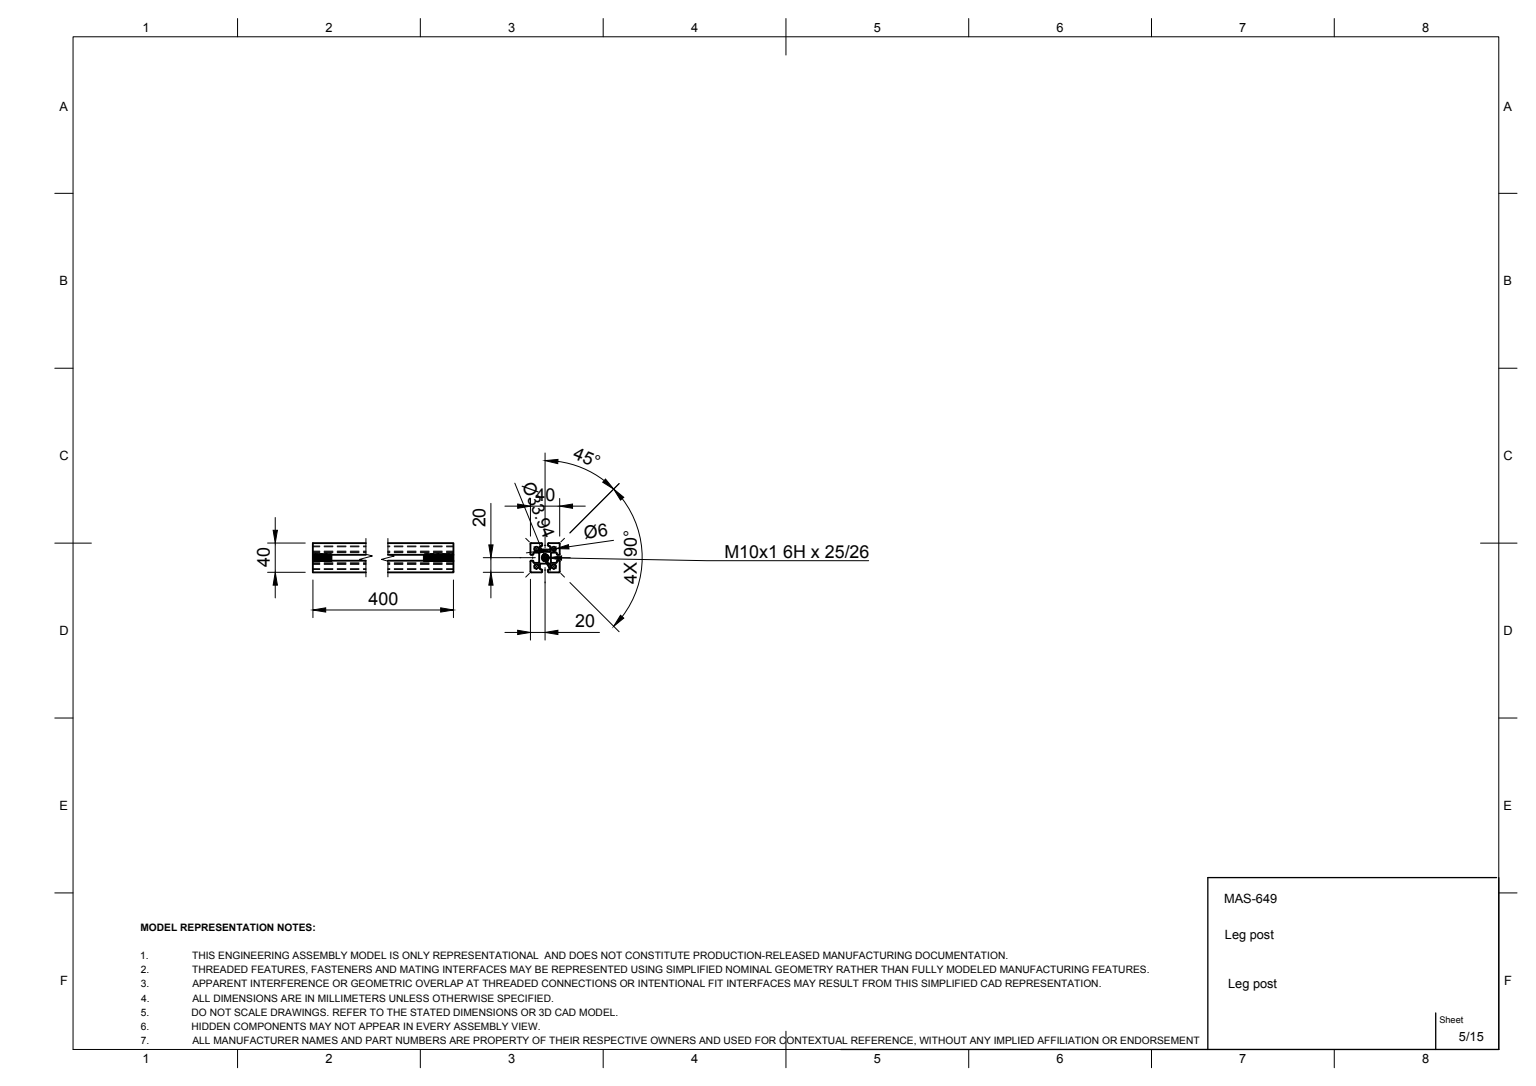
ISO-10303-21;
HEADER;
/* Generated by software containing ST-Developer
 * from STEP Tools, Inc. (www.steptools.com) 
 */

FILE_DESCRIPTION(
/* description */ ('Independent equipment support assembly with bolted 600 x 500 mm welde
d perimeter frame, four adjustable legs and swivel feet. Nominal overa
ll height 518 mm. No load rating assigned.'),
/* implementation_level */ '2;1');

FILE_NAME(
/* name */ 'Leg post.step',
/* time_stamp */ '2026-11-07T17:30:39-08:00',
/* author */ (''),
/* organization */ (''),
/* preprocessor_version */ 'ST-DEVELOPER v20.2',
/* originating_system */ 'Autodesk Translation Framework v15.17.0.0',
/* authorisation */ '');

FILE_SCHEMA (('AUTOMOTIVE_DESIGN { 1 0 10303 214 3 1 1 }'));
ENDSEC;

DATA;
#10=MECHANICAL_DESIGN_GEOMETRIC_PRESENTATION_REPRESENTATION('',(#2213),#63755);
#267=B_SPLINE_SURFACE_WITH_KNOTS('',3,3,((#36107,#36108,#36109,#36110,#36111,
#36112,#36113,#36114,#36115,#36116,#36117,#36118,#36119,#36120,#36121,#36122,
#36123,#36124,#36125,#36126,#36127,#36128,#36129,#36130,#36131,#36132,#36133,
#36134,#36135,#36136,#36137,#36138,#36139,#36140,#36141,#36142,#36143,#36144,
#36145,#36146,#36147,#36148,#36149,#36150,#36151,#36152,#36153,#36154,#36155,
#36156,#36157,#36158,#36159,#36160,#36161,#36162,#36163,#36164,#36165,#36166,
#36167,#36168,#36169,#36170,#36171,#36172,#36173,#36174,#36175,#36176,#36177,
#36178,#36179,#36180,#36181,#36182,#36183,#36184,#36185,#36186,#36187,#36188,
#36189,#36190,#36191,#36192,#36193,#36194,#36195,#36196,#36197,#36198,#36199,
#36200,#36201,#36202,#36203,#36204,#36205,#36206,#36207,#36208,#36209,#36210,
#36211,#36212,#36213,#36214,#36215,#36216,#36217,#36218,#36219,#36220,#36221,
#36222,#36223,#36224,#36225,#36226,#36227,#36228,#36229,#36230,#36231,#36232,
#36233,#36234,#36235,#36236,#36237,#36238,#36239,#36240,#36241,#36242,#36243,
#36244,#36245,#36246,#36247,#36248,#36249,#36250,#36251,#36252,#36253,#36254,
#36255,#36256,#36257,#36258,#36259,#36260,#36261,#36262,#36263,#36264,#36265,
#36266,#36267,#36268,#36269,#36270,#36271,#36272,#36273,#36274,#36275,#36276,
#36277,#36278,#36279,#36280,#36281,#36282,#36283,#36284,#36285,#36286,#36287,
#36288,#36289,#36290,#36291,#36292,#36293,#36294,#36295,#36296,#36297,#36298,
#36299,#36300,#36301,#36302,#36303,#36304,#36305,#36306,#36307,#36308,#36309,
#36310,#36311,#36312,#36313,#36314,#36315,#36316,#36317,#36318,#36319,#36320,
#36321,#36322,#36323,#36324,#36325,#36326,#36327,#36328,#36329,#36330,#36331,
#36332,#36333,#36334,#36335,#36336,#36337,#36338,#36339,#36340,#36341,#36342,
#36343,#36344,#36345,#36346,#36347,#36348,#36349,#36350,#36351,#36352,#36353,
#36354,#36355,#36356,#36357,#36358,#36359,#36360,#36361,#36362,#36363,#36364,
#36365,#36366,#36367,#36368,#36369,#36370,#36371,#36372,#36373,#36374,#36375,
#36376,#36377,#36378,#36379,#36380,#36381,#36382,#36383,#36384,#36385,#36386,
#36387,#36388,#36389,#36390,#36391,#36392,#36393,#36394,#36395,#36396,#36397,
#36398,#36399,#36400,#36401,#36402,#36403,#36404,#36405,#36406,#36407,#36408,
#36409,#36410,#36411,#36412,#36413,#36414,#36415,#36416,#36417,#36418,#36419,
#36420,#36421,#36422,#36423,#36424,#36425,#36426,#36427,#36428,#36429,#36430,
#36431,#36432,#36433,#36434,#36435,#36436,#36437,#36438,#36439,#36440,#36441,
#36442,#36443,#36444,#36445,#36446,#36447,#36448,#36449,#36450,#36451,#36452,
#36453,#36454,#36455,#36456,#36457,#36458,#36459,#36460,#36461,#36462,#36463,
#36464,#36465,#36466,#36467,#36468,#36469,#36470,#36471,#36472,#36473,#36474,
#36475,#36476,#36477,#36478,#36479,#36480,#36481,#36482,#36483,#36484,#36485,
#36486,#36487,#36488,#36489,#36490,#36491,#36492,#36493,#36494,#36495,#36496,
#36497,#36498,#36499,#36500,#36501,#36502,#36503,#36504,#36505,#36506,#36507,
#36508,#36509,#36510,#36511,#36512,#36513,#36514,#36515,#36516,#36517,#36518,
#36519,#36520,#36521,#36522,#36523,#36524,#36525,#36526,#36527,#36528,#36529,
#36530,#36531,#36532,#36533,#36534,#36535,#36536,#36537,#36538,#36539,#36540,
#36541,#36542,#36543,#36544,#36545,#36546,#36547,#36548,#36549,#36550,#36551,
#36552,#36553,#36554,#36555,#36556,#36557,#36558,#36559,#36560,#36561,#36562,
#36563,#36564,#36565,#36566,#36567,#36568,#36569,#36570,#36571,#36572,#36573,
#36574,#36575,#36576,#36577,#36578,#36579,#36580,#36581,#36582,#36583,#36584,
#36585,#36586,#36587,#36588,#36589,#36590,#36591,#36592,#36593,#36594,#36595,
#36596,#36597,#36598,#36599,#36600,#36601,#36602,#36603),(#36604,#36605,
#36606,#36607,#36608,#36609,#36610,#36611,#36612,#36613,#36614,#36615,#36616,
#36617,#36618,#36619,#36620,#36621,#36622,#36623,#36624,#36625,#36626,#36627,
#36628,#36629,#36630,#36631,#36632,#36633,#36634,#36635,#36636,#36637,#36638,
#36639,#36640,#36641,#36642,#36643,#36644,#36645,#36646,#36647,#36648,#36649,
#36650,#36651,#36652,#36653,#36654,#36655,#36656,#36657,#36658,#36659,#36660,
#36661,#36662,#36663,#36664,#36665,#36666,#36667,#36668,#36669,#36670,#36671,
#36672,#36673,#36674,#36675,#36676,#36677,#36678,#36679,#36680,#36681,#36682,
#36683,#36684,#36685,#36686,#36687,#36688,#36689,#36690,#36691,#36692,#36693,
#36694,#36695,#36696,#36697,#36698,#36699,#36700,#36701,#36702,#36703,#36704,
#36705,#36706,#36707,#36708,#36709,#36710,#36711,#36712,#36713,#36714,#36715,
#36716,#36717,#36718,#36719,#36720,#36721,#36722,#36723,#36724,#36725,#36726,
#36727,#36728,#36729,#36730,#36731,#36732,#36733,#36734,#36735,#36736,#36737,
#36738,#36739,#36740,#36741,#36742,#36743,#36744,#36745,#36746,#36747,#36748,
#36749,#36750,#36751,#36752,#36753,#36754,#36755,#36756,#36757,#36758,#36759,
#36760,#36761,#36762,#36763,#36764,#36765,#36766,#36767,#36768,#36769,#36770,
#36771,#36772,#36773,#36774,#36775,#36776,#36777,#36778,#36779,#36780,#36781,
#36782,#36783,#36784,#36785,#36786,#36787,#36788,#36789,#36790,#36791,#36792,
#36793,#36794,#36795,#36796,#36797,#36798,#36799,#36800,#36801,#36802,#36803,
#36804,#36805,#36806,#36807,#36808,#36809,#36810,#36811,#36812,#36813,#36814,
#36815,#36816,#36817,#36818,#36819,#36820,#36821,#36822,#36823,#36824,#36825,
#36826,#36827,#36828,#36829,#36830,#36831,#36832,#36833,#36834,#36835,#36836,
#36837,#36838,#36839,#36840,#36841,#36842,#36843,#36844,#36845,#36846,#36847,
#36848,#36849,#36850,#36851,#36852,#36853,#36854,#36855,#36856,#36857,#36858,
#36859,#36860,#36861,#36862,#36863,#36864,#36865,#36866,#36867,#36868,#36869,
#36870,#36871,#36872,#36873,#36874,#36875,#36876,#36877,#36878,#36879,#36880,
#36881,#36882,#36883,#36884,#36885,#36886,#36887,#36888,#36889,#36890,#36891,
#36892,#36893,#36894,#36895,#36896,#36897,#36898,#36899,#36900,#36901,#36902,
#36903,#36904,#36905,#36906,#36907,#36908,#36909,#36910,#36911,#36912,#36913,
#36914,#36915,#36916,#36917,#36918,#36919,#36920,#36921,#36922,#36923,#36924,
#36925,#36926,#36927,#36928,#36929,#36930,#36931,#36932,#36933,#36934,#36935,
#36936,#36937,#36938,#36939,#36940,#36941,#36942,#36943,#36944,#36945,#36946,
#36947,#36948,#36949,#36950,#36951,#36952,#36953,#36954,#36955,#36956,#36957,
#36958,#36959,#36960,#36961,#36962,#36963,#36964,#36965,#36966,#36967,#36968,
#36969,#36970,#36971,#36972,#36973,#36974,#36975,#36976,#36977,#36978,#36979,
#36980,#36981,#36982,#36983,#36984,#36985,#36986,#36987,#36988,#36989,#36990,
#36991,#36992,#36993,#36994,#36995,#36996,#36997,#36998,#36999,#37000,#37001,
#37002,#37003,#37004,#37005,#37006,#37007,#37008,#37009,#37010,#37011,#37012,
#37013,#37014,#37015,#37016,#37017,#37018,#37019,#37020,#37021,#37022,#37023,
#37024,#37025,#37026,#37027,#37028,#37029,#37030,#37031,#37032,#37033,#37034,
#37035,#37036,#37037,#37038,#37039,#37040,#37041,#37042,#37043,#37044,#37045,
#37046,#37047,#37048,#37049,#37050,#37051,#37052,#37053,#37054,#37055,#37056,
#37057,#37058,#37059,#37060,#37061,#37062,#37063,#37064,#37065,#37066,#37067,
#37068,#37069,#37070,#37071,#37072,#37073,#37074,#37075,#37076,#37077,#37078,
#37079,#37080,#37081,#37082,#37083,#37084,#37085,#37086,#37087,#37088,#37089,
#37090,#37091,#37092,#37093,#37094,#37095,#37096,#37097,#37098,#37099,#37100),
(#37101,#37102,#37103,#37104,#37105,#37106,#37107,#37108,#37109,#37110,
#37111,#37112,#37113,#37114,#37115,#37116,#37117,#37118,#37119,#37120,#37121,
#37122,#37123,#37124,#37125,#37126,#37127,#37128,#37129,#37130,#37131,#37132,
#37133,#37134,#37135,#37136,#37137,#37138,#37139,#37140,#37141,#37142,#37143,
#37144,#37145,#37146,#37147,#37148,#37149,#37150,#37151,#37152,#37153,#37154,
#37155,#37156,#37157,#37158,#37159,#37160,#37161,#37162,#37163,#37164,#37165,
#37166,#37167,#37168,#37169,#37170,#37171,#37172,#37173,#37174,#37175,#37176,
#37177,#37178,#37179,#37180,#37181,#37182,#37183,#37184,#37185,#37186,#37187,
#37188,#37189,#37190,#37191,#37192,#37193,#37194,#37195,#37196,#37197,#37198,
#37199,#37200,#37201,#37202,#37203,#37204,#37205,#37206,#37207,#37208,#37209,
#37210,#37211,#37212,#37213,#37214,#37215,#37216,#37217,#37218,#37219,#37220,
#37221,#37222,#37223,#37224,#37225,#37226,#37227,#37228,#37229,#37230,#37231,
#37232,#37233,#37234,#37235,#37236,#37237,#37238,#37239,#37240,#37241,#37242,
#37243,#37244,#37245,#37246,#37247,#37248,#37249,#37250,#37251,#37252,#37253,
#37254,#37255,#37256,#37257,#37258,#37259,#37260,#37261,#37262,#37263,#37264,
#37265,#37266,#37267,#37268,#37269,#37270,#37271,#37272,#37273,#37274,#37275,
#37276,#37277,#37278,#37279,#37280,#37281,#37282,#37283,#37284,#37285,#37286,
#37287,#37288,#37289,#37290,#37291,#37292,#37293,#37294,#37295,#37296,#37297,
#37298,#37299,#37300,#37301,#37302,#37303,#37304,#37305,#37306,#37307,#37308,
#37309,#37310,#37311,#37312,#37313,#37314,#37315,#37316,#37317,#37318,#37319,
#37320,#37321,#37322,#37323,#37324,#37325,#37326,#37327,#37328,#37329,#37330,
#37331,#37332,#37333,#37334,#37335,#37336,#37337,#37338,#37339,#37340,#37341,
#37342,#37343,#37344,#37345,#37346,#37347,#37348,#37349,#37350,#37351,#37352,
#37353,#37354,#37355,#37356,#37357,#37358,#37359,#37360,#37361,#37362,#37363,
#37364,#37365,#37366,#37367,#37368,#37369,#37370,#37371,#37372,#37373,#37374,
#37375,#37376,#37377,#37378,#37379,#37380,#37381,#37382,#37383,#37384,#37385,
#37386,#37387,#37388,#37389,#37390,#37391,#37392,#37393,#37394,#37395,#37396,
#37397,#37398,#37399,#37400,#37401,#37402,#37403,#37404,#37405,#37406,#37407,
#37408,#37409,#37410,#37411,#37412,#37413,#37414,#37415,#37416,#37417,#37418,
#37419,#37420,#37421,#37422,#37423,#37424,#37425,#37426,#37427,#37428,#37429,
#37430,#37431,#37432,#37433,#37434,#37435,#37436,#37437,#37438,#37439,#37440,
#37441,#37442,#37443,#37444,#37445,#37446,#37447,#37448,#37449,#37450,#37451,
#37452,#37453,#37454,#37455,#37456,#37457,#37458,#37459,#37460,#37461,#37462,
#37463,#37464,#37465,#37466,#37467,#37468,#37469,#37470,#37471,#37472,#37473,
#37474,#37475,#37476,#37477,#37478,#37479,#37480,#37481,#37482,#37483,#37484,
#37485,#37486,#37487,#37488,#37489,#37490,#37491,#37492,#37493,#37494,#37495,
#37496,#37497,#37498,#37499,#37500,#37501,#37502,#37503,#37504,#37505,#37506,
#37507,#37508,#37509,#37510,#37511,#37512,#37513,#37514,#37515,#37516,#37517,
#37518,#37519,#37520,#37521,#37522,#37523,#37524,#37525,#37526,#37527,#37528,
#37529,#37530,#37531,#37532,#37533,#37534,#37535,#37536,#37537,#37538,#37539,
#37540,#37541,#37542,#37543,#37544,#37545,#37546,#37547,#37548,#37549,#37550,
#37551,#37552,#37553,#37554,#37555,#37556,#37557,#37558,#37559,#37560,#37561,
#37562,#37563,#37564,#37565,#37566,#37567,#37568,#37569,#37570,#37571,#37572,
#37573,#37574,#37575,#37576,#37577,#37578,#37579,#37580,#37581,#37582,#37583,
#37584,#37585,#37586,#37587,#37588,#37589,#37590,#37591,#37592,#37593,#37594,
#37595,#37596,#37597),(#37598,#37599,#37600,#37601,#37602,#37603,#37604,
#37605,#37606,#37607,#37608,#37609,#37610,#37611,#37612,#37613,#37614,#37615,
#37616,#37617,#37618,#37619,#37620,#37621,#37622,#37623,#37624,#37625,#37626,
#37627,#37628,#37629,#37630,#37631,#37632,#37633,#37634,#37635,#37636,#37637,
#37638,#37639,#37640,#37641,#37642,#37643,#37644,#37645,#37646,#37647,#37648,
#37649,#37650,#37651,#37652,#37653,#37654,#37655,#37656,#37657,#37658,#37659,
#37660,#37661,#37662,#37663,#37664,#37665,#37666,#37667,#37668,#37669,#37670,
#37671,#37672,#37673,#37674,#37675,#37676,#37677,#37678,#37679,#37680,#37681,
#37682,#37683,#37684,#37685,#37686,#37687,#37688,#37689,#37690,#37691,#37692,
#37693,#37694,#37695,#37696,#37697,#37698,#37699,#37700,#37701,#37702,#37703,
#37704,#37705,#37706,#37707,#37708,#37709,#37710,#37711,#37712,#37713,#37714,
#37715,#37716,#37717,#37718,#37719,#37720,#37721,#37722,#37723,#37724,#37725,
#37726,#37727,#37728,#37729,#37730,#37731,#37732,#37733,#37734,#37735,#37736,
#37737,#37738,#37739,#37740,#37741,#37742,#37743,#37744,#37745,#37746,#37747,
#37748,#37749,#37750,#37751,#37752,#37753,#37754,#37755,#37756,#37757,#37758,
#37759,#37760,#37761,#37762,#37763,#37764,#37765,#37766,#37767,#37768,#37769,
#37770,#37771,#37772,#37773,#37774,#37775,#37776,#37777,#37778,#37779,#37780,
#37781,#37782,#37783,#37784,#37785,#37786,#37787,#37788,#37789,#37790,#37791,
#37792,#37793,#37794,#37795,#37796,#37797,#37798,#37799,#37800,#37801,#37802,
#37803,#37804,#37805,#37806,#37807,#37808,#37809,#37810,#37811,#37812,#37813,
#37814,#37815,#37816,#37817,#37818,#37819,#37820,#37821,#37822,#37823,#37824,
#37825,#37826,#37827,#37828,#37829,#37830,#37831,#37832,#37833,#37834,#37835,
#37836,#37837,#37838,#37839,#37840,#37841,#37842,#37843,#37844,#37845,#37846,
#37847,#37848,#37849,#37850,#37851,#37852,#37853,#37854,#37855,#37856,#37857,
#37858,#37859,#37860,#37861,#37862,#37863,#37864,#37865,#37866,#37867,#37868,
#37869,#37870,#37871,#37872,#37873,#37874,#37875,#37876,#37877,#37878,#37879,
#37880,#37881,#37882,#37883,#37884,#37885,#37886,#37887,#37888,#37889,#37890,
#37891,#37892,#37893,#37894,#37895,#37896,#37897,#37898,#37899,#37900,#37901,
#37902,#37903,#37904,#37905,#37906,#37907,#37908,#37909,#37910,#37911,#37912,
#37913,#37914,#37915,#37916,#37917,#37918,#37919,#37920,#37921,#37922,#37923,
#37924,#37925,#37926,#37927,#37928,#37929,#37930,#37931,#37932,#37933,#37934,
#37935,#37936,#37937,#37938,#37939,#37940,#37941,#37942,#37943,#37944,#37945,
#37946,#37947,#37948,#37949,#37950,#37951,#37952,#37953,#37954,#37955,#37956,
#37957,#37958,#37959,#37960,#37961,#37962,#37963,#37964,#37965,#37966,#37967,
#37968,#37969,#37970,#37971,#37972,#37973,#37974,#37975,#37976,#37977,#37978,
#37979,#37980,#37981,#37982,#37983,#37984,#37985,#37986,#37987,#37988,#37989,
#37990,#37991,#37992,#37993,#37994,#37995,#37996,#37997,#37998,#37999,#38000,
#38001,#38002,#38003,#38004,#38005,#38006,#38007,#38008,#38009,#38010,#38011,
#38012,#38013,#38014,#38015,#38016,#38017,#38018,#38019,#38020,#38021,#38022,
#38023,#38024,#38025,#38026,#38027,#38028,#38029,#38030,#38031,#38032,#38033,
#38034,#38035,#38036,#38037,#38038,#38039,#38040,#38041,#38042,#38043,#38044,
#38045,#38046,#38047,#38048,#38049,#38050,#38051,#38052,#38053,#38054,#38055,
#38056,#38057,#38058,#38059,#38060,#38061,#38062,#38063,#38064,#38065,#38066,
#38067,#38068,#38069,#38070,#38071,#38072,#38073,#38074,#38075,#38076,#38077,
#38078,#38079,#38080,#38081,#38082,#38083,#38084,#38085,#38086,#38087,#38088,
#38089,#38090,#38091,#38092,#38093,#38094)),.UNSPECIFIED.,.F.,.F.,.F.,(4,
4),(4,1,1,1,1,1,1,1,1,1,1,1,1,1,1,1,1,1,1,1,1,1,1,1,1,1,1,1,1,1,1,1,1,1,
1,1,1,1,1,1,1,1,1,1,1,1,1,1,1,1,1,1,1,1,1,1,1,1,1,1,1,1,1,1,1,1,1,1,1,1,
1,1,1,1,1,1,1,1,1,1,1,1,1,1,1,1,1,1,1,1,1,1,1,1,1,1,1,1,1,1,1,1,1,1,1,1,
1,1,1,1,1,1,1,1,1,1,1,1,1,1,1,1,1,1,1,1,1,1,1,1,1,1,1,1,1,1,1,1,1,1,1,1,
1,1,1,1,1,1,1,1,1,1,1,1,1,1,1,1,1,1,1,1,1,1,1,1,1,1,1,1,1,1,1,1,1,1,1,1,
1,1,1,1,1,1,1,1,1,1,1,1,1,1,1,1,1,1,1,1,1,1,1,1,1,1,1,1,1,1,1,1,1,1,1,1,
1,1,1,1,1,1,1,1,1,1,1,1,1,1,1,1,1,1,1,1,1,1,1,1,1,1,1,1,1,1,1,1,1,1,1,1,
1,1,1,1,1,1,1,1,1,1,1,1,1,1,1,1,1,1,1,1,1,1,1,1,1,1,1,1,1,1,1,1,1,1,1,1,
1,1,1,1,1,1,1,1,1,1,1,1,1,1,1,1,1,1,1,1,1,1,1,1,1,1,1,1,1,1,1,1,1,1,1,1,
1,1,1,1,1,1,1,1,1,1,1,1,1,1,1,1,1,1,1,1,1,1,1,1,1,1,1,1,1,1,1,1,1,1,1,1,
1,1,1,1,1,1,1,1,1,1,1,1,1,1,1,1,1,1,1,1,1,1,1,1,1,1,1,1,1,1,1,1,1,1,1,1,
1,1,1,1,1,1,1,1,1,1,1,1,1,1,1,1,1,1,1,1,1,1,1,1,1,1,1,1,1,1,1,1,1,1,1,1,
1,1,1,1,1,1,1,1,1,1,1,1,1,1,1,1,1,1,1,1,1,1,1,1,1,1,1,1,1,1,1,1,1,1,1,1,
1,1,1,1,1,1,1,1,1,1,1,1,1,1,1,1,1,1,1,1,1,1,1,1,1,1,1,1,4),(0.,0.0641840294258107),
(11.8589888623082,12.3576971556948,12.8564054490814,13.355113742468,13.8538220358547,
14.3525303292413,14.8512386226279,15.3499469160145,15.8486552094011,16.3473635027878,
16.8460717961744,17.344780089561,17.8434883829476,18.3421966763342,18.8409049697209,
19.3396132631075,19.8383215564941,20.3370298498807,20.8357381432673,21.334446436654,
21.8331547300406,22.3318630234272,22.8305713168138,23.3292796102004,23.8279879035871,
24.3266961969737,24.8254044903603,25.3241127837469,25.8228210771335,26.3215293705201,
26.8202376639068,27.3189459572934,27.81765425068,28.3163625440666,28.8150708374532,
29.3137791308399,29.8124874242265,30.3111957176131,30.8099040109997,31.3086123043863,
31.807320597773,32.3060288911596,32.8047371845462,33.3034454779328,33.8021537713194,
34.3008620647061,34.7995703580927,35.2982786514793,35.7969869448659,36.2956952382525,
36.7944035316392,37.2931118250258,37.7918201184124,38.290528411799,38.7892367051856,
39.2879449985723,39.7866532919589,40.2853615853455,40.7840698787321,41.2827781721187,
41.7814864655054,42.280194758892,42.7789030522786,43.2776113456652,43.7763196390518,
44.2750279324384,44.7737362258251,45.2724445192117,45.7711528125983,46.2698611059849,
46.7685693993716,47.2672776927582,47.7659859861448,48.2646942795314,48.763402572918,
49.2621108663046,49.7608191596913,50.2595274530779,50.7582357464645,51.2569440398511,
51.7556523332377,52.2543606266244,52.753068920011,53.2517772133976,53.7504855067842,
54.2491938001708,54.7479020935575,55.2466103869441,55.7453186803307,56.2440269737173,
56.7427352671039,57.2414435604906,57.7401518538772,58.2388601472638,58.7375684406504,
59.236276734037,59.7349850274237,60.2336933208103,60.7324016141969,61.2311099075835,
61.7298182009701,62.2285264943567,62.7272347877434,63.22594308113,63.7246513745166,
64.2233596679032,64.7220679612898,65.2207762546765,65.7194845480631,66.2181928414497,
66.7169011348363,67.2156094282229,67.7143177216096,68.2130260149962,68.7117343083828,
69.2104426017694,69.709150895156,70.2078591885427,70.7065674819293,71.2052757753159,
71.7039840687025,72.2026923620891,72.7014006554758,73.2001089488624,73.698817242249,
74.1975255356356,74.6962338290222,75.1949421224089,75.6936504157955,76.1923587091821,
76.6910670025687,77.1897752959553,77.6884835893419,78.1871918827286,78.6859001761152,
79.1846084695018,79.6833167628884,80.1820250562751,80.6807333496617,81.1794416430483,
81.6781499364349,82.1768582298215,82.6755665232081,83.1742748165948,83.6729831099814,
84.171691403368,84.6703996967546,85.1691079901412,85.6678162835279,86.1665245769145,
86.6652328703011,87.1639411636877,87.6626494570743,88.161357750461,88.6600660438476,
89.1587743372342,89.6574826306208,90.1561909240074,90.654899217394,91.1536075107807,
91.6523158041673,92.1510240975539,92.6497323909405,93.1484406843271,93.6471489777138,
94.1458572711004,94.644565564487,95.1432738578736,95.6419821512603,96.1406904446469,
96.6393987380335,97.1381070314201,97.6368153248067,98.1355236181933,98.63423191158,
99.1329402049666,99.6316484983532,100.13035679174,100.629065085126,101.127773378513,
101.6264816719,102.125189965286,102.623898258673,103.12260655206,103.621314845446,
104.120023138833,104.618731432219,105.117439725606,105.616148018993,106.114856312379,
106.613564605766,107.112272899152,107.610981192539,108.109689485926,108.608397779312,
109.107106072699,109.605814366086,110.104522659472,110.603230952859,111.101939246245,
111.600647539632,112.099355833019,112.598064126405,113.096772419792,113.595480713179,
114.094189006565,114.592897299952,115.091605593338,115.590313886725,116.089022180112,
116.587730473498,117.086438766885,117.585147060271,118.083855353658,118.582563647045,
119.081271940431,119.579980233818,120.078688527205,120.577396820591,121.076105113978,
121.574813407364,122.073521700751,122.572229994138,123.070938287524,123.569646580911,
124.068354874298,124.567063167684,125.065771461071,125.564479754457,126.063188047844,
126.561896341231,127.060604634617,127.559312928004,128.058021221391,128.556729514777,
129.055437808164,129.55414610155,130.052854394937,130.551562688324,131.05027098171,
131.548979275097,132.54639586187,133.543812448643,134.541229035417,135.53864562219,
136.536062208963,137.533478795736,138.53089538251,139.528311969283,140.525728556056,
141.523145142829,142.520561729602,143.517978316376,144.515394903149,145.512811489922,
146.011519783309,146.510228076695,147.008936370082,147.507644663469,148.006352956855,
148.505061250242,149.003769543629,149.502477837015,150.001186130402,150.499894423788,
150.998602717175,151.497311010562,151.996019303948,152.494727597335,152.993435890721,
153.492144184108,153.990852477495,154.489560770881,154.988269064268,155.486977357655,
155.985685651041,156.484393944428,156.983102237814,157.481810531201,157.980518824588,
158.479227117974,158.977935411361,159.476643704748,159.975351998134,160.474060291521,
160.972768584907,161.471476878294,161.970185171681,162.468893465067,162.967601758454,
163.466310051841,163.965018345227,164.463726638614,164.962434932,165.461143225387,
165.959851518774,166.45855981216,166.957268105547,167.455976398933,167.95468469232,
168.453392985707,168.952101279093,169.45080957248,169.949517865867,170.448226159253,
170.94693445264,171.445642746026,171.944351039413,172.4430593328,172.941767626186,
173.440475919573,173.93918421296,174.437892506346,174.936600799733,175.435309093119,
175.934017386506,176.432725679893,176.931433973279,177.430142266666,177.928850560052,
178.427558853439,178.926267146826,179.424975440212,179.923683733599,180.422392026986,
180.921100320372,181.419808613759,181.918516907145,182.417225200532,182.915933493919,
183.414641787305,183.913350080692,184.412058374079,184.910766667465,185.409474960852,
185.908183254238,186.406891547625,186.905599841012,187.404308134398,187.903016427785,
188.401724721171,188.900433014558,189.399141307945,189.897849601331,190.396557894718,
190.895266188105,191.393974481491,191.892682774878,192.391391068264,192.890099361651,
193.388807655038,193.887515948424,194.386224241811,194.884932535198,195.383640828584,
195.882349121971,196.381057415357,196.879765708744,197.378474002131,197.877182295517,
198.375890588904,198.87459888229,199.373307175677,199.872015469064,200.37072376245,
200.869432055837,201.368140349224,201.86684864261,202.365556935997,202.864265229383,
203.36297352277,203.861681816157,204.360390109543,204.85909840293,205.357806696317,
205.856514989703,206.35522328309,206.853931576476,207.352639869863,207.85134816325,
208.350056456636,208.848764750023,209.347473043409,209.846181336796,210.344889630183,
210.843597923569,211.342306216956,211.841014510343,212.339722803729,212.838431097116,
213.337139390502,213.835847683889,214.334555977276,214.833264270662,215.331972564049,
215.830680857436,216.329389150822,216.828097444209,217.326805737595,217.825514030982,
218.324222324369,218.822930617755,219.321638911142,219.820347204529,220.319055497915,
220.817763791302,221.316472084688,221.815180378075,222.313888671462,222.812596964848,
223.311305258235,223.810013551621,224.308721845008,224.807430138395,225.306138431781,
225.804846725168,226.303555018555,226.802263311941,227.300971605328,227.799679898714,
228.298388192101,228.797096485488,229.295804778874,229.794513072261,230.293221365647,
230.791929659034,231.290637952421,231.789346245807,232.288054539194,232.786762832581,
233.285471125967,233.784179419354,234.28288771274,234.781596006127,235.280304299514,
235.7790125929,236.277720886287,236.776429179674,237.27513747306,237.773845766447,
238.272554059833,238.77126235322,239.269970646607,239.768678939993,240.26738723338,
240.766095526767,241.264803820153,241.76351211354,242.262220406926,242.760928700313,
243.2596369937,243.758345287086,244.257053580473,244.755761873859,245.254470167246,
245.753178460633,246.251886754019,246.750595047406,247.249303340793,247.748011634179,
248.246719927566,248.745428220952,249.244136514339,249.742844807726,250.241553101112,
250.740261394499,251.238969687886,251.737677981272,252.236386274659,252.735094568045,
253.233802861432,253.732511154819,254.231219448205,254.729927741592,255.228636034978,
255.727344328365,256.226052621752,256.724760915138,257.223469208525,257.722177501912,
258.220885795298,258.719594088685,259.218302382071,259.717010675458,260.215718968845,
260.714427262231,261.213135555618,261.711843849004,262.210552142391,262.709260435778,
263.207968729164,263.706677022551,264.205385315938,264.704093609324,265.202801902711),
 .UNSPECIFIED.);
#268=B_SPLINE_SURFACE_WITH_KNOTS('',3,3,((#38244,#38245,#38246,#38247,#38248,
#38249,#38250,#38251,#38252,#38253,#38254,#38255,#38256,#38257,#38258,#38259,
#38260,#38261,#38262,#38263,#38264,#38265,#38266,#38267,#38268,#38269,#38270,
#38271,#38272,#38273,#38274,#38275,#38276,#38277,#38278,#38279,#38280,#38281,
#38282,#38283,#38284,#38285,#38286,#38287,#38288,#38289,#38290,#38291,#38292,
#38293,#38294,#38295,#38296,#38297,#38298,#38299,#38300,#38301,#38302,#38303,
#38304,#38305,#38306,#38307,#38308,#38309,#38310,#38311,#38312,#38313,#38314,
#38315,#38316,#38317,#38318,#38319,#38320,#38321,#38322,#38323,#38324,#38325,
#38326,#38327,#38328,#38329,#38330,#38331,#38332,#38333,#38334,#38335,#38336,
#38337,#38338,#38339,#38340,#38341,#38342,#38343,#38344,#38345,#38346,#38347,
#38348,#38349,#38350,#38351,#38352,#38353,#38354,#38355,#38356,#38357,#38358,
#38359,#38360,#38361,#38362,#38363,#38364,#38365,#38366,#38367,#38368,#38369,
#38370,#38371,#38372,#38373,#38374,#38375,#38376,#38377,#38378,#38379,#38380,
#38381,#38382,#38383,#38384,#38385,#38386,#38387,#38388,#38389,#38390,#38391,
#38392,#38393,#38394,#38395,#38396,#38397,#38398,#38399,#38400,#38401,#38402,
#38403,#38404,#38405,#38406,#38407,#38408,#38409,#38410,#38411,#38412,#38413,
#38414,#38415,#38416,#38417,#38418,#38419,#38420,#38421,#38422,#38423,#38424,
#38425,#38426,#38427,#38428,#38429,#38430,#38431,#38432,#38433,#38434,#38435,
#38436,#38437,#38438,#38439,#38440,#38441,#38442,#38443,#38444,#38445,#38446,
#38447,#38448,#38449,#38450,#38451,#38452,#38453,#38454,#38455,#38456,#38457,
#38458,#38459,#38460,#38461,#38462,#38463,#38464,#38465,#38466,#38467,#38468,
#38469,#38470,#38471,#38472,#38473,#38474,#38475,#38476,#38477,#38478,#38479,
#38480,#38481,#38482,#38483,#38484,#38485,#38486,#38487,#38488,#38489,#38490,
#38491,#38492,#38493,#38494,#38495,#38496,#38497,#38498,#38499,#38500,#38501,
#38502,#38503,#38504,#38505,#38506,#38507,#38508,#38509,#38510,#38511,#38512,
#38513,#38514,#38515,#38516,#38517,#38518,#38519,#38520,#38521,#38522,#38523,
#38524,#38525,#38526,#38527,#38528,#38529,#38530,#38531,#38532,#38533,#38534,
#38535,#38536,#38537,#38538,#38539,#38540,#38541,#38542,#38543,#38544,#38545,
#38546,#38547,#38548,#38549,#38550,#38551,#38552,#38553,#38554,#38555,#38556,
#38557,#38558,#38559,#38560,#38561,#38562,#38563,#38564,#38565,#38566,#38567,
#38568,#38569,#38570,#38571,#38572,#38573,#38574,#38575,#38576,#38577,#38578,
#38579,#38580,#38581,#38582,#38583,#38584,#38585,#38586,#38587,#38588,#38589,
#38590,#38591,#38592,#38593,#38594,#38595,#38596,#38597,#38598,#38599,#38600,
#38601,#38602,#38603,#38604,#38605,#38606,#38607,#38608,#38609,#38610,#38611,
#38612,#38613,#38614,#38615,#38616,#38617,#38618,#38619,#38620,#38621,#38622,
#38623,#38624,#38625,#38626,#38627,#38628,#38629,#38630,#38631,#38632,#38633,
#38634,#38635,#38636,#38637,#38638,#38639,#38640,#38641,#38642,#38643,#38644,
#38645,#38646,#38647,#38648,#38649,#38650,#38651,#38652,#38653,#38654,#38655,
#38656,#38657,#38658,#38659,#38660,#38661,#38662,#38663,#38664,#38665,#38666,
#38667,#38668,#38669,#38670,#38671,#38672,#38673,#38674,#38675,#38676,#38677,
#38678,#38679,#38680,#38681,#38682,#38683,#38684,#38685,#38686,#38687,#38688,
#38689,#38690,#38691,#38692,#38693,#38694,#38695,#38696,#38697,#38698,#38699,
#38700,#38701,#38702,#38703,#38704,#38705,#38706,#38707,#38708,#38709,#38710,
#38711,#38712,#38713,#38714,#38715,#38716,#38717,#38718,#38719,#38720,#38721,
#38722,#38723,#38724,#38725,#38726,#38727,#38728,#38729,#38730,#38731,#38732,
#38733,#38734,#38735,#38736,#38737,#38738,#38739,#38740),(#38741,#38742,
#38743,#38744,#38745,#38746,#38747,#38748,#38749,#38750,#38751,#38752,#38753,
#38754,#38755,#38756,#38757,#38758,#38759,#38760,#38761,#38762,#38763,#38764,
#38765,#38766,#38767,#38768,#38769,#38770,#38771,#38772,#38773,#38774,#38775,
#38776,#38777,#38778,#38779,#38780,#38781,#38782,#38783,#38784,#38785,#38786,
#38787,#38788,#38789,#38790,#38791,#38792,#38793,#38794,#38795,#38796,#38797,
#38798,#38799,#38800,#38801,#38802,#38803,#38804,#38805,#38806,#38807,#38808,
#38809,#38810,#38811,#38812,#38813,#38814,#38815,#38816,#38817,#38818,#38819,
#38820,#38821,#38822,#38823,#38824,#38825,#38826,#38827,#38828,#38829,#38830,
#38831,#38832,#38833,#38834,#38835,#38836,#38837,#38838,#38839,#38840,#38841,
#38842,#38843,#38844,#38845,#38846,#38847,#38848,#38849,#38850,#38851,#38852,
#38853,#38854,#38855,#38856,#38857,#38858,#38859,#38860,#38861,#38862,#38863,
#38864,#38865,#38866,#38867,#38868,#38869,#38870,#38871,#38872,#38873,#38874,
#38875,#38876,#38877,#38878,#38879,#38880,#38881,#38882,#38883,#38884,#38885,
#38886,#38887,#38888,#38889,#38890,#38891,#38892,#38893,#38894,#38895,#38896,
#38897,#38898,#38899,#38900,#38901,#38902,#38903,#38904,#38905,#38906,#38907,
#38908,#38909,#38910,#38911,#38912,#38913,#38914,#38915,#38916,#38917,#38918,
#38919,#38920,#38921,#38922,#38923,#38924,#38925,#38926,#38927,#38928,#38929,
#38930,#38931,#38932,#38933,#38934,#38935,#38936,#38937,#38938,#38939,#38940,
#38941,#38942,#38943,#38944,#38945,#38946,#38947,#38948,#38949,#38950,#38951,
#38952,#38953,#38954,#38955,#38956,#38957,#38958,#38959,#38960,#38961,#38962,
#38963,#38964,#38965,#38966,#38967,#38968,#38969,#38970,#38971,#38972,#38973,
#38974,#38975,#38976,#38977,#38978,#38979,#38980,#38981,#38982,#38983,#38984,
#38985,#38986,#38987,#38988,#38989,#38990,#38991,#38992,#38993,#38994,#38995,
#38996,#38997,#38998,#38999,#39000,#39001,#39002,#39003,#39004,#39005,#39006,
#39007,#39008,#39009,#39010,#39011,#39012,#39013,#39014,#39015,#39016,#39017,
#39018,#39019,#39020,#39021,#39022,#39023,#39024,#39025,#39026,#39027,#39028,
#39029,#39030,#39031,#39032,#39033,#39034,#39035,#39036,#39037,#39038,#39039,
#39040,#39041,#39042,#39043,#39044,#39045,#39046,#39047,#39048,#39049,#39050,
#39051,#39052,#39053,#39054,#39055,#39056,#39057,#39058,#39059,#39060,#39061,
#39062,#39063,#39064,#39065,#39066,#39067,#39068,#39069,#39070,#39071,#39072,
#39073,#39074,#39075,#39076,#39077,#39078,#39079,#39080,#39081,#39082,#39083,
#39084,#39085,#39086,#39087,#39088,#39089,#39090,#39091,#39092,#39093,#39094,
#39095,#39096,#39097,#39098,#39099,#39100,#39101,#39102,#39103,#39104,#39105,
#39106,#39107,#39108,#39109,#39110,#39111,#39112,#39113,#39114,#39115,#39116,
#39117,#39118,#39119,#39120,#39121,#39122,#39123,#39124,#39125,#39126,#39127,
#39128,#39129,#39130,#39131,#39132,#39133,#39134,#39135,#39136,#39137,#39138,
#39139,#39140,#39141,#39142,#39143,#39144,#39145,#39146,#39147,#39148,#39149,
#39150,#39151,#39152,#39153,#39154,#39155,#39156,#39157,#39158,#39159,#39160,
#39161,#39162,#39163,#39164,#39165,#39166,#39167,#39168,#39169,#39170,#39171,
#39172,#39173,#39174,#39175,#39176,#39177,#39178,#39179,#39180,#39181,#39182,
#39183,#39184,#39185,#39186,#39187,#39188,#39189,#39190,#39191,#39192,#39193,
#39194,#39195,#39196,#39197,#39198,#39199,#39200,#39201,#39202,#39203,#39204,
#39205,#39206,#39207,#39208,#39209,#39210,#39211,#39212,#39213,#39214,#39215,
#39216,#39217,#39218,#39219,#39220,#39221,#39222,#39223,#39224,#39225,#39226,
#39227,#39228,#39229,#39230,#39231,#39232,#39233,#39234,#39235,#39236,#39237),
(#39238,#39239,#39240,#39241,#39242,#39243,#39244,#39245,#39246,#39247,
#39248,#39249,#39250,#39251,#39252,#39253,#39254,#39255,#39256,#39257,#39258,
#39259,#39260,#39261,#39262,#39263,#39264,#39265,#39266,#39267,#39268,#39269,
#39270,#39271,#39272,#39273,#39274,#39275,#39276,#39277,#39278,#39279,#39280,
#39281,#39282,#39283,#39284,#39285,#39286,#39287,#39288,#39289,#39290,#39291,
#39292,#39293,#39294,#39295,#39296,#39297,#39298,#39299,#39300,#39301,#39302,
#39303,#39304,#39305,#39306,#39307,#39308,#39309,#39310,#39311,#39312,#39313,
#39314,#39315,#39316,#39317,#39318,#39319,#39320,#39321,#39322,#39323,#39324,
#39325,#39326,#39327,#39328,#39329,#39330,#39331,#39332,#39333,#39334,#39335,
#39336,#39337,#39338,#39339,#39340,#39341,#39342,#39343,#39344,#39345,#39346,
#39347,#39348,#39349,#39350,#39351,#39352,#39353,#39354,#39355,#39356,#39357,
#39358,#39359,#39360,#39361,#39362,#39363,#39364,#39365,#39366,#39367,#39368,
#39369,#39370,#39371,#39372,#39373,#39374,#39375,#39376,#39377,#39378,#39379,
#39380,#39381,#39382,#39383,#39384,#39385,#39386,#39387,#39388,#39389,#39390,
#39391,#39392,#39393,#39394,#39395,#39396,#39397,#39398,#39399,#39400,#39401,
#39402,#39403,#39404,#39405,#39406,#39407,#39408,#39409,#39410,#39411,#39412,
#39413,#39414,#39415,#39416,#39417,#39418,#39419,#39420,#39421,#39422,#39423,
#39424,#39425,#39426,#39427,#39428,#39429,#39430,#39431,#39432,#39433,#39434,
#39435,#39436,#39437,#39438,#39439,#39440,#39441,#39442,#39443,#39444,#39445,
#39446,#39447,#39448,#39449,#39450,#39451,#39452,#39453,#39454,#39455,#39456,
#39457,#39458,#39459,#39460,#39461,#39462,#39463,#39464,#39465,#39466,#39467,
#39468,#39469,#39470,#39471,#39472,#39473,#39474,#39475,#39476,#39477,#39478,
#39479,#39480,#39481,#39482,#39483,#39484,#39485,#39486,#39487,#39488,#39489,
#39490,#39491,#39492,#39493,#39494,#39495,#39496,#39497,#39498,#39499,#39500,
#39501,#39502,#39503,#39504,#39505,#39506,#39507,#39508,#39509,#39510,#39511,
#39512,#39513,#39514,#39515,#39516,#39517,#39518,#39519,#39520,#39521,#39522,
#39523,#39524,#39525,#39526,#39527,#39528,#39529,#39530,#39531,#39532,#39533,
#39534,#39535,#39536,#39537,#39538,#39539,#39540,#39541,#39542,#39543,#39544,
#39545,#39546,#39547,#39548,#39549,#39550,#39551,#39552,#39553,#39554,#39555,
#39556,#39557,#39558,#39559,#39560,#39561,#39562,#39563,#39564,#39565,#39566,
#39567,#39568,#39569,#39570,#39571,#39572,#39573,#39574,#39575,#39576,#39577,
#39578,#39579,#39580,#39581,#39582,#39583,#39584,#39585,#39586,#39587,#39588,
#39589,#39590,#39591,#39592,#39593,#39594,#39595,#39596,#39597,#39598,#39599,
#39600,#39601,#39602,#39603,#39604,#39605,#39606,#39607,#39608,#39609,#39610,
#39611,#39612,#39613,#39614,#39615,#39616,#39617,#39618,#39619,#39620,#39621,
#39622,#39623,#39624,#39625,#39626,#39627,#39628,#39629,#39630,#39631,#39632,
#39633,#39634,#39635,#39636,#39637,#39638,#39639,#39640,#39641,#39642,#39643,
#39644,#39645,#39646,#39647,#39648,#39649,#39650,#39651,#39652,#39653,#39654,
#39655,#39656,#39657,#39658,#39659,#39660,#39661,#39662,#39663,#39664,#39665,
#39666,#39667,#39668,#39669,#39670,#39671,#39672,#39673,#39674,#39675,#39676,
#39677,#39678,#39679,#39680,#39681,#39682,#39683,#39684,#39685,#39686,#39687,
#39688,#39689,#39690,#39691,#39692,#39693,#39694,#39695,#39696,#39697,#39698,
#39699,#39700,#39701,#39702,#39703,#39704,#39705,#39706,#39707,#39708,#39709,
#39710,#39711,#39712,#39713,#39714,#39715,#39716,#39717,#39718,#39719,#39720,
#39721,#39722,#39723,#39724,#39725,#39726,#39727,#39728,#39729,#39730,#39731,
#39732,#39733,#39734),(#39735,#39736,#39737,#39738,#39739,#39740,#39741,
#39742,#39743,#39744,#39745,#39746,#39747,#39748,#39749,#39750,#39751,#39752,
#39753,#39754,#39755,#39756,#39757,#39758,#39759,#39760,#39761,#39762,#39763,
#39764,#39765,#39766,#39767,#39768,#39769,#39770,#39771,#39772,#39773,#39774,
#39775,#39776,#39777,#39778,#39779,#39780,#39781,#39782,#39783,#39784,#39785,
#39786,#39787,#39788,#39789,#39790,#39791,#39792,#39793,#39794,#39795,#39796,
#39797,#39798,#39799,#39800,#39801,#39802,#39803,#39804,#39805,#39806,#39807,
#39808,#39809,#39810,#39811,#39812,#39813,#39814,#39815,#39816,#39817,#39818,
#39819,#39820,#39821,#39822,#39823,#39824,#39825,#39826,#39827,#39828,#39829,
#39830,#39831,#39832,#39833,#39834,#39835,#39836,#39837,#39838,#39839,#39840,
#39841,#39842,#39843,#39844,#39845,#39846,#39847,#39848,#39849,#39850,#39851,
#39852,#39853,#39854,#39855,#39856,#39857,#39858,#39859,#39860,#39861,#39862,
#39863,#39864,#39865,#39866,#39867,#39868,#39869,#39870,#39871,#39872,#39873,
#39874,#39875,#39876,#39877,#39878,#39879,#39880,#39881,#39882,#39883,#39884,
#39885,#39886,#39887,#39888,#39889,#39890,#39891,#39892,#39893,#39894,#39895,
#39896,#39897,#39898,#39899,#39900,#39901,#39902,#39903,#39904,#39905,#39906,
#39907,#39908,#39909,#39910,#39911,#39912,#39913,#39914,#39915,#39916,#39917,
#39918,#39919,#39920,#39921,#39922,#39923,#39924,#39925,#39926,#39927,#39928,
#39929,#39930,#39931,#39932,#39933,#39934,#39935,#39936,#39937,#39938,#39939,
#39940,#39941,#39942,#39943,#39944,#39945,#39946,#39947,#39948,#39949,#39950,
#39951,#39952,#39953,#39954,#39955,#39956,#39957,#39958,#39959,#39960,#39961,
#39962,#39963,#39964,#39965,#39966,#39967,#39968,#39969,#39970,#39971,#39972,
#39973,#39974,#39975,#39976,#39977,#39978,#39979,#39980,#39981,#39982,#39983,
#39984,#39985,#39986,#39987,#39988,#39989,#39990,#39991,#39992,#39993,#39994,
#39995,#39996,#39997,#39998,#39999,#40000,#40001,#40002,#40003,#40004,#40005,
#40006,#40007,#40008,#40009,#40010,#40011,#40012,#40013,#40014,#40015,#40016,
#40017,#40018,#40019,#40020,#40021,#40022,#40023,#40024,#40025,#40026,#40027,
#40028,#40029,#40030,#40031,#40032,#40033,#40034,#40035,#40036,#40037,#40038,
#40039,#40040,#40041,#40042,#40043,#40044,#40045,#40046,#40047,#40048,#40049,
#40050,#40051,#40052,#40053,#40054,#40055,#40056,#40057,#40058,#40059,#40060,
#40061,#40062,#40063,#40064,#40065,#40066,#40067,#40068,#40069,#40070,#40071,
#40072,#40073,#40074,#40075,#40076,#40077,#40078,#40079,#40080,#40081,#40082,
#40083,#40084,#40085,#40086,#40087,#40088,#40089,#40090,#40091,#40092,#40093,
#40094,#40095,#40096,#40097,#40098,#40099,#40100,#40101,#40102,#40103,#40104,
#40105,#40106,#40107,#40108,#40109,#40110,#40111,#40112,#40113,#40114,#40115,
#40116,#40117,#40118,#40119,#40120,#40121,#40122,#40123,#40124,#40125,#40126,
#40127,#40128,#40129,#40130,#40131,#40132,#40133,#40134,#40135,#40136,#40137,
#40138,#40139,#40140,#40141,#40142,#40143,#40144,#40145,#40146,#40147,#40148,
#40149,#40150,#40151,#40152,#40153,#40154,#40155,#40156,#40157,#40158,#40159,
#40160,#40161,#40162,#40163,#40164,#40165,#40166,#40167,#40168,#40169,#40170,
#40171,#40172,#40173,#40174,#40175,#40176,#40177,#40178,#40179,#40180,#40181,
#40182,#40183,#40184,#40185,#40186,#40187,#40188,#40189,#40190,#40191,#40192,
#40193,#40194,#40195,#40196,#40197,#40198,#40199,#40200,#40201,#40202,#40203,
#40204,#40205,#40206,#40207,#40208,#40209,#40210,#40211,#40212,#40213,#40214,
#40215,#40216,#40217,#40218,#40219,#40220,#40221,#40222,#40223,#40224,#40225,
#40226,#40227,#40228,#40229,#40230,#40231)),.UNSPECIFIED.,.F.,.F.,.F.,(4,
4),(4,1,1,1,1,1,1,1,1,1,1,1,1,1,1,1,1,1,1,1,1,1,1,1,1,1,1,1,1,1,1,1,1,1,
1,1,1,1,1,1,1,1,1,1,1,1,1,1,1,1,1,1,1,1,1,1,1,1,1,1,1,1,1,1,1,1,1,1,1,1,
1,1,1,1,1,1,1,1,1,1,1,1,1,1,1,1,1,1,1,1,1,1,1,1,1,1,1,1,1,1,1,1,1,1,1,1,
1,1,1,1,1,1,1,1,1,1,1,1,1,1,1,1,1,1,1,1,1,1,1,1,1,1,1,1,1,1,1,1,1,1,1,1,
1,1,1,1,1,1,1,1,1,1,1,1,1,1,1,1,1,1,1,1,1,1,1,1,1,1,1,1,1,1,1,1,1,1,1,1,
1,1,1,1,1,1,1,1,1,1,1,1,1,1,1,1,1,1,1,1,1,1,1,1,1,1,1,1,1,1,1,1,1,1,1,1,
1,1,1,1,1,1,1,1,1,1,1,1,1,1,1,1,1,1,1,1,1,1,1,1,1,1,1,1,1,1,1,1,1,1,1,1,
1,1,1,1,1,1,1,1,1,1,1,1,1,1,1,1,1,1,1,1,1,1,1,1,1,1,1,1,1,1,1,1,1,1,1,1,
1,1,1,1,1,1,1,1,1,1,1,1,1,1,1,1,1,1,1,1,1,1,1,1,1,1,1,1,1,1,1,1,1,1,1,1,
1,1,1,1,1,1,1,1,1,1,1,1,1,1,1,1,1,1,1,1,1,1,1,1,1,1,1,1,1,1,1,1,1,1,1,1,
1,1,1,1,1,1,1,1,1,1,1,1,1,1,1,1,1,1,1,1,1,1,1,1,1,1,1,1,1,1,1,1,1,1,1,1,
1,1,1,1,1,1,1,1,1,1,1,1,1,1,1,1,1,1,1,1,1,1,1,1,1,1,1,1,1,1,1,1,1,1,1,1,
1,1,1,1,1,1,1,1,1,1,1,1,1,1,1,1,1,1,1,1,1,1,1,1,1,1,1,1,1,1,1,1,1,1,1,1,
1,1,1,1,1,1,1,1,1,1,1,1,1,1,1,1,1,1,1,1,1,1,1,1,1,1,1,1,4),(0.,0.0641840294258107),
(14.3989442667815,14.8976525601681,15.3963608535547,15.8950691469414,16.393777440328,
16.8924857337146,17.3911940271012,17.8899023204878,18.3886106138744,18.8873189072611,
19.3860272006477,19.8847354940343,20.3834437874209,20.8821520808075,21.3808603741942,
21.8795686675808,22.3782769609674,22.876985254354,23.3756935477406,23.8744018411273,
24.3731101345139,24.8718184279005,25.3705267212871,25.8692350146737,26.3679433080604,
26.866651601447,27.3653598948336,27.8640681882202,28.3627764816068,28.8614847749935,
29.3601930683801,29.8589013617667,30.3576096551533,30.8563179485399,31.3550262419266,
31.8537345353132,32.3524428286998,32.8511511220864,33.349859415473,33.8485677088597,
34.3472760022463,34.8459842956329,35.3446925890195,35.8434008824061,36.3421091757927,
36.8408174691794,37.339525762566,37.8382340559526,38.3369423493392,38.8356506427259,
39.3343589361125,39.8330672294991,40.3317755228857,40.8304838162723,41.3291921096589,
41.8279004030456,42.3266086964322,42.8253169898188,43.3240252832054,43.822733576592,
44.3214418699787,44.8201501633653,45.3188584567519,45.8175667501385,46.3162750435251,
46.8149833369118,47.3136916302984,47.812399923685,48.3111082170716,48.8098165104582,
49.3085248038449,49.8072330972315,50.3059413906181,50.8046496840047,51.3033579773913,
51.802066270778,52.3007745641646,52.7994828575512,53.2981911509378,53.7968994443244,
54.2956077377111,54.7943160310977,55.2930243244843,55.7917326178709,56.2904409112575,
56.7891492046442,57.2878574980308,57.7865657914174,58.285274084804,58.7839823781906,
59.2826906715772,59.7813989649639,60.2801072583505,60.7788155517371,61.2775238451237,
61.7762321385104,62.274940431897,62.7736487252836,63.2723570186702,63.7710653120568,
64.2697736054434,64.7684818988301,65.2671901922167,65.7658984856033,66.2646067789899,
66.7633150723765,67.2620233657632,67.7607316591498,68.2594399525364,68.758148245923,
69.2568565393096,69.7555648326963,70.2542731260829,70.7529814194695,71.2516897128561,
71.7503980062427,72.2491062996294,72.747814593016,73.2465228864026,73.7452311797892,
74.2439394731758,74.7426477665625,75.2413560599491,75.7400643533357,76.2387726467223,
76.7374809401089,77.2361892334956,77.7348975268822,78.2336058202688,78.7323141136554,
79.231022407042,79.7297307004287,80.2284389938153,80.7271472872019,81.2258555805885,
81.7245638739751,82.2232721673618,82.7219804607484,83.220688754135,83.7193970475216,
84.2181053409082,84.7168136342949,85.2155219276815,85.7142302210681,86.2129385144547,
86.7116468078413,87.2103551012279,87.7090633946146,88.2077716880012,88.7064799813878,
89.2051882747744,89.703896568161,90.2026048615477,90.7013131549343,91.2000214483209,
91.6987297417075,92.1974380350942,92.6961463284808,93.1948546218674,93.693562915254,
94.1922712086406,94.6909795020272,95.1896877954139,95.6883960888005,96.1871043821871,
96.6858126755737,97.1845209689603,97.683229262347,98.1819375557336,98.6806458491202,
99.1793541425068,99.6780624358935,100.17677072928,100.675479022667,101.174187316053,
101.67289560944,102.171603902827,102.670312196213,103.1690204896,103.667728782986,
104.166437076373,104.66514536976,105.163853663146,105.662561956533,106.161270249919,
106.659978543306,107.158686836693,107.657395130079,108.156103423466,108.654811716853,
109.153520010239,109.652228303626,110.150936597012,110.649644890399,111.148353183786,
111.647061477172,112.145769770559,112.644478063946,113.143186357332,113.641894650719,
114.140602944105,114.639311237492,115.138019530879,115.636727824265,116.135436117652,
116.634144411039,117.132852704425,117.631560997812,118.130269291198,118.628977584585,
119.127685877972,119.626394171358,120.125102464745,120.623810758131,121.122519051518,
121.621227344905,122.119935638291,122.618643931678,123.117352225065,123.616060518451,
124.114768811838,124.613477105224,125.112185398611,125.610893691998,126.109601985384,
126.608310278771,127.107018572158,127.605726865544,128.104435158931,128.603143452317,
129.101851745704,129.600560039091,130.099268332477,130.597976625864,131.09668491925,
131.595393212637,132.094101506024,132.59280979941,133.091518092797,133.590226386184,
134.08893467957,135.086351266343,136.083767853117,137.08118443989,138.078601026663,
139.076017613436,140.07343420021,141.070850786983,142.068267373756,143.065683960529,
144.063100547303,145.060517134076,146.057933720849,147.055350307622,148.052766894396,
148.551475187782,149.050183481169,149.548891774555,150.047600067942,150.546308361329,
151.045016654715,151.543724948102,152.042433241488,152.541141534875,153.039849828262,
153.538558121648,154.037266415035,154.535974708422,155.034683001808,155.533391295195,
156.032099588581,156.530807881968,157.029516175355,157.528224468741,158.026932762128,
158.525641055515,159.024349348901,159.523057642288,160.021765935674,160.520474229061,
161.019182522448,161.517890815834,162.016599109221,162.515307402608,163.014015695994,
163.512723989381,164.011432282767,164.510140576154,165.008848869541,165.507557162927,
166.006265456314,166.5049737497,167.003682043087,167.502390336474,168.00109862986,
168.499806923247,168.998515216634,169.49722351002,169.995931803407,170.494640096793,
170.99334839018,171.492056683567,171.990764976953,172.48947327034,172.988181563726,
173.486889857113,173.9855981505,174.484306443886,174.983014737273,175.48172303066,
175.980431324046,176.479139617433,176.977847910819,177.476556204206,177.975264497593,
178.473972790979,178.972681084366,179.471389377753,179.970097671139,180.468805964526,
180.967514257912,181.466222551299,181.964930844686,182.463639138072,182.962347431459,
183.461055724845,183.959764018232,184.458472311619,184.957180605005,185.455888898392,
185.954597191779,186.453305485165,186.952013778552,187.450722071938,187.949430365325,
188.448138658712,188.946846952098,189.445555245485,189.944263538872,190.442971832258,
190.941680125645,191.440388419031,191.939096712418,192.437805005805,192.936513299191,
193.435221592578,193.933929885965,194.432638179351,194.931346472738,195.430054766124,
195.928763059511,196.427471352898,196.926179646284,197.424887939671,197.923596233057,
198.422304526444,198.921012819831,199.419721113217,199.918429406604,200.417137699991,
200.915845993377,201.414554286764,201.91326258015,202.411970873537,202.910679166924,
203.40938746031,203.908095753697,204.406804047084,204.90551234047,205.404220633857,
205.902928927243,206.40163722063,206.900345514017,207.399053807403,207.89776210079,
208.396470394177,208.895178687563,209.39388698095,209.892595274336,210.391303567723,
210.89001186111,211.388720154496,211.887428447883,212.386136741269,212.884845034656,
213.383553328043,213.882261621429,214.380969914816,214.879678208203,215.378386501589,
215.877094794976,216.375803088362,216.874511381749,217.373219675136,217.871927968522,
218.370636261909,218.869344555295,219.368052848682,219.866761142069,220.365469435455,
220.864177728842,221.362886022229,221.861594315615,222.360302609002,222.859010902388,
223.357719195775,223.856427489162,224.355135782548,224.853844075935,225.352552369322,
225.851260662708,226.349968956095,226.848677249481,227.347385542868,227.846093836255,
228.344802129641,228.843510423028,229.342218716414,229.840927009801,230.339635303188,
230.838343596574,231.337051889961,231.835760183348,232.334468476734,232.833176770121,
233.331885063507,233.830593356894,234.329301650281,234.828009943667,235.326718237054,
235.825426530441,236.324134823827,236.822843117214,237.3215514106,237.820259703987,
238.318967997374,238.81767629076,239.316384584147,239.815092877534,240.31380117092,
240.812509464307,241.311217757693,241.80992605108,242.308634344467,242.807342637853,
243.30605093124,243.804759224626,244.303467518013,244.8021758114,245.300884104786,
245.799592398173,246.29830069156,246.797008984946,247.295717278333,247.794425571719,
248.293133865106,248.791842158493,249.290550451879,249.789258745266,250.287967038653,
250.786675332039,251.285383625426,251.784091918812,252.282800212199,252.781508505586,
253.280216798972,253.778925092359,254.277633385745,254.776341679132,255.275049972519,
255.773758265905,256.272466559292,256.771174852679,257.269883146065,257.768591439452,
258.267299732838,258.766008026225,259.264716319612,259.763424612998,260.262132906385,
260.760841199772,261.259549493158,261.758257786545,262.256966079931,262.755674373318,
263.254382666705,263.753090960091,264.251799253478,264.750507546865,265.249215840251,
265.747924133638,266.246632427024,266.745340720411,267.244049013798,267.742757307184),
 .UNSPECIFIED.);
#269=B_SPLINE_SURFACE_WITH_KNOTS('',3,3,((#40624,#40625,#40626,#40627,#40628,
#40629,#40630,#40631,#40632,#40633,#40634,#40635,#40636,#40637,#40638,#40639,
#40640,#40641,#40642,#40643,#40644,#40645,#40646,#40647,#40648,#40649,#40650,
#40651,#40652,#40653,#40654,#40655,#40656,#40657,#40658,#40659,#40660,#40661,
#40662,#40663,#40664,#40665,#40666,#40667,#40668,#40669,#40670,#40671,#40672,
#40673,#40674,#40675,#40676,#40677,#40678,#40679,#40680,#40681,#40682,#40683,
#40684,#40685,#40686,#40687,#40688,#40689,#40690,#40691,#40692,#40693,#40694,
#40695,#40696,#40697,#40698,#40699,#40700,#40701,#40702,#40703,#40704,#40705,
#40706,#40707,#40708,#40709,#40710,#40711,#40712,#40713,#40714,#40715,#40716,
#40717,#40718,#40719,#40720,#40721,#40722,#40723,#40724,#40725,#40726,#40727,
#40728,#40729,#40730,#40731,#40732,#40733,#40734,#40735,#40736,#40737,#40738,
#40739,#40740,#40741,#40742,#40743,#40744,#40745,#40746,#40747,#40748,#40749,
#40750,#40751,#40752,#40753,#40754,#40755,#40756,#40757,#40758,#40759,#40760,
#40761,#40762,#40763,#40764,#40765,#40766,#40767,#40768,#40769,#40770,#40771,
#40772,#40773,#40774,#40775,#40776,#40777,#40778,#40779,#40780,#40781,#40782,
#40783,#40784,#40785,#40786,#40787,#40788,#40789,#40790,#40791,#40792,#40793,
#40794,#40795,#40796,#40797,#40798,#40799,#40800,#40801,#40802,#40803,#40804,
#40805,#40806,#40807,#40808,#40809,#40810,#40811,#40812,#40813,#40814,#40815,
#40816,#40817,#40818,#40819,#40820,#40821,#40822,#40823,#40824,#40825,#40826,
#40827,#40828,#40829,#40830,#40831,#40832,#40833,#40834,#40835,#40836,#40837,
#40838,#40839,#40840,#40841,#40842,#40843,#40844,#40845,#40846,#40847,#40848,
#40849,#40850,#40851,#40852,#40853,#40854,#40855,#40856,#40857,#40858,#40859,
#40860,#40861,#40862,#40863,#40864,#40865,#40866,#40867,#40868,#40869,#40870,
#40871,#40872,#40873,#40874,#40875,#40876,#40877,#40878,#40879,#40880,#40881,
#40882,#40883,#40884,#40885,#40886,#40887,#40888,#40889,#40890,#40891,#40892,
#40893,#40894,#40895,#40896,#40897,#40898,#40899,#40900,#40901,#40902,#40903,
#40904,#40905,#40906,#40907,#40908,#40909,#40910,#40911,#40912,#40913,#40914,
#40915,#40916,#40917,#40918,#40919,#40920,#40921,#40922,#40923,#40924,#40925,
#40926,#40927,#40928,#40929,#40930,#40931,#40932,#40933,#40934,#40935,#40936,
#40937,#40938,#40939,#40940,#40941,#40942,#40943,#40944,#40945,#40946),
(#40947,#40948,#40949,#40950,#40951,#40952,#40953,#40954,#40955,#40956,
#40957,#40958,#40959,#40960,#40961,#40962,#40963,#40964,#40965,#40966,#40967,
#40968,#40969,#40970,#40971,#40972,#40973,#40974,#40975,#40976,#40977,#40978,
#40979,#40980,#40981,#40982,#40983,#40984,#40985,#40986,#40987,#40988,#40989,
#40990,#40991,#40992,#40993,#40994,#40995,#40996,#40997,#40998,#40999,#41000,
#41001,#41002,#41003,#41004,#41005,#41006,#41007,#41008,#41009,#41010,#41011,
#41012,#41013,#41014,#41015,#41016,#41017,#41018,#41019,#41020,#41021,#41022,
#41023,#41024,#41025,#41026,#41027,#41028,#41029,#41030,#41031,#41032,#41033,
#41034,#41035,#41036,#41037,#41038,#41039,#41040,#41041,#41042,#41043,#41044,
#41045,#41046,#41047,#41048,#41049,#41050,#41051,#41052,#41053,#41054,#41055,
#41056,#41057,#41058,#41059,#41060,#41061,#41062,#41063,#41064,#41065,#41066,
#41067,#41068,#41069,#41070,#41071,#41072,#41073,#41074,#41075,#41076,#41077,
#41078,#41079,#41080,#41081,#41082,#41083,#41084,#41085,#41086,#41087,#41088,
#41089,#41090,#41091,#41092,#41093,#41094,#41095,#41096,#41097,#41098,#41099,
#41100,#41101,#41102,#41103,#41104,#41105,#41106,#41107,#41108,#41109,#41110,
#41111,#41112,#41113,#41114,#41115,#41116,#41117,#41118,#41119,#41120,#41121,
#41122,#41123,#41124,#41125,#41126,#41127,#41128,#41129,#41130,#41131,#41132,
#41133,#41134,#41135,#41136,#41137,#41138,#41139,#41140,#41141,#41142,#41143,
#41144,#41145,#41146,#41147,#41148,#41149,#41150,#41151,#41152,#41153,#41154,
#41155,#41156,#41157,#41158,#41159,#41160,#41161,#41162,#41163,#41164,#41165,
#41166,#41167,#41168,#41169,#41170,#41171,#41172,#41173,#41174,#41175,#41176,
#41177,#41178,#41179,#41180,#41181,#41182,#41183,#41184,#41185,#41186,#41187,
#41188,#41189,#41190,#41191,#41192,#41193,#41194,#41195,#41196,#41197,#41198,
#41199,#41200,#41201,#41202,#41203,#41204,#41205,#41206,#41207,#41208,#41209,
#41210,#41211,#41212,#41213,#41214,#41215,#41216,#41217,#41218,#41219,#41220,
#41221,#41222,#41223,#41224,#41225,#41226,#41227,#41228,#41229,#41230,#41231,
#41232,#41233,#41234,#41235,#41236,#41237,#41238,#41239,#41240,#41241,#41242,
#41243,#41244,#41245,#41246,#41247,#41248,#41249,#41250,#41251,#41252,#41253,
#41254,#41255,#41256,#41257,#41258,#41259,#41260,#41261,#41262,#41263,#41264,
#41265,#41266,#41267,#41268,#41269),(#41270,#41271,#41272,#41273,#41274,
#41275,#41276,#41277,#41278,#41279,#41280,#41281,#41282,#41283,#41284,#41285,
#41286,#41287,#41288,#41289,#41290,#41291,#41292,#41293,#41294,#41295,#41296,
#41297,#41298,#41299,#41300,#41301,#41302,#41303,#41304,#41305,#41306,#41307,
#41308,#41309,#41310,#41311,#41312,#41313,#41314,#41315,#41316,#41317,#41318,
#41319,#41320,#41321,#41322,#41323,#41324,#41325,#41326,#41327,#41328,#41329,
#41330,#41331,#41332,#41333,#41334,#41335,#41336,#41337,#41338,#41339,#41340,
#41341,#41342,#41343,#41344,#41345,#41346,#41347,#41348,#41349,#41350,#41351,
#41352,#41353,#41354,#41355,#41356,#41357,#41358,#41359,#41360,#41361,#41362,
#41363,#41364,#41365,#41366,#41367,#41368,#41369,#41370,#41371,#41372,#41373,
#41374,#41375,#41376,#41377,#41378,#41379,#41380,#41381,#41382,#41383,#41384,
#41385,#41386,#41387,#41388,#41389,#41390,#41391,#41392,#41393,#41394,#41395,
#41396,#41397,#41398,#41399,#41400,#41401,#41402,#41403,#41404,#41405,#41406,
#41407,#41408,#41409,#41410,#41411,#41412,#41413,#41414,#41415,#41416,#41417,
#41418,#41419,#41420,#41421,#41422,#41423,#41424,#41425,#41426,#41427,#41428,
#41429,#41430,#41431,#41432,#41433,#41434,#41435,#41436,#41437,#41438,#41439,
#41440,#41441,#41442,#41443,#41444,#41445,#41446,#41447,#41448,#41449,#41450,
#41451,#41452,#41453,#41454,#41455,#41456,#41457,#41458,#41459,#41460,#41461,
#41462,#41463,#41464,#41465,#41466,#41467,#41468,#41469,#41470,#41471,#41472,
#41473,#41474,#41475,#41476,#41477,#41478,#41479,#41480,#41481,#41482,#41483,
#41484,#41485,#41486,#41487,#41488,#41489,#41490,#41491,#41492,#41493,#41494,
#41495,#41496,#41497,#41498,#41499,#41500,#41501,#41502,#41503,#41504,#41505,
#41506,#41507,#41508,#41509,#41510,#41511,#41512,#41513,#41514,#41515,#41516,
#41517,#41518,#41519,#41520,#41521,#41522,#41523,#41524,#41525,#41526,#41527,
#41528,#41529,#41530,#41531,#41532,#41533,#41534,#41535,#41536,#41537,#41538,
#41539,#41540,#41541,#41542,#41543,#41544,#41545,#41546,#41547,#41548,#41549,
#41550,#41551,#41552,#41553,#41554,#41555,#41556,#41557,#41558,#41559,#41560,
#41561,#41562,#41563,#41564,#41565,#41566,#41567,#41568,#41569,#41570,#41571,
#41572,#41573,#41574,#41575,#41576,#41577,#41578,#41579,#41580,#41581,#41582,
#41583,#41584,#41585,#41586,#41587,#41588,#41589,#41590,#41591,#41592),
(#41593,#41594,#41595,#41596,#41597,#41598,#41599,#41600,#41601,#41602,
#41603,#41604,#41605,#41606,#41607,#41608,#41609,#41610,#41611,#41612,#41613,
#41614,#41615,#41616,#41617,#41618,#41619,#41620,#41621,#41622,#41623,#41624,
#41625,#41626,#41627,#41628,#41629,#41630,#41631,#41632,#41633,#41634,#41635,
#41636,#41637,#41638,#41639,#41640,#41641,#41642,#41643,#41644,#41645,#41646,
#41647,#41648,#41649,#41650,#41651,#41652,#41653,#41654,#41655,#41656,#41657,
#41658,#41659,#41660,#41661,#41662,#41663,#41664,#41665,#41666,#41667,#41668,
#41669,#41670,#41671,#41672,#41673,#41674,#41675,#41676,#41677,#41678,#41679,
#41680,#41681,#41682,#41683,#41684,#41685,#41686,#41687,#41688,#41689,#41690,
#41691,#41692,#41693,#41694,#41695,#41696,#41697,#41698,#41699,#41700,#41701,
#41702,#41703,#41704,#41705,#41706,#41707,#41708,#41709,#41710,#41711,#41712,
#41713,#41714,#41715,#41716,#41717,#41718,#41719,#41720,#41721,#41722,#41723,
#41724,#41725,#41726,#41727,#41728,#41729,#41730,#41731,#41732,#41733,#41734,
#41735,#41736,#41737,#41738,#41739,#41740,#41741,#41742,#41743,#41744,#41745,
#41746,#41747,#41748,#41749,#41750,#41751,#41752,#41753,#41754,#41755,#41756,
#41757,#41758,#41759,#41760,#41761,#41762,#41763,#41764,#41765,#41766,#41767,
#41768,#41769,#41770,#41771,#41772,#41773,#41774,#41775,#41776,#41777,#41778,
#41779,#41780,#41781,#41782,#41783,#41784,#41785,#41786,#41787,#41788,#41789,
#41790,#41791,#41792,#41793,#41794,#41795,#41796,#41797,#41798,#41799,#41800,
#41801,#41802,#41803,#41804,#41805,#41806,#41807,#41808,#41809,#41810,#41811,
#41812,#41813,#41814,#41815,#41816,#41817,#41818,#41819,#41820,#41821,#41822,
#41823,#41824,#41825,#41826,#41827,#41828,#41829,#41830,#41831,#41832,#41833,
#41834,#41835,#41836,#41837,#41838,#41839,#41840,#41841,#41842,#41843,#41844,
#41845,#41846,#41847,#41848,#41849,#41850,#41851,#41852,#41853,#41854,#41855,
#41856,#41857,#41858,#41859,#41860,#41861,#41862,#41863,#41864,#41865,#41866,
#41867,#41868,#41869,#41870,#41871,#41872,#41873,#41874,#41875,#41876,#41877,
#41878,#41879,#41880,#41881,#41882,#41883,#41884,#41885,#41886,#41887,#41888,
#41889,#41890,#41891,#41892,#41893,#41894,#41895,#41896,#41897,#41898,#41899,
#41900,#41901,#41902,#41903,#41904,#41905,#41906,#41907,#41908,#41909,#41910,
#41911,#41912,#41913,#41914,#41915)),.UNSPECIFIED.,.F.,.F.,.F.,(4,4),(4,
1,1,1,1,1,1,1,1,1,1,1,1,1,1,1,1,1,1,1,1,1,1,1,1,1,1,1,1,1,1,1,1,1,1,1,1,
1,1,1,1,1,1,1,1,1,1,1,1,1,1,1,1,1,1,1,1,1,1,1,1,1,1,1,1,1,1,1,1,1,1,1,1,
1,1,1,1,1,1,1,1,1,1,1,1,1,1,1,1,1,1,1,1,1,1,1,1,1,1,1,1,1,1,1,1,1,1,1,1,
1,1,1,1,1,1,1,1,1,1,1,1,1,1,1,1,1,1,1,1,1,1,1,1,1,1,1,1,1,1,1,1,1,1,1,1,
1,1,1,1,1,1,1,1,1,1,1,1,1,1,1,1,1,1,1,1,1,1,1,1,1,1,1,1,1,1,1,1,1,1,1,1,
1,1,1,1,1,1,1,1,1,1,1,1,1,1,1,1,1,1,1,1,1,1,1,1,1,1,1,1,1,1,1,1,1,1,1,1,
1,1,1,1,1,1,1,1,1,1,1,1,1,1,1,1,1,1,1,1,1,1,1,1,1,1,1,1,1,1,1,1,1,1,1,1,
1,1,1,1,1,1,1,1,1,1,1,1,1,1,1,1,1,1,1,1,1,1,1,1,1,1,1,1,1,1,1,1,1,1,1,1,
1,1,1,1,1,1,1,1,1,1,1,1,1,1,1,1,1,1,1,1,1,1,1,1,1,1,1,1,1,1,1,4),(0.,0.0641840294258124),
(11.8589888623079,12.3561639667852,12.8533390712624,13.3505141757396,13.8476892802168,
14.344864384694,14.8420394891712,15.3392145936484,15.8363896981257,16.3335648026029,
16.8307399070801,17.3279150115573,17.8250901160345,18.3222652205117,18.8194403249889,
19.3166154294662,19.8137905339434,20.3109656384206,20.8081407428978,21.305315847375,
21.8024909518522,22.2996660563294,22.7968411608067,23.2940162652839,23.7911913697611,
24.2883664742383,24.7855415787155,25.2827166831927,25.7798917876699,26.2770668921472,
26.7742419966244,27.2714171011016,27.7685922055788,28.265767310056,28.7629424145332,
29.2601175190104,29.7572926234877,30.2544677279649,30.7516428324421,31.2488179369193,
31.7459930413965,32.2431681458737,32.7403432503509,33.2375183548282,33.7346934593054,
34.2318685637826,34.7290436682598,35.226218772737,35.7233938772142,36.2205689816915,
36.7177440861687,37.2149191906459,37.7120942951231,38.2092693996003,38.7064445040775,
39.2036196085547,39.700794713032,40.1979698175092,40.6951449219864,41.1923200264636,
41.6894951309408,42.186670235418,42.6838453398952,43.1810204443725,43.6781955488497,
44.1753706533269,44.6725457578041,45.1697208622813,45.6668959667585,46.1640710712357,
46.661246175713,47.1584212801902,47.6555963846674,48.1527714891446,48.6499465936218,
49.147121698099,49.6442968025762,50.1414719070535,50.6386470115307,51.1358221160079,
51.6329972204851,52.1301723249623,52.6273474294395,53.1245225339167,53.621697638394,
54.1188727428712,54.6160478473484,55.1132229518256,55.6103980563028,56.10757316078,
56.6047482652572,57.1019233697345,57.5990984742117,58.0962735786889,58.5934486831661,
59.0906237876433,59.5877988921205,60.0849739965977,60.582149101075,61.0793242055522,
61.5764993100294,62.0736744145066,62.5708495189838,63.068024623461,63.5651997279382,
64.0623748324155,64.5595499368927,65.0567250413699,65.5539001458471,66.0510752503243,
66.5482503548015,67.0454254592788,67.542600563756,68.0397756682332,68.5369507727104,
69.0341258771876,69.5313009816648,70.028476086142,70.5256511906192,71.0228262950965,
71.5200013995737,72.0171765040509,72.5143516085281,73.0115267130053,73.5087018174825,
74.0058769219598,74.503052026437,75.0002271309142,75.4974022353914,75.9945773398686,
76.4917524443458,76.988927548823,77.4861026533003,77.9832777577775,78.4804528622547,
78.9776279667319,79.4748030712091,79.9719781756863,80.4691532801635,80.9663283846407,
81.463503489118,81.9606785935952,82.4578536980724,82.9550288025496,83.4522039070268,
83.949379011504,84.4465541159813,84.9437292204585,85.4409043249357,85.9380794294129,
86.4352545338901,86.9324296383673,87.4296047428445,87.9267798473217,88.423954951799,
88.9211300562762,89.4183051607534,89.9154802652306,90.4126553697078,90.909830474185,
91.4070055786623,91.9041806831395,92.4013557876167,92.8985308920939,93.3957059965711,
93.8928811010483,94.3900562055255,94.8872313100028,95.38440641448,95.8815815189572,
96.3787566234344,96.8759317279116,97.3731068323888,97.870281936866,98.3674570413433,
98.8646321458205,99.3618072502977,99.8589823547749,100.356157459252,100.853332563729,
101.350507668207,101.847682772684,102.344857877161,102.842032981638,103.339208086115,
103.836383190593,104.33355829507,104.830733399547,105.327908504024,105.825083608501,
106.322258712979,106.819433817456,107.316608921933,107.81378402641,108.310959130888,
108.808134235365,109.305309339842,109.802484444319,110.299659548796,110.796834653274,
111.294009757751,111.791184862228,112.288359966705,112.785535071182,113.28271017566,
113.779885280137,114.277060384614,114.774235489091,115.271410593569,115.768585698046,
116.265760802523,116.762935907,117.260111011477,117.757286115955,118.254461220432,
118.751636324909,119.248811429386,119.745986533863,120.243161638341,120.740336742818,
121.237511847295,121.734686951772,122.23186205625,122.729037160727,123.226212265204,
123.723387369681,124.220562474158,124.717737578636,125.214912683113,125.71208778759,
126.209262892067,126.706437996544,127.203613101022,127.700788205499,128.197963309976,
128.695138414453,129.192313518931,129.689488623408,130.186663727885,130.683838832362,
131.181013936839,131.678189041317,132.175364145794,132.672539250271,133.169714354748,
133.666889459226,134.164064563703,134.66123966818,135.158414772657,135.655589877134,
136.152764981612,136.649940086089,137.147115190566,137.644290295043,138.14146539952,
138.638640503998,139.135815608475,139.632990712952,140.130165817429,140.627340921906,
141.124516026384,141.621691130861,142.118866235338,142.616041339815,143.113216444293,
143.61039154877,144.107566653247,144.604741757724,145.101916862201,145.599091966679,
146.096267071156,146.593442175633,147.09061728011,147.587792384587,148.084967489065,
148.582142593542,149.079317698019,149.576492802496,150.073667906974,150.570843011451,
151.068018115928,151.565193220405,152.062368324882,152.55954342936,153.056718533837,
153.553893638314,154.051068742791,154.548243847269,155.045418951746,155.542594056223,
156.0397691607,156.536944265177,157.034119369655,157.531294474132,158.028469578609,
158.525644683086,159.022819787563,159.519994892041,160.017169996518,160.514345100995,
161.011520205472,161.508695309949,162.005870414427,162.503045518904,163.000220623381,
163.497395727858,163.994570832336,164.491745936813,164.98892104129,165.486096145767,
165.983271250244,166.480446354722,166.977621459199,167.474796563676,167.971971668153,
168.46914677263,168.966321877108,169.463496981585,169.960672086062,170.457847190539,
170.955022295017),.UNSPECIFIED.);
#270=B_SPLINE_SURFACE_WITH_KNOTS('',3,3,((#42065,#42066,#42067,#42068,#42069,
#42070,#42071,#42072,#42073,#42074,#42075,#42076,#42077,#42078,#42079,#42080,
#42081,#42082,#42083,#42084,#42085,#42086,#42087,#42088,#42089,#42090,#42091,
#42092,#42093,#42094,#42095,#42096,#42097,#42098,#42099,#42100,#42101,#42102,
#42103,#42104,#42105,#42106,#42107,#42108,#42109,#42110,#42111,#42112,#42113,
#42114,#42115,#42116,#42117,#42118,#42119,#42120,#42121,#42122,#42123,#42124,
#42125,#42126,#42127,#42128,#42129,#42130,#42131,#42132,#42133,#42134,#42135,
#42136,#42137,#42138,#42139,#42140,#42141,#42142,#42143,#42144,#42145,#42146,
#42147,#42148,#42149,#42150,#42151,#42152,#42153,#42154,#42155,#42156,#42157,
#42158,#42159,#42160,#42161,#42162,#42163,#42164,#42165,#42166,#42167,#42168,
#42169,#42170,#42171,#42172,#42173,#42174,#42175,#42176,#42177,#42178,#42179,
#42180,#42181,#42182,#42183,#42184,#42185,#42186,#42187,#42188,#42189,#42190,
#42191,#42192,#42193,#42194,#42195,#42196,#42197,#42198,#42199,#42200,#42201,
#42202,#42203,#42204,#42205,#42206,#42207,#42208,#42209,#42210,#42211,#42212,
#42213,#42214,#42215,#42216,#42217,#42218,#42219,#42220,#42221,#42222,#42223,
#42224,#42225,#42226,#42227,#42228,#42229,#42230,#42231,#42232,#42233,#42234,
#42235,#42236,#42237,#42238,#42239,#42240,#42241,#42242,#42243,#42244,#42245,
#42246,#42247,#42248,#42249,#42250,#42251,#42252,#42253,#42254,#42255,#42256,
#42257,#42258,#42259,#42260,#42261,#42262,#42263,#42264,#42265,#42266,#42267,
#42268,#42269,#42270,#42271,#42272,#42273,#42274,#42275,#42276,#42277,#42278,
#42279,#42280,#42281,#42282,#42283,#42284,#42285,#42286,#42287,#42288,#42289,
#42290,#42291,#42292,#42293,#42294,#42295,#42296,#42297,#42298,#42299,#42300,
#42301,#42302,#42303,#42304,#42305,#42306,#42307,#42308,#42309,#42310,#42311,
#42312,#42313,#42314,#42315,#42316,#42317,#42318,#42319,#42320,#42321,#42322,
#42323,#42324,#42325,#42326,#42327,#42328,#42329,#42330,#42331,#42332,#42333,
#42334,#42335,#42336,#42337,#42338,#42339,#42340,#42341,#42342,#42343,#42344,
#42345,#42346,#42347,#42348,#42349,#42350,#42351,#42352,#42353,#42354,#42355,
#42356,#42357,#42358,#42359,#42360,#42361,#42362,#42363,#42364,#42365,#42366,
#42367,#42368,#42369,#42370,#42371,#42372,#42373,#42374,#42375,#42376,#42377,
#42378,#42379,#42380,#42381,#42382,#42383,#42384,#42385,#42386,#42387),
(#42388,#42389,#42390,#42391,#42392,#42393,#42394,#42395,#42396,#42397,
#42398,#42399,#42400,#42401,#42402,#42403,#42404,#42405,#42406,#42407,#42408,
#42409,#42410,#42411,#42412,#42413,#42414,#42415,#42416,#42417,#42418,#42419,
#42420,#42421,#42422,#42423,#42424,#42425,#42426,#42427,#42428,#42429,#42430,
#42431,#42432,#42433,#42434,#42435,#42436,#42437,#42438,#42439,#42440,#42441,
#42442,#42443,#42444,#42445,#42446,#42447,#42448,#42449,#42450,#42451,#42452,
#42453,#42454,#42455,#42456,#42457,#42458,#42459,#42460,#42461,#42462,#42463,
#42464,#42465,#42466,#42467,#42468,#42469,#42470,#42471,#42472,#42473,#42474,
#42475,#42476,#42477,#42478,#42479,#42480,#42481,#42482,#42483,#42484,#42485,
#42486,#42487,#42488,#42489,#42490,#42491,#42492,#42493,#42494,#42495,#42496,
#42497,#42498,#42499,#42500,#42501,#42502,#42503,#42504,#42505,#42506,#42507,
#42508,#42509,#42510,#42511,#42512,#42513,#42514,#42515,#42516,#42517,#42518,
#42519,#42520,#42521,#42522,#42523,#42524,#42525,#42526,#42527,#42528,#42529,
#42530,#42531,#42532,#42533,#42534,#42535,#42536,#42537,#42538,#42539,#42540,
#42541,#42542,#42543,#42544,#42545,#42546,#42547,#42548,#42549,#42550,#42551,
#42552,#42553,#42554,#42555,#42556,#42557,#42558,#42559,#42560,#42561,#42562,
#42563,#42564,#42565,#42566,#42567,#42568,#42569,#42570,#42571,#42572,#42573,
#42574,#42575,#42576,#42577,#42578,#42579,#42580,#42581,#42582,#42583,#42584,
#42585,#42586,#42587,#42588,#42589,#42590,#42591,#42592,#42593,#42594,#42595,
#42596,#42597,#42598,#42599,#42600,#42601,#42602,#42603,#42604,#42605,#42606,
#42607,#42608,#42609,#42610,#42611,#42612,#42613,#42614,#42615,#42616,#42617,
#42618,#42619,#42620,#42621,#42622,#42623,#42624,#42625,#42626,#42627,#42628,
#42629,#42630,#42631,#42632,#42633,#42634,#42635,#42636,#42637,#42638,#42639,
#42640,#42641,#42642,#42643,#42644,#42645,#42646,#42647,#42648,#42649,#42650,
#42651,#42652,#42653,#42654,#42655,#42656,#42657,#42658,#42659,#42660,#42661,
#42662,#42663,#42664,#42665,#42666,#42667,#42668,#42669,#42670,#42671,#42672,
#42673,#42674,#42675,#42676,#42677,#42678,#42679,#42680,#42681,#42682,#42683,
#42684,#42685,#42686,#42687,#42688,#42689,#42690,#42691,#42692,#42693,#42694,
#42695,#42696,#42697,#42698,#42699,#42700,#42701,#42702,#42703,#42704,#42705,
#42706,#42707,#42708,#42709,#42710),(#42711,#42712,#42713,#42714,#42715,
#42716,#42717,#42718,#42719,#42720,#42721,#42722,#42723,#42724,#42725,#42726,
#42727,#42728,#42729,#42730,#42731,#42732,#42733,#42734,#42735,#42736,#42737,
#42738,#42739,#42740,#42741,#42742,#42743,#42744,#42745,#42746,#42747,#42748,
#42749,#42750,#42751,#42752,#42753,#42754,#42755,#42756,#42757,#42758,#42759,
#42760,#42761,#42762,#42763,#42764,#42765,#42766,#42767,#42768,#42769,#42770,
#42771,#42772,#42773,#42774,#42775,#42776,#42777,#42778,#42779,#42780,#42781,
#42782,#42783,#42784,#42785,#42786,#42787,#42788,#42789,#42790,#42791,#42792,
#42793,#42794,#42795,#42796,#42797,#42798,#42799,#42800,#42801,#42802,#42803,
#42804,#42805,#42806,#42807,#42808,#42809,#42810,#42811,#42812,#42813,#42814,
#42815,#42816,#42817,#42818,#42819,#42820,#42821,#42822,#42823,#42824,#42825,
#42826,#42827,#42828,#42829,#42830,#42831,#42832,#42833,#42834,#42835,#42836,
#42837,#42838,#42839,#42840,#42841,#42842,#42843,#42844,#42845,#42846,#42847,
#42848,#42849,#42850,#42851,#42852,#42853,#42854,#42855,#42856,#42857,#42858,
#42859,#42860,#42861,#42862,#42863,#42864,#42865,#42866,#42867,#42868,#42869,
#42870,#42871,#42872,#42873,#42874,#42875,#42876,#42877,#42878,#42879,#42880,
#42881,#42882,#42883,#42884,#42885,#42886,#42887,#42888,#42889,#42890,#42891,
#42892,#42893,#42894,#42895,#42896,#42897,#42898,#42899,#42900,#42901,#42902,
#42903,#42904,#42905,#42906,#42907,#42908,#42909,#42910,#42911,#42912,#42913,
#42914,#42915,#42916,#42917,#42918,#42919,#42920,#42921,#42922,#42923,#42924,
#42925,#42926,#42927,#42928,#42929,#42930,#42931,#42932,#42933,#42934,#42935,
#42936,#42937,#42938,#42939,#42940,#42941,#42942,#42943,#42944,#42945,#42946,
#42947,#42948,#42949,#42950,#42951,#42952,#42953,#42954,#42955,#42956,#42957,
#42958,#42959,#42960,#42961,#42962,#42963,#42964,#42965,#42966,#42967,#42968,
#42969,#42970,#42971,#42972,#42973,#42974,#42975,#42976,#42977,#42978,#42979,
#42980,#42981,#42982,#42983,#42984,#42985,#42986,#42987,#42988,#42989,#42990,
#42991,#42992,#42993,#42994,#42995,#42996,#42997,#42998,#42999,#43000,#43001,
#43002,#43003,#43004,#43005,#43006,#43007,#43008,#43009,#43010,#43011,#43012,
#43013,#43014,#43015,#43016,#43017,#43018,#43019,#43020,#43021,#43022,#43023,
#43024,#43025,#43026,#43027,#43028,#43029,#43030,#43031,#43032,#43033),
(#43034,#43035,#43036,#43037,#43038,#43039,#43040,#43041,#43042,#43043,
#43044,#43045,#43046,#43047,#43048,#43049,#43050,#43051,#43052,#43053,#43054,
#43055,#43056,#43057,#43058,#43059,#43060,#43061,#43062,#43063,#43064,#43065,
#43066,#43067,#43068,#43069,#43070,#43071,#43072,#43073,#43074,#43075,#43076,
#43077,#43078,#43079,#43080,#43081,#43082,#43083,#43084,#43085,#43086,#43087,
#43088,#43089,#43090,#43091,#43092,#43093,#43094,#43095,#43096,#43097,#43098,
#43099,#43100,#43101,#43102,#43103,#43104,#43105,#43106,#43107,#43108,#43109,
#43110,#43111,#43112,#43113,#43114,#43115,#43116,#43117,#43118,#43119,#43120,
#43121,#43122,#43123,#43124,#43125,#43126,#43127,#43128,#43129,#43130,#43131,
#43132,#43133,#43134,#43135,#43136,#43137,#43138,#43139,#43140,#43141,#43142,
#43143,#43144,#43145,#43146,#43147,#43148,#43149,#43150,#43151,#43152,#43153,
#43154,#43155,#43156,#43157,#43158,#43159,#43160,#43161,#43162,#43163,#43164,
#43165,#43166,#43167,#43168,#43169,#43170,#43171,#43172,#43173,#43174,#43175,
#43176,#43177,#43178,#43179,#43180,#43181,#43182,#43183,#43184,#43185,#43186,
#43187,#43188,#43189,#43190,#43191,#43192,#43193,#43194,#43195,#43196,#43197,
#43198,#43199,#43200,#43201,#43202,#43203,#43204,#43205,#43206,#43207,#43208,
#43209,#43210,#43211,#43212,#43213,#43214,#43215,#43216,#43217,#43218,#43219,
#43220,#43221,#43222,#43223,#43224,#43225,#43226,#43227,#43228,#43229,#43230,
#43231,#43232,#43233,#43234,#43235,#43236,#43237,#43238,#43239,#43240,#43241,
#43242,#43243,#43244,#43245,#43246,#43247,#43248,#43249,#43250,#43251,#43252,
#43253,#43254,#43255,#43256,#43257,#43258,#43259,#43260,#43261,#43262,#43263,
#43264,#43265,#43266,#43267,#43268,#43269,#43270,#43271,#43272,#43273,#43274,
#43275,#43276,#43277,#43278,#43279,#43280,#43281,#43282,#43283,#43284,#43285,
#43286,#43287,#43288,#43289,#43290,#43291,#43292,#43293,#43294,#43295,#43296,
#43297,#43298,#43299,#43300,#43301,#43302,#43303,#43304,#43305,#43306,#43307,
#43308,#43309,#43310,#43311,#43312,#43313,#43314,#43315,#43316,#43317,#43318,
#43319,#43320,#43321,#43322,#43323,#43324,#43325,#43326,#43327,#43328,#43329,
#43330,#43331,#43332,#43333,#43334,#43335,#43336,#43337,#43338,#43339,#43340,
#43341,#43342,#43343,#43344,#43345,#43346,#43347,#43348,#43349,#43350,#43351,
#43352,#43353,#43354,#43355,#43356)),.UNSPECIFIED.,.F.,.F.,.F.,(4,4),(4,
1,1,1,1,1,1,1,1,1,1,1,1,1,1,1,1,1,1,1,1,1,1,1,1,1,1,1,1,1,1,1,1,1,1,1,1,
1,1,1,1,1,1,1,1,1,1,1,1,1,1,1,1,1,1,1,1,1,1,1,1,1,1,1,1,1,1,1,1,1,1,1,1,
1,1,1,1,1,1,1,1,1,1,1,1,1,1,1,1,1,1,1,1,1,1,1,1,1,1,1,1,1,1,1,1,1,1,1,1,
1,1,1,1,1,1,1,1,1,1,1,1,1,1,1,1,1,1,1,1,1,1,1,1,1,1,1,1,1,1,1,1,1,1,1,1,
1,1,1,1,1,1,1,1,1,1,1,1,1,1,1,1,1,1,1,1,1,1,1,1,1,1,1,1,1,1,1,1,1,1,1,1,
1,1,1,1,1,1,1,1,1,1,1,1,1,1,1,1,1,1,1,1,1,1,1,1,1,1,1,1,1,1,1,1,1,1,1,1,
1,1,1,1,1,1,1,1,1,1,1,1,1,1,1,1,1,1,1,1,1,1,1,1,1,1,1,1,1,1,1,1,1,1,1,1,
1,1,1,1,1,1,1,1,1,1,1,1,1,1,1,1,1,1,1,1,1,1,1,1,1,1,1,1,1,1,1,1,1,1,1,1,
1,1,1,1,1,1,1,1,1,1,1,1,1,1,1,1,1,1,1,1,1,1,1,1,1,1,1,1,1,1,1,4),(0.,0.0641840294258124),
(14.398944266781,14.8961193712582,15.3932944757354,15.8904695802126,16.3876446846898,
16.884819789167,17.3819948936443,17.8791699981215,18.3763451025987,18.8735202070759,
19.3706953115531,19.8678704160303,20.3650455205075,20.8622206249848,21.359395729462,
21.8565708339392,22.3537459384164,22.8509210428936,23.3480961473708,23.845271251848,
24.3424463563253,24.8396214608025,25.3367965652797,25.8339716697569,26.3311467742341,
26.8283218787113,27.3254969831885,27.8226720876658,28.319847192143,28.8170222966202,
29.3141974010974,29.8113725055746,30.3085476100518,30.805722714529,31.3028978190063,
31.8000729234835,32.2972480279607,32.7944231324379,33.2915982369151,33.7887733413923,
34.2859484458695,34.7831235503468,35.280298654824,35.7774737593012,36.2746488637784,
36.7718239682556,37.2689990727328,37.76617417721,38.2633492816873,38.7605243861645,
39.2576994906417,39.7548745951189,40.2520496995961,40.7492248040733,41.2463999085505,
41.7435750130278,42.240750117505,42.7379252219822,43.2351003264594,43.7322754309366,
44.2294505354138,44.726625639891,45.2238007443683,45.7209758488455,46.2181509533227,
46.7153260577999,47.2125011622771,47.7096762667543,48.2068513712315,48.7040264757088,
49.201201580186,49.6983766846632,50.1955517891404,50.6927268936176,51.1899019980948,
51.687077102572,52.1842522070493,52.6814273115265,53.1786024160037,53.6757775204809,
54.1729526249581,54.6701277294353,55.1673028339125,55.6644779383898,56.161653042867,
56.6588281473442,57.1560032518214,57.6531783562986,58.1503534607758,58.647528565253,
59.1447036697303,59.6418787742075,60.1390538786847,60.6362289831619,61.1334040876391,
61.6305791921163,62.1277542965935,62.6249294010708,63.122104505548,63.6192796100252,
64.1164547145024,64.6136298189796,65.1108049234568,65.607980027934,66.1051551324113,
66.6023302368885,67.0995053413657,67.5966804458429,68.0938555503201,68.5910306547973,
69.0882057592745,69.5853808637518,70.082555968229,70.5797310727062,71.0769061771834,
71.5740812816606,72.0712563861378,72.568431490615,73.0656065950923,73.5627816995695,
74.0599568040467,74.5571319085239,75.0543070130011,75.5514821174783,76.0486572219556,
76.5458323264328,77.04300743091,77.5401825353872,78.0373576398644,78.5345327443416,
79.0317078488188,79.528882953296,80.0260580577733,80.5232331622505,81.0204082667277,
81.5175833712049,82.0147584756821,82.5119335801593,83.0091086846365,83.5062837891138,
84.003458893591,84.5006339980682,84.9978091025454,85.4949842070226,85.9921593114998,
86.4893344159771,86.9865095204543,87.4836846249315,87.9808597294087,88.4780348338859,
88.9752099383631,89.4723850428403,89.9695601473175,90.4667352517948,90.963910356272,
91.4610854607492,91.9582605652264,92.4554356697036,92.9526107741808,93.449785878658,
93.9469609831353,94.4441360876125,94.9413111920897,95.4384862965669,95.9356614010441,
96.4328365055213,96.9300116099986,97.4271867144758,97.924361818953,98.4215369234302,
98.9187120279074,99.4158871323846,99.9130622368618,100.410237341339,100.907412445816,
101.404587550293,101.901762654771,102.398937759248,102.896112863725,103.393287968202,
103.89046307268,104.387638177157,104.884813281634,105.381988386111,105.879163490588,
106.376338595066,106.873513699543,107.37068880402,107.867863908497,108.365039012974,
108.862214117452,109.359389221929,109.856564326406,110.353739430883,110.850914535361,
111.348089639838,111.845264744315,112.342439848792,112.839614953269,113.336790057747,
113.833965162224,114.331140266701,114.828315371178,115.325490475655,115.822665580133,
116.31984068461,116.817015789087,117.314190893564,117.811365998042,118.308541102519,
118.805716206996,119.302891311473,119.80006641595,120.297241520428,120.794416624905,
121.291591729382,121.788766833859,122.285941938336,122.783117042814,123.280292147291,
123.777467251768,124.274642356245,124.771817460723,125.2689925652,125.766167669677,
126.263342774154,126.760517878631,127.257692983109,127.754868087586,128.252043192063,
128.74921829654,129.246393401017,129.743568505495,130.240743609972,130.737918714449,
131.235093818926,131.732268923404,132.229444027881,132.726619132358,133.223794236835,
133.720969341312,134.21814444579,134.715319550267,135.212494654744,135.709669759221,
136.206844863698,136.704019968176,137.201195072653,137.69837017713,138.195545281607,
138.692720386085,139.189895490562,139.687070595039,140.184245699516,140.681420803993,
141.178595908471,141.675771012948,142.172946117425,142.670121221902,143.167296326379,
143.664471430857,144.161646535334,144.658821639811,145.155996744288,145.653171848766,
146.150346953243,146.64752205772,147.144697162197,147.641872266674,148.139047371152,
148.636222475629,149.133397580106,149.630572684583,150.12774778906,150.624922893538,
151.122097998015,151.619273102492,152.116448206969,152.613623311447,153.110798415924,
153.607973520401,154.105148624878,154.602323729355,155.099498833833,155.59667393831,
156.093849042787,156.591024147264,157.088199251742,157.585374356219,158.082549460696,
158.579724565173,159.07689966965,159.574074774128,160.071249878605,160.568424983082,
161.065600087559,161.562775192036,162.059950296514,162.557125400991,163.054300505468,
163.551475609945,164.048650714422,164.5458258189,165.043000923377,165.540176027854,
166.037351132331,166.534526236809,167.031701341286,167.528876445763,168.02605155024,
168.523226654717,169.020401759195,169.517576863672,170.014751968149,170.511927072626,
171.009102177104,171.506277281581,172.003452386058,172.500627490535,172.997802595012,
173.49497769949),.UNSPECIFIED.);
#312=CIRCLE('',#14743,4.51775);
#313=CIRCLE('',#14744,4.51775);
#314=CIRCLE('',#14745,4.51775);
#315=CIRCLE('',#14770,4.51775);
#316=CIRCLE('',#14772,5.0736);
#317=CIRCLE('',#14797,5.0736);
#318=CIRCLE('',#14799,4.51775);
#319=CIRCLE('',#14800,4.51775);
#320=CIRCLE('',#14801,4.51775);
#321=CIRCLE('',#14841,4.51775);
#322=CIRCLE('',#14843,5.07359999999999);
#323=CIRCLE('',#14883,5.0736);
#324=CIRCLE('',#14888,4.);
#325=CIRCLE('',#14893,4.);
#326=CIRCLE('',#14895,1.);
#327=CIRCLE('',#14896,1.);
#328=CIRCLE('',#14899,1.);
#329=CIRCLE('',#14900,1.);
#330=CIRCLE('',#14901,1.);
#331=CIRCLE('',#14902,1.);
#332=CIRCLE('',#14903,1.);
#333=CIRCLE('',#14904,1.);
#334=CIRCLE('',#14905,1.);
#335=CIRCLE('',#14906,1.);
#336=CIRCLE('',#14907,1.);
#337=CIRCLE('',#14908,1.);
#338=CIRCLE('',#14909,1.);
#339=CIRCLE('',#14910,1.);
#340=CIRCLE('',#14911,1.);
#341=CIRCLE('',#14912,1.);
#342=CIRCLE('',#14913,1.);
#343=CIRCLE('',#14914,1.);
#344=CIRCLE('',#14915,1.);
#345=CIRCLE('',#14916,1.);
#346=CIRCLE('',#14917,1.);
#347=CIRCLE('',#14918,1.);
#348=CIRCLE('',#14919,1.);
#349=CIRCLE('',#14920,1.);
#350=CIRCLE('',#14921,1.);
#351=CIRCLE('',#14922,1.);
#352=CIRCLE('',#14923,1.);
#353=CIRCLE('',#14924,1.);
#354=CIRCLE('',#14925,1.);
#355=CIRCLE('',#14926,1.);
#356=CIRCLE('',#14927,1.);
#357=CIRCLE('',#14928,1.);
#358=CIRCLE('',#14929,1.);
#359=CIRCLE('',#14930,1.);
#360=CIRCLE('',#14931,1.);
#361=CIRCLE('',#14932,1.);
#362=CIRCLE('',#14933,1.);
#363=CIRCLE('',#14934,3.);
#364=CIRCLE('',#14935,3.);
#365=CIRCLE('',#14936,3.);
#366=CIRCLE('',#14937,3.);
#367=CIRCLE('',#14939,1.);
#368=CIRCLE('',#14942,1.);
#369=CIRCLE('',#14945,1.);
#370=CIRCLE('',#14948,1.);
#371=CIRCLE('',#14951,1.);
#372=CIRCLE('',#14953,1.);
#373=CIRCLE('',#14956,1.);
#374=CIRCLE('',#14958,1.);
#375=CIRCLE('',#14961,1.);
#376=CIRCLE('',#14963,1.);
#377=CIRCLE('',#14966,1.);
#378=CIRCLE('',#14969,1.);
#379=CIRCLE('',#14972,1.);
#380=CIRCLE('',#14975,1.);
#381=CIRCLE('',#14977,1.);
#382=CIRCLE('',#14980,1.);
#383=CIRCLE('',#14982,1.);
#384=CIRCLE('',#14985,1.);
#385=CIRCLE('',#14987,1.);
#386=CIRCLE('',#14990,1.);
#387=CIRCLE('',#14993,1.);
#388=CIRCLE('',#14996,1.);
#389=CIRCLE('',#14999,1.);
#390=CIRCLE('',#15001,1.);
#391=CIRCLE('',#15004,1.);
#392=CIRCLE('',#15006,1.);
#393=CIRCLE('',#15009,1.);
#394=CIRCLE('',#15011,1.);
#395=CIRCLE('',#15014,1.);
#396=CIRCLE('',#15017,1.);
#397=CIRCLE('',#15020,1.);
#398=CIRCLE('',#15023,1.);
#399=CIRCLE('',#15025,1.);
#400=CIRCLE('',#15028,1.);
#401=CIRCLE('',#15030,1.);
#402=CIRCLE('',#15032,3.);
#403=CIRCLE('',#15034,3.);
#404=CIRCLE('',#15037,3.);
#405=CIRCLE('',#15039,3.);
#752=B_SPLINE_CURVE_WITH_KNOTS('',3,(#28046,#28047,#28048,#28049,#28050,
#28051,#28052),.UNSPECIFIED.,.F.,.F.,(4,3,4),(158.388651680658,158.598858328231,
159.096033432709),.UNSPECIFIED.);
#753=B_SPLINE_CURVE_WITH_KNOTS('',3,(#28060,#28061,#28062,#28063,#28064,
#28065,#28066,#28067,#28068,#28069,#28070,#28071,#28072,#28073,#28074,#28075),
 .UNSPECIFIED.,.F.,.F.,(4,3,3,3,3,4),(-157.079632679489,-156.610157910323,
-156.112982805845,-155.615807701368,-155.118632596891,-154.645421777951),
 .UNSPECIFIED.);
#754=B_SPLINE_CURVE_WITH_KNOTS('',3,(#28080,#28081,#28082,#28083,#28084,
#28085,#28086,#28087,#28088,#28089,#28090,#28091,#28092,#28093,#28094,#28095,
#28096,#28097,#28098,#28099,#28100,#28101,#28102,#28103,#28104,#28105,#28106,
#28107,#28108,#28109,#28110,#28111,#28112,#28113,#28114,#28115,#28116,#28117,
#28118,#28119,#28120,#28121,#28122),.UNSPECIFIED.,.F.,.F.,(4,3,3,3,3,3,
3,3,3,3,3,3,3,3,4),(152.105466373478,152.135581970028,152.632757074505,
153.129932178982,153.627107283459,154.124282387936,154.621457492414,155.118632596891,
155.615807701368,156.112982805845,156.610157910323,157.1073330148,157.604508119277,
158.101683223754,158.388651680658),.UNSPECIFIED.);
#755=B_SPLINE_CURVE_WITH_KNOTS('',3,(#28123,#28124,#28125,#28126,#28127,
#28128,#28129,#28130,#28131,#28132,#28133,#28134,#28135,#28136,#28137,#28138,
#28139,#28140,#28141,#28142,#28143,#28144,#28145,#28146,#28147,#28148,#28149,
#28150,#28151,#28152,#28153,#28154,#28155,#28156,#28157,#28158,#28159,#28160,
#28161,#28162,#28163,#28164,#28165),.UNSPECIFIED.,.F.,.F.,(4,3,3,3,3,3,
3,3,3,3,3,3,3,3,4),(-154.645421777951,-154.621457492414,-154.124282387936,
-153.627107283459,-153.129932178982,-152.632757074505,-152.135581970028,
-151.63840686555,-151.141231761073,-150.644056656596,-150.146881552119,
-149.649706447642,-149.152531343164,-148.655356238687,-148.362236470772),
 .UNSPECIFIED.);
#756=B_SPLINE_CURVE_WITH_KNOTS('',3,(#28170,#28171,#28172,#28173,#28174,
#28175,#28176,#28177,#28178,#28179,#28180,#28181,#28182,#28183,#28184,#28185,
#28186,#28187,#28188,#28189,#28190,#28191,#28192,#28193,#28194,#28195,#28196,
#28197,#28198,#28199,#28200,#28201,#28202,#28203,#28204,#28205,#28206,#28207,
#28208,#28209),.UNSPECIFIED.,.F.,.F.,(4,3,3,3,3,3,3,3,3,3,3,3,3,4),(145.822281066299,
146.169480716301,146.666655820778,147.163830925255,147.661006029733,148.15818113421,
148.655356238687,149.152531343164,149.649706447642,150.146881552119,150.644056656596,
151.141231761073,151.63840686555,152.105466373478),.UNSPECIFIED.);
#757=B_SPLINE_CURVE_WITH_KNOTS('',3,(#28210,#28211,#28212,#28213,#28214,
#28215,#28216,#28217,#28218,#28219,#28220,#28221,#28222,#28223,#28224,#28225,
#28226,#28227,#28228,#28229,#28230,#28231,#28232,#28233,#28234,#28235,#28236,
#28237,#28238,#28239,#28240,#28241,#28242,#28243,#28244,#28245,#28246,#28247,
#28248,#28249,#28250,#28251,#28252),.UNSPECIFIED.,.F.,.F.,(4,3,3,3,3,3,
3,3,3,3,3,3,3,3,4),(-148.362236470772,-148.15818113421,-147.661006029733,
-147.163830925255,-146.666655820778,-146.169480716301,-145.672305611824,
-145.175130507347,-144.677955402869,-144.180780298392,-143.683605193915,
-143.186430089438,-142.689254984961,-142.192079880483,-142.079051163592),
 .UNSPECIFIED.);
#758=B_SPLINE_CURVE_WITH_KNOTS('',3,(#28257,#28258,#28259,#28260,#28261,
#28262,#28263,#28264,#28265,#28266,#28267,#28268,#28269,#28270,#28271,#28272,
#28273,#28274,#28275,#28276,#28277,#28278,#28279,#28280,#28281,#28282,#28283,
#28284,#28285,#28286,#28287,#28288,#28289,#28290,#28291,#28292,#28293,#28294,
#28295,#28296,#28297,#28298,#28299),.UNSPECIFIED.,.F.,.F.,(4,3,3,3,3,3,
3,3,3,3,3,3,3,3,4),(139.539095759119,139.706204358097,140.203379462574,
140.700554567052,141.197729671529,141.694904776006,142.192079880483,142.689254984961,
143.186430089438,143.683605193915,144.180780298392,144.677955402869,145.175130507347,
145.672305611824,145.822281066299),.UNSPECIFIED.);
#759=B_SPLINE_CURVE_WITH_KNOTS('',3,(#28300,#28301,#28302,#28303,#28304,
#28305,#28306,#28307,#28308,#28309,#28310,#28311,#28312,#28313,#28314,#28315,
#28316,#28317,#28318,#28319,#28320,#28321,#28322,#28323,#28324,#28325,#28326,
#28327,#28328,#28329,#28330,#28331,#28332,#28333,#28334,#28335,#28336,#28337,
#28338,#28339),.UNSPECIFIED.,.F.,.F.,(4,3,3,3,3,3,3,3,3,3,3,3,3,4),(-142.079051163592,
-141.694904776006,-141.197729671529,-140.700554567052,-140.203379462574,
-139.706204358097,-139.20902925362,-138.711854149143,-138.214679044666,
-137.717503940188,-137.220328835711,-136.723153731234,-136.225978626757,
-135.795865856412),.UNSPECIFIED.);
#760=B_SPLINE_CURVE_WITH_KNOTS('',3,(#28344,#28345,#28346,#28347,#28348,
#28349,#28350,#28351,#28352,#28353,#28354,#28355,#28356,#28357,#28358,#28359,
#28360,#28361,#28362,#28363,#28364,#28365,#28366,#28367,#28368,#28369,#28370,
#28371,#28372,#28373,#28374,#28375,#28376,#28377,#28378,#28379,#28380,#28381,
#28382,#28383),.UNSPECIFIED.,.F.,.F.,(4,3,3,3,3,3,3,3,3,3,3,3,3,4),(133.255910451939,
133.740103104371,134.237278208848,134.734453313325,135.231628417802,135.72880352228,
136.225978626757,136.723153731234,137.220328835711,137.717503940188,138.214679044666,
138.711854149143,139.20902925362,139.539095759119),.UNSPECIFIED.);
#761=B_SPLINE_CURVE_WITH_KNOTS('',3,(#28384,#28385,#28386,#28387,#28388,
#28389,#28390,#28391,#28392,#28393,#28394,#28395,#28396,#28397,#28398,#28399,
#28400,#28401,#28402,#28403,#28404,#28405,#28406,#28407,#28408,#28409,#28410,
#28411,#28412,#28413,#28414,#28415,#28416,#28417,#28418,#28419,#28420,#28421,
#28422,#28423,#28424,#28425,#28426),.UNSPECIFIED.,.F.,.F.,(4,3,3,3,3,3,
3,3,3,3,3,3,3,3,4),(-135.795865856412,-135.72880352228,-135.231628417802,
-134.734453313325,-134.237278208848,-133.740103104371,-133.242927999893,
-132.745752895416,-132.248577790939,-131.751402686462,-131.254227581985,
-130.757052477507,-130.25987737303,-129.762702268553,-129.512680549233),
 .UNSPECIFIED.);
#762=B_SPLINE_CURVE_WITH_KNOTS('',3,(#28431,#28432,#28433,#28434,#28435,
#28436,#28437,#28438,#28439,#28440,#28441,#28442,#28443,#28444,#28445,#28446,
#28447,#28448,#28449,#28450,#28451,#28452,#28453,#28454,#28455,#28456,#28457,
#28458,#28459,#28460,#28461,#28462,#28463,#28464,#28465,#28466,#28467,#28468,
#28469,#28470,#28471,#28472,#28473),.UNSPECIFIED.,.F.,.F.,(4,3,3,3,3,3,
3,3,3,3,3,3,3,3,4),(126.97272514476,127.276826746167,127.774001850644,128.271176955121,
128.768352059598,129.265527164076,129.762702268553,130.25987737303,130.757052477507,
131.254227581985,131.751402686462,132.248577790939,132.745752895416,133.242927999893,
133.255910451939),.UNSPECIFIED.);
#763=B_SPLINE_CURVE_WITH_KNOTS('',3,(#28474,#28475,#28476,#28477,#28478,
#28479,#28480,#28481,#28482,#28483,#28484,#28485,#28486,#28487,#28488,#28489,
#28490,#28491,#28492,#28493,#28494,#28495,#28496,#28497,#28498,#28499,#28500,
#28501,#28502,#28503,#28504,#28505,#28506,#28507,#28508,#28509,#28510,#28511,
#28512,#28513,#28514,#28515,#28516),.UNSPECIFIED.,.F.,.F.,(4,3,3,3,3,3,
3,3,3,3,3,3,3,3,4),(-129.512680549233,-129.265527164076,-128.768352059599,
-128.271176955121,-127.774001850644,-127.276826746167,-126.77965164169,
-126.282476537213,-125.785301432735,-125.288126328258,-124.790951223781,
-124.293776119304,-123.796601014826,-123.299425910349,-123.229495242054),
 .UNSPECIFIED.);
#764=B_SPLINE_CURVE_WITH_KNOTS('',3,(#28521,#28522,#28523,#28524,#28525,
#28526,#28527,#28528,#28529,#28530,#28531,#28532,#28533,#28534,#28535,#28536,
#28537,#28538,#28539,#28540,#28541,#28542,#28543,#28544,#28545,#28546,#28547,
#28548,#28549,#28550,#28551,#28552,#28553,#28554,#28555,#28556,#28557,#28558,
#28559,#28560,#28561,#28562,#28563),.UNSPECIFIED.,.F.,.F.,(4,3,3,3,3,3,
3,3,3,3,3,3,3,3,4),(120.68953983758,120.813550387963,121.31072549244,121.807900596918,
122.305075701395,122.802250805872,123.299425910349,123.796601014826,124.293776119304,
124.790951223781,125.288126328258,125.785301432735,126.282476537212,126.77965164169,
126.97272514476),.UNSPECIFIED.);
#765=B_SPLINE_CURVE_WITH_KNOTS('',3,(#28564,#28565,#28566,#28567,#28568,
#28569,#28570,#28571,#28572,#28573,#28574,#28575,#28576,#28577,#28578,#28579,
#28580,#28581,#28582,#28583,#28584,#28585,#28586,#28587,#28588,#28589,#28590,
#28591,#28592,#28593,#28594,#28595,#28596,#28597,#28598,#28599,#28600,#28601,
#28602,#28603),.UNSPECIFIED.,.F.,.F.,(4,3,3,3,3,3,3,3,3,3,3,3,3,4),(-123.229495242054,
-122.802250805872,-122.305075701395,-121.807900596918,-121.31072549244,
-120.813550387963,-120.316375283486,-119.819200179009,-119.322025074531,
-118.824849970054,-118.327674865577,-117.8304997611,-117.333324656623,-116.946309934874),
 .UNSPECIFIED.);
#766=B_SPLINE_CURVE_WITH_KNOTS('',3,(#28608,#28609,#28610,#28611,#28612,
#28613,#28614,#28615,#28616,#28617,#28618,#28619,#28620,#28621,#28622,#28623,
#28624,#28625,#28626,#28627,#28628,#28629,#28630,#28631,#28632,#28633,#28634,
#28635,#28636,#28637,#28638,#28639,#28640,#28641,#28642,#28643,#28644,#28645,
#28646,#28647),.UNSPECIFIED.,.F.,.F.,(4,3,3,3,3,3,3,3,3,3,3,3,3,4),(114.406354530401,
114.847449134237,115.344624238714,115.841799343191,116.338974447668,116.836149552145,
117.333324656623,117.8304997611,118.327674865577,118.824849970054,119.322025074531,
119.819200179009,120.316375283486,120.68953983758),.UNSPECIFIED.);
#767=B_SPLINE_CURVE_WITH_KNOTS('',3,(#28648,#28649,#28650,#28651,#28652,
#28653,#28654,#28655,#28656,#28657,#28658,#28659,#28660,#28661,#28662,#28663,
#28664,#28665,#28666,#28667,#28668,#28669,#28670,#28671,#28672,#28673,#28674,
#28675,#28676,#28677,#28678,#28679,#28680,#28681,#28682,#28683,#28684,#28685,
#28686,#28687,#28688,#28689,#28690),.UNSPECIFIED.,.F.,.F.,(4,3,3,3,3,3,
3,3,3,3,3,3,3,3,4),(-116.946309934874,-116.836149552145,-116.338974447668,
-115.841799343191,-115.344624238714,-114.847449134237,-114.350274029759,
-113.853098925282,-113.355923820805,-112.858748716328,-112.36157361185,
-111.864398507373,-111.367223402896,-110.870048298419,-110.663124627694),
 .UNSPECIFIED.);
#768=B_SPLINE_CURVE_WITH_KNOTS('',3,(#28695,#28696,#28697,#28698,#28699,
#28700,#28701,#28702,#28703,#28704,#28705,#28706,#28707,#28708,#28709,#28710,
#28711,#28712,#28713,#28714,#28715,#28716,#28717,#28718,#28719,#28720,#28721,
#28722,#28723,#28724,#28725,#28726,#28727,#28728,#28729,#28730,#28731,#28732,
#28733,#28734,#28735,#28736,#28737),.UNSPECIFIED.,.F.,.F.,(4,3,3,3,3,3,
3,3,3,3,3,3,3,3,4),(108.123169223221,108.384172776033,108.88134788051,109.378522984987,
109.875698089464,110.372873193942,110.870048298419,111.367223402896,111.864398507373,
112.36157361185,112.858748716328,113.355923820805,113.853098925282,114.350274029759,
114.406354530401),.UNSPECIFIED.);
#769=B_SPLINE_CURVE_WITH_KNOTS('',3,(#28738,#28739,#28740,#28741,#28742,
#28743,#28744,#28745,#28746,#28747,#28748,#28749,#28750,#28751,#28752,#28753,
#28754,#28755,#28756,#28757,#28758,#28759,#28760,#28761,#28762,#28763,#28764,
#28765,#28766,#28767,#28768,#28769,#28770,#28771,#28772,#28773,#28774,#28775,
#28776,#28777,#28778,#28779,#28780),.UNSPECIFIED.,.F.,.F.,(4,3,3,3,3,3,
3,3,3,3,3,3,3,3,4),(-110.663124627694,-110.372873193942,-109.875698089464,
-109.378522984987,-108.88134788051,-108.384172776033,-107.886997671556,
-107.389822567078,-106.892647462601,-106.395472358124,-105.898297253647,
-105.401122149169,-104.903947044692,-104.406771940215,-104.379939320514),
 .UNSPECIFIED.);
#770=B_SPLINE_CURVE_WITH_KNOTS('',3,(#28785,#28786,#28787,#28788,#28789,
#28790,#28791,#28792,#28793,#28794,#28795,#28796,#28797,#28798,#28799,#28800,
#28801,#28802,#28803,#28804,#28805,#28806,#28807,#28808,#28809,#28810,#28811,
#28812,#28813,#28814,#28815,#28816,#28817,#28818,#28819,#28820,#28821,#28822,
#28823,#28824,#28825,#28826,#28827),.UNSPECIFIED.,.F.,.F.,(4,3,3,3,3,3,
3,3,3,3,3,3,3,3,4),(101.839983916041,101.920896417829,102.418071522306,
102.915246626783,103.412421731261,103.909596835738,104.406771940215,104.903947044692,
105.401122149169,105.898297253647,106.395472358124,106.892647462601,107.389822567078,
107.886997671556,108.123169223221),.UNSPECIFIED.);
#771=B_SPLINE_CURVE_WITH_KNOTS('',3,(#28828,#28829,#28830,#28831,#28832,
#28833,#28834,#28835,#28836,#28837,#28838,#28839,#28840,#28841,#28842,#28843,
#28844,#28845,#28846,#28847,#28848,#28849,#28850,#28851,#28852,#28853,#28854,
#28855,#28856,#28857,#28858,#28859,#28860,#28861,#28862,#28863,#28864,#28865,
#28866,#28867),.UNSPECIFIED.,.F.,.F.,(4,3,3,3,3,3,3,3,3,3,3,3,3,4),(-104.379939320514,
-103.909596835738,-103.412421731261,-102.915246626783,-102.418071522306,
-101.920896417829,-101.423721313352,-100.926546208875,-100.429371104397,
-99.9321959999201,-99.4350208954429,-98.9378457909657,-98.4406706864885,
-98.0967540133348),.UNSPECIFIED.);
#772=B_SPLINE_CURVE_WITH_KNOTS('',3,(#28872,#28873,#28874,#28875,#28876,
#28877,#28878,#28879,#28880,#28881,#28882,#28883,#28884,#28885,#28886,#28887,
#28888,#28889,#28890,#28891,#28892,#28893,#28894,#28895,#28896,#28897,#28898,
#28899,#28900,#28901,#28902,#28903,#28904,#28905,#28906,#28907,#28908,#28909,
#28910,#28911),.UNSPECIFIED.,.F.,.F.,(4,3,3,3,3,3,3,3,3,3,3,3,3,4),(95.5567986088618,
95.9547951641024,96.4519702685796,96.9491453730568,97.446320477534,97.9434955820112,
98.4406706864884,98.9378457909657,99.4350208954429,99.9321959999201,100.429371104397,
100.926546208875,101.423721313352,101.839983916041),.UNSPECIFIED.);
#773=B_SPLINE_CURVE_WITH_KNOTS('',3,(#28912,#28913,#28914,#28915,#28916,
#28917,#28918,#28919,#28920,#28921,#28922,#28923,#28924,#28925,#28926,#28927,
#28928,#28929,#28930,#28931,#28932,#28933,#28934,#28935,#28936,#28937,#28938,
#28939,#28940,#28941,#28942,#28943,#28944,#28945,#28946,#28947,#28948,#28949,
#28950,#28951,#28952,#28953,#28954),.UNSPECIFIED.,.F.,.F.,(4,3,3,3,3,3,
3,3,3,3,3,3,3,3,4),(-98.0967540133348,-97.9434955820113,-97.446320477534,
-96.9491453730568,-96.4519702685796,-95.9547951641024,-95.4576200596252,
-94.960444955148,-94.4632698506707,-93.9660947461935,-93.4689196417163,
-92.9717445372391,-92.4745694327619,-91.9773943282847,-91.8135687061551),
 .UNSPECIFIED.);
#774=B_SPLINE_CURVE_WITH_KNOTS('',3,(#28959,#28960,#28961,#28962,#28963,
#28964,#28965,#28966,#28967,#28968,#28969,#28970,#28971,#28972,#28973,#28974,
#28975,#28976,#28977,#28978,#28979,#28980,#28981,#28982,#28983,#28984,#28985,
#28986,#28987,#28988,#28989,#28990,#28991,#28992,#28993,#28994,#28995,#28996,
#28997,#28998,#28999,#29000,#29001),.UNSPECIFIED.,.F.,.F.,(4,3,3,3,3,3,
3,3,3,3,3,3,3,3,4),(89.2736133016821,89.4915188058986,89.9886939103758,
90.485869014853,90.9830441193302,91.4802192238075,91.9773943282847,92.4745694327619,
92.9717445372391,93.4689196417163,93.9660947461935,94.4632698506707,94.9604449551479,
95.4576200596252,95.5567986088618),.UNSPECIFIED.);
#775=B_SPLINE_CURVE_WITH_KNOTS('',3,(#29002,#29003,#29004,#29005,#29006,
#29007,#29008,#29009,#29010,#29011,#29012,#29013,#29014,#29015,#29016,#29017,
#29018,#29019,#29020,#29021,#29022,#29023,#29024,#29025,#29026,#29027,#29028,
#29029,#29030,#29031,#29032,#29033,#29034,#29035,#29036,#29037,#29038,#29039,
#29040,#29041),.UNSPECIFIED.,.F.,.F.,(4,3,3,3,3,3,3,3,3,3,3,3,3,4),(-91.8135687061551,
-91.4802192238075,-90.9830441193302,-90.485869014853,-89.9886939103758,
-89.4915188058986,-88.9943437014214,-88.4971685969442,-87.9999934924669,
-87.5028183879897,-87.0056432835125,-86.5084681790353,-86.0112930745581,
-85.5303833989759),.UNSPECIFIED.);
#776=B_SPLINE_CURVE_WITH_KNOTS('',3,(#29046,#29047,#29048,#29049,#29050,
#29051,#29052,#29053,#29054,#29055,#29056,#29057,#29058,#29059,#29060,#29061,
#29062,#29063,#29064,#29065,#29066,#29067,#29068,#29069,#29070,#29071,#29072,
#29073,#29074,#29075,#29076,#29077,#29078,#29079,#29080,#29081,#29082,#29083,
#29084,#29085,#29086,#29087,#29088),.UNSPECIFIED.,.F.,.F.,(4,3,3,3,3,3,
3,3,3,3,3,3,3,3,4),(82.9904279945029,83.0282424476948,83.525417552172,84.0225926566493,
84.5197677611265,85.0169428656037,85.5141179700809,86.0112930745581,86.5084681790353,
87.0056432835125,87.5028183879897,87.9999934924669,88.4971685969441,88.9943437014214,
89.2736133016821),.UNSPECIFIED.);
#777=B_SPLINE_CURVE_WITH_KNOTS('',3,(#29089,#29090,#29091,#29092,#29093,
#29094,#29095,#29096,#29097,#29098,#29099,#29100,#29101,#29102,#29103,#29104,
#29105,#29106,#29107,#29108,#29109,#29110,#29111,#29112,#29113,#29114,#29115,
#29116,#29117,#29118,#29119,#29120,#29121,#29122,#29123,#29124,#29125,#29126,
#29127,#29128,#29129,#29130,#29131),.UNSPECIFIED.,.F.,.F.,(4,3,3,3,3,3,
3,3,3,3,3,3,3,3,4),(-85.5303833989759,-85.5141179700809,-85.0169428656037,
-84.5197677611264,-84.0225926566492,-83.525417552172,-83.0282424476948,
-82.5310673432176,-82.0338922387404,-81.5367171342632,-81.039542029786,
-80.5423669253087,-80.0451918208315,-79.5480167163543,-79.2471980917962),
 .UNSPECIFIED.);
#778=B_SPLINE_CURVE_WITH_KNOTS('',3,(#29136,#29137,#29138,#29139,#29140,
#29141,#29142,#29143,#29144,#29145,#29146,#29147,#29148,#29149,#29150,#29151,
#29152,#29153,#29154,#29155,#29156,#29157,#29158,#29159,#29160,#29161,#29162,
#29163,#29164,#29165,#29166,#29167,#29168,#29169,#29170,#29171,#29172,#29173,
#29174,#29175),.UNSPECIFIED.,.F.,.F.,(4,3,3,3,3,3,3,3,3,3,3,3,3,4),(76.7072426873232,
77.0621411939682,77.5593162984454,78.0564914029227,78.5536665073999,79.0508416118771,
79.5480167163543,80.0451918208315,80.5423669253087,81.0395420297859,81.5367171342632,
82.0338922387404,82.5310673432176,82.9904279945029),.UNSPECIFIED.);
#779=B_SPLINE_CURVE_WITH_KNOTS('',3,(#29176,#29177,#29178,#29179,#29180,
#29181,#29182,#29183,#29184,#29185,#29186,#29187,#29188,#29189,#29190,#29191,
#29192,#29193,#29194,#29195,#29196,#29197,#29198,#29199,#29200,#29201,#29202,
#29203,#29204,#29205,#29206,#29207,#29208,#29209,#29210,#29211,#29212,#29213,
#29214,#29215,#29216,#29217,#29218),.UNSPECIFIED.,.F.,.F.,(4,3,3,3,3,3,
3,3,3,3,3,3,3,3,4),(-79.2471980917962,-79.0508416118771,-78.5536665073999,
-78.0564914029227,-77.5593162984455,-77.0621411939683,-76.564966089491,
-76.0677909850138,-75.5706158805366,-75.0734407760594,-74.5762656715822,
-74.079090567105,-73.5819154626277,-73.0847403581505,-72.9640127846165),
 .UNSPECIFIED.);
#780=B_SPLINE_CURVE_WITH_KNOTS('',3,(#29223,#29224,#29225,#29226,#29227,
#29228,#29229,#29230,#29231,#29232,#29233,#29234,#29235,#29236,#29237,#29238,
#29239,#29240,#29241,#29242,#29243,#29244,#29245,#29246,#29247,#29248,#29249,
#29250,#29251,#29252,#29253,#29254,#29255,#29256,#29257,#29258,#29259,#29260,
#29261,#29262,#29263,#29264,#29265),.UNSPECIFIED.,.F.,.F.,(4,3,3,3,3,3,
3,3,3,3,3,3,3,3,4),(70.4240573801435,70.5988648357644,71.0960399402417,
71.5932150447189,72.0903901491961,72.5875652536733,73.0847403581505,73.5819154626277,
74.0790905671049,74.5762656715822,75.0734407760594,75.5706158805366,76.0677909850138,
76.564966089491,76.7072426873232),.UNSPECIFIED.);
#781=B_SPLINE_CURVE_WITH_KNOTS('',3,(#29266,#29267,#29268,#29269,#29270,
#29271,#29272,#29273,#29274,#29275,#29276,#29277,#29278,#29279,#29280,#29281,
#29282,#29283,#29284,#29285,#29286,#29287,#29288,#29289,#29290,#29291,#29292,
#29293,#29294,#29295,#29296,#29297,#29298,#29299,#29300,#29301,#29302,#29303,
#29304,#29305),.UNSPECIFIED.,.F.,.F.,(4,3,3,3,3,3,3,3,3,3,3,3,3,4),(-72.9640127846165,
-72.5875652536733,-72.0903901491961,-71.5932150447189,-71.0960399402417,
-70.5988648357645,-70.1016897312873,-69.60451462681,-69.1073395223328,-68.6101644178556,
-68.1129893133784,-67.6158142089012,-67.1186391044239,-66.6808274774369),
 .UNSPECIFIED.);
#782=B_SPLINE_CURVE_WITH_KNOTS('',3,(#29310,#29311,#29312,#29313,#29314,
#29315,#29316,#29317,#29318,#29319,#29320,#29321,#29322,#29323,#29324,#29325,
#29326,#29327,#29328,#29329,#29330,#29331,#29332,#29333,#29334,#29335,#29336,
#29337,#29338,#29339,#29340,#29341,#29342,#29343,#29344,#29345,#29346,#29347,
#29348,#29349),.UNSPECIFIED.,.F.,.F.,(4,3,3,3,3,3,3,3,3,3,3,3,3,4),(64.1408720729639,
64.6327635820379,65.1299386865151,65.6271137909923,66.1242888954695,66.6214639999467,
67.1186391044239,67.6158142089012,68.1129893133784,68.6101644178556,69.1073395223328,
69.60451462681,70.1016897312872,70.4240573801435),.UNSPECIFIED.);
#783=B_SPLINE_CURVE_WITH_KNOTS('',3,(#29350,#29351,#29352,#29353,#29354,
#29355,#29356,#29357,#29358,#29359,#29360,#29361,#29362,#29363,#29364,#29365,
#29366,#29367,#29368,#29369,#29370,#29371,#29372,#29373,#29374,#29375,#29376,
#29377,#29378,#29379,#29380,#29381,#29382,#29383,#29384,#29385,#29386,#29387,
#29388,#29389,#29390,#29391,#29392),.UNSPECIFIED.,.F.,.F.,(4,3,3,3,3,3,
3,3,3,3,3,3,3,3,4),(-66.6808274774369,-66.6214639999467,-66.1242888954695,
-65.6271137909923,-65.1299386865151,-64.6327635820379,-64.1355884775607,
-63.6384133730835,-63.1412382686062,-62.644063164129,-62.1468880596518,
-61.6497129551746,-61.1525378506974,-60.6553627462202,-60.3976421702572),
 .UNSPECIFIED.);
#784=B_SPLINE_CURVE_WITH_KNOTS('',3,(#29397,#29398,#29399,#29400,#29401,
#29402,#29403,#29404,#29405,#29406,#29407,#29408,#29409,#29410,#29411,#29412,
#29413,#29414,#29415,#29416,#29417,#29418,#29419,#29420,#29421,#29422,#29423,
#29424,#29425,#29426,#29427,#29428,#29429,#29430,#29431,#29432,#29433,#29434,
#29435,#29436,#29437,#29438,#29439),.UNSPECIFIED.,.F.,.F.,(4,3,3,3,3,3,
3,3,3,3,3,3,3,3,4),(57.8576867657842,58.1694872238341,58.6666623283113,
59.1638374327885,59.6610125372657,60.1581876417429,60.6553627462201,61.1525378506974,
61.6497129551746,62.1468880596518,62.644063164129,63.1412382686062,63.6384133730835,
64.1355884775607,64.1408720729639),.UNSPECIFIED.);
#785=B_SPLINE_CURVE_WITH_KNOTS('',3,(#29440,#29441,#29442,#29443,#29444,
#29445,#29446,#29447,#29448,#29449,#29450,#29451,#29452,#29453,#29454,#29455,
#29456,#29457,#29458,#29459,#29460,#29461,#29462,#29463,#29464,#29465,#29466,
#29467,#29468,#29469,#29470,#29471,#29472,#29473,#29474,#29475,#29476,#29477,
#29478,#29479,#29480,#29481,#29482),.UNSPECIFIED.,.F.,.F.,(4,3,3,3,3,3,
3,3,3,3,3,3,3,3,4),(-60.3976421702572,-60.158187641743,-59.6610125372657,
-59.1638374327885,-58.6666623283113,-58.1694872238341,-57.6723121193569,
-57.1751370148797,-56.6779619104025,-56.1807868059252,-55.683611701448,
-55.1864365969708,-54.6892614924936,-54.1920863880164,-54.114456863078),
 .UNSPECIFIED.);
#786=B_SPLINE_CURVE_WITH_KNOTS('',3,(#29487,#29488,#29489,#29490,#29491,
#29492,#29493,#29494,#29495,#29496,#29497,#29498,#29499,#29500,#29501,#29502,
#29503,#29504,#29505,#29506,#29507,#29508,#29509,#29510,#29511,#29512,#29513,
#29514,#29515,#29516,#29517,#29518,#29519,#29520,#29521,#29522,#29523,#29524,
#29525,#29526,#29527,#29528,#29529),.UNSPECIFIED.,.F.,.F.,(4,3,3,3,3,3,
3,3,3,3,3,3,3,3,4),(51.5745014586045,51.7062108656303,52.2033859701075,
52.7005610745847,53.1977361790619,53.6949112835391,54.1920863880164,54.6892614924936,
55.1864365969708,55.683611701448,56.1807868059252,56.6779619104024,57.1751370148797,
57.6723121193569,57.8576867657842),.UNSPECIFIED.);
#787=B_SPLINE_CURVE_WITH_KNOTS('',3,(#29530,#29531,#29532,#29533,#29534,
#29535,#29536,#29537,#29538,#29539,#29540,#29541,#29542,#29543,#29544,#29545,
#29546,#29547,#29548,#29549,#29550,#29551,#29552,#29553,#29554,#29555,#29556,
#29557,#29558,#29559,#29560,#29561,#29562,#29563,#29564,#29565,#29566,#29567,
#29568,#29569),.UNSPECIFIED.,.F.,.F.,(4,3,3,3,3,3,3,3,3,3,3,3,3,4),(-54.114456863078,
-53.6949112835392,-53.197736179062,-52.7005610745847,-52.2033859701075,
-51.7062108656303,-51.2090357611531,-50.7118606566759,-50.2146855521987,
-49.7175104477215,-49.2203353432442,-48.723160238767,-48.2259851342898,
-47.8312715558983),.UNSPECIFIED.);
#788=B_SPLINE_CURVE_WITH_KNOTS('',3,(#29574,#29575,#29576,#29577,#29578,
#29579,#29580,#29581,#29582,#29583,#29584,#29585,#29586,#29587,#29588,#29589,
#29590,#29591,#29592,#29593,#29594,#29595,#29596,#29597,#29598,#29599,#29600,
#29601,#29602,#29603,#29604,#29605,#29606,#29607,#29608,#29609,#29610,#29611,
#29612,#29613),.UNSPECIFIED.,.F.,.F.,(4,3,3,3,3,3,3,3,3,3,3,3,3,4),(45.2913161514253,
45.7401096119037,46.2372847163809,46.7344598208582,47.2316349253354,47.7288100298126,
48.2259851342898,48.723160238767,49.2203353432442,49.7175104477214,50.2146855521987,
50.7118606566759,51.2090357611531,51.5745014586045),.UNSPECIFIED.);
#789=B_SPLINE_CURVE_WITH_KNOTS('',3,(#29614,#29615,#29616,#29617,#29618,
#29619,#29620,#29621,#29622,#29623,#29624,#29625,#29626,#29627,#29628,#29629,
#29630,#29631,#29632,#29633,#29634,#29635,#29636,#29637,#29638,#29639,#29640,
#29641,#29642,#29643,#29644,#29645,#29646,#29647,#29648,#29649,#29650,#29651,
#29652,#29653,#29654,#29655,#29656),.UNSPECIFIED.,.F.,.F.,(4,3,3,3,3,3,
3,3,3,3,3,3,3,3,4),(-47.8312715558983,-47.7288100298126,-47.2316349253354,
-46.7344598208582,-46.2372847163809,-45.7401096119037,-45.2429345074265,
-44.7457594029493,-44.2485842984721,-43.7514091939949,-43.2542340895177,
-42.7570589850404,-42.2598838805632,-41.762708776086,-41.5480862487186),
 .UNSPECIFIED.);
#790=B_SPLINE_CURVE_WITH_KNOTS('',3,(#29661,#29662,#29663,#29664,#29665,
#29666,#29667,#29668,#29669,#29670,#29671,#29672,#29673,#29674,#29675,#29676,
#29677,#29678,#29679,#29680,#29681,#29682,#29683,#29684,#29685,#29686,#29687,
#29688,#29689,#29690,#29691,#29692,#29693,#29694,#29695,#29696,#29697,#29698,
#29699,#29700,#29701,#29702,#29703),.UNSPECIFIED.,.F.,.F.,(4,3,3,3,3,3,
3,3,3,3,3,3,3,3,4),(39.0081308442456,39.2768332536999,39.7740083581771,
40.2711834626544,40.7683585671316,41.2655336716088,41.762708776086,42.2598838805632,
42.7570589850404,43.2542340895177,43.7514091939949,44.2485842984721,44.7457594029493,
45.2429345074265,45.2913161514253),.UNSPECIFIED.);
#791=B_SPLINE_CURVE_WITH_KNOTS('',3,(#29704,#29705,#29706,#29707,#29708,
#29709,#29710,#29711,#29712,#29713,#29714,#29715,#29716,#29717,#29718,#29719,
#29720,#29721,#29722,#29723,#29724,#29725,#29726,#29727,#29728,#29729,#29730,
#29731,#29732,#29733,#29734,#29735,#29736,#29737,#29738,#29739,#29740,#29741,
#29742,#29743,#29744,#29745,#29746),.UNSPECIFIED.,.F.,.F.,(4,3,3,3,3,3,
3,3,3,3,3,3,3,3,4),(-41.5480862487186,-41.2655336716088,-40.7683585671316,
-40.2711834626544,-39.7740083581772,-39.2768332536999,-38.7796581492227,
-38.2824830447455,-37.7853079402683,-37.2881328357911,-36.7909577313139,
-36.2937826268367,-35.7966075223594,-35.2994324178822,-35.2649009415389),
 .UNSPECIFIED.);
#792=B_SPLINE_CURVE_WITH_KNOTS('',3,(#29751,#29752,#29753,#29754,#29755,
#29756,#29757,#29758,#29759,#29760,#29761,#29762,#29763,#29764,#29765,#29766,
#29767,#29768,#29769,#29770,#29771,#29772,#29773,#29774,#29775,#29776,#29777,
#29778,#29779,#29780,#29781,#29782,#29783,#29784,#29785,#29786,#29787,#29788,
#29789,#29790,#29791,#29792,#29793),.UNSPECIFIED.,.F.,.F.,(4,3,3,3,3,3,
3,3,3,3,3,3,3,3,4),(32.7249455370659,32.8135568954961,33.3107319999734,
33.8079071044506,34.3050822089278,34.802257313405,35.2994324178822,35.7966075223594,
36.2937826268367,36.7909577313139,37.2881328357911,37.7853079402683,38.2824830447455,
38.7796581492227,39.0081308442456),.UNSPECIFIED.);
#793=B_SPLINE_CURVE_WITH_KNOTS('',3,(#29794,#29795,#29796,#29797,#29798,
#29799,#29800,#29801,#29802,#29803,#29804,#29805,#29806,#29807,#29808,#29809,
#29810,#29811,#29812,#29813,#29814,#29815,#29816,#29817,#29818,#29819,#29820,
#29821,#29822,#29823,#29824,#29825,#29826,#29827,#29828,#29829,#29830,#29831,
#29832,#29833),.UNSPECIFIED.,.F.,.F.,(4,3,3,3,3,3,3,3,3,3,3,3,3,4),(-35.2649009415389,
-34.802257313405,-34.3050822089278,-33.8079071044506,-33.3107319999734,
-32.8135568954962,-32.3163817910189,-31.8192066865417,-31.3220315820645,
-30.8248564775873,-30.3276813731101,-29.8305062686329,-29.3333311641557,
-28.9817156343593),.UNSPECIFIED.);
#794=B_SPLINE_CURVE_WITH_KNOTS('',3,(#29838,#29839,#29840,#29841,#29842,
#29843,#29844,#29845,#29846,#29847,#29848,#29849,#29850,#29851,#29852,#29853,
#29854,#29855,#29856,#29857,#29858,#29859,#29860,#29861,#29862,#29863,#29864,
#29865,#29866,#29867,#29868,#29869,#29870,#29871,#29872,#29873,#29874,#29875,
#29876,#29877),.UNSPECIFIED.,.F.,.F.,(4,3,3,3,3,3,3,3,3,3,3,3,3,4),(26.4417602298863,
26.8474556417696,27.3446307462468,27.841805850724,28.3389809552012,28.8361560596784,
29.3333311641556,29.8305062686329,30.3276813731101,30.8248564775873,31.3220315820645,
31.8192066865417,32.3163817910189,32.7249455370659),.UNSPECIFIED.);
#795=B_SPLINE_CURVE_WITH_KNOTS('',3,(#29878,#29879,#29880,#29881,#29882,
#29883,#29884,#29885,#29886,#29887,#29888,#29889,#29890,#29891,#29892,#29893,
#29894,#29895,#29896,#29897,#29898,#29899,#29900,#29901,#29902,#29903,#29904,
#29905,#29906,#29907,#29908,#29909,#29910,#29911,#29912,#29913,#29914,#29915,
#29916,#29917,#29918,#29919,#29920),.UNSPECIFIED.,.F.,.F.,(4,3,3,3,3,3,
3,3,3,3,3,3,3,3,4),(-28.9817156343593,-28.8361560596784,-28.3389809552012,
-27.841805850724,-27.3446307462468,-26.8474556417696,-26.3502805372924,
-25.8531054328152,-25.3559303283379,-24.8587552238607,-24.3615801193835,
-23.8644050149063,-23.3672299104291,-22.8700548059519,-22.69853032718),
 .UNSPECIFIED.);
#796=B_SPLINE_CURVE_WITH_KNOTS('',3,(#29925,#29926,#29927,#29928,#29929,
#29930,#29931,#29932,#29933,#29934,#29935,#29936,#29937,#29938,#29939,#29940,
#29941,#29942,#29943,#29944,#29945,#29946,#29947,#29948,#29949,#29950,#29951,
#29952,#29953,#29954,#29955,#29956,#29957,#29958,#29959,#29960,#29961,#29962,
#29963,#29964,#29965,#29966,#29967),.UNSPECIFIED.,.F.,.F.,(4,3,3,3,3,3,
3,3,3,3,3,3,3,3,4),(20.1585749227066,20.3841792835658,20.881354388043,21.3785294925202,
21.8757045969974,22.3728797014746,22.8700548059519,23.3672299104291,23.8644050149063,
24.3615801193835,24.8587552238607,25.3559303283379,25.8531054328151,26.3502805372924,
26.4417602298863),.UNSPECIFIED.);
#797=B_SPLINE_CURVE_WITH_KNOTS('',3,(#29968,#29969,#29970,#29971,#29972,
#29973,#29974,#29975,#29976,#29977,#29978,#29979,#29980,#29981,#29982,#29983,
#29984,#29985,#29986,#29987,#29988,#29989,#29990,#29991,#29992,#29993,#29994,
#29995,#29996,#29997,#29998,#29999,#30000,#30001,#30002,#30003,#30004,#30005,
#30006,#30007),.UNSPECIFIED.,.F.,.F.,(4,3,3,3,3,3,3,3,3,3,3,3,3,4),(-22.69853032718,
-22.3728797014747,-21.8757045969974,-21.3785294925202,-20.881354388043,
-20.3841792835658,-19.8870041790886,-19.3898290746114,-18.8926539701342,
-18.3954788656569,-17.8983037611797,-17.4011286567025,-16.9039535522253,
-16.4153450200004),.UNSPECIFIED.);
#798=B_SPLINE_CURVE_WITH_KNOTS('',3,(#30012,#30013,#30014,#30015,#30016,
#30017,#30018,#30019,#30020,#30021,#30022,#30023,#30024,#30025,#30026,#30027,
#30028,#30029,#30030,#30031,#30032,#30033,#30034,#30035,#30036,#30037,#30038,
#30039,#30040,#30041,#30042,#30043,#30044,#30045,#30046,#30047,#30048,#30049,
#30050,#30051,#30052,#30053,#30054),.UNSPECIFIED.,.F.,.F.,(4,3,3,3,3,3,
3,3,3,3,3,3,3,3,4),(13.8753896155273,13.920902925362,14.4180780298392,14.9152531343164,
15.4124282387936,15.9096033432709,16.4067784477481,16.9039535522253,17.4011286567025,
17.8983037611797,18.3954788656569,18.8926539701341,19.3898290746114,19.8870041790886,
20.1585749227066),.UNSPECIFIED.);
#799=B_SPLINE_CURVE_WITH_KNOTS('',3,(#30055,#30056,#30057,#30058,#30059,
#30060,#30061,#30062,#30063,#30064,#30065,#30066,#30067,#30068,#30069,#30070,
#30071,#30072,#30073,#30074,#30075,#30076,#30077,#30078,#30079,#30080,#30081,
#30082,#30083,#30084,#30085,#30086,#30087,#30088,#30089,#30090,#30091,#30092,
#30093,#30094,#30095,#30096,#30097),.UNSPECIFIED.,.F.,.F.,(4,3,3,3,3,3,
3,3,3,3,3,3,3,3,4),(-16.4153450200004,-16.4067784477481,-15.9096033432709,
-15.4124282387936,-14.9152531343164,-14.4180780298392,-13.920902925362,
-13.4237278208848,-12.9265527164076,-12.4293776119304,-11.9322025074531,
-11.4350274029759,-10.9378522984987,-10.4406771940215,-10.1321597128207),
 .UNSPECIFIED.);
#800=B_SPLINE_CURVE_WITH_KNOTS('',3,(#30103,#30104,#30105,#30106,#30107,
#30108,#30109,#30110,#30111,#30112,#30113,#30114,#30115,#30116,#30117,#30118,
#30119,#30120,#30121,#30122,#30123,#30124,#30125,#30126,#30127),
 .UNSPECIFIED.,.F.,.F.,(4,3,3,3,3,3,3,3,4),(-3.848974405641,-3.4802257313405,
-2.98305062686329,-2.48587552238607,-1.98870041790886,-1.49152531343164,
-0.99435020895443,-0.497175104477215,0.),.UNSPECIFIED.);
#801=B_SPLINE_CURVE_WITH_KNOTS('',3,(#30130,#30131,#30132,#30133,#30134,
#30135,#30136,#30137,#30138,#30139,#30140,#30141,#30142,#30143,#30144,#30145,
#30146,#30147,#30148,#30149,#30150,#30151,#30152,#30153,#30154,#30155,#30156,
#30157,#30158,#30159,#30160,#30161,#30162,#30163,#30164,#30165,#30166),
 .UNSPECIFIED.,.F.,.F.,(4,3,3,3,3,3,3,3,3,3,3,3,4),(2.01640075321939,2.48587552238607,
2.98305062686328,3.4802257313405,3.97740083581771,4.47457594029493,4.97175104477214,
5.46892614924935,5.96610125372657,6.46327635820378,6.960451462681,7.45762656715821,
7.59220430834767),.UNSPECIFIED.);
#802=B_SPLINE_CURVE_WITH_KNOTS('',3,(#30172,#30173,#30174,#30175,#30176,
#30177,#30178,#30179,#30180,#30181,#30182,#30183),.UNSPECIFIED.,.F.,.F.,
(4,1,1,1,1,1,1,1,1,4),(166.504410640259,166.977621459199,167.474796563676,
167.971971668153,168.46914677263,168.966321877108,169.463496981585,169.960672086062,
170.457847190539,170.955022295017),.UNSPECIFIED.);
#803=B_SPLINE_CURVE_WITH_KNOTS('',3,(#30186,#30187,#30188,#30189,#30190,
#30191,#30192,#30193,#30194,#30195,#30196,#30197,#30198,#30199),
 .UNSPECIFIED.,.F.,.F.,(4,1,1,1,1,1,1,1,1,1,1,4),(166.504410640259,166.534526236809,
167.031701341286,167.528876445763,168.02605155024,168.523226654717,169.020401759195,
169.517576863672,170.014751968149,170.511927072626,171.009102177104,171.47857694627),
 .UNSPECIFIED.);
#804=B_SPLINE_CURVE_WITH_KNOTS('',3,(#30204,#30205,#30206,#30207,#30208,
#30209,#30210,#30211,#30212,#30213,#30214,#30215,#30216,#30217,#30218,#30219,
#30220),.UNSPECIFIED.,.F.,.F.,(4,1,1,1,1,1,1,1,1,1,1,1,1,1,4),(160.22122533308,
160.514345100995,161.011520205472,161.508695309949,162.005870414427,162.503045518904,
163.000220623381,163.497395727858,163.994570832336,164.491745936813,164.98892104129,
165.486096145767,165.983271250244,166.480446354722,166.504410640259),
 .UNSPECIFIED.);
#805=B_SPLINE_CURVE_WITH_KNOTS('',3,(#30221,#30222,#30223,#30224,#30225,
#30226,#30227,#30228,#30229,#30230,#30231,#30232,#30233,#30234,#30235,#30236),
 .UNSPECIFIED.,.F.,.F.,(4,1,1,1,1,1,1,1,1,1,1,1,1,4),(160.22122533308,160.568424983082,
161.065600087559,161.562775192036,162.059950296514,162.557125400991,163.054300505468,
163.551475609945,164.048650714422,164.5458258189,165.043000923377,165.540176027854,
166.037351132331,166.504410640259),.UNSPECIFIED.);
#806=B_SPLINE_CURVE_WITH_KNOTS('',3,(#30241,#30242,#30243,#30244,#30245,
#30246,#30247,#30248,#30249,#30250,#30251,#30252,#30253,#30254,#30255,#30256,
#30257),.UNSPECIFIED.,.F.,.F.,(4,1,1,1,1,1,1,1,1,1,1,1,1,1,4),(153.9380400259,
154.051068742791,154.548243847269,155.045418951746,155.542594056223,156.0397691607,
156.536944265177,157.034119369655,157.531294474132,158.028469578609,158.525644683086,
159.022819787563,159.519994892041,160.017169996518,160.22122533308),
 .UNSPECIFIED.);
#807=B_SPLINE_CURVE_WITH_KNOTS('',3,(#30258,#30259,#30260,#30261,#30262,
#30263,#30264,#30265,#30266,#30267,#30268,#30269,#30270,#30271,#30272,#30273,
#30274),.UNSPECIFIED.,.F.,.F.,(4,1,1,1,1,1,1,1,1,1,1,1,1,1,4),(153.9380400259,
154.105148624878,154.602323729355,155.099498833833,155.59667393831,156.093849042787,
156.591024147264,157.088199251742,157.585374356219,158.082549460696,158.579724565173,
159.07689966965,159.574074774128,160.071249878605,160.22122533308),
 .UNSPECIFIED.);
#808=B_SPLINE_CURVE_WITH_KNOTS('',3,(#30279,#30280,#30281,#30282,#30283,
#30284,#30285,#30286,#30287,#30288,#30289,#30290,#30291,#30292,#30293,#30294),
 .UNSPECIFIED.,.F.,.F.,(4,1,1,1,1,1,1,1,1,1,1,1,1,4),(147.65485471872,148.084967489065,
148.582142593542,149.079317698019,149.576492802496,150.073667906974,150.570843011451,
151.068018115928,151.565193220405,152.062368324882,152.55954342936,153.056718533837,
153.553893638314,153.9380400259),.UNSPECIFIED.);
#809=B_SPLINE_CURVE_WITH_KNOTS('',3,(#30295,#30296,#30297,#30298,#30299,
#30300,#30301,#30302,#30303,#30304,#30305,#30306,#30307,#30308,#30309,#30310),
 .UNSPECIFIED.,.F.,.F.,(4,1,1,1,1,1,1,1,1,1,1,1,1,4),(147.65485471872,148.139047371152,
148.636222475629,149.133397580106,149.630572684583,150.12774778906,150.624922893538,
151.122097998015,151.619273102492,152.116448206969,152.613623311447,153.110798415924,
153.607973520401,153.9380400259),.UNSPECIFIED.);
#810=B_SPLINE_CURVE_WITH_KNOTS('',3,(#30315,#30316,#30317,#30318,#30319,
#30320,#30321,#30322,#30323,#30324,#30325,#30326,#30327,#30328,#30329,#30330,
#30331),.UNSPECIFIED.,.F.,.F.,(4,1,1,1,1,1,1,1,1,1,1,1,1,1,4),(141.371669411541,
141.621691130861,142.118866235338,142.616041339815,143.113216444293,143.61039154877,
144.107566653247,144.604741757724,145.101916862201,145.599091966679,146.096267071156,
146.593442175633,147.09061728011,147.587792384587,147.65485471872),
 .UNSPECIFIED.);
#811=B_SPLINE_CURVE_WITH_KNOTS('',3,(#30332,#30333,#30334,#30335,#30336,
#30337,#30338,#30339,#30340,#30341,#30342,#30343,#30344,#30345,#30346,#30347,
#30348),.UNSPECIFIED.,.F.,.F.,(4,1,1,1,1,1,1,1,1,1,1,1,1,1,4),(141.371669411541,
141.675771012948,142.172946117425,142.670121221902,143.167296326379,143.664471430857,
144.161646535334,144.658821639811,145.155996744288,145.653171848766,146.150346953243,
146.64752205772,147.144697162197,147.641872266674,147.65485471872),
 .UNSPECIFIED.);
#812=B_SPLINE_CURVE_WITH_KNOTS('',3,(#30353,#30354,#30355,#30356,#30357,
#30358,#30359,#30360,#30361,#30362,#30363,#30364,#30365,#30366,#30367,#30368,
#30369),.UNSPECIFIED.,.F.,.F.,(4,1,1,1,1,1,1,1,1,1,1,1,1,1,4),(135.088484104361,
135.158414772657,135.655589877134,136.152764981612,136.649940086089,137.147115190566,
137.644290295043,138.14146539952,138.638640503998,139.135815608475,139.632990712952,
140.130165817429,140.627340921906,141.124516026384,141.371669411541),
 .UNSPECIFIED.);
#813=B_SPLINE_CURVE_WITH_KNOTS('',3,(#30370,#30371,#30372,#30373,#30374,
#30375,#30376,#30377,#30378,#30379,#30380,#30381,#30382,#30383,#30384,#30385,
#30386),.UNSPECIFIED.,.F.,.F.,(4,1,1,1,1,1,1,1,1,1,1,1,1,1,4),(135.088484104361,
135.212494654744,135.709669759221,136.206844863698,136.704019968176,137.201195072653,
137.69837017713,138.195545281607,138.692720386085,139.189895490562,139.687070595039,
140.184245699516,140.681420803993,141.178595908471,141.371669411541),
 .UNSPECIFIED.);
#814=B_SPLINE_CURVE_WITH_KNOTS('',3,(#30391,#30392,#30393,#30394,#30395,
#30396,#30397,#30398,#30399,#30400,#30401,#30402,#30403,#30404,#30405,#30406),
 .UNSPECIFIED.,.F.,.F.,(4,1,1,1,1,1,1,1,1,1,1,1,1,4),(128.805298797182,
129.192313518931,129.689488623408,130.186663727885,130.683838832362,131.181013936839,
131.678189041317,132.175364145794,132.672539250271,133.169714354748,133.666889459226,
134.164064563703,134.66123966818,135.088484104361),.UNSPECIFIED.);
#815=B_SPLINE_CURVE_WITH_KNOTS('',3,(#30407,#30408,#30409,#30410,#30411,
#30412,#30413,#30414,#30415,#30416,#30417,#30418,#30419,#30420,#30421,#30422),
 .UNSPECIFIED.,.F.,.F.,(4,1,1,1,1,1,1,1,1,1,1,1,1,4),(128.805298797182,
129.246393401017,129.743568505495,130.240743609972,130.737918714449,131.235093818926,
131.732268923404,132.229444027881,132.726619132358,133.223794236835,133.720969341312,
134.21814444579,134.715319550267,135.088484104361),.UNSPECIFIED.);
#816=B_SPLINE_CURVE_WITH_KNOTS('',3,(#30427,#30428,#30429,#30430,#30431,
#30432,#30433,#30434,#30435,#30436,#30437,#30438,#30439,#30440,#30441,#30442,
#30443),.UNSPECIFIED.,.F.,.F.,(4,1,1,1,1,1,1,1,1,1,1,1,1,1,4),(122.522113490002,
122.729037160727,123.226212265204,123.723387369681,124.220562474158,124.717737578636,
125.214912683113,125.71208778759,126.209262892067,126.706437996544,127.203613101022,
127.700788205499,128.197963309976,128.695138414453,128.805298797182),
 .UNSPECIFIED.);
#817=B_SPLINE_CURVE_WITH_KNOTS('',3,(#30444,#30445,#30446,#30447,#30448,
#30449,#30450,#30451,#30452,#30453,#30454,#30455,#30456,#30457,#30458,#30459,
#30460),.UNSPECIFIED.,.F.,.F.,(4,1,1,1,1,1,1,1,1,1,1,1,1,1,4),(122.522113490002,
122.783117042814,123.280292147291,123.777467251768,124.274642356245,124.771817460723,
125.2689925652,125.766167669677,126.263342774154,126.760517878631,127.257692983109,
127.754868087586,128.252043192063,128.74921829654,128.805298797182),
 .UNSPECIFIED.);
#818=B_SPLINE_CURVE_WITH_KNOTS('',3,(#30465,#30466,#30467,#30468,#30469,
#30470,#30471,#30472,#30473,#30474,#30475,#30476,#30477,#30478,#30479,#30480,
#30481),.UNSPECIFIED.,.F.,.F.,(4,1,1,1,1,1,1,1,1,1,1,1,1,1,4),(116.238928182822,
116.265760802523,116.762935907,117.260111011477,117.757286115955,118.254461220432,
118.751636324909,119.248811429386,119.745986533863,120.243161638341,120.740336742818,
121.237511847295,121.734686951772,122.23186205625,122.522113490002),
 .UNSPECIFIED.);
#819=B_SPLINE_CURVE_WITH_KNOTS('',3,(#30482,#30483,#30484,#30485,#30486,
#30487,#30488,#30489,#30490,#30491,#30492,#30493,#30494,#30495,#30496,#30497,
#30498),.UNSPECIFIED.,.F.,.F.,(4,1,1,1,1,1,1,1,1,1,1,1,1,1,4),(116.238928182822,
116.31984068461,116.817015789087,117.314190893564,117.811365998042,118.308541102519,
118.805716206996,119.302891311473,119.80006641595,120.297241520428,120.794416624905,
121.291591729382,121.788766833859,122.285941938336,122.522113490002),
 .UNSPECIFIED.);
#820=B_SPLINE_CURVE_WITH_KNOTS('',3,(#30503,#30504,#30505,#30506,#30507,
#30508,#30509,#30510,#30511,#30512,#30513,#30514,#30515,#30516,#30517,#30518),
 .UNSPECIFIED.,.F.,.F.,(4,1,1,1,1,1,1,1,1,1,1,1,1,4),(109.955742875643,
110.299659548796,110.796834653274,111.294009757751,111.791184862228,112.288359966705,
112.785535071182,113.28271017566,113.779885280137,114.277060384614,114.774235489091,
115.271410593569,115.768585698046,116.238928182822),.UNSPECIFIED.);
#821=B_SPLINE_CURVE_WITH_KNOTS('',3,(#30519,#30520,#30521,#30522,#30523,
#30524,#30525,#30526,#30527,#30528,#30529,#30530,#30531,#30532,#30533,#30534),
 .UNSPECIFIED.,.F.,.F.,(4,1,1,1,1,1,1,1,1,1,1,1,1,4),(109.955742875643,
110.353739430883,110.850914535361,111.348089639838,111.845264744315,112.342439848792,
112.839614953269,113.336790057747,113.833965162224,114.331140266701,114.828315371178,
115.325490475655,115.822665580133,116.238928182822),.UNSPECIFIED.);
#822=B_SPLINE_CURVE_WITH_KNOTS('',3,(#30539,#30540,#30541,#30542,#30543,
#30544,#30545,#30546,#30547,#30548,#30549,#30550,#30551,#30552,#30553,#30554,
#30555),.UNSPECIFIED.,.F.,.F.,(4,1,1,1,1,1,1,1,1,1,1,1,1,1,4),(103.672557568463,
103.836383190593,104.33355829507,104.830733399547,105.327908504024,105.825083608501,
106.322258712979,106.819433817456,107.316608921933,107.81378402641,108.310959130888,
108.808134235365,109.305309339842,109.802484444319,109.955742875643),
 .UNSPECIFIED.);
#823=B_SPLINE_CURVE_WITH_KNOTS('',3,(#30556,#30557,#30558,#30559,#30560,
#30561,#30562,#30563,#30564,#30565,#30566,#30567,#30568,#30569,#30570,#30571,
#30572),.UNSPECIFIED.,.F.,.F.,(4,1,1,1,1,1,1,1,1,1,1,1,1,1,4),(103.672557568463,
103.89046307268,104.387638177157,104.884813281634,105.381988386111,105.879163490588,
106.376338595066,106.873513699543,107.37068880402,107.867863908497,108.365039012974,
108.862214117452,109.359389221929,109.856564326406,109.955742875643),
 .UNSPECIFIED.);
#824=B_SPLINE_CURVE_WITH_KNOTS('',3,(#30577,#30578,#30579,#30580,#30581,
#30582,#30583,#30584,#30585,#30586,#30587,#30588,#30589,#30590,#30591,#30592),
 .UNSPECIFIED.,.F.,.F.,(4,1,1,1,1,1,1,1,1,1,1,1,1,4),(97.3893722612839,
97.870281936866,98.3674570413433,98.8646321458205,99.3618072502977,99.8589823547749,
100.356157459252,100.853332563729,101.350507668207,101.847682772684,102.344857877161,
102.842032981638,103.339208086115,103.672557568463),.UNSPECIFIED.);
#825=B_SPLINE_CURVE_WITH_KNOTS('',3,(#30593,#30594,#30595,#30596,#30597,
#30598,#30599,#30600,#30601,#30602,#30603,#30604,#30605,#30606,#30607,#30608,
#30609),.UNSPECIFIED.,.F.,.F.,(4,1,1,1,1,1,1,1,1,1,1,1,1,1,4),(97.3893722612839,
97.4271867144758,97.924361818953,98.4215369234302,98.9187120279074,99.4158871323846,
99.9130622368618,100.410237341339,100.907412445816,101.404587550293,101.901762654771,
102.398937759248,102.896112863725,103.393287968202,103.672557568463),
 .UNSPECIFIED.);
#826=B_SPLINE_CURVE_WITH_KNOTS('',3,(#30614,#30615,#30616,#30617,#30618,
#30619,#30620,#30621,#30622,#30623,#30624,#30625,#30626,#30627,#30628,#30629,
#30630),.UNSPECIFIED.,.F.,.F.,(4,1,1,1,1,1,1,1,1,1,1,1,1,1,4),(91.1061869541042,
91.4070055786623,91.9041806831395,92.4013557876167,92.8985308920939,93.3957059965711,
93.8928811010483,94.3900562055255,94.8872313100028,95.38440641448,95.8815815189572,
96.3787566234344,96.8759317279116,97.3731068323888,97.3893722612839),
 .UNSPECIFIED.);
#827=B_SPLINE_CURVE_WITH_KNOTS('',3,(#30631,#30632,#30633,#30634,#30635,
#30636,#30637,#30638,#30639,#30640,#30641,#30642,#30643,#30644,#30645,#30646),
 .UNSPECIFIED.,.F.,.F.,(4,1,1,1,1,1,1,1,1,1,1,1,1,4),(91.1061869541042,
91.4610854607492,91.9582605652264,92.4554356697036,92.9526107741808,93.449785878658,
93.9469609831353,94.4441360876125,94.9413111920897,95.4384862965669,95.9356614010441,
96.4328365055213,96.9300116099986,97.3893722612839),.UNSPECIFIED.);
#828=B_SPLINE_CURVE_WITH_KNOTS('',3,(#30651,#30652,#30653,#30654,#30655,
#30656,#30657,#30658,#30659,#30660,#30661,#30662,#30663,#30664,#30665,#30666,
#30667),.UNSPECIFIED.,.F.,.F.,(4,1,1,1,1,1,1,1,1,1,1,1,1,1,4),(84.8230016469245,
84.9437292204585,85.4409043249357,85.9380794294129,86.4352545338901,86.9324296383673,
87.4296047428445,87.9267798473217,88.423954951799,88.9211300562762,89.4183051607534,
89.9154802652306,90.4126553697078,90.909830474185,91.1061869541042),
 .UNSPECIFIED.);
#829=B_SPLINE_CURVE_WITH_KNOTS('',3,(#30668,#30669,#30670,#30671,#30672,
#30673,#30674,#30675,#30676,#30677,#30678,#30679,#30680,#30681,#30682,#30683,
#30684),.UNSPECIFIED.,.F.,.F.,(4,1,1,1,1,1,1,1,1,1,1,1,1,1,4),(84.8230016469245,
84.9978091025454,85.4949842070226,85.9921593114998,86.4893344159771,86.9865095204543,
87.4836846249315,87.9808597294087,88.4780348338859,88.9752099383631,89.4723850428403,
89.9695601473175,90.4667352517948,90.963910356272,91.1061869541042),
 .UNSPECIFIED.);
#830=B_SPLINE_CURVE_WITH_KNOTS('',3,(#30689,#30690,#30691,#30692,#30693,
#30694,#30695,#30696,#30697,#30698,#30699,#30700,#30701,#30702,#30703,#30704),
 .UNSPECIFIED.,.F.,.F.,(4,1,1,1,1,1,1,1,1,1,1,1,1,4),(78.5398163397448,
78.9776279667319,79.4748030712091,79.9719781756863,80.4691532801635,80.9663283846407,
81.463503489118,81.9606785935952,82.4578536980724,82.9550288025496,83.4522039070268,
83.949379011504,84.4465541159813,84.8230016469245),.UNSPECIFIED.);
#831=B_SPLINE_CURVE_WITH_KNOTS('',3,(#30705,#30706,#30707,#30708,#30709,
#30710,#30711,#30712,#30713,#30714,#30715,#30716,#30717,#30718,#30719,#30720),
 .UNSPECIFIED.,.F.,.F.,(4,1,1,1,1,1,1,1,1,1,1,1,1,4),(78.5398163397448,
79.0317078488188,79.528882953296,80.0260580577733,80.5232331622505,81.0204082667277,
81.5175833712049,82.0147584756821,82.5119335801593,83.0091086846365,83.5062837891138,
84.003458893591,84.5006339980682,84.8230016469245),.UNSPECIFIED.);
#832=B_SPLINE_CURVE_WITH_KNOTS('',3,(#30725,#30726,#30727,#30728,#30729,
#30730,#30731,#30732,#30733,#30734,#30735,#30736,#30737,#30738,#30739,#30740,
#30741),.UNSPECIFIED.,.F.,.F.,(4,1,1,1,1,1,1,1,1,1,1,1,1,1,4),(72.2566310325651,
72.5143516085281,73.0115267130053,73.5087018174825,74.0058769219598,74.503052026437,
75.0002271309142,75.4974022353914,75.9945773398686,76.4917524443458,76.988927548823,
77.4861026533003,77.9832777577775,78.4804528622547,78.5398163397448),
 .UNSPECIFIED.);
#833=B_SPLINE_CURVE_WITH_KNOTS('',3,(#30742,#30743,#30744,#30745,#30746,
#30747,#30748,#30749,#30750,#30751,#30752,#30753,#30754,#30755,#30756,#30757,
#30758),.UNSPECIFIED.,.F.,.F.,(4,1,1,1,1,1,1,1,1,1,1,1,1,1,4),(72.2566310325651,
72.568431490615,73.0656065950923,73.5627816995695,74.0599568040467,74.5571319085239,
75.0543070130011,75.5514821174783,76.0486572219556,76.5458323264328,77.04300743091,
77.5401825353872,78.0373576398644,78.5345327443416,78.5398163397448),
 .UNSPECIFIED.);
#834=B_SPLINE_CURVE_WITH_KNOTS('',3,(#30763,#30764,#30765,#30766,#30767,
#30768,#30769,#30770,#30771,#30772,#30773,#30774,#30775,#30776,#30777,#30778,
#30779),.UNSPECIFIED.,.F.,.F.,(4,1,1,1,1,1,1,1,1,1,1,1,1,1,4),(65.9734457253859,
66.0510752503243,66.5482503548015,67.0454254592788,67.542600563756,68.0397756682332,
68.5369507727104,69.0341258771876,69.5313009816648,70.028476086142,70.5256511906192,
71.0228262950965,71.5200013995737,72.0171765040509,72.2566310325651),
 .UNSPECIFIED.);
#835=B_SPLINE_CURVE_WITH_KNOTS('',3,(#30780,#30781,#30782,#30783,#30784,
#30785,#30786,#30787,#30788,#30789,#30790,#30791,#30792,#30793,#30794,#30795,
#30796),.UNSPECIFIED.,.F.,.F.,(4,1,1,1,1,1,1,1,1,1,1,1,1,1,4),(65.9734457253859,
66.1051551324113,66.6023302368885,67.0995053413657,67.5966804458429,68.0938555503201,
68.5910306547973,69.0882057592745,69.5853808637518,70.082555968229,70.5797310727062,
71.0769061771834,71.5740812816606,72.0712563861378,72.2566310325651),
 .UNSPECIFIED.);
#836=B_SPLINE_CURVE_WITH_KNOTS('',3,(#30801,#30802,#30803,#30804,#30805,
#30806,#30807,#30808,#30809,#30810,#30811,#30812,#30813,#30814,#30815,#30816),
 .UNSPECIFIED.,.F.,.F.,(4,1,1,1,1,1,1,1,1,1,1,1,1,4),(59.6902604182062,
60.0849739965977,60.582149101075,61.0793242055522,61.5764993100294,62.0736744145066,
62.5708495189838,63.068024623461,63.5651997279382,64.0623748324155,64.5595499368927,
65.0567250413699,65.5539001458471,65.9734457253859),.UNSPECIFIED.);
#837=B_SPLINE_CURVE_WITH_KNOTS('',3,(#30817,#30818,#30819,#30820,#30821,
#30822,#30823,#30824,#30825,#30826,#30827,#30828,#30829,#30830,#30831,#30832),
 .UNSPECIFIED.,.F.,.F.,(4,1,1,1,1,1,1,1,1,1,1,1,1,4),(59.6902604182062,
60.1390538786847,60.6362289831619,61.1334040876391,61.6305791921163,62.1277542965935,
62.6249294010708,63.122104505548,63.6192796100252,64.1164547145024,64.6136298189796,
65.1108049234568,65.607980027934,65.9734457253859),.UNSPECIFIED.);
#838=B_SPLINE_CURVE_WITH_KNOTS('',3,(#30837,#30838,#30839,#30840,#30841,
#30842,#30843,#30844,#30845,#30846,#30847,#30848,#30849,#30850,#30851,#30852,
#30853),.UNSPECIFIED.,.F.,.F.,(4,1,1,1,1,1,1,1,1,1,1,1,1,1,4),(53.4070751110266,
53.621697638394,54.1188727428712,54.6160478473484,55.1132229518256,55.6103980563028,
56.10757316078,56.6047482652572,57.1019233697345,57.5990984742117,58.0962735786889,
58.5934486831661,59.0906237876433,59.5877988921205,59.6902604182062),
 .UNSPECIFIED.);
#839=B_SPLINE_CURVE_WITH_KNOTS('',3,(#30854,#30855,#30856,#30857,#30858,
#30859,#30860,#30861,#30862,#30863,#30864,#30865,#30866,#30867,#30868,#30869,
#30870),.UNSPECIFIED.,.F.,.F.,(4,1,1,1,1,1,1,1,1,1,1,1,1,1,4),(53.4070751110266,
53.6757775204809,54.1729526249581,54.6701277294353,55.1673028339125,55.6644779383898,
56.161653042867,56.6588281473442,57.1560032518214,57.6531783562986,58.1503534607758,
58.647528565253,59.1447036697303,59.6418787742075,59.6902604182062),
 .UNSPECIFIED.);
#840=B_SPLINE_CURVE_WITH_KNOTS('',3,(#30875,#30876,#30877,#30878,#30879,
#30880,#30881,#30882,#30883,#30884,#30885,#30886,#30887,#30888,#30889,#30890,
#30891),.UNSPECIFIED.,.F.,.F.,(4,1,1,1,1,1,1,1,1,1,1,1,1,1,4),(47.1238898038469,
47.1584212801902,47.6555963846674,48.1527714891446,48.6499465936218,49.147121698099,
49.6442968025762,50.1414719070535,50.6386470115307,51.1358221160079,51.6329972204851,
52.1301723249623,52.6273474294395,53.1245225339167,53.4070751110266),
 .UNSPECIFIED.);
#841=B_SPLINE_CURVE_WITH_KNOTS('',3,(#30892,#30893,#30894,#30895,#30896,
#30897,#30898,#30899,#30900,#30901,#30902,#30903,#30904,#30905,#30906,#30907,
#30908),.UNSPECIFIED.,.F.,.F.,(4,1,1,1,1,1,1,1,1,1,1,1,1,1,4),(47.1238898038469,
47.2125011622771,47.7096762667543,48.2068513712315,48.7040264757088,49.201201580186,
49.6983766846632,50.1955517891404,50.6927268936176,51.1899019980948,51.687077102572,
52.1842522070493,52.6814273115265,53.1786024160037,53.4070751110266),
 .UNSPECIFIED.);
#842=B_SPLINE_CURVE_WITH_KNOTS('',3,(#30913,#30914,#30915,#30916,#30917,
#30918,#30919,#30920,#30921,#30922,#30923,#30924,#30925,#30926,#30927,#30928),
 .UNSPECIFIED.,.F.,.F.,(4,1,1,1,1,1,1,1,1,1,1,1,1,4),(40.8407044966672,
41.1923200264636,41.6894951309408,42.186670235418,42.6838453398952,43.1810204443725,
43.6781955488497,44.1753706533269,44.6725457578041,45.1697208622813,45.6668959667585,
46.1640710712357,46.661246175713,47.1238898038469),.UNSPECIFIED.);
#843=B_SPLINE_CURVE_WITH_KNOTS('',3,(#30929,#30930,#30931,#30932,#30933,
#30934,#30935,#30936,#30937,#30938,#30939,#30940,#30941,#30942,#30943,#30944),
 .UNSPECIFIED.,.F.,.F.,(4,1,1,1,1,1,1,1,1,1,1,1,1,4),(40.8407044966672,
41.2463999085505,41.7435750130278,42.240750117505,42.7379252219822,43.2351003264594,
43.7322754309366,44.2294505354138,44.726625639891,45.2238007443683,45.7209758488455,
46.2181509533227,46.7153260577999,47.1238898038469),.UNSPECIFIED.);
#844=B_SPLINE_CURVE_WITH_KNOTS('',3,(#30949,#30950,#30951,#30952,#30953,
#30954,#30955,#30956,#30957,#30958,#30959,#30960,#30961,#30962,#30963,#30964,
#30965),.UNSPECIFIED.,.F.,.F.,(4,1,1,1,1,1,1,1,1,1,1,1,1,1,4),(34.557519189488,
34.7290436682598,35.226218772737,35.7233938772142,36.2205689816915,36.7177440861687,
37.2149191906459,37.7120942951231,38.2092693996003,38.7064445040775,39.2036196085547,
39.700794713032,40.1979698175092,40.6951449219864,40.8407044966672),
 .UNSPECIFIED.);
#845=B_SPLINE_CURVE_WITH_KNOTS('',3,(#30966,#30967,#30968,#30969,#30970,
#30971,#30972,#30973,#30974,#30975,#30976,#30977,#30978,#30979,#30980,#30981,
#30982),.UNSPECIFIED.,.F.,.F.,(4,1,1,1,1,1,1,1,1,1,1,1,1,1,4),(34.557519189488,
34.7831235503468,35.280298654824,35.7774737593012,36.2746488637784,36.7718239682556,
37.2689990727328,37.76617417721,38.2633492816873,38.7605243861645,39.2576994906417,
39.7548745951189,40.2520496995961,40.7492248040733,40.8407044966672),
 .UNSPECIFIED.);
#846=B_SPLINE_CURVE_WITH_KNOTS('',3,(#30987,#30988,#30989,#30990,#30991,
#30992,#30993,#30994,#30995,#30996,#30997,#30998,#30999,#31000,#31001,#31002),
 .UNSPECIFIED.,.F.,.F.,(4,1,1,1,1,1,1,1,1,1,1,1,1,4),(28.2743338823083,
28.7629424145332,29.2601175190104,29.7572926234877,30.2544677279649,30.7516428324421,
31.2488179369193,31.7459930413965,32.2431681458737,32.7403432503509,33.2375183548282,
33.7346934593054,34.2318685637826,34.557519189488),.UNSPECIFIED.);
#847=B_SPLINE_CURVE_WITH_KNOTS('',3,(#31003,#31004,#31005,#31006,#31007,
#31008,#31009,#31010,#31011,#31012,#31013,#31014,#31015,#31016,#31017,#31018,
#31019),.UNSPECIFIED.,.F.,.F.,(4,1,1,1,1,1,1,1,1,1,1,1,1,1,4),(28.2743338823083,
28.319847192143,28.8170222966202,29.3141974010974,29.8113725055746,30.3085476100518,
30.805722714529,31.3028978190063,31.8000729234835,32.2972480279607,32.7944231324379,
33.2915982369151,33.7887733413923,34.2859484458695,34.557519189488),
 .UNSPECIFIED.);
#848=B_SPLINE_CURVE_WITH_KNOTS('',3,(#31024,#31025,#31026,#31027,#31028,
#31029,#31030,#31031,#31032,#31033,#31034,#31035,#31036,#31037,#31038,#31039,
#31040),.UNSPECIFIED.,.F.,.F.,(4,1,1,1,1,1,1,1,1,1,1,1,1,1,4),(21.9911485751286,
22.2996660563294,22.7968411608067,23.2940162652839,23.7911913697611,24.2883664742383,
24.7855415787155,25.2827166831927,25.7798917876699,26.2770668921472,26.7742419966244,
27.2714171011016,27.7685922055788,28.265767310056,28.2743338823083),
 .UNSPECIFIED.);
#849=B_SPLINE_CURVE_WITH_KNOTS('',3,(#31041,#31042,#31043,#31044,#31045,
#31046,#31047,#31048,#31049,#31050,#31051,#31052,#31053,#31054,#31055,#31056),
 .UNSPECIFIED.,.F.,.F.,(4,1,1,1,1,1,1,1,1,1,1,1,1,4),(21.9911485751286,
22.3537459384164,22.8509210428936,23.3480961473708,23.845271251848,24.3424463563253,
24.8396214608025,25.3367965652797,25.8339716697569,26.3311467742341,26.8283218787113,
27.3254969831885,27.8226720876658,28.2743338823083),.UNSPECIFIED.);
#850=B_SPLINE_CURVE_WITH_KNOTS('',3,(#31062,#31063,#31064,#31065,#31066,
#31067),.UNSPECIFIED.,.F.,.F.,(4,1,1,4),(14.398944266781,14.8961193712582,
15.3932944757354,15.707963267949),.UNSPECIFIED.);
#851=B_SPLINE_CURVE_WITH_KNOTS('',3,(#31070,#31071,#31072,#31073,#31074,
#31075,#31076),.UNSPECIFIED.,.F.,.F.,(4,1,1,1,4),(13.8753896155273,14.344864384694,
14.8420394891712,15.3392145936484,15.707963267949),.UNSPECIFIED.);
#852=B_SPLINE_CURVE_WITH_KNOTS('',3,(#31082,#31083,#31084,#31085,#31086,
#31087,#31088),.UNSPECIFIED.,.F.,.F.,(4,3,4),(252.636431288351,252.845104747016,
253.343813040403),.UNSPECIFIED.);
#853=B_SPLINE_CURVE_WITH_KNOTS('',3,(#31096,#31097,#31098,#31099,#31100,
#31101,#31102,#31103,#31104,#31105,#31106,#31107,#31108,#31109,#31110,#31111),
 .UNSPECIFIED.,.F.,.F.,(4,3,3,3,3,4),(-251.327412287183,-250.85027157347,
-250.351563280083,-249.852854986696,-249.35414669331,-248.893201385645),
 .UNSPECIFIED.);
#854=B_SPLINE_CURVE_WITH_KNOTS('',3,(#31116,#31117,#31118,#31119,#31120,
#31121,#31122,#31123,#31124,#31125,#31126,#31127,#31128,#31129,#31130,#31131,
#31132,#31133,#31134,#31135,#31136,#31137,#31138,#31139,#31140,#31141,#31142,
#31143,#31144,#31145,#31146,#31147,#31148,#31149,#31150,#31151,#31152,#31153,
#31154,#31155,#31156,#31157,#31158),.UNSPECIFIED.,.F.,.F.,(4,3,3,3,3,3,
3,3,3,3,3,3,3,3,4),(246.353245981172,246.36189693299,246.860605226377,247.359313519763,
247.85802181315,248.356730106537,248.855438399923,249.35414669331,249.852854986696,
250.351563280083,250.85027157347,251.348979866856,251.847688160243,252.346396453629,
252.636431288351),.UNSPECIFIED.);
#855=B_SPLINE_CURVE_WITH_KNOTS('',3,(#31159,#31160,#31161,#31162,#31163,
#31164,#31165,#31166,#31167,#31168,#31169,#31170,#31171,#31172,#31173,#31174,
#31175,#31176,#31177,#31178,#31179,#31180,#31181,#31182,#31183,#31184,#31185,
#31186,#31187,#31188,#31189,#31190,#31191,#31192,#31193,#31194,#31195,#31196,
#31197,#31198,#31199,#31200,#31201),.UNSPECIFIED.,.F.,.F.,(4,3,3,3,3,3,
3,3,3,3,3,3,3,3,4),(-248.893201385645,-248.855438399923,-248.356730106536,
-247.85802181315,-247.359313519763,-246.860605226377,-246.36189693299,-245.863188639603,
-245.364480346217,-244.86577205283,-244.367063759444,-243.868355466057,
-243.36964717267,-242.870938879284,-242.610016078465),.UNSPECIFIED.);
#856=B_SPLINE_CURVE_WITH_KNOTS('',3,(#31206,#31207,#31208,#31209,#31210,
#31211,#31212,#31213,#31214,#31215,#31216,#31217,#31218,#31219,#31220,#31221,
#31222,#31223,#31224,#31225,#31226,#31227,#31228,#31229,#31230,#31231,#31232,
#31233,#31234,#31235,#31236,#31237,#31238,#31239,#31240,#31241,#31242,#31243,
#31244,#31245),.UNSPECIFIED.,.F.,.F.,(4,3,3,3,3,3,3,3,3,3,3,3,3,4),(240.070060673992,
240.377397412351,240.876105705737,241.374813999124,241.873522292511,242.372230585897,
242.870938879284,243.36964717267,243.868355466057,244.367063759444,244.86577205283,
245.364480346217,245.863188639603,246.353245981172),.UNSPECIFIED.);
#857=B_SPLINE_CURVE_WITH_KNOTS('',3,(#31246,#31247,#31248,#31249,#31250,
#31251,#31252,#31253,#31254,#31255,#31256,#31257,#31258,#31259,#31260,#31261,
#31262,#31263,#31264,#31265,#31266,#31267,#31268,#31269,#31270,#31271,#31272,
#31273,#31274,#31275,#31276,#31277,#31278,#31279,#31280,#31281,#31282,#31283,
#31284,#31285,#31286,#31287,#31288),.UNSPECIFIED.,.F.,.F.,(4,3,3,3,3,3,
3,3,3,3,3,3,3,3,4),(-242.610016078465,-242.372230585897,-241.87352229251,
-241.374813999124,-240.876105705737,-240.377397412351,-239.878689118964,
-239.379980825577,-238.881272532191,-238.382564238804,-237.883855945417,
-237.385147652031,-236.886439358644,-236.387731065258,-236.326830771286),
 .UNSPECIFIED.);
#858=B_SPLINE_CURVE_WITH_KNOTS('',3,(#31293,#31294,#31295,#31296,#31297,
#31298,#31299,#31300,#31301,#31302,#31303,#31304,#31305,#31306,#31307,#31308,
#31309,#31310,#31311,#31312,#31313,#31314,#31315,#31316,#31317,#31318,#31319,
#31320,#31321,#31322,#31323,#31324,#31325,#31326,#31327,#31328,#31329,#31330,
#31331,#31332,#31333,#31334,#31335),.UNSPECIFIED.,.F.,.F.,(4,3,3,3,3,3,
3,3,3,3,3,3,3,3,4),(233.786875366813,233.894189598325,234.392897891711,
234.891606185098,235.390314478484,235.889022771871,236.387731065258,236.886439358644,
237.385147652031,237.883855945418,238.382564238804,238.881272532191,239.379980825577,
239.878689118964,240.070060673992),.UNSPECIFIED.);
#859=B_SPLINE_CURVE_WITH_KNOTS('',3,(#31336,#31337,#31338,#31339,#31340,
#31341,#31342,#31343,#31344,#31345,#31346,#31347,#31348,#31349,#31350,#31351,
#31352,#31353,#31354,#31355,#31356,#31357,#31358,#31359,#31360,#31361,#31362,
#31363,#31364,#31365,#31366,#31367,#31368,#31369,#31370,#31371,#31372,#31373,
#31374,#31375),.UNSPECIFIED.,.F.,.F.,(4,3,3,3,3,3,3,3,3,3,3,3,3,4),(-236.326830771286,
-235.889022771871,-235.390314478484,-234.891606185098,-234.392897891711,
-233.894189598325,-233.395481304938,-232.896773011551,-232.398064718165,
-231.899356424778,-231.400648131391,-230.901939838005,-230.403231544618,
-230.043645464106),.UNSPECIFIED.);
#860=B_SPLINE_CURVE_WITH_KNOTS('',3,(#31380,#31381,#31382,#31383,#31384,
#31385,#31386,#31387,#31388,#31389,#31390,#31391,#31392,#31393,#31394,#31395,
#31396,#31397,#31398,#31399,#31400,#31401,#31402,#31403,#31404,#31405,#31406,
#31407,#31408,#31409,#31410,#31411,#31412,#31413,#31414,#31415,#31416,#31417,
#31418,#31419),.UNSPECIFIED.,.F.,.F.,(4,3,3,3,3,3,3,3,3,3,3,3,3,4),(227.503690059633,
227.909690077685,228.408398371072,228.907106664458,229.405814957845,229.904523251232,
230.403231544618,230.901939838005,231.400648131391,231.899356424778,232.398064718165,
232.896773011551,233.395481304938,233.786875366813),.UNSPECIFIED.);
#861=B_SPLINE_CURVE_WITH_KNOTS('',3,(#31420,#31421,#31422,#31423,#31424,
#31425,#31426,#31427,#31428,#31429,#31430,#31431,#31432,#31433,#31434,#31435,
#31436,#31437,#31438,#31439,#31440,#31441,#31442,#31443,#31444,#31445,#31446,
#31447,#31448,#31449,#31450,#31451,#31452,#31453,#31454,#31455,#31456,#31457,
#31458,#31459,#31460,#31461,#31462),.UNSPECIFIED.,.F.,.F.,(4,3,3,3,3,3,
3,3,3,3,3,3,3,3,4),(-230.043645464106,-229.904523251232,-229.405814957845,
-228.907106664458,-228.408398371072,-227.909690077685,-227.410981784298,
-226.912273490912,-226.413565197525,-225.914856904139,-225.416148610752,
-224.917440317365,-224.418732023979,-223.920023730592,-223.760460156926),
 .UNSPECIFIED.);
#862=B_SPLINE_CURVE_WITH_KNOTS('',3,(#31467,#31468,#31469,#31470,#31471,
#31472,#31473,#31474,#31475,#31476,#31477,#31478,#31479,#31480,#31481,#31482,
#31483,#31484,#31485,#31486,#31487,#31488,#31489,#31490,#31491,#31492,#31493,
#31494,#31495,#31496,#31497,#31498,#31499,#31500,#31501,#31502,#31503,#31504,
#31505,#31506,#31507,#31508,#31509),.UNSPECIFIED.,.F.,.F.,(4,3,3,3,3,3,
3,3,3,3,3,3,3,3,4),(221.220504752453,221.426482263659,221.925190557046,
222.423898850432,222.922607143819,223.421315437206,223.920023730592,224.418732023979,
224.917440317365,225.416148610752,225.914856904139,226.413565197525,226.912273490912,
227.410981784299,227.503690059633),.UNSPECIFIED.);
#863=B_SPLINE_CURVE_WITH_KNOTS('',3,(#31510,#31511,#31512,#31513,#31514,
#31515,#31516,#31517,#31518,#31519,#31520,#31521,#31522,#31523,#31524,#31525,
#31526,#31527,#31528,#31529,#31530,#31531,#31532,#31533,#31534,#31535,#31536,
#31537,#31538,#31539,#31540,#31541,#31542,#31543,#31544,#31545,#31546,#31547,
#31548,#31549),.UNSPECIFIED.,.F.,.F.,(4,3,3,3,3,3,3,3,3,3,3,3,3,4),(-223.760460156926,
-223.421315437206,-222.922607143819,-222.423898850432,-221.925190557046,
-221.426482263659,-220.927773970272,-220.429065676886,-219.930357383499,
-219.431649090113,-218.932940796726,-218.434232503339,-217.935524209953,
-217.477274849747),.UNSPECIFIED.);
#864=B_SPLINE_CURVE_WITH_KNOTS('',3,(#31554,#31555,#31556,#31557,#31558,
#31559,#31560,#31561,#31562,#31563,#31564,#31565,#31566,#31567,#31568,#31569,
#31570,#31571,#31572,#31573,#31574,#31575,#31576,#31577,#31578,#31579,#31580,
#31581,#31582,#31583,#31584,#31585,#31586,#31587,#31588,#31589,#31590,#31591,
#31592,#31593,#31594,#31595,#31596),.UNSPECIFIED.,.F.,.F.,(4,3,3,3,3,3,
3,3,3,3,3,3,3,3,4),(214.937319445274,214.943274449633,215.44198274302,215.940691036406,
216.439399329793,216.93810762318,217.436815916566,217.935524209953,218.434232503339,
218.932940796726,219.431649090113,219.930357383499,220.429065676886,220.927773970272,
221.220504752453),.UNSPECIFIED.);
#865=B_SPLINE_CURVE_WITH_KNOTS('',3,(#31597,#31598,#31599,#31600,#31601,
#31602,#31603,#31604,#31605,#31606,#31607,#31608,#31609,#31610,#31611,#31612,
#31613,#31614,#31615,#31616,#31617,#31618,#31619,#31620,#31621,#31622,#31623,
#31624,#31625,#31626,#31627,#31628,#31629,#31630,#31631,#31632,#31633,#31634,
#31635,#31636,#31637,#31638,#31639),.UNSPECIFIED.,.F.,.F.,(4,3,3,3,3,3,
3,3,3,3,3,3,3,3,4),(-217.477274849747,-217.436815916566,-216.938107623179,
-216.439399329793,-215.940691036406,-215.44198274302,-214.943274449633,
-214.444566156246,-213.94585786286,-213.447149569473,-212.948441276087,
-212.4497329827,-211.951024689313,-211.452316395927,-211.194089542567),
 .UNSPECIFIED.);
#866=B_SPLINE_CURVE_WITH_KNOTS('',3,(#31644,#31645,#31646,#31647,#31648,
#31649,#31650,#31651,#31652,#31653,#31654,#31655,#31656,#31657,#31658,#31659,
#31660,#31661,#31662,#31663,#31664,#31665,#31666,#31667,#31668,#31669,#31670,
#31671,#31672,#31673,#31674,#31675,#31676,#31677,#31678,#31679,#31680,#31681,
#31682,#31683),.UNSPECIFIED.,.F.,.F.,(4,3,3,3,3,3,3,3,3,3,3,3,3,4),(208.654134138094,
208.958774928994,209.45748322238,209.956191515767,210.454899809153,210.95360810254,
211.452316395927,211.951024689313,212.4497329827,212.948441276087,213.447149569473,
213.94585786286,214.444566156246,214.937319445274),.UNSPECIFIED.);
#867=B_SPLINE_CURVE_WITH_KNOTS('',3,(#31684,#31685,#31686,#31687,#31688,
#31689,#31690,#31691,#31692,#31693,#31694,#31695,#31696,#31697,#31698,#31699,
#31700,#31701,#31702,#31703,#31704,#31705,#31706,#31707,#31708,#31709,#31710,
#31711,#31712,#31713,#31714,#31715,#31716,#31717,#31718,#31719,#31720,#31721,
#31722,#31723,#31724,#31725,#31726),.UNSPECIFIED.,.F.,.F.,(4,3,3,3,3,3,
3,3,3,3,3,3,3,3,4),(-211.194089542567,-210.95360810254,-210.454899809153,
-209.956191515767,-209.45748322238,-208.958774928994,-208.460066635607,
-207.96135834222,-207.462650048834,-206.963941755447,-206.46523346206,-205.966525168674,
-205.467816875287,-204.969108581901,-204.910904235388),.UNSPECIFIED.);
#868=B_SPLINE_CURVE_WITH_KNOTS('',3,(#31731,#31732,#31733,#31734,#31735,
#31736,#31737,#31738,#31739,#31740,#31741,#31742,#31743,#31744,#31745,#31746,
#31747,#31748,#31749,#31750,#31751,#31752,#31753,#31754,#31755,#31756,#31757,
#31758,#31759,#31760,#31761,#31762,#31763,#31764,#31765,#31766,#31767,#31768,
#31769,#31770,#31771,#31772,#31773),.UNSPECIFIED.,.F.,.F.,(4,3,3,3,3,3,
3,3,3,3,3,3,3,3,4),(202.370948830915,202.475567114968,202.974275408354,
203.472983701741,203.971691995127,204.470400288514,204.969108581901,205.467816875287,
205.966525168674,206.46523346206,206.963941755447,207.462650048834,207.96135834222,
208.460066635607,208.654134138094),.UNSPECIFIED.);
#869=B_SPLINE_CURVE_WITH_KNOTS('',3,(#31774,#31775,#31776,#31777,#31778,
#31779,#31780,#31781,#31782,#31783,#31784,#31785,#31786,#31787,#31788,#31789,
#31790,#31791,#31792,#31793,#31794,#31795,#31796,#31797,#31798,#31799,#31800,
#31801,#31802,#31803,#31804,#31805,#31806,#31807,#31808,#31809,#31810,#31811,
#31812,#31813),.UNSPECIFIED.,.F.,.F.,(4,3,3,3,3,3,3,3,3,3,3,3,3,4),(-204.910904235388,
-204.470400288514,-203.971691995127,-203.472983701741,-202.974275408354,
-202.475567114968,-201.976858821581,-201.478150528194,-200.979442234808,
-200.480733941421,-199.982025648034,-199.483317354648,-198.984609061261,
-198.627718928208),.UNSPECIFIED.);
#870=B_SPLINE_CURVE_WITH_KNOTS('',3,(#31818,#31819,#31820,#31821,#31822,
#31823,#31824,#31825,#31826,#31827,#31828,#31829,#31830,#31831,#31832,#31833,
#31834,#31835,#31836,#31837,#31838,#31839,#31840,#31841,#31842,#31843,#31844,
#31845,#31846,#31847,#31848,#31849,#31850,#31851,#31852,#31853,#31854,#31855,
#31856,#31857),.UNSPECIFIED.,.F.,.F.,(4,3,3,3,3,3,3,3,3,3,3,3,3,4),(196.087763523735,
196.491067594328,196.989775887715,197.488484181101,197.987192474488,198.485900767875,
198.984609061261,199.483317354648,199.982025648034,200.480733941421,200.979442234808,
201.478150528194,201.976858821581,202.370948830915),.UNSPECIFIED.);
#871=B_SPLINE_CURVE_WITH_KNOTS('',3,(#31858,#31859,#31860,#31861,#31862,
#31863,#31864,#31865,#31866,#31867,#31868,#31869,#31870,#31871,#31872,#31873,
#31874,#31875,#31876,#31877,#31878,#31879,#31880,#31881,#31882,#31883,#31884,
#31885,#31886,#31887,#31888,#31889,#31890,#31891,#31892,#31893,#31894,#31895,
#31896,#31897,#31898,#31899,#31900),.UNSPECIFIED.,.F.,.F.,(4,3,3,3,3,3,
3,3,3,3,3,3,3,3,4),(-198.627718928208,-198.485900767875,-197.987192474488,
-197.488484181101,-196.989775887715,-196.491067594328,-195.992359300941,
-195.493651007555,-194.994942714168,-194.496234420782,-193.997526127395,
-193.498817834008,-193.000109540622,-192.501401247235,-192.344533621029),
 .UNSPECIFIED.);
#872=B_SPLINE_CURVE_WITH_KNOTS('',3,(#31905,#31906,#31907,#31908,#31909,
#31910,#31911,#31912,#31913,#31914,#31915,#31916,#31917,#31918,#31919,#31920,
#31921,#31922,#31923,#31924,#31925,#31926,#31927,#31928,#31929,#31930,#31931,
#31932,#31933,#31934,#31935,#31936,#31937,#31938,#31939,#31940,#31941,#31942,
#31943,#31944,#31945,#31946,#31947),.UNSPECIFIED.,.F.,.F.,(4,3,3,3,3,3,
3,3,3,3,3,3,3,3,4),(189.804578216556,190.007859780302,190.506568073689,
191.005276367075,191.503984660462,192.002692953849,192.501401247235,193.000109540622,
193.498817834008,193.997526127395,194.496234420782,194.994942714168,195.493651007555,
195.992359300941,196.087763523735),.UNSPECIFIED.);
#873=B_SPLINE_CURVE_WITH_KNOTS('',3,(#31948,#31949,#31950,#31951,#31952,
#31953,#31954,#31955,#31956,#31957,#31958,#31959,#31960,#31961,#31962,#31963,
#31964,#31965,#31966,#31967,#31968,#31969,#31970,#31971,#31972,#31973,#31974,
#31975,#31976,#31977,#31978,#31979,#31980,#31981,#31982,#31983,#31984,#31985,
#31986,#31987),.UNSPECIFIED.,.F.,.F.,(4,3,3,3,3,3,3,3,3,3,3,3,3,4),(-192.344533621029,
-192.002692953848,-191.503984660462,-191.005276367075,-190.506568073689,
-190.007859780302,-189.509151486915,-189.010443193529,-188.511734900142,
-188.013026606756,-187.514318313369,-187.015610019982,-186.516901726596,
-186.061348313849),.UNSPECIFIED.);
#874=B_SPLINE_CURVE_WITH_KNOTS('',3,(#31992,#31993,#31994,#31995,#31996,
#31997,#31998,#31999,#32000,#32001,#32002,#32003,#32004,#32005,#32006,#32007,
#32008,#32009,#32010,#32011,#32012,#32013,#32014,#32015,#32016,#32017,#32018,
#32019,#32020,#32021,#32022,#32023,#32024,#32025,#32026,#32027,#32028,#32029,
#32030,#32031,#32032,#32033,#32034),.UNSPECIFIED.,.F.,.F.,(4,3,3,3,3,3,
3,3,3,3,3,3,3,3,4),(183.521392909376,183.524651966276,184.023360259663,
184.522068553049,185.020776846436,185.519485139823,186.018193433209,186.516901726596,
187.015610019982,187.514318313369,188.013026606756,188.511734900142,189.010443193529,
189.509151486915,189.804578216556),.UNSPECIFIED.);
#875=B_SPLINE_CURVE_WITH_KNOTS('',3,(#32035,#32036,#32037,#32038,#32039,
#32040,#32041,#32042,#32043,#32044,#32045,#32046,#32047,#32048,#32049,#32050,
#32051,#32052,#32053,#32054,#32055,#32056,#32057,#32058,#32059,#32060,#32061,
#32062,#32063,#32064,#32065,#32066,#32067,#32068,#32069,#32070,#32071,#32072,
#32073,#32074,#32075,#32076,#32077),.UNSPECIFIED.,.F.,.F.,(4,3,3,3,3,3,
3,3,3,3,3,3,3,3,4),(-186.061348313849,-186.018193433209,-185.519485139822,
-185.020776846436,-184.522068553049,-184.023360259663,-183.524651966276,
-183.025943672889,-182.527235379503,-182.028527086116,-181.529818792729,
-181.031110499343,-180.532402205956,-180.03369391257,-179.77816300667),
 .UNSPECIFIED.);
#876=B_SPLINE_CURVE_WITH_KNOTS('',3,(#32082,#32083,#32084,#32085,#32086,
#32087,#32088,#32089,#32090,#32091,#32092,#32093,#32094,#32095,#32096,#32097,
#32098,#32099,#32100,#32101,#32102,#32103,#32104,#32105,#32106,#32107,#32108,
#32109,#32110,#32111,#32112,#32113,#32114,#32115,#32116,#32117,#32118,#32119,
#32120,#32121),.UNSPECIFIED.,.F.,.F.,(4,3,3,3,3,3,3,3,3,3,3,3,3,4),(177.238207602196,
177.540152445637,178.038860739023,178.53756903241,179.036277325796,179.534985619183,
180.03369391257,180.532402205956,181.031110499343,181.52981879273,182.028527086116,
182.527235379503,183.025943672889,183.521392909376),.UNSPECIFIED.);
#877=B_SPLINE_CURVE_WITH_KNOTS('',3,(#32122,#32123,#32124,#32125,#32126,
#32127,#32128,#32129,#32130,#32131,#32132,#32133,#32134,#32135,#32136,#32137,
#32138,#32139,#32140,#32141,#32142,#32143,#32144,#32145,#32146,#32147,#32148,
#32149,#32150,#32151,#32152,#32153,#32154,#32155,#32156,#32157,#32158,#32159,
#32160,#32161,#32162,#32163,#32164),.UNSPECIFIED.,.F.,.F.,(4,3,3,3,3,3,
3,3,3,3,3,3,3,3,4),(-179.77816300667,-179.534985619183,-179.036277325796,
-178.53756903241,-178.038860739023,-177.540152445637,-177.04144415225,-176.542735858863,
-176.044027565477,-175.54531927209,-175.046610978703,-174.547902685317,
-174.04919439193,-173.550486098544,-173.49497769949),.UNSPECIFIED.);
#878=B_SPLINE_CURVE_WITH_KNOTS('',3,(#32169,#32170,#32171,#32172,#32173,
#32174,#32175,#32176,#32177,#32178,#32179,#32180,#32181,#32182,#32183,#32184,
#32185,#32186,#32187,#32188,#32189,#32190,#32191,#32192,#32193,#32194,#32195,
#32196,#32197,#32198,#32199,#32200,#32201,#32202,#32203,#32204,#32205,#32206,
#32207,#32208,#32209,#32210,#32211),.UNSPECIFIED.,.F.,.F.,(4,3,3,3,3,3,
3,3,3,3,3,3,3,3,4),(170.955022295017,171.056944631611,171.555652924997,
172.054361218384,172.55306951177,173.051777805157,173.550486098544,174.04919439193,
174.547902685317,175.046610978703,175.54531927209,176.044027565477,176.542735858863,
177.04144415225,177.238207602196),.UNSPECIFIED.);
#879=B_SPLINE_CURVE_WITH_KNOTS('',3,(#32212,#32213,#32214,#32215,#32216,
#32217,#32218,#32219,#32220,#32221,#32222,#32223,#32224,#32225,#32226,#32227,
#32228,#32229,#32230,#32231,#32232,#32233,#32234,#32235,#32236,#32237,#32238,
#32239,#32240,#32241,#32242,#32243,#32244,#32245,#32246,#32247,#32248,#32249,
#32250,#32251),.UNSPECIFIED.,.F.,.F.,(4,3,3,3,3,3,3,3,3,3,3,3,3,4),(-173.49497769949,
-173.051777805157,-172.55306951177,-172.054361218384,-171.555652924997,
-171.05694463161,-170.558236338224,-170.059528044837,-169.560819751451,
-169.062111458064,-168.563403164677,-168.064694871291,-167.565986577904,
-167.21179239231),.UNSPECIFIED.);
#880=B_SPLINE_CURVE_WITH_KNOTS('',3,(#32256,#32257,#32258,#32259,#32260,
#32261,#32262,#32263,#32264,#32265,#32266,#32267,#32268,#32269,#32270,#32271,
#32272,#32273,#32274,#32275,#32276,#32277,#32278,#32279,#32280,#32281,#32282,
#32283,#32284,#32285,#32286,#32287,#32288,#32289,#32290,#32291,#32292,#32293,
#32294,#32295),.UNSPECIFIED.,.F.,.F.,(4,3,3,3,3,3,3,3,3,3,3,3,3,4),(164.671836987837,
165.072445110971,165.571153404358,166.069861697744,166.568569991131,167.067278284518,
167.565986577904,168.064694871291,168.563403164677,169.062111458064,169.560819751451,
170.059528044837,170.558236338224,170.955022295017),.UNSPECIFIED.);
#881=B_SPLINE_CURVE_WITH_KNOTS('',3,(#32296,#32297,#32298,#32299,#32300,
#32301,#32302,#32303,#32304,#32305,#32306,#32307,#32308,#32309,#32310,#32311,
#32312,#32313,#32314,#32315,#32316,#32317,#32318,#32319,#32320,#32321,#32322,
#32323,#32324,#32325,#32326,#32327,#32328,#32329,#32330,#32331,#32332,#32333,
#32334,#32335,#32336,#32337,#32338),.UNSPECIFIED.,.F.,.F.,(4,3,3,3,3,3,
3,3,3,3,3,3,3,3,4),(-167.21179239231,-167.067278284517,-166.568569991131,
-166.069861697744,-165.571153404358,-165.072445110971,-164.573736817584,
-164.075028524198,-163.576320230811,-163.077611937425,-162.578903644038,
-162.080195350651,-161.581487057265,-161.082778763878,-160.928607085131),
 .UNSPECIFIED.);
#882=B_SPLINE_CURVE_WITH_KNOTS('',3,(#32343,#32344,#32345,#32346,#32347,
#32348,#32349,#32350,#32351,#32352,#32353,#32354,#32355,#32356,#32357,#32358,
#32359,#32360,#32361,#32362,#32363,#32364,#32365,#32366,#32367,#32368,#32369,
#32370,#32371,#32372,#32373,#32374,#32375,#32376,#32377,#32378,#32379,#32380,
#32381,#32382,#32383,#32384,#32385),.UNSPECIFIED.,.F.,.F.,(4,3,3,3,3,3,
3,3,3,3,3,3,3,3,4),(158.388651680658,158.589237296945,159.087945590332,
159.586653883718,160.085362177105,160.584070470491,161.082778763878,161.581487057265,
162.080195350651,162.578903644038,163.077611937425,163.576320230811,164.075028524198,
164.573736817584,164.671836987837),.UNSPECIFIED.);
#883=B_SPLINE_CURVE_WITH_KNOTS('',3,(#32386,#32387,#32388,#32389,#32390,
#32391,#32392,#32393,#32394,#32395,#32396,#32397,#32398,#32399,#32400,#32401,
#32402,#32403,#32404,#32405,#32406,#32407,#32408,#32409,#32410,#32411,#32412,
#32413,#32414,#32415,#32416,#32417,#32418,#32419,#32420,#32421,#32422,#32423,
#32424,#32425),.UNSPECIFIED.,.F.,.F.,(4,3,3,3,3,3,3,3,3,3,3,3,3,4),(-160.928607085131,
-160.584070470491,-160.085362177105,-159.586653883718,-159.087945590332,
-158.589237296945,-158.090529003558,-157.591820710172,-157.093112416785,
-156.594404123399,-156.095695830012,-155.596987536625,-155.098279243239,
-154.645421777951),.UNSPECIFIED.);
#884=B_SPLINE_CURVE_WITH_KNOTS('',3,(#32430,#32431,#32432,#32433,#32434,
#32435,#32436,#32437,#32438,#32439,#32440,#32441,#32442,#32443,#32444,#32445,
#32446,#32447,#32448,#32449,#32450,#32451,#32452,#32453,#32454,#32455,#32456,
#32457,#32458,#32459,#32460,#32461,#32462,#32463,#32464,#32465,#32466,#32467,
#32468,#32469),.UNSPECIFIED.,.F.,.F.,(4,3,3,3,3,3,3,3,3,3,3,3,3,4),(152.105466373478,
152.604737776306,153.103446069692,153.602154363079,154.100862656465,154.599570949852,
155.098279243239,155.596987536625,156.095695830012,156.594404123399,157.093112416785,
157.591820710172,158.090529003558,158.388651680658),.UNSPECIFIED.);
#885=B_SPLINE_CURVE_WITH_KNOTS('',3,(#32470,#32471,#32472,#32473,#32474,
#32475,#32476,#32477,#32478,#32479,#32480,#32481,#32482,#32483,#32484,#32485,
#32486,#32487,#32488,#32489,#32490,#32491,#32492,#32493,#32494,#32495,#32496,
#32497,#32498,#32499,#32500,#32501,#32502,#32503,#32504,#32505,#32506,#32507,
#32508,#32509,#32510,#32511,#32512),.UNSPECIFIED.,.F.,.F.,(4,3,3,3,3,3,
3,3,3,3,3,3,3,3,4),(-154.645421777951,-154.599570949852,-154.100862656465,
-153.602154363079,-153.103446069692,-152.604737776306,-152.106029482919,
-151.607321189532,-151.108612896146,-150.609904602759,-150.111196309372,
-149.612488015986,-149.113779722599,-148.615071429213,-148.362236470772),
 .UNSPECIFIED.);
#886=B_SPLINE_CURVE_WITH_KNOTS('',3,(#32517,#32518,#32519,#32520,#32521,
#32522,#32523,#32524,#32525,#32526,#32527,#32528,#32529,#32530,#32531,#32532,
#32533,#32534,#32535,#32536,#32537,#32538,#32539,#32540,#32541,#32542,#32543,
#32544,#32545,#32546,#32547,#32548,#32549,#32550,#32551,#32552,#32553,#32554,
#32555,#32556),.UNSPECIFIED.,.F.,.F.,(4,3,3,3,3,3,3,3,3,3,3,3,3,4),(145.822281066299,
146.121529962279,146.620238255666,147.118946549053,147.617654842439,148.116363135826,
148.615071429213,149.113779722599,149.612488015986,150.111196309372,150.609904602759,
151.108612896146,151.607321189532,152.105466373478),.UNSPECIFIED.);
#887=B_SPLINE_CURVE_WITH_KNOTS('',3,(#32557,#32558,#32559,#32560,#32561,
#32562,#32563,#32564,#32565,#32566,#32567,#32568,#32569,#32570,#32571,#32572,
#32573,#32574,#32575,#32576,#32577,#32578,#32579,#32580,#32581,#32582,#32583,
#32584,#32585,#32586,#32587,#32588,#32589,#32590,#32591,#32592,#32593,#32594,
#32595,#32596,#32597,#32598,#32599),.UNSPECIFIED.,.F.,.F.,(4,3,3,3,3,3,
3,3,3,3,3,3,3,3,4),(-148.362236470772,-148.116363135826,-147.617654842439,
-147.118946549053,-146.620238255666,-146.12152996228,-145.622821668893,
-145.124113375506,-144.62540508212,-144.126696788733,-143.627988495346,
-143.12928020196,-142.630571908573,-142.131863615187,-142.079051163592),
 .UNSPECIFIED.);
#888=B_SPLINE_CURVE_WITH_KNOTS('',3,(#32604,#32605,#32606,#32607,#32608,
#32609,#32610,#32611,#32612,#32613,#32614,#32615,#32616,#32617,#32618,#32619,
#32620,#32621,#32622,#32623,#32624,#32625,#32626,#32627,#32628,#32629,#32630,
#32631,#32632,#32633,#32634,#32635,#32636,#32637,#32638,#32639,#32640,#32641,
#32642,#32643,#32644,#32645,#32646),.UNSPECIFIED.,.F.,.F.,(4,3,3,3,3,3,
3,3,3,3,3,3,3,3,4),(139.539095759119,139.638322148253,140.13703044164,140.635738735027,
141.134447028413,141.6331553218,142.131863615187,142.630571908573,143.12928020196,
143.627988495346,144.126696788733,144.62540508212,145.124113375506,145.622821668893,
145.822281066299),.UNSPECIFIED.);
#889=B_SPLINE_CURVE_WITH_KNOTS('',3,(#32647,#32648,#32649,#32650,#32651,
#32652,#32653,#32654,#32655,#32656,#32657,#32658,#32659,#32660,#32661,#32662,
#32663,#32664,#32665,#32666,#32667,#32668,#32669,#32670,#32671,#32672,#32673,
#32674,#32675,#32676,#32677,#32678,#32679,#32680,#32681,#32682,#32683,#32684,
#32685,#32686),.UNSPECIFIED.,.F.,.F.,(4,3,3,3,3,3,3,3,3,3,3,3,3,4),(-142.079051163592,
-141.6331553218,-141.134447028413,-140.635738735027,-140.13703044164,-139.638322148253,
-139.139613854867,-138.64090556148,-138.142197268094,-137.643488974707,
-137.14478068132,-136.646072387934,-136.147364094547,-135.795865856413),
 .UNSPECIFIED.);
#890=B_SPLINE_CURVE_WITH_KNOTS('',3,(#32691,#32692,#32693,#32694,#32695,
#32696,#32697,#32698,#32699,#32700,#32701,#32702,#32703,#32704,#32705,#32706,
#32707,#32708,#32709,#32710,#32711,#32712,#32713,#32714,#32715,#32716,#32717,
#32718,#32719,#32720,#32721,#32722,#32723,#32724,#32725,#32726,#32727,#32728,
#32729,#32730),.UNSPECIFIED.,.F.,.F.,(4,3,3,3,3,3,3,3,3,3,3,3,3,4),(133.25591045194,
133.653822627614,134.152530921001,134.651239214387,135.149947507774,135.648655801161,
136.147364094547,136.646072387934,137.14478068132,137.643488974707,138.142197268094,
138.64090556148,139.139613854867,139.539095759119),.UNSPECIFIED.);
#891=B_SPLINE_CURVE_WITH_KNOTS('',3,(#32731,#32732,#32733,#32734,#32735,
#32736,#32737,#32738,#32739,#32740,#32741,#32742,#32743,#32744,#32745,#32746,
#32747,#32748,#32749,#32750,#32751,#32752,#32753,#32754,#32755,#32756,#32757,
#32758,#32759,#32760,#32761),.UNSPECIFIED.,.F.,.F.,(4,3,3,3,3,3,3,3,3,3,
4),(-135.795865856413,-135.648655801161,-135.149947507774,-134.651239214387,
-134.152530921001,-133.653822627614,-132.656406040841,-131.658989454068,
-130.661572867294,-129.664156280521,-129.512680549233),.UNSPECIFIED.);
#892=B_SPLINE_CURVE_WITH_KNOTS('',3,(#32766,#32767,#32768,#32769,#32770,
#32771,#32772,#32773,#32774,#32775,#32776,#32777,#32778,#32779,#32780,#32781,
#32782,#32783,#32784,#32785,#32786,#32787),.UNSPECIFIED.,.F.,.F.,(4,3,3,
3,3,3,3,4),(126.97272514476,127.669323106975,128.666739693748,129.664156280521,
130.661572867294,131.658989454068,132.656406040841,133.25591045194),
 .UNSPECIFIED.);
#893=B_SPLINE_CURVE_WITH_KNOTS('',3,(#32788,#32789,#32790,#32791,#32792,
#32793,#32794,#32795,#32796,#32797,#32798,#32799,#32800,#32801,#32802,#32803,
#32804,#32805,#32806,#32807,#32808,#32809),.UNSPECIFIED.,.F.,.F.,(4,3,3,
3,3,3,3,4),(-129.512680549233,-128.666739693748,-127.669323106975,-126.671906520201,
-125.674489933428,-124.677073346655,-123.679656759882,-123.229495242053),
 .UNSPECIFIED.);
#894=B_SPLINE_CURVE_WITH_KNOTS('',3,(#32814,#32815,#32816,#32817,#32818,
#32819,#32820,#32821,#32822,#32823,#32824,#32825,#32826,#32827,#32828,#32829,
#32830,#32831,#32832,#32833,#32834,#32835),.UNSPECIFIED.,.F.,.F.,(4,3,3,
3,3,3,3,4),(120.68953983758,121.684823586335,122.682240173108,123.679656759882,
124.677073346655,125.674489933428,126.671906520201,126.97272514476),
 .UNSPECIFIED.);
#895=B_SPLINE_CURVE_WITH_KNOTS('',3,(#32836,#32837,#32838,#32839,#32840,
#32841,#32842,#32843,#32844,#32845,#32846,#32847,#32848,#32849,#32850,#32851,
#32852,#32853,#32854,#32855,#32856,#32857,#32858,#32859,#32860,#32861,#32862,
#32863,#32864,#32865,#32866),.UNSPECIFIED.,.F.,.F.,(4,3,3,3,3,3,3,3,3,3,
4),(-123.229495242053,-122.682240173108,-121.684823586335,-120.687406999562,
-119.689990412789,-119.191282119402,-118.692573826015,-118.193865532629,
-117.695157239242,-117.196448945856,-116.946309934874),.UNSPECIFIED.);
#896=B_SPLINE_CURVE_WITH_KNOTS('',3,(#32871,#32872,#32873,#32874,#32875,
#32876,#32877,#32878,#32879,#32880,#32881,#32882,#32883,#32884,#32885,#32886,
#32887,#32888,#32889,#32890,#32891,#32892,#32893,#32894,#32895,#32896,#32897,
#32898,#32899,#32900,#32901,#32902,#32903,#32904,#32905,#32906,#32907,#32908,
#32909,#32910),.UNSPECIFIED.,.F.,.F.,(4,3,3,3,3,3,3,3,3,3,3,3,3,4),(114.406354530401,
114.702907478922,115.201615772309,115.700324065696,116.199032359082,116.697740652469,
117.196448945856,117.695157239242,118.193865532629,118.692573826015,119.191282119402,
119.689990412789,120.687406999562,120.68953983758),.UNSPECIFIED.);
#897=B_SPLINE_CURVE_WITH_KNOTS('',3,(#32911,#32912,#32913,#32914,#32915,
#32916,#32917,#32918,#32919,#32920,#32921,#32922,#32923,#32924,#32925,#32926,
#32927,#32928,#32929,#32930,#32931,#32932,#32933,#32934,#32935,#32936,#32937,
#32938,#32939,#32940,#32941,#32942,#32943,#32944,#32945,#32946,#32947,#32948,
#32949,#32950,#32951,#32952,#32953),.UNSPECIFIED.,.F.,.F.,(4,3,3,3,3,3,
3,3,3,3,3,3,3,3,4),(-116.946309934874,-116.697740652469,-116.199032359082,
-115.700324065696,-115.201615772309,-114.702907478922,-114.204199185536,
-113.705490892149,-113.206782598763,-112.708074305376,-112.209366011989,
-111.710657718603,-111.211949425216,-110.71324113183,-110.663124627694),
 .UNSPECIFIED.);
#898=B_SPLINE_CURVE_WITH_KNOTS('',3,(#32958,#32959,#32960,#32961,#32962,
#32963,#32964,#32965,#32966,#32967,#32968,#32969,#32970,#32971,#32972,#32973,
#32974,#32975,#32976,#32977,#32978,#32979,#32980,#32981,#32982,#32983,#32984,
#32985,#32986,#32987,#32988,#32989,#32990,#32991,#32992,#32993,#32994,#32995,
#32996,#32997,#32998,#32999,#33000),.UNSPECIFIED.,.F.,.F.,(4,3,3,3,3,3,
3,3,3,3,3,3,3,3,4),(108.123169223221,108.219699664896,108.718407958283,
109.21711625167,109.715824545056,110.214532838443,110.71324113183,111.211949425216,
111.710657718603,112.209366011989,112.708074305376,113.206782598763,113.705490892149,
114.204199185536,114.406354530401),.UNSPECIFIED.);
#899=B_SPLINE_CURVE_WITH_KNOTS('',3,(#33001,#33002,#33003,#33004,#33005,
#33006,#33007,#33008,#33009,#33010,#33011,#33012,#33013,#33014,#33015,#33016,
#33017,#33018,#33019,#33020,#33021,#33022,#33023,#33024,#33025,#33026,#33027,
#33028,#33029,#33030,#33031,#33032,#33033,#33034,#33035,#33036,#33037,#33038,
#33039,#33040),.UNSPECIFIED.,.F.,.F.,(4,3,3,3,3,3,3,3,3,3,3,3,3,4),(-110.663124627694,
-110.214532838443,-109.715824545056,-109.21711625167,-108.718407958283,
-108.219699664896,-107.72099137151,-107.222283078123,-106.723574784737,
-106.22486649135,-105.726158197963,-105.227449904577,-104.72874161119,-104.379939320515),
 .UNSPECIFIED.);
#900=B_SPLINE_CURVE_WITH_KNOTS('',3,(#33045,#33046,#33047,#33048,#33049,
#33050,#33051,#33052,#33053,#33054,#33055,#33056,#33057,#33058,#33059,#33060,
#33061,#33062,#33063,#33064,#33065,#33066,#33067,#33068,#33069,#33070,#33071,
#33072,#33073,#33074,#33075,#33076,#33077,#33078,#33079,#33080,#33081,#33082,
#33083,#33084),.UNSPECIFIED.,.F.,.F.,(4,3,3,3,3,3,3,3,3,3,3,3,3,4),(101.839983916042,
102.235200144257,102.733908437644,103.23261673103,103.731325024417,104.230033317804,
104.72874161119,105.227449904577,105.726158197963,106.22486649135,106.723574784737,
107.222283078123,107.72099137151,108.123169223221),.UNSPECIFIED.);
#901=B_SPLINE_CURVE_WITH_KNOTS('',3,(#33085,#33086,#33087,#33088,#33089,
#33090,#33091,#33092,#33093,#33094,#33095,#33096,#33097,#33098,#33099,#33100,
#33101,#33102,#33103,#33104,#33105,#33106,#33107,#33108,#33109,#33110,#33111,
#33112,#33113,#33114,#33115,#33116,#33117,#33118,#33119,#33120,#33121,#33122,
#33123,#33124,#33125,#33126,#33127),.UNSPECIFIED.,.F.,.F.,(4,3,3,3,3,3,
3,3,3,3,3,3,3,3,4),(-104.379939320515,-104.230033317803,-103.731325024417,
-103.23261673103,-102.733908437644,-102.235200144257,-101.73649185087,-101.237783557484,
-100.739075264097,-100.24036697071,-99.7416586773239,-99.2429503839373,
-98.7442420905506,-98.245533797164,-98.096754013335),.UNSPECIFIED.);
#902=B_SPLINE_CURVE_WITH_KNOTS('',3,(#33132,#33133,#33134,#33135,#33136,
#33137,#33138,#33139,#33140,#33141,#33142,#33143,#33144,#33145,#33146,#33147,
#33148,#33149,#33150,#33151,#33152,#33153,#33154,#33155,#33156,#33157,#33158,
#33159,#33160,#33161,#33162,#33163,#33164,#33165,#33166,#33167,#33168,#33169,
#33170,#33171,#33172,#33173,#33174),.UNSPECIFIED.,.F.,.F.,(4,3,3,3,3,3,
3,3,3,3,3,3,3,3,4),(95.556798608862,95.751992330231,96.2507006236176,96.7494089170042,
97.2481172103908,97.7468255037774,98.2455337971641,98.7442420905507,99.2429503839373,
99.7416586773239,100.240366970711,100.739075264097,101.237783557484,101.73649185087,
101.839983916042),.UNSPECIFIED.);
#903=B_SPLINE_CURVE_WITH_KNOTS('',3,(#33175,#33176,#33177,#33178,#33179,
#33180,#33181,#33182,#33183,#33184,#33185,#33186,#33187,#33188,#33189,#33190,
#33191,#33192,#33193,#33194,#33195,#33196,#33197,#33198,#33199,#33200,#33201,
#33202,#33203,#33204,#33205,#33206,#33207,#33208,#33209,#33210,#33211,#33212,
#33213,#33214),.UNSPECIFIED.,.F.,.F.,(4,3,3,3,3,3,3,3,3,3,3,3,3,4),(-98.096754013335,
-97.7468255037774,-97.2481172103908,-96.7494089170042,-96.2507006236176,
-95.7519923302309,-95.2532840368443,-94.7545757434577,-94.2558674500711,
-93.7571591566845,-93.2584508632978,-92.7597425699112,-92.2610342765246,
-91.8135687061554),.UNSPECIFIED.);
#904=B_SPLINE_CURVE_WITH_KNOTS('',3,(#33219,#33220,#33221,#33222,#33223,
#33224,#33225,#33226,#33227,#33228,#33229,#33230,#33231,#33232,#33233,#33234,
#33235,#33236,#33237,#33238,#33239,#33240,#33241,#33242,#33243,#33244,#33245,
#33246,#33247,#33248,#33249,#33250,#33251,#33252,#33253,#33254,#33255,#33256,
#33257,#33258),.UNSPECIFIED.,.F.,.F.,(4,3,3,3,3,3,3,3,3,3,3,3,3,4),(89.2736133016824,
89.7674928095915,90.2662011029781,90.7649093963648,91.2636176897514,91.762325983138,
92.2610342765246,92.7597425699113,93.2584508632979,93.7571591566845,94.2558674500711,
94.7545757434577,95.2532840368443,95.556798608862),.UNSPECIFIED.);
#905=B_SPLINE_CURVE_WITH_KNOTS('',3,(#33259,#33260,#33261,#33262,#33263,
#33264,#33265,#33266,#33267,#33268,#33269,#33270,#33271,#33272,#33273,#33274,
#33275,#33276,#33277,#33278,#33279,#33280,#33281,#33282,#33283,#33284,#33285,
#33286,#33287,#33288,#33289,#33290,#33291,#33292,#33293,#33294,#33295,#33296,
#33297,#33298,#33299,#33300,#33301),.UNSPECIFIED.,.F.,.F.,(4,3,3,3,3,3,
3,3,3,3,3,3,3,3,4),(-91.8135687061554,-91.762325983138,-91.2636176897513,
-90.7649093963647,-90.2662011029781,-89.7674928095915,-89.2687845162049,
-88.7700762228182,-88.2713679294316,-87.772659636045,-87.2739513426584,
-86.7752430492718,-86.2765347558852,-85.7778264624986,-85.5303833989758),
 .UNSPECIFIED.);
#906=B_SPLINE_CURVE_WITH_KNOTS('',3,(#33306,#33307,#33308,#33309,#33310,
#33311,#33312,#33313,#33314,#33315,#33316,#33317,#33318,#33319,#33320,#33321,
#33322,#33323,#33324,#33325,#33326,#33327,#33328,#33329,#33330,#33331,#33332,
#33333,#33334,#33335,#33336,#33337,#33338,#33339,#33340,#33341,#33342,#33343,
#33344,#33345,#33346,#33347,#33348),.UNSPECIFIED.,.F.,.F.,(4,3,3,3,3,3,
3,3,3,3,3,3,3,3,4),(82.9904279945028,83.2842849955655,83.7829932889521,
84.2817015823387,84.7804098757253,85.279118169112,85.7778264624986,86.2765347558852,
86.7752430492718,87.2739513426584,87.772659636045,88.2713679294317,88.7700762228183,
89.2687845162049,89.2736133016824),.UNSPECIFIED.);
#907=B_SPLINE_CURVE_WITH_KNOTS('',3,(#33349,#33350,#33351,#33352,#33353,
#33354,#33355,#33356,#33357,#33358,#33359,#33360,#33361,#33362,#33363,#33364,
#33365,#33366,#33367,#33368,#33369,#33370,#33371,#33372,#33373,#33374,#33375,
#33376,#33377,#33378,#33379,#33380,#33381,#33382,#33383,#33384,#33385,#33386,
#33387,#33388,#33389,#33390,#33391),.UNSPECIFIED.,.F.,.F.,(4,3,3,3,3,3,
3,3,3,3,3,3,3,3,4),(-85.5303833989758,-85.2791181691119,-84.7804098757253,
-84.2817015823387,-83.7829932889521,-83.2842849955654,-82.7855767021788,
-82.2868684087922,-81.7881601154056,-81.289451822019,-80.7907435286323,
-80.2920352352457,-79.7933269418591,-79.2946186484725,-79.2471980917962),
 .UNSPECIFIED.);
#908=B_SPLINE_CURVE_WITH_KNOTS('',3,(#33396,#33397,#33398,#33399,#33400,
#33401,#33402,#33403,#33404,#33405,#33406,#33407,#33408,#33409,#33410,#33411,
#33412,#33413,#33414,#33415,#33416,#33417,#33418,#33419,#33420,#33421,#33422,
#33423,#33424,#33425,#33426,#33427,#33428,#33429,#33430,#33431,#33432,#33433,
#33434,#33435,#33436,#33437,#33438),.UNSPECIFIED.,.F.,.F.,(4,3,3,3,3,3,
3,3,3,3,3,3,3,3,4),(76.7072426873232,76.8010771815394,77.299785474926,77.7984937683127,
78.2972020616993,78.7959103550859,79.2946186484725,79.7933269418591,80.2920352352457,
80.7907435286324,81.289451822019,81.7881601154056,82.2868684087922,82.7855767021789,
82.9904279945028),.UNSPECIFIED.);
#909=B_SPLINE_CURVE_WITH_KNOTS('',3,(#33439,#33440,#33441,#33442,#33443,
#33444,#33445,#33446,#33447,#33448,#33449,#33450,#33451,#33452,#33453,#33454,
#33455,#33456,#33457,#33458,#33459,#33460,#33461,#33462,#33463,#33464,#33465,
#33466,#33467,#33468,#33469,#33470,#33471,#33472,#33473,#33474,#33475,#33476,
#33477,#33478),.UNSPECIFIED.,.F.,.F.,(4,3,3,3,3,3,3,3,3,3,3,3,3,4),(-79.2471980917962,
-78.7959103550859,-78.2972020616993,-77.7984937683126,-77.299785474926,
-76.8010771815394,-76.3023688881528,-75.8036605947662,-75.3049523013795,
-74.8062440079929,-74.3075357146063,-73.8088274212197,-73.3101191278331,
-72.9640127846166),.UNSPECIFIED.);
#910=B_SPLINE_CURVE_WITH_KNOTS('',3,(#33483,#33484,#33485,#33486,#33487,
#33488,#33489,#33490,#33491,#33492,#33493,#33494,#33495,#33496,#33497,#33498,
#33499,#33500,#33501,#33502,#33503,#33504,#33505,#33506,#33507,#33508,#33509,
#33510,#33511,#33512,#33513,#33514,#33515,#33516,#33517,#33518,#33519,#33520,
#33521,#33522),.UNSPECIFIED.,.F.,.F.,(4,3,3,3,3,3,3,3,3,3,3,3,3,4),(70.4240573801436,
70.8165776609,71.3152859542866,71.8139942476732,72.3127025410598,72.8114108344465,
73.3101191278331,73.8088274212197,74.3075357146063,74.8062440079929,75.3049523013796,
75.8036605947662,76.3023688881528,76.7072426873232),.UNSPECIFIED.);
#911=B_SPLINE_CURVE_WITH_KNOTS('',3,(#33523,#33524,#33525,#33526,#33527,
#33528,#33529,#33530,#33531,#33532,#33533,#33534,#33535,#33536,#33537,#33538,
#33539,#33540,#33541,#33542,#33543,#33544,#33545,#33546,#33547,#33548,#33549,
#33550,#33551,#33552,#33553,#33554,#33555,#33556,#33557,#33558,#33559,#33560,
#33561,#33562,#33563,#33564,#33565),.UNSPECIFIED.,.F.,.F.,(4,3,3,3,3,3,
3,3,3,3,3,3,3,3,4),(-72.9640127846166,-72.8114108344464,-72.3127025410598,
-71.8139942476732,-71.3152859542866,-70.8165776609,-70.3178693675133,-69.8191610741267,
-69.3204527807401,-68.8217444873535,-68.3230361939669,-67.8243279005802,
-67.3256196071936,-66.826911313807,-66.680827477437),.UNSPECIFIED.);
#912=B_SPLINE_CURVE_WITH_KNOTS('',3,(#33570,#33571,#33572,#33573,#33574,
#33575,#33576,#33577,#33578,#33579,#33580,#33581,#33582,#33583,#33584,#33585,
#33586,#33587,#33588,#33589,#33590,#33591,#33592,#33593,#33594,#33595,#33596,
#33597,#33598,#33599,#33600,#33601,#33602,#33603,#33604,#33605,#33606,#33607,
#33608,#33609,#33610,#33611,#33612),.UNSPECIFIED.,.F.,.F.,(4,3,3,3,3,3,
3,3,3,3,3,3,3,3,4),(64.140872072964,64.3333698468739,64.8320781402605,65.3307864336472,
65.8294947270338,66.3282030204204,66.826911313807,67.3256196071937,67.8243279005803,
68.3230361939669,68.8217444873535,69.3204527807401,69.8191610741268,70.3178693675134,
70.4240573801436),.UNSPECIFIED.);
#913=B_SPLINE_CURVE_WITH_KNOTS('',3,(#33613,#33614,#33615,#33616,#33617,
#33618,#33619,#33620,#33621,#33622,#33623,#33624,#33625,#33626,#33627,#33628,
#33629,#33630,#33631,#33632,#33633,#33634,#33635,#33636,#33637,#33638,#33639,
#33640,#33641,#33642,#33643,#33644,#33645,#33646,#33647,#33648,#33649,#33650,
#33651,#33652),.UNSPECIFIED.,.F.,.F.,(4,3,3,3,3,3,3,3,3,3,3,3,3,4),(-66.680827477437,
-66.3282030204204,-65.8294947270337,-65.3307864336471,-64.8320781402605,
-64.3333698468739,-63.8346615534873,-63.3359532601007,-62.837244966714,
-62.3385366733274,-61.8398283799408,-61.3411200865542,-60.8424117931676,
-60.3976421702575),.UNSPECIFIED.);
#914=B_SPLINE_CURVE_WITH_KNOTS('',3,(#33657,#33658,#33659,#33660,#33661,
#33662,#33663,#33664,#33665,#33666,#33667,#33668,#33669,#33670,#33671,#33672,
#33673,#33674,#33675,#33676,#33677,#33678,#33679,#33680,#33681,#33682,#33683,
#33684,#33685,#33686,#33687,#33688,#33689,#33690,#33691,#33692,#33693,#33694,
#33695,#33696),.UNSPECIFIED.,.F.,.F.,(4,3,3,3,3,3,3,3,3,3,3,3,3,4),(57.8576867657844,
58.3488703262345,58.8475786196211,59.3462869130077,59.8449952063944,60.343703499781,
60.8424117931676,61.3411200865542,61.8398283799408,62.3385366733274,62.8372449667141,
63.3359532601007,63.8346615534873,64.140872072964),.UNSPECIFIED.);
#915=B_SPLINE_CURVE_WITH_KNOTS('',3,(#33697,#33698,#33699,#33700,#33701,
#33702,#33703,#33704,#33705,#33706,#33707,#33708,#33709,#33710,#33711,#33712,
#33713,#33714,#33715,#33716,#33717,#33718,#33719,#33720,#33721,#33722,#33723,
#33724,#33725,#33726,#33727,#33728,#33729,#33730,#33731,#33732,#33733,#33734,
#33735,#33736,#33737,#33738,#33739),.UNSPECIFIED.,.F.,.F.,(4,3,3,3,3,3,
3,3,3,3,3,3,3,3,4),(-60.3976421702575,-60.3437034997809,-59.8449952063943,
-59.3462869130077,-58.8475786196211,-58.3488703262345,-57.8501620328479,
-57.3514537394612,-56.8527454460746,-56.354037152688,-55.8553288593014,
-55.3566205659148,-54.8579122725281,-54.3592039791415,-54.1144568630779),
 .UNSPECIFIED.);
#916=B_SPLINE_CURVE_WITH_KNOTS('',3,(#33744,#33745,#33746,#33747,#33748,
#33749,#33750,#33751,#33752,#33753,#33754,#33755,#33756,#33757,#33758,#33759,
#33760,#33761,#33762,#33763,#33764,#33765,#33766,#33767,#33768,#33769,#33770,
#33771,#33772,#33773,#33774,#33775,#33776,#33777,#33778,#33779,#33780,#33781,
#33782,#33783,#33784,#33785,#33786),.UNSPECIFIED.,.F.,.F.,(4,3,3,3,3,3,
3,3,3,3,3,3,3,3,4),(51.5745014586048,51.8656625122084,52.3643708055951,
52.8630790989817,53.3617873923683,53.8604956857549,54.3592039791415,54.8579122725282,
55.3566205659148,55.8553288593014,56.354037152688,56.8527454460746,57.3514537394612,
57.8501620328479,57.8576867657844),.UNSPECIFIED.);
#917=B_SPLINE_CURVE_WITH_KNOTS('',3,(#33787,#33788,#33789,#33790,#33791,
#33792,#33793,#33794,#33795,#33796,#33797,#33798,#33799,#33800,#33801,#33802,
#33803,#33804,#33805,#33806,#33807,#33808,#33809,#33810,#33811,#33812,#33813,
#33814,#33815,#33816,#33817,#33818,#33819,#33820,#33821,#33822,#33823,#33824,
#33825,#33826,#33827,#33828,#33829),.UNSPECIFIED.,.F.,.F.,(4,3,3,3,3,3,
3,3,3,3,3,3,3,3,4),(-54.1144568630779,-53.8604956857549,-53.3617873923683,
-52.8630790989817,-52.3643708055951,-51.8656625122084,-51.3669542188218,
-50.8682459254352,-50.3695376320486,-49.8708293386619,-49.3721210452753,
-48.8734127518887,-48.3747044585021,-47.8759961651155,-47.8312715558983),
 .UNSPECIFIED.);
#918=B_SPLINE_CURVE_WITH_KNOTS('',3,(#33834,#33835,#33836,#33837,#33838,
#33839,#33840,#33841,#33842,#33843,#33844,#33845,#33846,#33847,#33848,#33849,
#33850,#33851,#33852,#33853,#33854,#33855,#33856,#33857,#33858,#33859,#33860,
#33861,#33862,#33863,#33864,#33865,#33866,#33867,#33868,#33869,#33870,#33871,
#33872,#33873,#33874,#33875,#33876),.UNSPECIFIED.,.F.,.F.,(4,3,3,3,3,3,
3,3,3,3,3,3,3,3,4),(45.2913161514252,45.3824546981824,45.881162991569,46.3798712849556,
46.8785795783422,47.3772878717289,47.8759961651155,48.3747044585021,48.8734127518887,
49.3721210452753,49.870829338662,50.3695376320486,50.8682459254352,51.3669542188218,
51.5745014586048),.UNSPECIFIED.);
#919=B_SPLINE_CURVE_WITH_KNOTS('',3,(#33877,#33878,#33879,#33880,#33881,
#33882,#33883,#33884,#33885,#33886,#33887,#33888,#33889,#33890,#33891,#33892,
#33893,#33894,#33895,#33896,#33897,#33898,#33899,#33900,#33901,#33902,#33903,
#33904,#33905,#33906,#33907,#33908,#33909,#33910,#33911,#33912,#33913,#33914,
#33915,#33916),.UNSPECIFIED.,.F.,.F.,(4,3,3,3,3,3,3,3,3,3,3,3,3,4),(-47.8312715558983,
-47.3772878717289,-46.8785795783422,-46.3798712849556,-45.881162991569,
-45.3824546981824,-44.8837464047958,-44.3850381114091,-43.8863298180225,
-43.3876215246359,-42.8889132312493,-42.3902049378627,-41.891496644476,
-41.5480862487187),.UNSPECIFIED.);
#920=B_SPLINE_CURVE_WITH_KNOTS('',3,(#33921,#33922,#33923,#33924,#33925,
#33926,#33927,#33928,#33929,#33930,#33931,#33932,#33933,#33934,#33935,#33936,
#33937,#33938,#33939,#33940,#33941,#33942,#33943,#33944,#33945,#33946,#33947,
#33948,#33949,#33950,#33951,#33952,#33953,#33954,#33955,#33956,#33957,#33958,
#33959,#33960),.UNSPECIFIED.,.F.,.F.,(4,3,3,3,3,3,3,3,3,3,3,3,3,4),(39.0081308442456,
39.3979551775429,39.8966634709296,40.3953717643162,40.8940800577028,41.3927883510894,
41.891496644476,42.3902049378627,42.8889132312493,43.3876215246359,43.8863298180225,
44.3850381114091,44.8837464047958,45.2913161514252),.UNSPECIFIED.);
#921=B_SPLINE_CURVE_WITH_KNOTS('',3,(#33961,#33962,#33963,#33964,#33965,
#33966,#33967,#33968,#33969,#33970,#33971,#33972,#33973,#33974,#33975,#33976,
#33977,#33978,#33979,#33980,#33981,#33982,#33983,#33984,#33985,#33986,#33987,
#33988,#33989,#33990,#33991,#33992,#33993,#33994,#33995,#33996,#33997,#33998,
#33999,#34000,#34001,#34002,#34003),.UNSPECIFIED.,.F.,.F.,(4,3,3,3,3,3,
3,3,3,3,3,3,3,3,4),(-41.5480862487187,-41.3927883510894,-40.8940800577028,
-40.3953717643162,-39.8966634709296,-39.3979551775429,-38.8992468841563,
-38.4005385907697,-37.9018302973831,-37.4031220039965,-36.9044137106098,
-36.4057054172232,-35.9069971238366,-35.40828883045,-35.2649009415391),
 .UNSPECIFIED.);
#922=B_SPLINE_CURVE_WITH_KNOTS('',3,(#34008,#34009,#34010,#34011,#34012,
#34013,#34014,#34015,#34016,#34017,#34018,#34019,#34020,#34021,#34022,#34023,
#34024,#34025,#34026,#34027,#34028,#34029,#34030,#34031,#34032,#34033,#34034,
#34035,#34036,#34037,#34038,#34039,#34040,#34041,#34042,#34043,#34044,#34045,
#34046,#34047,#34048,#34049,#34050),.UNSPECIFIED.,.F.,.F.,(4,3,3,3,3,3,
3,3,3,3,3,3,3,3,4),(32.7249455370661,32.9147473635169,33.4134556569035,
33.9121639502901,34.4108722436767,34.9095805370634,35.40828883045,35.9069971238366,
36.4057054172232,36.9044137106099,37.4031220039965,37.9018302973831,38.4005385907697,
38.8992468841563,39.0081308442456),.UNSPECIFIED.);
#923=B_SPLINE_CURVE_WITH_KNOTS('',3,(#34051,#34052,#34053,#34054,#34055,
#34056,#34057,#34058,#34059,#34060,#34061,#34062,#34063,#34064,#34065,#34066,
#34067,#34068,#34069,#34070,#34071,#34072,#34073,#34074,#34075,#34076,#34077,
#34078,#34079,#34080,#34081,#34082,#34083,#34084,#34085,#34086,#34087,#34088,
#34089,#34090),.UNSPECIFIED.,.F.,.F.,(4,3,3,3,3,3,3,3,3,3,3,3,3,4),(-35.2649009415391,
-34.9095805370634,-34.4108722436767,-33.9121639502901,-33.4134556569035,
-32.9147473635169,-32.4160390701303,-31.9173307767436,-31.418622483357,
-30.9199141899704,-30.4212058965838,-29.9224976031972,-29.4237893098105,
-28.9817156343595),.UNSPECIFIED.);
#924=B_SPLINE_CURVE_WITH_KNOTS('',3,(#34095,#34096,#34097,#34098,#34099,
#34100,#34101,#34102,#34103,#34104,#34105,#34106,#34107,#34108,#34109,#34110,
#34111,#34112,#34113,#34114,#34115,#34116,#34117,#34118,#34119,#34120,#34121,
#34122,#34123,#34124,#34125,#34126,#34127,#34128,#34129,#34130,#34131,#34132,
#34133,#34134),.UNSPECIFIED.,.F.,.F.,(4,3,3,3,3,3,3,3,3,3,3,3,3,4),(26.4417602298865,
26.9302478428775,27.4289561362641,27.9276644296507,28.4263727230373,28.9250810164239,
29.4237893098106,29.9224976031972,30.4212058965838,30.9199141899704,31.418622483357,
31.9173307767437,32.4160390701303,32.7249455370661),.UNSPECIFIED.);
#925=B_SPLINE_CURVE_WITH_KNOTS('',3,(#34135,#34136,#34137,#34138,#34139,
#34140,#34141,#34142,#34143,#34144,#34145,#34146,#34147,#34148,#34149,#34150,
#34151,#34152,#34153,#34154,#34155,#34156,#34157,#34158,#34159,#34160,#34161,
#34162,#34163,#34164,#34165,#34166,#34167,#34168,#34169,#34170,#34171,#34172,
#34173,#34174,#34175,#34176,#34177),.UNSPECIFIED.,.F.,.F.,(4,3,3,3,3,3,
3,3,3,3,3,3,3,3,4),(-28.9817156343595,-28.9250810164239,-28.4263727230373,
-27.9276644296507,-27.4289561362641,-26.9302478428774,-26.4315395494908,
-25.9328312561042,-25.4341229627176,-24.935414669331,-24.4367063759443,
-23.9379980825577,-23.4392897891711,-22.9405814957845,-22.6985303271799),
 .UNSPECIFIED.);
#926=B_SPLINE_CURVE_WITH_KNOTS('',3,(#34182,#34183,#34184,#34185,#34186,
#34187,#34188,#34189,#34190,#34191,#34192,#34193,#34194,#34195,#34196,#34197,
#34198,#34199,#34200,#34201,#34202,#34203,#34204,#34205,#34206,#34207,#34208,
#34209,#34210,#34211,#34212,#34213,#34214,#34215,#34216,#34217,#34218,#34219,
#34220,#34221,#34222,#34223,#34224),.UNSPECIFIED.,.F.,.F.,(4,3,3,3,3,3,
3,3,3,3,3,3,3,3,4),(20.1585749227069,20.4470400288514,20.945748322238,21.4444566156246,
21.9431649090113,22.4418732023979,22.9405814957845,23.4392897891711,23.9379980825577,
24.4367063759444,24.935414669331,25.4341229627176,25.9328312561042,26.4315395494908,
26.4417602298865),.UNSPECIFIED.);
#927=B_SPLINE_CURVE_WITH_KNOTS('',3,(#34225,#34226,#34227,#34228,#34229,
#34230,#34231,#34232,#34233,#34234,#34235,#34236,#34237,#34238,#34239,#34240,
#34241,#34242,#34243,#34244,#34245,#34246,#34247,#34248,#34249,#34250,#34251,
#34252,#34253,#34254,#34255,#34256,#34257,#34258,#34259,#34260,#34261,#34262,
#34263,#34264,#34265,#34266,#34267),.UNSPECIFIED.,.F.,.F.,(4,3,3,3,3,3,
3,3,3,3,3,3,3,3,4),(-22.6985303271799,-22.4418732023979,-21.9431649090112,
-21.4444566156246,-20.945748322238,-20.4470400288514,-19.9483317354648,
-19.4496234420782,-18.9509151486915,-18.4522068553049,-17.9534985619183,
-17.4547902685317,-16.9560819751451,-16.4573736817584,-16.4153450200003),
 .UNSPECIFIED.);
#928=B_SPLINE_CURVE_WITH_KNOTS('',3,(#34272,#34273,#34274,#34275,#34276,
#34277,#34278,#34279,#34280,#34281,#34282,#34283,#34284,#34285,#34286,#34287,
#34288,#34289,#34290,#34291,#34292,#34293,#34294,#34295,#34296,#34297,#34298,
#34299,#34300,#34301,#34302,#34303,#34304,#34305,#34306,#34307,#34308,#34309,
#34310,#34311,#34312,#34313,#34314),.UNSPECIFIED.,.F.,.F.,(4,3,3,3,3,3,
3,3,3,3,3,3,3,3,4),(13.8753896155273,13.9638322148253,14.462540508212,14.9612488015986,
15.4599570949852,15.9586653883718,16.4573736817584,16.9560819751451,17.4547902685317,
17.9534985619183,18.4522068553049,18.9509151486915,19.4496234420782,19.9483317354648,
20.1585749227069),.UNSPECIFIED.);
#929=B_SPLINE_CURVE_WITH_KNOTS('',3,(#34315,#34316,#34317,#34318,#34319,
#34320,#34321,#34322,#34323,#34324,#34325,#34326,#34327,#34328,#34329,#34330,
#34331,#34332,#34333,#34334,#34335,#34336,#34337,#34338,#34339,#34340,#34341,
#34342,#34343,#34344,#34345,#34346,#34347,#34348,#34349,#34350,#34351,#34352,
#34353,#34354),.UNSPECIFIED.,.F.,.F.,(4,3,3,3,3,3,3,3,3,3,3,3,3,4),(-16.4153450200003,
-15.9586653883718,-15.4599570949852,-14.9612488015986,-14.462540508212,
-13.9638322148253,-13.4651239214387,-12.9664156280521,-12.4677073346655,
-11.9689990412789,-11.4702907478922,-10.9715824545056,-10.472874161119,
-10.1321597128207),.UNSPECIFIED.);
#930=B_SPLINE_CURVE_WITH_KNOTS('',3,(#34360,#34361,#34362,#34363,#34364,
#34365,#34366,#34367,#34368,#34369,#34370,#34371,#34372,#34373,#34374,#34375,
#34376,#34377,#34378,#34379,#34380,#34381,#34382,#34383,#34384),
 .UNSPECIFIED.,.F.,.F.,(4,3,3,3,3,3,3,3,4),(-3.84897440564115,-3.49095805370634,
-2.99224976031972,-2.4935414669331,-1.99483317354648,-1.49612488015986,
-0.997416586773239,-0.49870829338662,0.),.UNSPECIFIED.);
#931=B_SPLINE_CURVE_WITH_KNOTS('',3,(#34387,#34388,#34389,#34390,#34391,
#34392,#34393,#34394,#34395,#34396,#34397,#34398,#34399,#34400,#34401,#34402,
#34403,#34404,#34405,#34406,#34407,#34408,#34409,#34410,#34411,#34412,#34413,
#34414,#34415,#34416,#34417,#34418,#34419,#34420,#34421,#34422,#34423),
 .UNSPECIFIED.,.F.,.F.,(4,3,3,3,3,3,3,3,3,3,3,3,4),(2.01640075321917,2.4935414669331,
2.99224976031972,3.49095805370634,3.98966634709296,4.48837464047958,4.9870829338662,
5.48579122725282,5.98449952063944,6.48320781402605,6.98191610741268,7.48062440079929,
7.59220430834772),.UNSPECIFIED.);
#932=B_SPLINE_CURVE_WITH_KNOTS('',3,(#34429,#34430,#34431,#34432,#34433,
#34434,#34435,#34436,#34437,#34438,#34439,#34440),.UNSPECIFIED.,.F.,.F.,
(4,1,1,1,1,1,1,1,1,4),(260.752190247953,261.213135555618,261.711843849004,
262.210552142391,262.709260435778,263.207968729164,263.706677022551,264.205385315938,
264.704093609324,265.202801902711),.UNSPECIFIED.);
#933=B_SPLINE_CURVE_WITH_KNOTS('',3,(#34443,#34444,#34445,#34446,#34447,
#34448,#34449,#34450,#34451,#34452,#34453,#34454,#34455,#34456),
 .UNSPECIFIED.,.F.,.F.,(4,1,1,1,1,1,1,1,1,1,1,4),(260.752190247953,260.760841199772,
261.259549493158,261.758257786545,262.256966079931,262.755674373318,263.254382666705,
263.753090960091,264.251799253478,264.750507546865,265.249215840251,265.726356553965),
 .UNSPECIFIED.);
#934=B_SPLINE_CURVE_WITH_KNOTS('',3,(#34461,#34462,#34463,#34464,#34465,
#34466,#34467,#34468,#34469,#34470,#34471,#34472,#34473,#34474,#34475,#34476,
#34477),.UNSPECIFIED.,.F.,.F.,(4,1,1,1,1,1,1,1,1,1,1,1,1,1,4),(254.469004940773,
254.729927741592,255.228636034978,255.727344328365,256.226052621752,256.724760915138,
257.223469208525,257.722177501912,258.220885795298,258.719594088685,259.218302382071,
259.717010675458,260.215718968845,260.714427262231,260.752190247953),
 .UNSPECIFIED.);
#935=B_SPLINE_CURVE_WITH_KNOTS('',3,(#34478,#34479,#34480,#34481,#34482,
#34483,#34484,#34485,#34486,#34487,#34488,#34489,#34490,#34491,#34492,#34493),
 .UNSPECIFIED.,.F.,.F.,(4,1,1,1,1,1,1,1,1,1,1,1,1,4),(254.469004940773,
254.776341679132,255.275049972519,255.773758265905,256.272466559292,256.771174852679,
257.269883146065,257.768591439452,258.267299732838,258.766008026225,259.264716319612,
259.763424612998,260.262132906385,260.752190247953),.UNSPECIFIED.);
#936=B_SPLINE_CURVE_WITH_KNOTS('',3,(#34498,#34499,#34500,#34501,#34502,
#34503,#34504,#34505,#34506,#34507,#34508,#34509,#34510,#34511,#34512,#34513,
#34514),.UNSPECIFIED.,.F.,.F.,(4,1,1,1,1,1,1,1,1,1,1,1,1,1,4),(248.185819633594,
248.246719927566,248.745428220952,249.244136514339,249.742844807726,250.241553101112,
250.740261394499,251.238969687886,251.737677981272,252.236386274659,252.735094568045,
253.233802861432,253.732511154819,254.231219448205,254.469004940773),
 .UNSPECIFIED.);
#937=B_SPLINE_CURVE_WITH_KNOTS('',3,(#34515,#34516,#34517,#34518,#34519,
#34520,#34521,#34522,#34523,#34524,#34525,#34526,#34527,#34528,#34529,#34530,
#34531),.UNSPECIFIED.,.F.,.F.,(4,1,1,1,1,1,1,1,1,1,1,1,1,1,4),(248.185819633594,
248.293133865106,248.791842158493,249.290550451879,249.789258745266,250.287967038653,
250.786675332039,251.285383625426,251.784091918812,252.282800212199,252.781508505586,
253.280216798972,253.778925092359,254.277633385745,254.469004940773),
 .UNSPECIFIED.);
#938=B_SPLINE_CURVE_WITH_KNOTS('',3,(#34536,#34537,#34538,#34539,#34540,
#34541,#34542,#34543,#34544,#34545,#34546,#34547,#34548,#34549,#34550,#34551),
 .UNSPECIFIED.,.F.,.F.,(4,1,1,1,1,1,1,1,1,1,1,1,1,4),(241.902634326414,
242.262220406926,242.760928700313,243.2596369937,243.758345287086,244.257053580473,
244.755761873859,245.254470167246,245.753178460633,246.251886754019,246.750595047406,
247.249303340793,247.748011634179,248.185819633594),.UNSPECIFIED.);
#939=B_SPLINE_CURVE_WITH_KNOTS('',3,(#34552,#34553,#34554,#34555,#34556,
#34557,#34558,#34559,#34560,#34561,#34562,#34563,#34564,#34565,#34566,#34567),
 .UNSPECIFIED.,.F.,.F.,(4,1,1,1,1,1,1,1,1,1,1,1,1,4),(241.902634326414,
242.308634344467,242.807342637853,243.30605093124,243.804759224626,244.303467518013,
244.8021758114,245.300884104786,245.799592398173,246.29830069156,246.797008984946,
247.295717278333,247.794425571719,248.185819633594),.UNSPECIFIED.);
#940=B_SPLINE_CURVE_WITH_KNOTS('',3,(#34572,#34573,#34574,#34575,#34576,
#34577,#34578,#34579,#34580,#34581,#34582,#34583,#34584,#34585,#34586,#34587,
#34588),.UNSPECIFIED.,.F.,.F.,(4,1,1,1,1,1,1,1,1,1,1,1,1,1,4),(235.619449019235,
235.7790125929,236.277720886287,236.776429179674,237.27513747306,237.773845766447,
238.272554059833,238.77126235322,239.269970646607,239.768678939993,240.26738723338,
240.766095526767,241.264803820153,241.76351211354,241.902634326414),
 .UNSPECIFIED.);
#941=B_SPLINE_CURVE_WITH_KNOTS('',3,(#34589,#34590,#34591,#34592,#34593,
#34594,#34595,#34596,#34597,#34598,#34599,#34600,#34601,#34602,#34603,#34604,
#34605),.UNSPECIFIED.,.F.,.F.,(4,1,1,1,1,1,1,1,1,1,1,1,1,1,4),(235.619449019235,
235.825426530441,236.324134823827,236.822843117214,237.3215514106,237.820259703987,
238.318967997374,238.81767629076,239.316384584147,239.815092877534,240.31380117092,
240.812509464307,241.311217757693,241.80992605108,241.902634326414),
 .UNSPECIFIED.);
#942=B_SPLINE_CURVE_WITH_KNOTS('',3,(#34610,#34611,#34612,#34613,#34614,
#34615,#34616,#34617,#34618,#34619,#34620,#34621,#34622,#34623,#34624,#34625),
 .UNSPECIFIED.,.F.,.F.,(4,1,1,1,1,1,1,1,1,1,1,1,1,4),(229.336263712055,
229.794513072261,230.293221365647,230.791929659034,231.290637952421,231.789346245807,
232.288054539194,232.786762832581,233.285471125967,233.784179419354,234.28288771274,
234.781596006127,235.280304299514,235.619449019235),.UNSPECIFIED.);
#943=B_SPLINE_CURVE_WITH_KNOTS('',3,(#34626,#34627,#34628,#34629,#34630,
#34631,#34632,#34633,#34634,#34635,#34636,#34637,#34638,#34639,#34640,#34641,
#34642),.UNSPECIFIED.,.F.,.F.,(4,1,1,1,1,1,1,1,1,1,1,1,1,1,4),(229.336263712055,
229.342218716414,229.840927009801,230.339635303188,230.838343596574,231.337051889961,
231.835760183348,232.334468476734,232.833176770121,233.331885063507,233.830593356894,
234.329301650281,234.828009943667,235.326718237054,235.619449019235),
 .UNSPECIFIED.);
#944=B_SPLINE_CURVE_WITH_KNOTS('',3,(#34647,#34648,#34649,#34650,#34651,
#34652,#34653,#34654,#34655,#34656,#34657,#34658,#34659,#34660,#34661,#34662,
#34663),.UNSPECIFIED.,.F.,.F.,(4,1,1,1,1,1,1,1,1,1,1,1,1,1,4),(223.053078404875,
223.311305258235,223.810013551621,224.308721845008,224.807430138395,225.306138431781,
225.804846725168,226.303555018555,226.802263311941,227.300971605328,227.799679898714,
228.298388192101,228.797096485488,229.295804778874,229.336263712055),
 .UNSPECIFIED.);
#945=B_SPLINE_CURVE_WITH_KNOTS('',3,(#34664,#34665,#34666,#34667,#34668,
#34669,#34670,#34671,#34672,#34673,#34674,#34675,#34676,#34677,#34678,#34679),
 .UNSPECIFIED.,.F.,.F.,(4,1,1,1,1,1,1,1,1,1,1,1,1,4),(223.053078404875,
223.357719195775,223.856427489162,224.355135782548,224.853844075935,225.352552369322,
225.851260662708,226.349968956095,226.848677249481,227.347385542868,227.846093836255,
228.344802129641,228.843510423028,229.336263712055),.UNSPECIFIED.);
#946=B_SPLINE_CURVE_WITH_KNOTS('',3,(#34684,#34685,#34686,#34687,#34688,
#34689,#34690,#34691,#34692,#34693,#34694,#34695,#34696,#34697,#34698,#34699,
#34700),.UNSPECIFIED.,.F.,.F.,(4,1,1,1,1,1,1,1,1,1,1,1,1,1,4),(216.769893097696,
216.828097444209,217.326805737595,217.825514030982,218.324222324369,218.822930617755,
219.321638911142,219.820347204529,220.319055497915,220.817763791302,221.316472084688,
221.815180378075,222.313888671462,222.812596964848,223.053078404875),
 .UNSPECIFIED.);
#947=B_SPLINE_CURVE_WITH_KNOTS('',3,(#34701,#34702,#34703,#34704,#34705,
#34706,#34707,#34708,#34709,#34710,#34711,#34712,#34713,#34714,#34715,#34716,
#34717),.UNSPECIFIED.,.F.,.F.,(4,1,1,1,1,1,1,1,1,1,1,1,1,1,4),(216.769893097696,
216.874511381749,217.373219675136,217.871927968522,218.370636261909,218.869344555295,
219.368052848682,219.866761142069,220.365469435455,220.864177728842,221.362886022229,
221.861594315615,222.360302609002,222.859010902388,223.053078404875),
 .UNSPECIFIED.);
#948=B_SPLINE_CURVE_WITH_KNOTS('',3,(#34722,#34723,#34724,#34725,#34726,
#34727,#34728,#34729,#34730,#34731,#34732,#34733,#34734,#34735,#34736,#34737),
 .UNSPECIFIED.,.F.,.F.,(4,1,1,1,1,1,1,1,1,1,1,1,1,4),(210.486707790516,
210.843597923569,211.342306216956,211.841014510343,212.339722803729,212.838431097116,
213.337139390502,213.835847683889,214.334555977276,214.833264270662,215.331972564049,
215.830680857436,216.329389150822,216.769893097696),.UNSPECIFIED.);
#949=B_SPLINE_CURVE_WITH_KNOTS('',3,(#34738,#34739,#34740,#34741,#34742,
#34743,#34744,#34745,#34746,#34747,#34748,#34749,#34750,#34751,#34752,#34753),
 .UNSPECIFIED.,.F.,.F.,(4,1,1,1,1,1,1,1,1,1,1,1,1,4),(210.486707790516,
210.89001186111,211.388720154496,211.887428447883,212.386136741269,212.884845034656,
213.383553328043,213.882261621429,214.380969914816,214.879678208203,215.378386501589,
215.877094794976,216.375803088362,216.769893097696),.UNSPECIFIED.);
#950=B_SPLINE_CURVE_WITH_KNOTS('',3,(#34758,#34759,#34760,#34761,#34762,
#34763,#34764,#34765,#34766,#34767,#34768,#34769,#34770,#34771,#34772,#34773,
#34774),.UNSPECIFIED.,.F.,.F.,(4,1,1,1,1,1,1,1,1,1,1,1,1,1,4),(204.203522483337,
204.360390109543,204.85909840293,205.357806696317,205.856514989703,206.35522328309,
206.853931576476,207.352639869863,207.85134816325,208.350056456636,208.848764750023,
209.347473043409,209.846181336796,210.344889630183,210.486707790516),
 .UNSPECIFIED.);
#951=B_SPLINE_CURVE_WITH_KNOTS('',3,(#34775,#34776,#34777,#34778,#34779,
#34780,#34781,#34782,#34783,#34784,#34785,#34786,#34787,#34788,#34789,#34790,
#34791),.UNSPECIFIED.,.F.,.F.,(4,1,1,1,1,1,1,1,1,1,1,1,1,1,4),(204.203522483337,
204.406804047084,204.90551234047,205.404220633857,205.902928927243,206.40163722063,
206.900345514017,207.399053807403,207.89776210079,208.396470394177,208.895178687563,
209.39388698095,209.892595274336,210.391303567723,210.486707790516),
 .UNSPECIFIED.);
#952=B_SPLINE_CURVE_WITH_KNOTS('',3,(#34796,#34797,#34798,#34799,#34800,
#34801,#34802,#34803,#34804,#34805,#34806,#34807,#34808,#34809,#34810,#34811),
 .UNSPECIFIED.,.F.,.F.,(4,1,1,1,1,1,1,1,1,1,1,1,1,4),(197.920337176157,
198.375890588904,198.87459888229,199.373307175677,199.872015469064,200.37072376245,
200.869432055837,201.368140349224,201.86684864261,202.365556935997,202.864265229383,
203.36297352277,203.861681816157,204.203522483337),.UNSPECIFIED.);
#953=B_SPLINE_CURVE_WITH_KNOTS('',3,(#34812,#34813,#34814,#34815,#34816,
#34817,#34818,#34819,#34820,#34821,#34822,#34823,#34824,#34825,#34826,#34827,
#34828),.UNSPECIFIED.,.F.,.F.,(4,1,1,1,1,1,1,1,1,1,1,1,1,1,4),(197.920337176157,
197.923596233057,198.422304526444,198.921012819831,199.419721113217,199.918429406604,
200.417137699991,200.915845993377,201.414554286764,201.91326258015,202.411970873537,
202.910679166924,203.40938746031,203.908095753697,204.203522483337),
 .UNSPECIFIED.);
#954=B_SPLINE_CURVE_WITH_KNOTS('',3,(#34833,#34834,#34835,#34836,#34837,
#34838,#34839,#34840,#34841,#34842,#34843,#34844,#34845,#34846,#34847,#34848,
#34849),.UNSPECIFIED.,.F.,.F.,(4,1,1,1,1,1,1,1,1,1,1,1,1,1,4),(191.637151868978,
191.892682774878,192.391391068264,192.890099361651,193.388807655038,193.887515948424,
194.386224241811,194.884932535198,195.383640828584,195.882349121971,196.381057415357,
196.879765708744,197.378474002131,197.877182295517,197.920337176157),
 .UNSPECIFIED.);
#955=B_SPLINE_CURVE_WITH_KNOTS('',3,(#34850,#34851,#34852,#34853,#34854,
#34855,#34856,#34857,#34858,#34859,#34860,#34861,#34862,#34863,#34864,#34865),
 .UNSPECIFIED.,.F.,.F.,(4,1,1,1,1,1,1,1,1,1,1,1,1,4),(191.637151868978,
191.939096712418,192.437805005805,192.936513299191,193.435221592578,193.933929885965,
194.432638179351,194.931346472738,195.430054766124,195.928763059511,196.427471352898,
196.926179646284,197.424887939671,197.920337176157),.UNSPECIFIED.);
#956=B_SPLINE_CURVE_WITH_KNOTS('',3,(#34870,#34871,#34872,#34873,#34874,
#34875,#34876,#34877,#34878,#34879,#34880,#34881,#34882,#34883,#34884,#34885,
#34886),.UNSPECIFIED.,.F.,.F.,(4,1,1,1,1,1,1,1,1,1,1,1,1,1,4),(185.353966561798,
185.409474960852,185.908183254238,186.406891547625,186.905599841012,187.404308134398,
187.903016427785,188.401724721171,188.900433014558,189.399141307945,189.897849601331,
190.396557894718,190.895266188105,191.393974481491,191.637151868978),
 .UNSPECIFIED.);
#957=B_SPLINE_CURVE_WITH_KNOTS('',3,(#34887,#34888,#34889,#34890,#34891,
#34892,#34893,#34894,#34895,#34896,#34897,#34898,#34899,#34900,#34901,#34902,
#34903),.UNSPECIFIED.,.F.,.F.,(4,1,1,1,1,1,1,1,1,1,1,1,1,1,4),(185.353966561798,
185.455888898392,185.954597191779,186.453305485165,186.952013778552,187.450722071938,
187.949430365325,188.448138658712,188.946846952098,189.445555245485,189.944263538872,
190.442971832258,190.941680125645,191.440388419031,191.637151868978),
 .UNSPECIFIED.);
#958=B_SPLINE_CURVE_WITH_KNOTS('',3,(#34908,#34909,#34910,#34911,#34912,
#34913,#34914,#34915,#34916,#34917,#34918,#34919,#34920,#34921,#34922,#34923),
 .UNSPECIFIED.,.F.,.F.,(4,1,1,1,1,1,1,1,1,1,1,1,1,4),(179.070781254618,
179.424975440212,179.923683733599,180.422392026986,180.921100320372,181.419808613759,
181.918516907145,182.417225200532,182.915933493919,183.414641787305,183.913350080692,
184.412058374079,184.910766667465,185.353966561798),.UNSPECIFIED.);
#959=B_SPLINE_CURVE_WITH_KNOTS('',3,(#34924,#34925,#34926,#34927,#34928,
#34929,#34930,#34931,#34932,#34933,#34934,#34935,#34936,#34937,#34938,#34939),
 .UNSPECIFIED.,.F.,.F.,(4,1,1,1,1,1,1,1,1,1,1,1,1,4),(179.070781254618,
179.471389377753,179.970097671139,180.468805964526,180.967514257912,181.466222551299,
181.964930844686,182.463639138072,182.962347431459,183.461055724845,183.959764018232,
184.458472311619,184.957180605005,185.353966561798),.UNSPECIFIED.);
#960=B_SPLINE_CURVE_WITH_KNOTS('',3,(#34944,#34945,#34946,#34947,#34948,
#34949,#34950,#34951,#34952,#34953,#34954,#34955,#34956,#34957,#34958,#34959,
#34960),.UNSPECIFIED.,.F.,.F.,(4,1,1,1,1,1,1,1,1,1,1,1,1,1,4),(172.787595947439,
172.941767626186,173.440475919573,173.93918421296,174.437892506346,174.936600799733,
175.435309093119,175.934017386506,176.432725679893,176.931433973279,177.430142266666,
177.928850560052,178.427558853439,178.926267146826,179.070781254618),
 .UNSPECIFIED.);
#961=B_SPLINE_CURVE_WITH_KNOTS('',3,(#34961,#34962,#34963,#34964,#34965,
#34966,#34967,#34968,#34969,#34970,#34971,#34972,#34973,#34974,#34975,#34976,
#34977),.UNSPECIFIED.,.F.,.F.,(4,1,1,1,1,1,1,1,1,1,1,1,1,1,4),(172.787595947439,
172.988181563726,173.486889857113,173.9855981505,174.484306443886,174.983014737273,
175.48172303066,175.980431324046,176.479139617433,176.977847910819,177.476556204206,
177.975264497593,178.473972790979,178.972681084366,179.070781254618),
 .UNSPECIFIED.);
#962=B_SPLINE_CURVE_WITH_KNOTS('',3,(#34982,#34983,#34984,#34985,#34986,
#34987,#34988,#34989,#34990,#34991,#34992,#34993,#34994,#34995,#34996,#34997),
 .UNSPECIFIED.,.F.,.F.,(4,1,1,1,1,1,1,1,1,1,1,1,1,4),(166.504410640259,
166.957268105547,167.455976398933,167.95468469232,168.453392985707,168.952101279093,
169.45080957248,169.949517865867,170.448226159253,170.94693445264,171.445642746026,
171.944351039413,172.4430593328,172.787595947439),.UNSPECIFIED.);
#963=B_SPLINE_CURVE_WITH_KNOTS('',3,(#34998,#34999,#35000,#35001,#35002,
#35003,#35004,#35005,#35006,#35007,#35008,#35009,#35010,#35011,#35012,#35013,
#35014),.UNSPECIFIED.,.F.,.F.,(4,1,1,1,1,1,1,1,1,1,1,1,1,1,4),(166.504410640259,
166.5049737497,167.003682043087,167.502390336474,168.00109862986,168.499806923247,
168.998515216634,169.49722351002,169.995931803407,170.494640096793,170.99334839018,
171.492056683567,171.990764976953,172.48947327034,172.787595947439),
 .UNSPECIFIED.);
#964=B_SPLINE_CURVE_WITH_KNOTS('',3,(#35019,#35020,#35021,#35022,#35023,
#35024,#35025,#35026,#35027,#35028,#35029,#35030,#35031,#35032,#35033,#35034,
#35035),.UNSPECIFIED.,.F.,.F.,(4,1,1,1,1,1,1,1,1,1,1,1,1,1,4),(160.22122533308,
160.474060291521,160.972768584907,161.471476878294,161.970185171681,162.468893465067,
162.967601758454,163.466310051841,163.965018345227,164.463726638614,164.962434932,
165.461143225387,165.959851518774,166.45855981216,166.504410640259),
 .UNSPECIFIED.);
#965=B_SPLINE_CURVE_WITH_KNOTS('',3,(#35036,#35037,#35038,#35039,#35040,
#35041,#35042,#35043,#35044,#35045,#35046,#35047,#35048,#35049,#35050,#35051),
 .UNSPECIFIED.,.F.,.F.,(4,1,1,1,1,1,1,1,1,1,1,1,1,4),(160.22122533308,160.520474229061,
161.019182522448,161.517890815834,162.016599109221,162.515307402608,163.014015695994,
163.512723989381,164.011432282767,164.510140576154,165.008848869541,165.507557162927,
166.006265456314,166.504410640259),.UNSPECIFIED.);
#966=B_SPLINE_CURVE_WITH_KNOTS('',3,(#35056,#35057,#35058,#35059,#35060,
#35061,#35062,#35063,#35064,#35065,#35066,#35067,#35068,#35069,#35070,#35071,
#35072),.UNSPECIFIED.,.F.,.F.,(4,1,1,1,1,1,1,1,1,1,1,1,1,1,4),(153.9380400259,
153.990852477495,154.489560770881,154.988269064268,155.486977357655,155.985685651041,
156.484393944428,156.983102237814,157.481810531201,157.980518824588,158.479227117974,
158.977935411361,159.476643704748,159.975351998134,160.22122533308),
 .UNSPECIFIED.);
#967=B_SPLINE_CURVE_WITH_KNOTS('',3,(#35073,#35074,#35075,#35076,#35077,
#35078,#35079,#35080,#35081,#35082,#35083,#35084,#35085,#35086,#35087,#35088,
#35089),.UNSPECIFIED.,.F.,.F.,(4,1,1,1,1,1,1,1,1,1,1,1,1,1,4),(153.9380400259,
154.037266415035,154.535974708422,155.034683001808,155.533391295195,156.032099588581,
156.530807881968,157.029516175355,157.528224468741,158.026932762128,158.525641055515,
159.024349348901,159.523057642288,160.021765935674,160.22122533308),
 .UNSPECIFIED.);
#968=B_SPLINE_CURVE_WITH_KNOTS('',3,(#35094,#35095,#35096,#35097,#35098,
#35099,#35100,#35101,#35102,#35103,#35104,#35105,#35106,#35107,#35108,#35109),
 .UNSPECIFIED.,.F.,.F.,(4,1,1,1,1,1,1,1,1,1,1,1,1,4),(147.654854718721,
148.006352956855,148.505061250242,149.003769543629,149.502477837015,150.001186130402,
150.499894423788,150.998602717175,151.497311010562,151.996019303948,152.494727597335,
152.993435890721,153.492144184108,153.9380400259),.UNSPECIFIED.);
#969=B_SPLINE_CURVE_WITH_KNOTS('',3,(#35110,#35111,#35112,#35113,#35114,
#35115,#35116,#35117,#35118,#35119,#35120,#35121,#35122,#35123,#35124,#35125),
 .UNSPECIFIED.,.F.,.F.,(4,1,1,1,1,1,1,1,1,1,1,1,1,4),(147.654854718721,
148.052766894396,148.551475187782,149.050183481169,149.548891774555,150.047600067942,
150.546308361329,151.045016654715,151.543724948102,152.042433241488,152.541141534875,
153.039849828262,153.538558121648,153.9380400259),.UNSPECIFIED.);
#970=B_SPLINE_CURVE_WITH_KNOTS('',3,(#35130,#35131,#35132,#35133,#35134,
#35135,#35136,#35137,#35138,#35139,#35140,#35141,#35142),.UNSPECIFIED.,
 .F.,.F.,(4,1,1,1,1,1,1,1,1,1,4),(141.371669411541,141.523145142829,142.520561729602,
143.517978316376,144.515394903149,145.512811489922,146.011519783309,146.510228076695,
147.008936370082,147.507644663469,147.654854718721),.UNSPECIFIED.);
#971=B_SPLINE_CURVE_WITH_KNOTS('',3,(#35143,#35144,#35145,#35146,#35147,
#35148,#35149,#35150,#35151,#35152),.UNSPECIFIED.,.F.,.F.,(4,1,1,1,1,1,
1,4),(141.371669411541,142.068267373756,143.065683960529,144.063100547303,
145.060517134076,146.057933720849,147.055350307622,147.654854718721),
 .UNSPECIFIED.);
#972=B_SPLINE_CURVE_WITH_KNOTS('',3,(#35157,#35158,#35159,#35160,#35161,
#35162,#35163,#35164,#35165,#35166),.UNSPECIFIED.,.F.,.F.,(4,1,1,1,1,1,
1,4),(135.088484104362,135.53864562219,136.536062208963,137.533478795736,
138.53089538251,139.528311969283,140.525728556056,141.371669411541),
 .UNSPECIFIED.);
#973=B_SPLINE_CURVE_WITH_KNOTS('',3,(#35167,#35168,#35169,#35170,#35171,
#35172,#35173,#35174,#35175,#35176),.UNSPECIFIED.,.F.,.F.,(4,1,1,1,1,1,
1,4),(135.088484104362,136.083767853117,137.08118443989,138.078601026663,
139.076017613436,140.07343420021,141.070850786983,141.371669411541),
 .UNSPECIFIED.);
#974=B_SPLINE_CURVE_WITH_KNOTS('',3,(#35181,#35182,#35183,#35184,#35185,
#35186,#35187,#35188,#35189,#35190,#35191,#35192,#35193),.UNSPECIFIED.,
 .F.,.F.,(4,1,1,1,1,1,1,1,1,1,4),(128.805298797182,129.055437808164,129.55414610155,
130.052854394937,130.551562688324,131.05027098171,131.548979275097,132.54639586187,
133.543812448643,134.541229035417,135.088484104362),.UNSPECIFIED.);
#975=B_SPLINE_CURVE_WITH_KNOTS('',3,(#35194,#35195,#35196,#35197,#35198,
#35199,#35200,#35201,#35202,#35203,#35204,#35205,#35206,#35207,#35208,#35209),
 .UNSPECIFIED.,.F.,.F.,(4,1,1,1,1,1,1,1,1,1,1,1,1,4),(128.805298797182,
129.101851745704,129.600560039091,130.099268332477,130.597976625864,131.09668491925,
131.595393212637,132.094101506024,132.59280979941,133.091518092797,133.590226386184,
134.08893467957,135.086351266343,135.088484104362),.UNSPECIFIED.);
#976=B_SPLINE_CURVE_WITH_KNOTS('',3,(#35214,#35215,#35216,#35217,#35218,
#35219,#35220,#35221,#35222,#35223,#35224,#35225,#35226,#35227,#35228,#35229,
#35230),.UNSPECIFIED.,.F.,.F.,(4,1,1,1,1,1,1,1,1,1,1,1,1,1,4),(122.522113490002,
122.572229994138,123.070938287524,123.569646580911,124.068354874298,124.567063167684,
125.065771461071,125.564479754457,126.063188047844,126.561896341231,127.060604634617,
127.559312928004,128.058021221391,128.556729514777,128.805298797182),
 .UNSPECIFIED.);
#977=B_SPLINE_CURVE_WITH_KNOTS('',3,(#35231,#35232,#35233,#35234,#35235,
#35236,#35237,#35238,#35239,#35240,#35241,#35242,#35243,#35244,#35245,#35246,
#35247),.UNSPECIFIED.,.F.,.F.,(4,1,1,1,1,1,1,1,1,1,1,1,1,1,4),(122.522113490002,
122.618643931678,123.117352225065,123.616060518451,124.114768811838,124.613477105224,
125.112185398611,125.610893691998,126.109601985384,126.608310278771,127.107018572158,
127.605726865544,128.104435158931,128.603143452317,128.805298797182),
 .UNSPECIFIED.);
#978=B_SPLINE_CURVE_WITH_KNOTS('',3,(#35252,#35253,#35254,#35255,#35256,
#35257,#35258,#35259,#35260,#35261,#35262,#35263,#35264,#35265,#35266,#35267),
 .UNSPECIFIED.,.F.,.F.,(4,1,1,1,1,1,1,1,1,1,1,1,1,4),(116.238928182823,
116.587730473498,117.086438766885,117.585147060271,118.083855353658,118.582563647045,
119.081271940431,119.579980233818,120.078688527205,120.577396820591,121.076105113978,
121.574813407364,122.073521700751,122.522113490002),.UNSPECIFIED.);
#979=B_SPLINE_CURVE_WITH_KNOTS('',3,(#35268,#35269,#35270,#35271,#35272,
#35273,#35274,#35275,#35276,#35277,#35278,#35279,#35280,#35281,#35282,#35283),
 .UNSPECIFIED.,.F.,.F.,(4,1,1,1,1,1,1,1,1,1,1,1,1,4),(116.238928182823,
116.634144411039,117.132852704425,117.631560997812,118.130269291198,118.628977584585,
119.127685877972,119.626394171358,120.125102464745,120.623810758131,121.122519051518,
121.621227344905,122.119935638291,122.522113490002),.UNSPECIFIED.);
#980=B_SPLINE_CURVE_WITH_KNOTS('',3,(#35288,#35289,#35290,#35291,#35292,
#35293,#35294,#35295,#35296,#35297,#35298,#35299,#35300,#35301,#35302,#35303,
#35304),.UNSPECIFIED.,.F.,.F.,(4,1,1,1,1,1,1,1,1,1,1,1,1,1,4),(109.955742875643,
110.104522659472,110.603230952859,111.101939246245,111.600647539632,112.099355833019,
112.598064126405,113.096772419792,113.595480713179,114.094189006565,114.592897299952,
115.091605593338,115.590313886725,116.089022180112,116.238928182823),
 .UNSPECIFIED.);
#981=B_SPLINE_CURVE_WITH_KNOTS('',3,(#35305,#35306,#35307,#35308,#35309,
#35310,#35311,#35312,#35313,#35314,#35315,#35316,#35317,#35318,#35319,#35320,
#35321),.UNSPECIFIED.,.F.,.F.,(4,1,1,1,1,1,1,1,1,1,1,1,1,1,4),(109.955742875643,
110.150936597012,110.649644890399,111.148353183786,111.647061477172,112.145769770559,
112.644478063946,113.143186357332,113.641894650719,114.140602944105,114.639311237492,
115.138019530879,115.636727824265,116.135436117652,116.238928182823),
 .UNSPECIFIED.);
#982=B_SPLINE_CURVE_WITH_KNOTS('',3,(#35326,#35327,#35328,#35329,#35330,
#35331,#35332,#35333,#35334,#35335,#35336,#35337,#35338,#35339,#35340,#35341),
 .UNSPECIFIED.,.F.,.F.,(4,1,1,1,1,1,1,1,1,1,1,1,1,4),(103.672557568464,
104.120023138833,104.618731432219,105.117439725606,105.616148018993,106.114856312379,
106.613564605766,107.112272899152,107.610981192539,108.109689485926,108.608397779312,
109.107106072699,109.605814366086,109.955742875643),.UNSPECIFIED.);
#983=B_SPLINE_CURVE_WITH_KNOTS('',3,(#35342,#35343,#35344,#35345,#35346,
#35347,#35348,#35349,#35350,#35351,#35352,#35353,#35354,#35355,#35356,#35357),
 .UNSPECIFIED.,.F.,.F.,(4,1,1,1,1,1,1,1,1,1,1,1,1,4),(103.672557568464,
104.166437076373,104.66514536976,105.163853663146,105.662561956533,106.161270249919,
106.659978543306,107.158686836693,107.657395130079,108.156103423466,108.654811716853,
109.153520010239,109.652228303626,109.955742875643),.UNSPECIFIED.);
#984=B_SPLINE_CURVE_WITH_KNOTS('',3,(#35362,#35363,#35364,#35365,#35366,
#35367,#35368,#35369,#35370,#35371,#35372,#35373,#35374,#35375,#35376,#35377,
#35378),.UNSPECIFIED.,.F.,.F.,(4,1,1,1,1,1,1,1,1,1,1,1,1,1,4),(97.389372261284,
97.6368153248067,98.1355236181933,98.63423191158,99.1329402049666,99.6316484983532,
100.13035679174,100.629065085126,101.127773378513,101.6264816719,102.125189965286,
102.623898258673,103.12260655206,103.621314845446,103.672557568464),
 .UNSPECIFIED.);
#985=B_SPLINE_CURVE_WITH_KNOTS('',3,(#35379,#35380,#35381,#35382,#35383,
#35384,#35385,#35386,#35387,#35388,#35389,#35390,#35391,#35392,#35393,#35394,
#35395),.UNSPECIFIED.,.F.,.F.,(4,1,1,1,1,1,1,1,1,1,1,1,1,1,4),(97.389372261284,
97.683229262347,98.1819375557336,98.6806458491202,99.1793541425068,99.6780624358935,
100.17677072928,100.675479022667,101.174187316053,101.67289560944,102.171603902827,
102.670312196213,103.1690204896,103.667728782986,103.672557568464),
 .UNSPECIFIED.);
#986=B_SPLINE_CURVE_WITH_KNOTS('',3,(#35400,#35401,#35402,#35403,#35404,
#35405,#35406,#35407,#35408,#35409,#35410,#35411,#35412,#35413,#35414,#35415,
#35416),.UNSPECIFIED.,.F.,.F.,(4,1,1,1,1,1,1,1,1,1,1,1,1,1,4),(91.1061869541044,
91.1536075107807,91.6523158041673,92.1510240975539,92.6497323909405,93.1484406843271,
93.6471489777138,94.1458572711004,94.644565564487,95.1432738578736,95.6419821512603,
96.1406904446469,96.6393987380335,97.1381070314201,97.389372261284),
 .UNSPECIFIED.);
#987=B_SPLINE_CURVE_WITH_KNOTS('',3,(#35417,#35418,#35419,#35420,#35421,
#35422,#35423,#35424,#35425,#35426,#35427,#35428,#35429,#35430,#35431,#35432,
#35433),.UNSPECIFIED.,.F.,.F.,(4,1,1,1,1,1,1,1,1,1,1,1,1,1,4),(91.1061869541044,
91.2000214483209,91.6987297417075,92.1974380350942,92.6961463284808,93.1948546218674,
93.693562915254,94.1922712086406,94.6909795020272,95.1896877954139,95.6883960888005,
96.1871043821871,96.6858126755737,97.1845209689603,97.389372261284),
 .UNSPECIFIED.);
#988=B_SPLINE_CURVE_WITH_KNOTS('',3,(#35438,#35439,#35440,#35441,#35442,
#35443,#35444,#35445,#35446,#35447,#35448,#35449,#35450,#35451,#35452,#35453),
 .UNSPECIFIED.,.F.,.F.,(4,1,1,1,1,1,1,1,1,1,1,1,1,4),(84.8230016469248,
85.1691079901412,85.6678162835279,86.1665245769145,86.6652328703011,87.1639411636877,
87.6626494570743,88.161357750461,88.6600660438476,89.1587743372342,89.6574826306208,
90.1561909240074,90.654899217394,91.1061869541044),.UNSPECIFIED.);
#989=B_SPLINE_CURVE_WITH_KNOTS('',3,(#35454,#35455,#35456,#35457,#35458,
#35459,#35460,#35461,#35462,#35463,#35464,#35465,#35466,#35467,#35468,#35469),
 .UNSPECIFIED.,.F.,.F.,(4,1,1,1,1,1,1,1,1,1,1,1,1,4),(84.8230016469248,
85.2155219276815,85.7142302210681,86.2129385144547,86.7116468078413,87.2103551012279,
87.7090633946146,88.2077716880012,88.7064799813878,89.2051882747744,89.703896568161,
90.2026048615477,90.7013131549343,91.1061869541044),.UNSPECIFIED.);
#990=B_SPLINE_CURVE_WITH_KNOTS('',3,(#35474,#35475,#35476,#35477,#35478,
#35479,#35480,#35481,#35482,#35483,#35484,#35485,#35486,#35487,#35488,#35489,
#35490),.UNSPECIFIED.,.F.,.F.,(4,1,1,1,1,1,1,1,1,1,1,1,1,1,4),(78.5398163397452,
78.6859001761152,79.1846084695018,79.6833167628884,80.1820250562751,80.6807333496617,
81.1794416430483,81.6781499364349,82.1768582298215,82.6755665232081,83.1742748165948,
83.6729831099814,84.171691403368,84.6703996967546,84.8230016469248),
 .UNSPECIFIED.);
#991=B_SPLINE_CURVE_WITH_KNOTS('',3,(#35491,#35492,#35493,#35494,#35495,
#35496,#35497,#35498,#35499,#35500,#35501,#35502,#35503,#35504,#35505,#35506,
#35507),.UNSPECIFIED.,.F.,.F.,(4,1,1,1,1,1,1,1,1,1,1,1,1,1,4),(78.5398163397452,
78.7323141136554,79.231022407042,79.7297307004287,80.2284389938153,80.7271472872019,
81.2258555805885,81.7245638739751,82.2232721673618,82.7219804607484,83.220688754135,
83.7193970475216,84.2181053409082,84.7168136342949,84.8230016469248),
 .UNSPECIFIED.);
#992=B_SPLINE_CURVE_WITH_KNOTS('',3,(#35512,#35513,#35514,#35515,#35516,
#35517,#35518,#35519,#35520,#35521,#35522,#35523,#35524,#35525,#35526,#35527),
 .UNSPECIFIED.,.F.,.F.,(4,1,1,1,1,1,1,1,1,1,1,1,1,4),(72.2566310325657,
72.7014006554758,73.2001089488624,73.698817242249,74.1975255356356,74.6962338290222,
75.1949421224089,75.6936504157955,76.1923587091821,76.6910670025687,77.1897752959553,
77.6884835893419,78.1871918827286,78.5398163397452),.UNSPECIFIED.);
#993=B_SPLINE_CURVE_WITH_KNOTS('',3,(#35528,#35529,#35530,#35531,#35532,
#35533,#35534,#35535,#35536,#35537,#35538,#35539,#35540,#35541,#35542,#35543),
 .UNSPECIFIED.,.F.,.F.,(4,1,1,1,1,1,1,1,1,1,1,1,1,4),(72.2566310325657,
72.747814593016,73.2465228864026,73.7452311797892,74.2439394731758,74.7426477665625,
75.2413560599491,75.7400643533357,76.2387726467223,76.7374809401089,77.2361892334956,
77.7348975268822,78.2336058202688,78.5398163397452),.UNSPECIFIED.);
#994=B_SPLINE_CURVE_WITH_KNOTS('',3,(#35548,#35549,#35550,#35551,#35552,
#35553,#35554,#35555,#35556,#35557,#35558,#35559,#35560,#35561,#35562,#35563,
#35564),.UNSPECIFIED.,.F.,.F.,(4,1,1,1,1,1,1,1,1,1,1,1,1,1,4),(65.973445725386,
66.2181928414497,66.7169011348363,67.2156094282229,67.7143177216096,68.2130260149962,
68.7117343083828,69.2104426017694,69.709150895156,70.2078591885427,70.7065674819293,
71.2052757753159,71.7039840687025,72.2026923620891,72.2566310325657),
 .UNSPECIFIED.);
#995=B_SPLINE_CURVE_WITH_KNOTS('',3,(#35565,#35566,#35567,#35568,#35569,
#35570,#35571,#35572,#35573,#35574,#35575,#35576,#35577,#35578,#35579,#35580,
#35581),.UNSPECIFIED.,.F.,.F.,(4,1,1,1,1,1,1,1,1,1,1,1,1,1,4),(65.973445725386,
66.2646067789899,66.7633150723765,67.2620233657632,67.7607316591498,68.2594399525364,
68.758148245923,69.2568565393096,69.7555648326963,70.2542731260829,70.7529814194695,
71.2516897128561,71.7503980062427,72.2491062996294,72.2566310325657),
 .UNSPECIFIED.);
#996=B_SPLINE_CURVE_WITH_KNOTS('',3,(#35586,#35587,#35588,#35589,#35590,
#35591,#35592,#35593,#35594,#35595,#35596,#35597,#35598,#35599,#35600,#35601,
#35602),.UNSPECIFIED.,.F.,.F.,(4,1,1,1,1,1,1,1,1,1,1,1,1,1,4),(59.6902604182065,
59.7349850274237,60.2336933208103,60.7324016141969,61.2311099075835,61.7298182009701,
62.2285264943567,62.7272347877434,63.22594308113,63.7246513745166,64.2233596679032,
64.7220679612898,65.2207762546765,65.7194845480631,65.973445725386),
 .UNSPECIFIED.);
#997=B_SPLINE_CURVE_WITH_KNOTS('',3,(#35603,#35604,#35605,#35606,#35607,
#35608,#35609,#35610,#35611,#35612,#35613,#35614,#35615,#35616,#35617,#35618,
#35619),.UNSPECIFIED.,.F.,.F.,(4,1,1,1,1,1,1,1,1,1,1,1,1,1,4),(59.6902604182065,
59.7813989649639,60.2801072583505,60.7788155517371,61.2775238451237,61.7762321385104,
62.274940431897,62.7736487252836,63.2723570186702,63.7710653120568,64.2697736054434,
64.7684818988301,65.2671901922167,65.7658984856033,65.973445725386),
 .UNSPECIFIED.);
#998=B_SPLINE_CURVE_WITH_KNOTS('',3,(#35624,#35625,#35626,#35627,#35628,
#35629,#35630,#35631,#35632,#35633,#35634,#35635,#35636,#35637,#35638,#35639),
 .UNSPECIFIED.,.F.,.F.,(4,1,1,1,1,1,1,1,1,1,1,1,1,4),(53.4070751110269,
53.7504855067842,54.2491938001708,54.7479020935575,55.2466103869441,55.7453186803307,
56.2440269737173,56.7427352671039,57.2414435604906,57.7401518538772,58.2388601472638,
58.7375684406504,59.236276734037,59.6902604182065),.UNSPECIFIED.);
#999=B_SPLINE_CURVE_WITH_KNOTS('',3,(#35640,#35641,#35642,#35643,#35644,
#35645,#35646,#35647,#35648,#35649,#35650,#35651,#35652,#35653,#35654,#35655),
 .UNSPECIFIED.,.F.,.F.,(4,1,1,1,1,1,1,1,1,1,1,1,1,4),(53.4070751110269,
53.7968994443244,54.2956077377111,54.7943160310977,55.2930243244843,55.7917326178709,
56.2904409112575,56.7891492046442,57.2878574980308,57.7865657914174,58.285274084804,
58.7839823781906,59.2826906715772,59.6902604182065),.UNSPECIFIED.);
#1000=B_SPLINE_CURVE_WITH_KNOTS('',3,(#35660,#35661,#35662,#35663,#35664,
#35665,#35666,#35667,#35668,#35669,#35670,#35671,#35672,#35673,#35674,#35675,
#35676),.UNSPECIFIED.,.F.,.F.,(4,1,1,1,1,1,1,1,1,1,1,1,1,1,4),(47.1238898038473,
47.2672776927582,47.7659859861448,48.2646942795314,48.763402572918,49.2621108663046,
49.7608191596913,50.2595274530779,50.7582357464645,51.2569440398511,51.7556523332377,
52.2543606266244,52.753068920011,53.2517772133976,53.4070751110269),
 .UNSPECIFIED.);
#1001=B_SPLINE_CURVE_WITH_KNOTS('',3,(#35677,#35678,#35679,#35680,#35681,
#35682,#35683,#35684,#35685,#35686,#35687,#35688,#35689,#35690,#35691,#35692,
#35693),.UNSPECIFIED.,.F.,.F.,(4,1,1,1,1,1,1,1,1,1,1,1,1,1,4),(47.1238898038473,
47.3136916302984,47.812399923685,48.3111082170716,48.8098165104582,49.3085248038449,
49.8072330972315,50.3059413906181,50.8046496840047,51.3033579773913,51.802066270778,
52.3007745641646,52.7994828575512,53.2981911509378,53.4070751110269),
 .UNSPECIFIED.);
#1002=B_SPLINE_CURVE_WITH_KNOTS('',3,(#35698,#35699,#35700,#35701,#35702,
#35703,#35704,#35705,#35706,#35707,#35708,#35709,#35710,#35711,#35712,#35713),
 .UNSPECIFIED.,.F.,.F.,(4,1,1,1,1,1,1,1,1,1,1,1,1,4),(40.8407044966677,
41.2827781721187,41.7814864655054,42.280194758892,42.7789030522786,43.2776113456652,
43.7763196390518,44.2750279324384,44.7737362258251,45.2724445192117,45.7711528125983,
46.2698611059849,46.7685693993716,47.1238898038473),.UNSPECIFIED.);
#1003=B_SPLINE_CURVE_WITH_KNOTS('',3,(#35714,#35715,#35716,#35717,#35718,
#35719,#35720,#35721,#35722,#35723,#35724,#35725,#35726,#35727,#35728,#35729),
 .UNSPECIFIED.,.F.,.F.,(4,1,1,1,1,1,1,1,1,1,1,1,1,4),(40.8407044966677,
41.3291921096589,41.8279004030456,42.3266086964322,42.8253169898188,43.3240252832054,
43.822733576592,44.3214418699787,44.8201501633653,45.3188584567519,45.8175667501385,
46.3162750435251,46.8149833369118,47.1238898038473),.UNSPECIFIED.);
#1004=B_SPLINE_CURVE_WITH_KNOTS('',3,(#35734,#35735,#35736,#35737,#35738,
#35739,#35740,#35741,#35742,#35743,#35744,#35745,#35746,#35747,#35748,#35749,
#35750),.UNSPECIFIED.,.F.,.F.,(4,1,1,1,1,1,1,1,1,1,1,1,1,1,4),(34.5575191894881,
34.7995703580927,35.2982786514793,35.7969869448659,36.2956952382525,36.7944035316392,
37.2931118250258,37.7918201184124,38.290528411799,38.7892367051856,39.2879449985723,
39.7866532919589,40.2853615853455,40.7840698787321,40.8407044966677),
 .UNSPECIFIED.);
#1005=B_SPLINE_CURVE_WITH_KNOTS('',3,(#35751,#35752,#35753,#35754,#35755,
#35756,#35757,#35758,#35759,#35760,#35761,#35762,#35763,#35764,#35765,#35766,
#35767),.UNSPECIFIED.,.F.,.F.,(4,1,1,1,1,1,1,1,1,1,1,1,1,1,4),(34.5575191894881,
34.8459842956329,35.3446925890195,35.8434008824061,36.3421091757927,36.8408174691794,
37.339525762566,37.8382340559526,38.3369423493392,38.8356506427259,39.3343589361125,
39.8330672294991,40.3317755228857,40.8304838162723,40.8407044966677),
 .UNSPECIFIED.);
#1006=B_SPLINE_CURVE_WITH_KNOTS('',3,(#35772,#35773,#35774,#35775,#35776,
#35777,#35778,#35779,#35780,#35781,#35782,#35783,#35784,#35785,#35786,#35787,
#35788),.UNSPECIFIED.,.F.,.F.,(4,1,1,1,1,1,1,1,1,1,1,1,1,1,4),(28.2743338823085,
28.3163625440666,28.8150708374532,29.3137791308399,29.8124874242265,30.3111957176131,
30.8099040109997,31.3086123043863,31.807320597773,32.3060288911596,32.8047371845462,
33.3034454779328,33.8021537713194,34.3008620647061,34.5575191894881),
 .UNSPECIFIED.);
#1007=B_SPLINE_CURVE_WITH_KNOTS('',3,(#35789,#35790,#35791,#35792,#35793,
#35794,#35795,#35796,#35797,#35798,#35799,#35800,#35801,#35802,#35803,#35804,
#35805),.UNSPECIFIED.,.F.,.F.,(4,1,1,1,1,1,1,1,1,1,1,1,1,1,4),(28.2743338823085,
28.3627764816068,28.8614847749935,29.3601930683801,29.8589013617667,30.3576096551533,
30.8563179485399,31.3550262419266,31.8537345353132,32.3524428286998,32.8511511220864,
33.349859415473,33.8485677088597,34.3472760022463,34.5575191894881),
 .UNSPECIFIED.);
#1008=B_SPLINE_CURVE_WITH_KNOTS('',3,(#35810,#35811,#35812,#35813,#35814,
#35815,#35816,#35817,#35818,#35819,#35820,#35821,#35822,#35823,#35824,#35825),
 .UNSPECIFIED.,.F.,.F.,(4,1,1,1,1,1,1,1,1,1,1,1,1,4),(21.9911485751289,
22.3318630234272,22.8305713168138,23.3292796102004,23.8279879035871,24.3266961969737,
24.8254044903603,25.3241127837469,25.8228210771335,26.3215293705201,26.8202376639068,
27.3189459572934,27.81765425068,28.2743338823085),.UNSPECIFIED.);
#1009=B_SPLINE_CURVE_WITH_KNOTS('',3,(#35826,#35827,#35828,#35829,#35830,
#35831,#35832,#35833,#35834,#35835,#35836,#35837,#35838,#35839,#35840,#35841),
 .UNSPECIFIED.,.F.,.F.,(4,1,1,1,1,1,1,1,1,1,1,1,1,4),(21.9911485751289,
22.3782769609674,22.876985254354,23.3756935477406,23.8744018411273,24.3731101345139,
24.8718184279005,25.3705267212871,25.8692350146737,26.3679433080604,26.866651601447,
27.3653598948336,27.8640681882202,28.2743338823085),.UNSPECIFIED.);
#1010=B_SPLINE_CURVE_WITH_KNOTS('',3,(#35847,#35848,#35849,#35850,#35851,
#35852),.UNSPECIFIED.,.F.,.F.,(4,1,1,4),(14.3989442667815,14.8976525601681,
15.3963608535547,15.7079632679493),.UNSPECIFIED.);
#1011=B_SPLINE_CURVE_WITH_KNOTS('',3,(#35855,#35856,#35857,#35858,#35859,
#35860,#35861),.UNSPECIFIED.,.F.,.F.,(4,1,1,1,4),(13.8753896155274,14.3525303292413,
14.8512386226279,15.3499469160145,15.7079632679493),.UNSPECIFIED.);
#1012=B_SPLINE_CURVE_WITH_KNOTS('',3,(#35863,#35864,#35865,#35866,#35867,
#35868,#35869,#35870,#35871,#35872,#35873,#35874,#35875,#35876,#35877,#35878,
#35879,#35880,#35881,#35882,#35883,#35884,#35885,#35886,#35887,#35888,#35889,
#35890,#35891,#35892,#35893,#35894,#35895,#35896,#35897,#35898,#35899,#35900,
#35901,#35902,#35903,#35904,#35905,#35906,#35907,#35908,#35909,#35910,#35911,
#35912,#35913,#35914,#35915,#35916,#35917,#35918,#35919,#35920,#35921,#35922,
#35923,#35924,#35925,#35926,#35927,#35928,#35929,#35930,#35931,#35932,#35933,
#35934,#35935,#35936,#35937,#35938,#35939,#35940,#35941,#35942,#35943,#35944,
#35945,#35946,#35947,#35948,#35949,#35950,#35951,#35952,#35953,#35954,#35955,
#35956,#35957,#35958,#35959,#35960,#35961,#35962,#35963,#35964,#35965,#35966,
#35967,#35968),.UNSPECIFIED.,.F.,.F.,(4,3,3,3,3,3,3,3,3,3,3,3,3,3,3,3,3,
3,3,3,3,3,3,3,3,3,3,3,3,3,3,3,3,3,3,4),(-0.972375876542216,-0.931557379101648,
-0.890218542042487,-0.869392708916521,-0.861677237530619,-0.819813801882793,
-0.781167845425456,-0.769475619651221,-0.760546025724648,-0.754411794373795,
-0.74252188896812,-0.700976733031894,-0.65877791376378,-0.616292150528589,
-0.588572673703484,-0.579879678859757,-0.574332463387633,-0.531223905437004,
-0.505414243228169,-0.462559206201071,-0.419378313085458,-0.399643768345371,
-0.391565714980685,-0.383732909736738,-0.340135839018284,-0.296193649678293,
-0.261501955164762,-0.217668074296404,-0.204748702273309,-0.197210738162037,
-0.192140598791969,-0.1468449795757,-0.102253744983165,-0.0566059334550285,
-0.0109581219268922,0.),.UNSPECIFIED.);
#1013=B_SPLINE_CURVE_WITH_KNOTS('',3,(#35969,#35970,#35971,#35972,#35973,
#35974,#35975,#35976,#35977,#35978,#35979,#35980,#35981,#35982,#35983,#35984,
#35985,#35986,#35987,#35988,#35989,#35990,#35991,#35992,#35993,#35994,#35995,
#35996,#35997,#35998,#35999,#36000,#36001,#36002,#36003,#36004,#36005,#36006,
#36007,#36008,#36009,#36010,#36011,#36012,#36013,#36014,#36015,#36016,#36017,
#36018,#36019,#36020,#36021,#36022,#36023,#36024,#36025,#36026,#36027,#36028,
#36029,#36030,#36031,#36032,#36033,#36034,#36035,#36036,#36037,#36038,#36039,
#36040,#36041,#36042,#36043,#36044,#36045,#36046,#36047,#36048,#36049,#36050,
#36051,#36052,#36053,#36054,#36055,#36056,#36057,#36058,#36059,#36060,#36061,
#36062,#36063,#36064,#36065,#36066,#36067,#36068,#36069,#36070,#36071),
 .UNSPECIFIED.,.F.,.F.,(4,3,3,3,3,3,3,3,3,3,3,3,3,3,3,3,3,3,3,3,3,3,3,3,
3,3,3,3,3,3,3,3,3,3,4),(-0.970006587573357,-0.925489021709122,-0.880831606117785,
-0.860106336836479,-0.852213503588024,-0.808023919462815,-0.764142093829507,
-0.741127929891385,-0.732995659095006,-0.720260268196198,-0.676886083169421,
-0.633189091074775,-0.58989356338977,-0.561603730397805,-0.548456029491321,
-0.542926374323804,-0.500045602531121,-0.476734231421911,-0.433752968122039,
-0.390893110149348,-0.372012672166435,-0.363955407652349,-0.356648068723258,
-0.314412819484753,-0.272458136815843,-0.239849606286048,-0.197688110523089,
-0.185715478561588,-0.179206252930902,-0.173732780061183,-0.132200928727762,
-0.0907046629355285,-0.0499294541163457,-0.00977294415302305,0.),
 .UNSPECIFIED.);
#1014=B_SPLINE_CURVE_WITH_KNOTS('',3,(#36073,#36074,#36075,#36076,#36077,
#36078,#36079,#36080,#36081,#36082,#36083,#36084,#36085,#36086,#36087,#36088,
#36089),.UNSPECIFIED.,.F.,.F.,(4,1,1,1,1,1,1,1,1,1,1,1,1,1,4),(15.7079632679493,
15.8486552094011,16.3473635027878,16.8460717961744,17.344780089561,17.8434883829476,
18.3421966763342,18.8409049697209,19.3396132631075,19.8383215564941,20.3370298498807,
20.8357381432673,21.334446436654,21.8331547300406,21.9911485751289),
 .UNSPECIFIED.);
#1015=B_SPLINE_CURVE_WITH_KNOTS('',3,(#36090,#36091,#36092,#36093,#36094,
#36095,#36096,#36097,#36098,#36099,#36100,#36101,#36102,#36103,#36104,#36105,
#36106),.UNSPECIFIED.,.F.,.F.,(4,1,1,1,1,1,1,1,1,1,1,1,1,1,4),(15.7079632679493,
15.8950691469414,16.393777440328,16.8924857337146,17.3911940271012,17.8899023204878,
18.3886106138744,18.8873189072611,19.3860272006477,19.8847354940343,20.3834437874209,
20.8821520808075,21.3808603741942,21.8795686675808,21.9911485751289),
 .UNSPECIFIED.);
#1016=B_SPLINE_CURVE_WITH_KNOTS('',3,(#38095,#38096,#38097,#38098,#38099,
#38100,#38101,#38102,#38103,#38104,#38105,#38106,#38107,#38108,#38109,#38110,
#38111,#38112,#38113,#38114,#38115,#38116,#38117,#38118,#38119,#38120,#38121,
#38122,#38123,#38124,#38125,#38126,#38127,#38128,#38129,#38130,#38131,#38132,
#38133,#38134,#38135,#38136,#38137,#38138,#38139,#38140,#38141,#38142,#38143,
#38144,#38145,#38146,#38147,#38148,#38149,#38150,#38151,#38152,#38153,#38154,
#38155,#38156,#38157,#38158,#38159,#38160,#38161,#38162,#38163,#38164,#38165,
#38166,#38167,#38168,#38169,#38170,#38171,#38172,#38173,#38174,#38175,#38176,
#38177,#38178,#38179,#38180,#38181,#38182,#38183,#38184,#38185,#38186,#38187,
#38188,#38189,#38190,#38191,#38192,#38193,#38194,#38195,#38196,#38197,#38198,
#38199,#38200),.UNSPECIFIED.,.F.,.F.,(4,3,3,3,3,3,3,3,3,3,3,3,3,3,3,3,3,
3,3,3,3,3,3,3,3,3,3,3,3,3,3,3,3,3,3,4),(0.,0.040424976116911,0.081552621191953,
0.123116379418818,0.164484386952486,0.177258002125512,0.182429040513286,
0.224585211732574,0.229750939065668,0.271485437391992,0.313663426362065,
0.351832391899687,0.358992185792409,0.364434825962351,0.407093430609824,
0.45008484068709,0.466339288512555,0.509174339674324,0.534227886997736,
0.545013114142881,0.550666578456316,0.593964513128218,0.637614398405316,
0.68114810979745,0.709602718261623,0.725600523556765,0.736529828545389,
0.743509911151027,0.78723345430323,0.830193673824424,0.848440235266336,
0.858098500020291,0.902703209392534,0.947246712359152,0.959074332388006,
0.970006587573436),.UNSPECIFIED.);
#1017=B_SPLINE_CURVE_WITH_KNOTS('',3,(#38201,#38202,#38203,#38204,#38205,
#38206,#38207,#38208,#38209,#38210,#38211,#38212,#38213,#38214,#38215,#38216,
#38217,#38218,#38219,#38220,#38221,#38222,#38223,#38224,#38225,#38226,#38227,
#38228,#38229,#38230,#38231,#38232,#38233,#38234,#38235,#38236,#38237,#38238,
#38239,#38240,#38241,#38242,#38243),.UNSPECIFIED.,.F.,.F.,(4,3,3,3,3,3,
3,3,3,3,3,3,3,3,4),(-10.1321597128207,-9.97416586773239,-9.47545757434577,
-8.97674928095915,-8.47804098757253,-7.97933269418591,-7.48062440079929,
-6.98191610741267,-6.48320781402605,-5.98449952063943,-5.48579122725281,
-4.98708293386619,-4.48837464047957,-3.98966634709295,-3.84897440564115),
 .UNSPECIFIED.);
#1018=B_SPLINE_CURVE_WITH_KNOTS('',3,(#40232,#40233,#40234,#40235,#40236,
#40237,#40238,#40239,#40240,#40241,#40242,#40243,#40244,#40245,#40246,#40247,
#40248,#40249,#40250,#40251,#40252,#40253,#40254,#40255,#40256,#40257,#40258,
#40259,#40260,#40261,#40262,#40263,#40264,#40265,#40266,#40267,#40268,#40269,
#40270,#40271),.UNSPECIFIED.,.F.,.F.,(4,3,3,3,3,3,3,3,3,3,3,3,3,4),(7.59220430834772,
7.97933269418591,8.47804098757253,8.97674928095915,9.47545757434577,9.97416586773239,
10.472874161119,10.9715824545056,11.4702907478922,11.9689990412789,12.4677073346655,
12.9664156280521,13.4651239214387,13.8753896155273),.UNSPECIFIED.);
#1019=B_SPLINE_CURVE_WITH_KNOTS('',3,(#40272,#40273,#40274,#40275,#40276,
#40277,#40278,#40279,#40280,#40281,#40282,#40283,#40284,#40285,#40286,#40287,
#40288,#40289,#40290,#40291,#40292,#40293,#40294,#40295,#40296,#40297,#40298,
#40299,#40300,#40301,#40302,#40303,#40304,#40305,#40306,#40307,#40308,#40309,
#40310,#40311,#40312,#40313,#40314,#40315,#40316,#40317,#40318,#40319,#40320,
#40321,#40322,#40323,#40324,#40325,#40326,#40327,#40328,#40329,#40330,#40331,
#40332,#40333,#40334,#40335,#40336,#40337,#40338,#40339,#40340,#40341,#40342,
#40343,#40344,#40345,#40346,#40347,#40348,#40349,#40350,#40351,#40352,#40353,
#40354,#40355,#40356,#40357,#40358,#40359,#40360,#40361,#40362,#40363,#40364,
#40365,#40366,#40367,#40368,#40369,#40370,#40371,#40372,#40373,#40374,#40375,
#40376,#40377),.UNSPECIFIED.,.F.,.F.,(4,3,3,3,3,3,3,3,3,3,3,3,3,3,3,3,3,
3,3,3,3,3,3,3,3,3,3,3,3,3,3,3,3,3,3,4),(0.,0.0441576970943254,0.088758491595093,
0.133154322886181,0.177017836347152,0.193697049021019,0.19965188566726,
0.243475277581627,0.250795014009384,0.294669452308725,0.338569619728244,
0.37767568962022,0.38721824859893,0.393275053464473,0.436458598855563,0.479377262352089,
0.494993899296151,0.538189921814499,0.562468636762688,0.572092716170009,
0.579226787127647,0.621711263641225,0.664154373258728,0.70594102510778,
0.732419641400012,0.748330061688134,0.757222465646011,0.763401818269173,
0.80529293424602,0.844615778238015,0.861173358979439,0.871344162504664,
0.912748133225373,0.953576775379504,0.962584310214001,0.972375876542313),
 .UNSPECIFIED.);
#1020=B_SPLINE_CURVE_WITH_KNOTS('',3,(#40383,#40384,#40385,#40386,#40387,
#40388,#40389,#40390,#40391,#40392,#40393,#40394,#40395,#40396,#40397,#40398,
#40399,#40400,#40401,#40402,#40403,#40404,#40405,#40406,#40407,#40408,#40409,
#40410,#40411,#40412,#40413,#40414,#40415,#40416,#40417,#40418,#40419,#40420,
#40421,#40422,#40423,#40424,#40425,#40426,#40427,#40428,#40429,#40430,#40431,
#40432,#40433,#40434,#40435,#40436,#40437,#40438,#40439,#40440,#40441,#40442,
#40443,#40444,#40445,#40446,#40447,#40448,#40449,#40450,#40451,#40452,#40453,
#40454,#40455,#40456,#40457,#40458,#40459,#40460,#40461,#40462,#40463,#40464,
#40465,#40466,#40467,#40468,#40469,#40470,#40471,#40472,#40473,#40474,#40475,
#40476,#40477,#40478,#40479,#40480,#40481,#40482,#40483,#40484,#40485),
 .UNSPECIFIED.,.F.,.F.,(4,3,3,3,3,3,3,3,3,3,3,3,3,3,3,3,3,3,3,3,3,3,3,3,
3,3,3,3,3,3,3,3,3,3,4),(-0.972375876542414,-0.931565253728255,-0.890231005347033,
-0.869571408761885,-0.861266125665987,-0.819404433385386,-0.781321836236662,
-0.759040374121689,-0.752934683192443,-0.743239239087938,-0.701695078724687,
-0.659497058703992,-0.617009387497169,-0.589480672868744,-0.57644702705794,
-0.5714452780933,-0.528325351620324,-0.506894528983471,-0.464054318866617,
-0.420876860304666,-0.401240281040809,-0.388666227231065,-0.383537192824514,
-0.339939758883143,-0.295998103578765,-0.263784226193809,-0.219954566467475,
-0.204809517925579,-0.197308554950036,-0.192241015625869,-0.147699202975487,
-0.103111401264591,-0.0585925831444644,-0.0140737650243382,0.),
 .UNSPECIFIED.);
#1021=B_SPLINE_CURVE_WITH_KNOTS('',3,(#40486,#40487,#40488,#40489,#40490,
#40491,#40492,#40493,#40494,#40495,#40496,#40497,#40498,#40499,#40500,#40501,
#40502,#40503,#40504,#40505,#40506,#40507,#40508,#40509,#40510,#40511,#40512,
#40513,#40514,#40515,#40516,#40517,#40518,#40519,#40520,#40521,#40522,#40523,
#40524,#40525,#40526,#40527,#40528,#40529,#40530,#40531,#40532,#40533,#40534,
#40535,#40536,#40537,#40538,#40539,#40540,#40541,#40542,#40543,#40544,#40545,
#40546,#40547,#40548,#40549,#40550,#40551,#40552,#40553,#40554,#40555,#40556,
#40557,#40558,#40559,#40560,#40561,#40562,#40563,#40564,#40565,#40566,#40567,
#40568,#40569,#40570,#40571,#40572,#40573,#40574,#40575,#40576,#40577,#40578,
#40579,#40580,#40581,#40582,#40583,#40584,#40585,#40586,#40587,#40588),
 .UNSPECIFIED.,.F.,.F.,(4,3,3,3,3,3,3,3,3,3,3,3,3,3,3,3,3,3,3,3,3,3,3,3,
3,3,3,3,3,3,3,3,3,3,4),(-0.97000658757332,-0.925493326456513,-0.880835987444213,
-0.86024842639854,-0.852333874766883,-0.808142692209155,-0.764580356539862,
-0.742334794451242,-0.733010188832428,-0.721018020870569,-0.677646574841948,
-0.633950360266973,-0.590648734368262,-0.562539792613221,-0.550153753024242,
-0.542978093928587,-0.50009796533363,-0.478212967348099,-0.435235450336473,
-0.392367497022972,-0.373572235159268,-0.361228651726056,-0.355614322341834,
-0.313378921971217,-0.271427075980555,-0.242005402113342,-0.199831951142943,
-0.186315085816715,-0.179649707786883,-0.174232916759018,-0.132703725702247,
-0.0912075908119877,-0.0504161836307489,-0.0125558726020182,0.),
 .UNSPECIFIED.);
#1022=B_SPLINE_CURVE_WITH_KNOTS('',3,(#40590,#40591,#40592,#40593,#40594,
#40595,#40596,#40597,#40598,#40599,#40600,#40601,#40602,#40603,#40604,#40605,
#40606),.UNSPECIFIED.,.F.,.F.,(4,1,1,1,1,1,1,1,1,1,1,1,1,1,4),(15.707963267949,
15.8363896981257,16.3335648026029,16.8307399070801,17.3279150115573,17.8250901160345,
18.3222652205117,18.8194403249889,19.3166154294662,19.8137905339434,20.3109656384206,
20.8081407428978,21.305315847375,21.8024909518522,21.9911485751286),
 .UNSPECIFIED.);
#1023=B_SPLINE_CURVE_WITH_KNOTS('',3,(#40607,#40608,#40609,#40610,#40611,
#40612,#40613,#40614,#40615,#40616,#40617,#40618,#40619,#40620,#40621,#40622,
#40623),.UNSPECIFIED.,.F.,.F.,(4,1,1,1,1,1,1,1,1,1,1,1,1,1,4),(15.707963267949,
15.8904695802126,16.3876446846898,16.884819789167,17.3819948936443,17.8791699981215,
18.3763451025987,18.8735202070759,19.3706953115531,19.8678704160303,20.3650455205075,
20.8622206249848,21.359395729462,21.8565708339392,21.9911485751286),
 .UNSPECIFIED.);
#1024=B_SPLINE_CURVE_WITH_KNOTS('',3,(#41916,#41917,#41918,#41919,#41920,
#41921,#41922,#41923,#41924,#41925,#41926,#41927,#41928,#41929,#41930,#41931,
#41932,#41933,#41934,#41935,#41936,#41937,#41938,#41939,#41940,#41941,#41942,
#41943,#41944,#41945,#41946,#41947,#41948,#41949,#41950,#41951,#41952,#41953,
#41954,#41955,#41956,#41957,#41958,#41959,#41960,#41961,#41962,#41963,#41964,
#41965,#41966,#41967,#41968,#41969,#41970,#41971,#41972,#41973,#41974,#41975,
#41976,#41977,#41978,#41979,#41980,#41981,#41982,#41983,#41984,#41985,#41986,
#41987,#41988,#41989,#41990,#41991,#41992,#41993,#41994,#41995,#41996,#41997,
#41998,#41999,#42000,#42001,#42002,#42003,#42004,#42005,#42006,#42007,#42008,
#42009,#42010,#42011,#42012,#42013,#42014,#42015,#42016,#42017,#42018,#42019,
#42020,#42021),.UNSPECIFIED.,.F.,.F.,(4,3,3,3,3,3,3,3,3,3,3,3,3,3,3,3,3,
3,3,3,3,3,3,3,3,3,3,3,3,3,3,3,3,3,3,4),(0.,0.0404156030320338,0.0815364170314856,
0.123099442202208,0.164471164259153,0.177417333177223,0.182894508577368,
0.225046885757466,0.229033692090525,0.270767557602402,0.312945697761686,
0.350924838148176,0.357993918766748,0.363846074008531,0.406502560546029,
0.449493818503337,0.464862259307647,0.507689818261392,0.532644888553053,
0.54674918267878,0.552366866895522,0.595682545020243,0.639338821245014,
0.682868010841828,0.707330380594682,0.725816624679753,0.736955855775304,
0.74358314378864,0.787317407834192,0.829479796072424,0.846856648451819,
0.854114186312316,0.898699022066203,0.94326334774114,0.955966960787121,
0.97000658757331),.UNSPECIFIED.);
#1025=B_SPLINE_CURVE_WITH_KNOTS('',3,(#42022,#42023,#42024,#42025,#42026,
#42027,#42028,#42029,#42030,#42031,#42032,#42033,#42034,#42035,#42036,#42037,
#42038,#42039,#42040,#42041,#42042,#42043,#42044,#42045,#42046,#42047,#42048,
#42049,#42050,#42051,#42052,#42053,#42054,#42055,#42056,#42057,#42058,#42059,
#42060,#42061,#42062,#42063,#42064),.UNSPECIFIED.,.F.,.F.,(4,3,3,3,3,3,
3,3,3,3,3,3,3,3,4),(-10.1321597128207,-9.94350208954429,-9.44632698506708,
-8.94915188058987,-8.45197677611265,-7.95480167163544,-7.45762656715822,
-6.96045146268101,-6.46327635820379,-5.96610125372657,-5.46892614924936,
-4.97175104477214,-4.47457594029493,-3.97740083581771,-3.848974405641),
 .UNSPECIFIED.);
#1026=B_SPLINE_CURVE_WITH_KNOTS('',3,(#43357,#43358,#43359,#43360,#43361,
#43362,#43363,#43364,#43365,#43366,#43367,#43368,#43369,#43370,#43371,#43372,
#43373,#43374,#43375,#43376,#43377,#43378,#43379,#43380,#43381,#43382,#43383,
#43384,#43385,#43386,#43387,#43388,#43389,#43390,#43391,#43392,#43393,#43394,
#43395,#43396),.UNSPECIFIED.,.F.,.F.,(4,3,3,3,3,3,3,3,3,3,3,3,3,4),(7.59220430834767,
7.95480167163543,8.45197677611264,8.94915188058986,9.44632698506707,9.94350208954429,
10.4406771940215,10.9378522984987,11.4350274029759,11.9322025074531,12.4293776119304,
12.9265527164076,13.4237278208848,13.8753896155273),.UNSPECIFIED.);
#1027=B_SPLINE_CURVE_WITH_KNOTS('',3,(#43397,#43398,#43399,#43400,#43401,
#43402,#43403,#43404,#43405,#43406,#43407,#43408,#43409,#43410,#43411,#43412,
#43413,#43414,#43415,#43416,#43417,#43418,#43419,#43420,#43421,#43422,#43423,
#43424,#43425,#43426,#43427,#43428,#43429,#43430,#43431,#43432,#43433,#43434,
#43435,#43436,#43437,#43438,#43439,#43440,#43441,#43442,#43443,#43444,#43445,
#43446,#43447,#43448,#43449,#43450,#43451,#43452,#43453,#43454,#43455,#43456,
#43457,#43458,#43459,#43460,#43461,#43462,#43463,#43464,#43465,#43466,#43467,
#43468,#43469,#43470,#43471,#43472,#43473,#43474,#43475,#43476,#43477,#43478,
#43479,#43480,#43481,#43482,#43483,#43484,#43485,#43486,#43487,#43488,#43489,
#43490,#43491,#43492,#43493,#43494,#43495,#43496,#43497,#43498,#43499,#43500,
#43501,#43502),.UNSPECIFIED.,.F.,.F.,(4,3,3,3,3,3,3,3,3,3,3,3,3,3,3,3,3,
3,3,3,3,3,3,3,3,3,3,3,3,3,3,3,3,3,3,4),(0.,0.044150773052086,0.0887487507111273,
0.133148741969068,0.177019043965151,0.193023436662248,0.199907412815446,
0.24373234733986,0.250033573379215,0.293906609053928,0.337808296166161,
0.376734021006827,0.385567082155686,0.391401994113249,0.434581851246655,
0.477513379513922,0.493511195528826,0.53671130462677,0.560905212030567,
0.574207000071321,0.579201605029167,0.62168463125547,0.664125603281933,
0.705919109414855,0.730262563857148,0.748325604460628,0.757394747707568,
0.762943677116111,0.804834492856293,0.843575066915537,0.859283154994003,
0.866889043776386,0.908311110283104,0.949189929713081,0.959796789093269,
0.972375876542504),.UNSPECIFIED.);
#1715=CYLINDRICAL_SURFACE('',#14742,4.51775);
#1716=CYLINDRICAL_SURFACE('',#14746,4.51775);
#1717=CYLINDRICAL_SURFACE('',#14747,4.51775);
#1718=CYLINDRICAL_SURFACE('',#14748,4.51775);
#1719=CYLINDRICAL_SURFACE('',#14749,4.51775);
#1720=CYLINDRICAL_SURFACE('',#14750,4.51775);
#1721=CYLINDRICAL_SURFACE('',#14751,4.51775);
#1722=CYLINDRICAL_SURFACE('',#14752,4.51775);
#1723=CYLINDRICAL_SURFACE('',#14753,4.51775);
#1724=CYLINDRICAL_SURFACE('',#14754,4.51775);
#1725=CYLINDRICAL_SURFACE('',#14755,4.51775);
#1726=CYLINDRICAL_SURFACE('',#14756,4.51775);
#1727=CYLINDRICAL_SURFACE('',#14757,4.51775);
#1728=CYLINDRICAL_SURFACE('',#14758,4.51775);
#1729=CYLINDRICAL_SURFACE('',#14759,4.51775);
#1730=CYLINDRICAL_SURFACE('',#14760,4.51775);
#1731=CYLINDRICAL_SURFACE('',#14761,4.51775);
#1732=CYLINDRICAL_SURFACE('',#14762,4.51775);
#1733=CYLINDRICAL_SURFACE('',#14763,4.51775);
#1734=CYLINDRICAL_SURFACE('',#14764,4.51775);
#1735=CYLINDRICAL_SURFACE('',#14765,4.51775);
#1736=CYLINDRICAL_SURFACE('',#14766,4.51775);
#1737=CYLINDRICAL_SURFACE('',#14767,4.51775);
#1738=CYLINDRICAL_SURFACE('',#14768,4.51775);
#1739=CYLINDRICAL_SURFACE('',#14769,4.51775);
#1740=CYLINDRICAL_SURFACE('',#14771,5.0736);
#1741=CYLINDRICAL_SURFACE('',#14773,5.0736);
#1742=CYLINDRICAL_SURFACE('',#14774,5.0736);
#1743=CYLINDRICAL_SURFACE('',#14775,5.0736);
#1744=CYLINDRICAL_SURFACE('',#14776,5.0736);
#1745=CYLINDRICAL_SURFACE('',#14777,5.0736);
#1746=CYLINDRICAL_SURFACE('',#14778,5.0736);
#1747=CYLINDRICAL_SURFACE('',#14779,5.0736);
#1748=CYLINDRICAL_SURFACE('',#14780,5.0736);
#1749=CYLINDRICAL_SURFACE('',#14781,5.0736);
#1750=CYLINDRICAL_SURFACE('',#14782,5.0736);
#1751=CYLINDRICAL_SURFACE('',#14783,5.0736);
#1752=CYLINDRICAL_SURFACE('',#14784,5.0736);
#1753=CYLINDRICAL_SURFACE('',#14785,5.0736);
#1754=CYLINDRICAL_SURFACE('',#14786,5.0736);
#1755=CYLINDRICAL_SURFACE('',#14787,5.0736);
#1756=CYLINDRICAL_SURFACE('',#14788,5.0736);
#1757=CYLINDRICAL_SURFACE('',#14789,5.0736);
#1758=CYLINDRICAL_SURFACE('',#14790,5.0736);
#1759=CYLINDRICAL_SURFACE('',#14791,5.0736);
#1760=CYLINDRICAL_SURFACE('',#14792,5.0736);
#1761=CYLINDRICAL_SURFACE('',#14793,5.0736);
#1762=CYLINDRICAL_SURFACE('',#14794,5.0736);
#1763=CYLINDRICAL_SURFACE('',#14795,5.0736);
#1764=CYLINDRICAL_SURFACE('',#14796,5.0736);
#1765=CYLINDRICAL_SURFACE('',#14798,4.51775);
#1766=CYLINDRICAL_SURFACE('',#14802,4.51775);
#1767=CYLINDRICAL_SURFACE('',#14803,4.51775);
#1768=CYLINDRICAL_SURFACE('',#14804,4.51775);
#1769=CYLINDRICAL_SURFACE('',#14805,4.51775);
#1770=CYLINDRICAL_SURFACE('',#14806,4.51775);
#1771=CYLINDRICAL_SURFACE('',#14807,4.51775);
#1772=CYLINDRICAL_SURFACE('',#14808,4.51775);
#1773=CYLINDRICAL_SURFACE('',#14809,4.51775);
#1774=CYLINDRICAL_SURFACE('',#14810,4.51775);
#1775=CYLINDRICAL_SURFACE('',#14811,4.51775);
#1776=CYLINDRICAL_SURFACE('',#14812,4.51775);
#1777=CYLINDRICAL_SURFACE('',#14813,4.51775);
#1778=CYLINDRICAL_SURFACE('',#14814,4.51775);
#1779=CYLINDRICAL_SURFACE('',#14815,4.51775);
#1780=CYLINDRICAL_SURFACE('',#14816,4.51775);
#1781=CYLINDRICAL_SURFACE('',#14817,4.51775);
#1782=CYLINDRICAL_SURFACE('',#14818,4.51775);
#1783=CYLINDRICAL_SURFACE('',#14819,4.51775);
#1784=CYLINDRICAL_SURFACE('',#14820,4.51775);
#1785=CYLINDRICAL_SURFACE('',#14821,4.51775);
#1786=CYLINDRICAL_SURFACE('',#14822,4.51775);
#1787=CYLINDRICAL_SURFACE('',#14823,4.51775);
#1788=CYLINDRICAL_SURFACE('',#14824,4.51775);
#1789=CYLINDRICAL_SURFACE('',#14825,4.51775);
#1790=CYLINDRICAL_SURFACE('',#14826,4.51775);
#1791=CYLINDRICAL_SURFACE('',#14827,4.51775);
#1792=CYLINDRICAL_SURFACE('',#14828,4.51775);
#1793=CYLINDRICAL_SURFACE('',#14829,4.51775);
#1794=CYLINDRICAL_SURFACE('',#14830,4.51775);
#1795=CYLINDRICAL_SURFACE('',#14831,4.51775);
#1796=CYLINDRICAL_SURFACE('',#14832,4.51775);
#1797=CYLINDRICAL_SURFACE('',#14833,4.51775);
#1798=CYLINDRICAL_SURFACE('',#14834,4.51775);
#1799=CYLINDRICAL_SURFACE('',#14835,4.51775);
#1800=CYLINDRICAL_SURFACE('',#14836,4.51775);
#1801=CYLINDRICAL_SURFACE('',#14837,4.51775);
#1802=CYLINDRICAL_SURFACE('',#14838,4.51775);
#1803=CYLINDRICAL_SURFACE('',#14839,4.51775);
#1804=CYLINDRICAL_SURFACE('',#14840,4.51775);
#1805=CYLINDRICAL_SURFACE('',#14842,5.0736);
#1806=CYLINDRICAL_SURFACE('',#14844,5.0736);
#1807=CYLINDRICAL_SURFACE('',#14845,5.0736);
#1808=CYLINDRICAL_SURFACE('',#14846,5.0736);
#1809=CYLINDRICAL_SURFACE('',#14847,5.0736);
#1810=CYLINDRICAL_SURFACE('',#14848,5.0736);
#1811=CYLINDRICAL_SURFACE('',#14849,5.0736);
#1812=CYLINDRICAL_SURFACE('',#14850,5.0736);
#1813=CYLINDRICAL_SURFACE('',#14851,5.0736);
#1814=CYLINDRICAL_SURFACE('',#14852,5.0736);
#1815=CYLINDRICAL_SURFACE('',#14853,5.0736);
#1816=CYLINDRICAL_SURFACE('',#14854,5.0736);
#1817=CYLINDRICAL_SURFACE('',#14855,5.0736);
#1818=CYLINDRICAL_SURFACE('',#14856,5.0736);
#1819=CYLINDRICAL_SURFACE('',#14857,5.0736);
#1820=CYLINDRICAL_SURFACE('',#14858,5.0736);
#1821=CYLINDRICAL_SURFACE('',#14859,5.0736);
#1822=CYLINDRICAL_SURFACE('',#14860,5.0736);
#1823=CYLINDRICAL_SURFACE('',#14861,5.0736);
#1824=CYLINDRICAL_SURFACE('',#14862,5.0736);
#1825=CYLINDRICAL_SURFACE('',#14863,5.0736);
#1826=CYLINDRICAL_SURFACE('',#14864,5.0736);
#1827=CYLINDRICAL_SURFACE('',#14865,5.0736);
#1828=CYLINDRICAL_SURFACE('',#14866,5.0736);
#1829=CYLINDRICAL_SURFACE('',#14867,5.0736);
#1830=CYLINDRICAL_SURFACE('',#14868,5.0736);
#1831=CYLINDRICAL_SURFACE('',#14869,5.0736);
#1832=CYLINDRICAL_SURFACE('',#14870,5.0736);
#1833=CYLINDRICAL_SURFACE('',#14871,5.0736);
#1834=CYLINDRICAL_SURFACE('',#14872,5.0736);
#1835=CYLINDRICAL_SURFACE('',#14873,5.0736);
#1836=CYLINDRICAL_SURFACE('',#14874,5.0736);
#1837=CYLINDRICAL_SURFACE('',#14875,5.0736);
#1838=CYLINDRICAL_SURFACE('',#14876,5.0736);
#1839=CYLINDRICAL_SURFACE('',#14877,5.0736);
#1840=CYLINDRICAL_SURFACE('',#14878,5.0736);
#1841=CYLINDRICAL_SURFACE('',#14879,5.0736);
#1842=CYLINDRICAL_SURFACE('',#14880,5.0736);
#1843=CYLINDRICAL_SURFACE('',#14881,5.0736);
#1844=CYLINDRICAL_SURFACE('',#14882,5.0736);
#1845=CYLINDRICAL_SURFACE('',#14885,5.0736);
#1846=CYLINDRICAL_SURFACE('',#14886,4.51775);
#1847=CYLINDRICAL_SURFACE('',#14890,5.0736);
#1848=CYLINDRICAL_SURFACE('',#14891,4.51775);
#1849=CYLINDRICAL_SURFACE('',#14894,1.);
#1850=CYLINDRICAL_SURFACE('',#14938,1.);
#1851=CYLINDRICAL_SURFACE('',#14941,1.);
#1852=CYLINDRICAL_SURFACE('',#14944,1.);
#1853=CYLINDRICAL_SURFACE('',#14947,1.);
#1854=CYLINDRICAL_SURFACE('',#14950,1.);
#1855=CYLINDRICAL_SURFACE('',#14952,1.);
#1856=CYLINDRICAL_SURFACE('',#14955,1.);
#1857=CYLINDRICAL_SURFACE('',#14957,1.);
#1858=CYLINDRICAL_SURFACE('',#14960,1.);
#1859=CYLINDRICAL_SURFACE('',#14962,1.);
#1860=CYLINDRICAL_SURFACE('',#14965,1.);
#1861=CYLINDRICAL_SURFACE('',#14968,1.);
#1862=CYLINDRICAL_SURFACE('',#14971,1.);
#1863=CYLINDRICAL_SURFACE('',#14974,1.);
#1864=CYLINDRICAL_SURFACE('',#14976,1.);
#1865=CYLINDRICAL_SURFACE('',#14979,1.);
#1866=CYLINDRICAL_SURFACE('',#14981,1.);
#1867=CYLINDRICAL_SURFACE('',#14984,1.);
#1868=CYLINDRICAL_SURFACE('',#14986,1.);
#1869=CYLINDRICAL_SURFACE('',#14989,1.);
#1870=CYLINDRICAL_SURFACE('',#14992,1.);
#1871=CYLINDRICAL_SURFACE('',#14995,1.);
#1872=CYLINDRICAL_SURFACE('',#14998,1.);
#1873=CYLINDRICAL_SURFACE('',#15000,1.);
#1874=CYLINDRICAL_SURFACE('',#15003,1.);
#1875=CYLINDRICAL_SURFACE('',#15005,1.);
#1876=CYLINDRICAL_SURFACE('',#15008,1.);
#1877=CYLINDRICAL_SURFACE('',#15010,1.);
#1878=CYLINDRICAL_SURFACE('',#15013,1.);
#1879=CYLINDRICAL_SURFACE('',#15016,1.);
#1880=CYLINDRICAL_SURFACE('',#15019,1.);
#1881=CYLINDRICAL_SURFACE('',#15022,1.);
#1882=CYLINDRICAL_SURFACE('',#15024,1.);
#1883=CYLINDRICAL_SURFACE('',#15027,1.);
#1884=CYLINDRICAL_SURFACE('',#15029,1.);
#1885=CYLINDRICAL_SURFACE('',#15031,3.);
#1886=CYLINDRICAL_SURFACE('',#15033,3.);
#1887=CYLINDRICAL_SURFACE('',#15035,4.);
#1888=CYLINDRICAL_SURFACE('',#15036,3.);
#1889=CYLINDRICAL_SURFACE('',#15038,3.);
#2181=SHAPE_REPRESENTATION_RELATIONSHIP('SRR','None',#63866,#2197);
#2197=ADVANCED_BREP_SHAPE_REPRESENTATION('',(#2229),#63744);
#2213=STYLED_ITEM('',(#63958),#2229);
#2229=MANIFOLD_SOLID_BREP('Aluminum slotted profile',#14314);
#2256=FACE_BOUND('',#3389,.T.);
#2257=FACE_BOUND('',#3396,.T.);
#2258=FACE_BOUND('',#3400,.T.);
#2259=FACE_BOUND('',#3401,.T.);
#2260=FACE_BOUND('',#3402,.T.);
#2261=FACE_BOUND('',#3403,.T.);
#2262=FACE_BOUND('',#3404,.T.);
#2263=FACE_BOUND('',#3481,.T.);
#2264=FACE_BOUND('',#3482,.T.);
#2265=FACE_BOUND('',#3483,.T.);
#2266=FACE_BOUND('',#3484,.T.);
#2267=FACE_BOUND('',#3485,.T.);
#2477=FACE_OUTER_BOUND('',#3253,.T.);
#2478=FACE_OUTER_BOUND('',#3254,.T.);
#2479=FACE_OUTER_BOUND('',#3255,.T.);
#2480=FACE_OUTER_BOUND('',#3256,.T.);
#2481=FACE_OUTER_BOUND('',#3257,.T.);
#2482=FACE_OUTER_BOUND('',#3258,.T.);
#2483=FACE_OUTER_BOUND('',#3259,.T.);
#2484=FACE_OUTER_BOUND('',#3260,.T.);
#2485=FACE_OUTER_BOUND('',#3261,.T.);
#2486=FACE_OUTER_BOUND('',#3262,.T.);
#2487=FACE_OUTER_BOUND('',#3263,.T.);
#2488=FACE_OUTER_BOUND('',#3264,.T.);
#2489=FACE_OUTER_BOUND('',#3265,.T.);
#2490=FACE_OUTER_BOUND('',#3266,.T.);
#2491=FACE_OUTER_BOUND('',#3267,.T.);
#2492=FACE_OUTER_BOUND('',#3268,.T.);
#2493=FACE_OUTER_BOUND('',#3269,.T.);
#2494=FACE_OUTER_BOUND('',#3270,.T.);
#2495=FACE_OUTER_BOUND('',#3271,.T.);
#2496=FACE_OUTER_BOUND('',#3272,.T.);
#2497=FACE_OUTER_BOUND('',#3273,.T.);
#2498=FACE_OUTER_BOUND('',#3274,.T.);
#2499=FACE_OUTER_BOUND('',#3275,.T.);
#2500=FACE_OUTER_BOUND('',#3276,.T.);
#2501=FACE_OUTER_BOUND('',#3277,.T.);
#2502=FACE_OUTER_BOUND('',#3278,.T.);
#2503=FACE_OUTER_BOUND('',#3279,.T.);
#2504=FACE_OUTER_BOUND('',#3280,.T.);
#2505=FACE_OUTER_BOUND('',#3281,.T.);
#2506=FACE_OUTER_BOUND('',#3282,.T.);
#2507=FACE_OUTER_BOUND('',#3283,.T.);
#2508=FACE_OUTER_BOUND('',#3284,.T.);
#2509=FACE_OUTER_BOUND('',#3285,.T.);
#2510=FACE_OUTER_BOUND('',#3286,.T.);
#2511=FACE_OUTER_BOUND('',#3287,.T.);
#2512=FACE_OUTER_BOUND('',#3288,.T.);
#2513=FACE_OUTER_BOUND('',#3289,.T.);
#2514=FACE_OUTER_BOUND('',#3290,.T.);
#2515=FACE_OUTER_BOUND('',#3291,.T.);
#2516=FACE_OUTER_BOUND('',#3292,.T.);
#2517=FACE_OUTER_BOUND('',#3293,.T.);
#2518=FACE_OUTER_BOUND('',#3294,.T.);
#2519=FACE_OUTER_BOUND('',#3295,.T.);
#2520=FACE_OUTER_BOUND('',#3296,.T.);
#2521=FACE_OUTER_BOUND('',#3297,.T.);
#2522=FACE_OUTER_BOUND('',#3298,.T.);
#2523=FACE_OUTER_BOUND('',#3299,.T.);
#2524=FACE_OUTER_BOUND('',#3300,.T.);
#2525=FACE_OUTER_BOUND('',#3301,.T.);
#2526=FACE_OUTER_BOUND('',#3302,.T.);
#2527=FACE_OUTER_BOUND('',#3303,.T.);
#2528=FACE_OUTER_BOUND('',#3304,.T.);
#2529=FACE_OUTER_BOUND('',#3305,.T.);
#2530=FACE_OUTER_BOUND('',#3306,.T.);
#2531=FACE_OUTER_BOUND('',#3307,.T.);
#2532=FACE_OUTER_BOUND('',#3308,.T.);
#2533=FACE_OUTER_BOUND('',#3309,.T.);
#2534=FACE_OUTER_BOUND('',#3310,.T.);
#2535=FACE_OUTER_BOUND('',#3311,.T.);
#2536=FACE_OUTER_BOUND('',#3312,.T.);
#2537=FACE_OUTER_BOUND('',#3313,.T.);
#2538=FACE_OUTER_BOUND('',#3314,.T.);
#2539=FACE_OUTER_BOUND('',#3315,.T.);
#2540=FACE_OUTER_BOUND('',#3316,.T.);
#2541=FACE_OUTER_BOUND('',#3317,.T.);
#2542=FACE_OUTER_BOUND('',#3318,.T.);
#2543=FACE_OUTER_BOUND('',#3319,.T.);
#2544=FACE_OUTER_BOUND('',#3320,.T.);
#2545=FACE_OUTER_BOUND('',#3321,.T.);
#2546=FACE_OUTER_BOUND('',#3322,.T.);
#2547=FACE_OUTER_BOUND('',#3323,.T.);
#2548=FACE_OUTER_BOUND('',#3324,.T.);
#2549=FACE_OUTER_BOUND('',#3325,.T.);
#2550=FACE_OUTER_BOUND('',#3326,.T.);
#2551=FACE_OUTER_BOUND('',#3327,.T.);
#2552=FACE_OUTER_BOUND('',#3328,.T.);
#2553=FACE_OUTER_BOUND('',#3329,.T.);
#2554=FACE_OUTER_BOUND('',#3330,.T.);
#2555=FACE_OUTER_BOUND('',#3331,.T.);
#2556=FACE_OUTER_BOUND('',#3332,.T.);
#2557=FACE_OUTER_BOUND('',#3333,.T.);
#2558=FACE_OUTER_BOUND('',#3334,.T.);
#2559=FACE_OUTER_BOUND('',#3335,.T.);
#2560=FACE_OUTER_BOUND('',#3336,.T.);
#2561=FACE_OUTER_BOUND('',#3337,.T.);
#2562=FACE_OUTER_BOUND('',#3338,.T.);
#2563=FACE_OUTER_BOUND('',#3339,.T.);
#2564=FACE_OUTER_BOUND('',#3340,.T.);
#2565=FACE_OUTER_BOUND('',#3341,.T.);
#2566=FACE_OUTER_BOUND('',#3342,.T.);
#2567=FACE_OUTER_BOUND('',#3343,.T.);
#2568=FACE_OUTER_BOUND('',#3344,.T.);
#2569=FACE_OUTER_BOUND('',#3345,.T.);
#2570=FACE_OUTER_BOUND('',#3346,.T.);
#2571=FACE_OUTER_BOUND('',#3347,.T.);
#2572=FACE_OUTER_BOUND('',#3348,.T.);
#2573=FACE_OUTER_BOUND('',#3349,.T.);
#2574=FACE_OUTER_BOUND('',#3350,.T.);
#2575=FACE_OUTER_BOUND('',#3351,.T.);
#2576=FACE_OUTER_BOUND('',#3352,.T.);
#2577=FACE_OUTER_BOUND('',#3353,.T.);
#2578=FACE_OUTER_BOUND('',#3354,.T.);
#2579=FACE_OUTER_BOUND('',#3355,.T.);
#2580=FACE_OUTER_BOUND('',#3356,.T.);
#2581=FACE_OUTER_BOUND('',#3357,.T.);
#2582=FACE_OUTER_BOUND('',#3358,.T.);
#2583=FACE_OUTER_BOUND('',#3359,.T.);
#2584=FACE_OUTER_BOUND('',#3360,.T.);
#2585=FACE_OUTER_BOUND('',#3361,.T.);
#2586=FACE_OUTER_BOUND('',#3362,.T.);
#2587=FACE_OUTER_BOUND('',#3363,.T.);
#2588=FACE_OUTER_BOUND('',#3364,.T.);
#2589=FACE_OUTER_BOUND('',#3365,.T.);
#2590=FACE_OUTER_BOUND('',#3366,.T.);
#2591=FACE_OUTER_BOUND('',#3367,.T.);
#2592=FACE_OUTER_BOUND('',#3368,.T.);
#2593=FACE_OUTER_BOUND('',#3369,.T.);
#2594=FACE_OUTER_BOUND('',#3370,.T.);
#2595=FACE_OUTER_BOUND('',#3371,.T.);
#2596=FACE_OUTER_BOUND('',#3372,.T.);
#2597=FACE_OUTER_BOUND('',#3373,.T.);
#2598=FACE_OUTER_BOUND('',#3374,.T.);
#2599=FACE_OUTER_BOUND('',#3375,.T.);
#2600=FACE_OUTER_BOUND('',#3376,.T.);
#2601=FACE_OUTER_BOUND('',#3377,.T.);
#2602=FACE_OUTER_BOUND('',#3378,.T.);
#2603=FACE_OUTER_BOUND('',#3379,.T.);
#2604=FACE_OUTER_BOUND('',#3380,.T.);
#2605=FACE_OUTER_BOUND('',#3381,.T.);
#2606=FACE_OUTER_BOUND('',#3382,.T.);
#2607=FACE_OUTER_BOUND('',#3383,.T.);
#2608=FACE_OUTER_BOUND('',#3384,.T.);
#2609=FACE_OUTER_BOUND('',#3385,.T.);
#2610=FACE_OUTER_BOUND('',#3386,.T.);
#2611=FACE_OUTER_BOUND('',#3387,.T.);
#2612=FACE_OUTER_BOUND('',#3388,.T.);
#2613=FACE_OUTER_BOUND('',#3390,.T.);
#2614=FACE_OUTER_BOUND('',#3391,.T.);
#2615=FACE_OUTER_BOUND('',#3392,.T.);
#2616=FACE_OUTER_BOUND('',#3393,.T.);
#2617=FACE_OUTER_BOUND('',#3394,.T.);
#2618=FACE_OUTER_BOUND('',#3395,.T.);
#2619=FACE_OUTER_BOUND('',#3397,.T.);
#2620=FACE_OUTER_BOUND('',#3398,.T.);
#2621=FACE_OUTER_BOUND('',#3399,.T.);
#2622=FACE_OUTER_BOUND('',#3405,.T.);
#2623=FACE_OUTER_BOUND('',#3406,.T.);
#2624=FACE_OUTER_BOUND('',#3407,.T.);
#2625=FACE_OUTER_BOUND('',#3408,.T.);
#2626=FACE_OUTER_BOUND('',#3409,.T.);
#2627=FACE_OUTER_BOUND('',#3410,.T.);
#2628=FACE_OUTER_BOUND('',#3411,.T.);
#2629=FACE_OUTER_BOUND('',#3412,.T.);
#2630=FACE_OUTER_BOUND('',#3413,.T.);
#2631=FACE_OUTER_BOUND('',#3414,.T.);
#2632=FACE_OUTER_BOUND('',#3415,.T.);
#2633=FACE_OUTER_BOUND('',#3416,.T.);
#2634=FACE_OUTER_BOUND('',#3417,.T.);
#2635=FACE_OUTER_BOUND('',#3418,.T.);
#2636=FACE_OUTER_BOUND('',#3419,.T.);
#2637=FACE_OUTER_BOUND('',#3420,.T.);
#2638=FACE_OUTER_BOUND('',#3421,.T.);
#2639=FACE_OUTER_BOUND('',#3422,.T.);
#2640=FACE_OUTER_BOUND('',#3423,.T.);
#2641=FACE_OUTER_BOUND('',#3424,.T.);
#2642=FACE_OUTER_BOUND('',#3425,.T.);
#2643=FACE_OUTER_BOUND('',#3426,.T.);
#2644=FACE_OUTER_BOUND('',#3427,.T.);
#2645=FACE_OUTER_BOUND('',#3428,.T.);
#2646=FACE_OUTER_BOUND('',#3429,.T.);
#2647=FACE_OUTER_BOUND('',#3430,.T.);
#2648=FACE_OUTER_BOUND('',#3431,.T.);
#2649=FACE_OUTER_BOUND('',#3432,.T.);
#2650=FACE_OUTER_BOUND('',#3433,.T.);
#2651=FACE_OUTER_BOUND('',#3434,.T.);
#2652=FACE_OUTER_BOUND('',#3435,.T.);
#2653=FACE_OUTER_BOUND('',#3436,.T.);
#2654=FACE_OUTER_BOUND('',#3437,.T.);
#2655=FACE_OUTER_BOUND('',#3438,.T.);
#2656=FACE_OUTER_BOUND('',#3439,.T.);
#2657=FACE_OUTER_BOUND('',#3440,.T.);
#2658=FACE_OUTER_BOUND('',#3441,.T.);
#2659=FACE_OUTER_BOUND('',#3442,.T.);
#2660=FACE_OUTER_BOUND('',#3443,.T.);
#2661=FACE_OUTER_BOUND('',#3444,.T.);
#2662=FACE_OUTER_BOUND('',#3445,.T.);
#2663=FACE_OUTER_BOUND('',#3446,.T.);
#2664=FACE_OUTER_BOUND('',#3447,.T.);
#2665=FACE_OUTER_BOUND('',#3448,.T.);
#2666=FACE_OUTER_BOUND('',#3449,.T.);
#2667=FACE_OUTER_BOUND('',#3450,.T.);
#2668=FACE_OUTER_BOUND('',#3451,.T.);
#2669=FACE_OUTER_BOUND('',#3452,.T.);
#2670=FACE_OUTER_BOUND('',#3453,.T.);
#2671=FACE_OUTER_BOUND('',#3454,.T.);
#2672=FACE_OUTER_BOUND('',#3455,.T.);
#2673=FACE_OUTER_BOUND('',#3456,.T.);
#2674=FACE_OUTER_BOUND('',#3457,.T.);
#2675=FACE_OUTER_BOUND('',#3458,.T.);
#2676=FACE_OUTER_BOUND('',#3459,.T.);
#2677=FACE_OUTER_BOUND('',#3460,.T.);
#2678=FACE_OUTER_BOUND('',#3461,.T.);
#2679=FACE_OUTER_BOUND('',#3462,.T.);
#2680=FACE_OUTER_BOUND('',#3463,.T.);
#2681=FACE_OUTER_BOUND('',#3464,.T.);
#2682=FACE_OUTER_BOUND('',#3465,.T.);
#2683=FACE_OUTER_BOUND('',#3466,.T.);
#2684=FACE_OUTER_BOUND('',#3467,.T.);
#2685=FACE_OUTER_BOUND('',#3468,.T.);
#2686=FACE_OUTER_BOUND('',#3469,.T.);
#2687=FACE_OUTER_BOUND('',#3470,.T.);
#2688=FACE_OUTER_BOUND('',#3471,.T.);
#2689=FACE_OUTER_BOUND('',#3472,.T.);
#2690=FACE_OUTER_BOUND('',#3473,.T.);
#2691=FACE_OUTER_BOUND('',#3474,.T.);
#2692=FACE_OUTER_BOUND('',#3475,.T.);
#2693=FACE_OUTER_BOUND('',#3476,.T.);
#2694=FACE_OUTER_BOUND('',#3477,.T.);
#2695=FACE_OUTER_BOUND('',#3478,.T.);
#2696=FACE_OUTER_BOUND('',#3479,.T.);
#2697=FACE_OUTER_BOUND('',#3480,.T.);
#3253=EDGE_LOOP('',(#10099,#10100,#10101,#10102,#10103,#10104,#10105,#10106));
#3254=EDGE_LOOP('',(#10107,#10108,#10109,#10110));
#3255=EDGE_LOOP('',(#10111,#10112,#10113,#10114));
#3256=EDGE_LOOP('',(#10115,#10116,#10117,#10118));
#3257=EDGE_LOOP('',(#10119,#10120,#10121,#10122));
#3258=EDGE_LOOP('',(#10123,#10124,#10125,#10126));
#3259=EDGE_LOOP('',(#10127,#10128,#10129,#10130));
#3260=EDGE_LOOP('',(#10131,#10132,#10133,#10134));
#3261=EDGE_LOOP('',(#10135,#10136,#10137,#10138));
#3262=EDGE_LOOP('',(#10139,#10140,#10141,#10142));
#3263=EDGE_LOOP('',(#10143,#10144,#10145,#10146));
#3264=EDGE_LOOP('',(#10147,#10148,#10149,#10150));
#3265=EDGE_LOOP('',(#10151,#10152,#10153,#10154));
#3266=EDGE_LOOP('',(#10155,#10156,#10157,#10158));
#3267=EDGE_LOOP('',(#10159,#10160,#10161,#10162));
#3268=EDGE_LOOP('',(#10163,#10164,#10165,#10166));
#3269=EDGE_LOOP('',(#10167,#10168,#10169,#10170));
#3270=EDGE_LOOP('',(#10171,#10172,#10173,#10174));
#3271=EDGE_LOOP('',(#10175,#10176,#10177,#10178));
#3272=EDGE_LOOP('',(#10179,#10180,#10181,#10182));
#3273=EDGE_LOOP('',(#10183,#10184,#10185,#10186));
#3274=EDGE_LOOP('',(#10187,#10188,#10189,#10190));
#3275=EDGE_LOOP('',(#10191,#10192,#10193,#10194));
#3276=EDGE_LOOP('',(#10195,#10196,#10197,#10198));
#3277=EDGE_LOOP('',(#10199,#10200,#10201,#10202));
#3278=EDGE_LOOP('',(#10203,#10204,#10205,#10206));
#3279=EDGE_LOOP('',(#10207,#10208,#10209,#10210));
#3280=EDGE_LOOP('',(#10211,#10212,#10213,#10214));
#3281=EDGE_LOOP('',(#10215,#10216,#10217,#10218));
#3282=EDGE_LOOP('',(#10219,#10220,#10221,#10222));
#3283=EDGE_LOOP('',(#10223,#10224,#10225,#10226));
#3284=EDGE_LOOP('',(#10227,#10228,#10229,#10230));
#3285=EDGE_LOOP('',(#10231,#10232,#10233,#10234));
#3286=EDGE_LOOP('',(#10235,#10236,#10237,#10238));
#3287=EDGE_LOOP('',(#10239,#10240,#10241,#10242));
#3288=EDGE_LOOP('',(#10243,#10244,#10245,#10246));
#3289=EDGE_LOOP('',(#10247,#10248,#10249,#10250));
#3290=EDGE_LOOP('',(#10251,#10252,#10253,#10254));
#3291=EDGE_LOOP('',(#10255,#10256,#10257,#10258));
#3292=EDGE_LOOP('',(#10259,#10260,#10261,#10262));
#3293=EDGE_LOOP('',(#10263,#10264,#10265,#10266));
#3294=EDGE_LOOP('',(#10267,#10268,#10269,#10270));
#3295=EDGE_LOOP('',(#10271,#10272,#10273,#10274));
#3296=EDGE_LOOP('',(#10275,#10276,#10277,#10278));
#3297=EDGE_LOOP('',(#10279,#10280,#10281,#10282));
#3298=EDGE_LOOP('',(#10283,#10284,#10285,#10286));
#3299=EDGE_LOOP('',(#10287,#10288,#10289,#10290));
#3300=EDGE_LOOP('',(#10291,#10292,#10293,#10294));
#3301=EDGE_LOOP('',(#10295,#10296,#10297,#10298));
#3302=EDGE_LOOP('',(#10299,#10300,#10301,#10302));
#3303=EDGE_LOOP('',(#10303,#10304,#10305,#10306,#10307,#10308,#10309,#10310));
#3304=EDGE_LOOP('',(#10311,#10312,#10313,#10314));
#3305=EDGE_LOOP('',(#10315,#10316,#10317,#10318));
#3306=EDGE_LOOP('',(#10319,#10320,#10321,#10322));
#3307=EDGE_LOOP('',(#10323,#10324,#10325,#10326));
#3308=EDGE_LOOP('',(#10327,#10328,#10329,#10330));
#3309=EDGE_LOOP('',(#10331,#10332,#10333,#10334));
#3310=EDGE_LOOP('',(#10335,#10336,#10337,#10338));
#3311=EDGE_LOOP('',(#10339,#10340,#10341,#10342));
#3312=EDGE_LOOP('',(#10343,#10344,#10345,#10346));
#3313=EDGE_LOOP('',(#10347,#10348,#10349,#10350));
#3314=EDGE_LOOP('',(#10351,#10352,#10353,#10354));
#3315=EDGE_LOOP('',(#10355,#10356,#10357,#10358));
#3316=EDGE_LOOP('',(#10359,#10360,#10361,#10362));
#3317=EDGE_LOOP('',(#10363,#10364,#10365,#10366));
#3318=EDGE_LOOP('',(#10367,#10368,#10369,#10370));
#3319=EDGE_LOOP('',(#10371,#10372,#10373,#10374));
#3320=EDGE_LOOP('',(#10375,#10376,#10377,#10378));
#3321=EDGE_LOOP('',(#10379,#10380,#10381,#10382));
#3322=EDGE_LOOP('',(#10383,#10384,#10385,#10386));
#3323=EDGE_LOOP('',(#10387,#10388,#10389,#10390));
#3324=EDGE_LOOP('',(#10391,#10392,#10393,#10394));
#3325=EDGE_LOOP('',(#10395,#10396,#10397,#10398));
#3326=EDGE_LOOP('',(#10399,#10400,#10401,#10402));
#3327=EDGE_LOOP('',(#10403,#10404,#10405,#10406));
#3328=EDGE_LOOP('',(#10407,#10408,#10409,#10410));
#3329=EDGE_LOOP('',(#10411,#10412,#10413,#10414));
#3330=EDGE_LOOP('',(#10415,#10416,#10417,#10418));
#3331=EDGE_LOOP('',(#10419,#10420,#10421,#10422));
#3332=EDGE_LOOP('',(#10423,#10424,#10425,#10426));
#3333=EDGE_LOOP('',(#10427,#10428,#10429,#10430));
#3334=EDGE_LOOP('',(#10431,#10432,#10433,#10434));
#3335=EDGE_LOOP('',(#10435,#10436,#10437,#10438));
#3336=EDGE_LOOP('',(#10439,#10440,#10441,#10442));
#3337=EDGE_LOOP('',(#10443,#10444,#10445,#10446));
#3338=EDGE_LOOP('',(#10447,#10448,#10449,#10450));
#3339=EDGE_LOOP('',(#10451,#10452,#10453,#10454));
#3340=EDGE_LOOP('',(#10455,#10456,#10457,#10458));
#3341=EDGE_LOOP('',(#10459,#10460,#10461,#10462));
#3342=EDGE_LOOP('',(#10463,#10464,#10465,#10466));
#3343=EDGE_LOOP('',(#10467,#10468,#10469,#10470));
#3344=EDGE_LOOP('',(#10471,#10472,#10473,#10474));
#3345=EDGE_LOOP('',(#10475,#10476,#10477,#10478));
#3346=EDGE_LOOP('',(#10479,#10480,#10481,#10482));
#3347=EDGE_LOOP('',(#10483,#10484,#10485,#10486));
#3348=EDGE_LOOP('',(#10487,#10488,#10489,#10490));
#3349=EDGE_LOOP('',(#10491,#10492,#10493,#10494));
#3350=EDGE_LOOP('',(#10495,#10496,#10497,#10498));
#3351=EDGE_LOOP('',(#10499,#10500,#10501,#10502));
#3352=EDGE_LOOP('',(#10503,#10504,#10505,#10506));
#3353=EDGE_LOOP('',(#10507,#10508,#10509,#10510));
#3354=EDGE_LOOP('',(#10511,#10512,#10513,#10514));
#3355=EDGE_LOOP('',(#10515,#10516,#10517,#10518));
#3356=EDGE_LOOP('',(#10519,#10520,#10521,#10522));
#3357=EDGE_LOOP('',(#10523,#10524,#10525,#10526));
#3358=EDGE_LOOP('',(#10527,#10528,#10529,#10530));
#3359=EDGE_LOOP('',(#10531,#10532,#10533,#10534));
#3360=EDGE_LOOP('',(#10535,#10536,#10537,#10538));
#3361=EDGE_LOOP('',(#10539,#10540,#10541,#10542));
#3362=EDGE_LOOP('',(#10543,#10544,#10545,#10546));
#3363=EDGE_LOOP('',(#10547,#10548,#10549,#10550));
#3364=EDGE_LOOP('',(#10551,#10552,#10553,#10554));
#3365=EDGE_LOOP('',(#10555,#10556,#10557,#10558));
#3366=EDGE_LOOP('',(#10559,#10560,#10561,#10562));
#3367=EDGE_LOOP('',(#10563,#10564,#10565,#10566));
#3368=EDGE_LOOP('',(#10567,#10568,#10569,#10570));
#3369=EDGE_LOOP('',(#10571,#10572,#10573,#10574));
#3370=EDGE_LOOP('',(#10575,#10576,#10577,#10578));
#3371=EDGE_LOOP('',(#10579,#10580,#10581,#10582));
#3372=EDGE_LOOP('',(#10583,#10584,#10585,#10586));
#3373=EDGE_LOOP('',(#10587,#10588,#10589,#10590));
#3374=EDGE_LOOP('',(#10591,#10592,#10593,#10594));
#3375=EDGE_LOOP('',(#10595,#10596,#10597,#10598));
#3376=EDGE_LOOP('',(#10599,#10600,#10601,#10602));
#3377=EDGE_LOOP('',(#10603,#10604,#10605,#10606));
#3378=EDGE_LOOP('',(#10607,#10608,#10609,#10610));
#3379=EDGE_LOOP('',(#10611,#10612,#10613,#10614));
#3380=EDGE_LOOP('',(#10615,#10616,#10617,#10618));
#3381=EDGE_LOOP('',(#10619,#10620,#10621,#10622));
#3382=EDGE_LOOP('',(#10623,#10624,#10625,#10626));
#3383=EDGE_LOOP('',(#10627,#10628,#10629,#10630,#10631));
#3384=EDGE_LOOP('',(#10632,#10633,#10634,#10635));
#3385=EDGE_LOOP('',(#10636,#10637,#10638,#10639,#10640,#10641,#10642,#10643,
#10644,#10645,#10646,#10647,#10648,#10649,#10650,#10651,#10652,#10653,#10654,
#10655,#10656,#10657,#10658,#10659,#10660,#10661,#10662,#10663,#10664,#10665,
#10666,#10667,#10668,#10669,#10670,#10671,#10672,#10673,#10674,#10675,#10676,
#10677,#10678,#10679,#10680,#10681,#10682,#10683,#10684,#10685,#10686,#10687,
#10688,#10689,#10690,#10691,#10692,#10693,#10694,#10695,#10696,#10697,#10698,
#10699,#10700,#10701,#10702,#10703,#10704,#10705,#10706,#10707,#10708,#10709,
#10710,#10711,#10712,#10713,#10714,#10715,#10716,#10717,#10718,#10719));
#3386=EDGE_LOOP('',(#10720,#10721,#10722,#10723,#10724,#10725,#10726,#10727,
#10728,#10729,#10730,#10731,#10732,#10733,#10734,#10735,#10736,#10737,#10738,
#10739,#10740,#10741,#10742,#10743,#10744,#10745,#10746,#10747,#10748,#10749,
#10750,#10751,#10752,#10753,#10754,#10755,#10756,#10757,#10758,#10759,#10760,
#10761,#10762,#10763,#10764,#10765,#10766,#10767,#10768,#10769,#10770,#10771,
#10772,#10773,#10774,#10775,#10776,#10777,#10778,#10779,#10780,#10781,#10782,
#10783,#10784,#10785,#10786,#10787,#10788,#10789,#10790,#10791,#10792,#10793,
#10794,#10795,#10796,#10797,#10798,#10799,#10800,#10801,#10802,#10803));
#3387=EDGE_LOOP('',(#10804,#10805,#10806,#10807));
#3388=EDGE_LOOP('',(#10808));
#3389=EDGE_LOOP('',(#10809));
#3390=EDGE_LOOP('',(#10810,#10811,#10812,#10813,#10814));
#3391=EDGE_LOOP('',(#10815,#10816,#10817,#10818));
#3392=EDGE_LOOP('',(#10819,#10820,#10821,#10822,#10823,#10824,#10825,#10826,
#10827,#10828,#10829,#10830,#10831,#10832,#10833,#10834,#10835,#10836,#10837,
#10838,#10839,#10840,#10841,#10842,#10843,#10844,#10845,#10846,#10847,#10848,
#10849,#10850,#10851,#10852,#10853,#10854,#10855,#10856,#10857,#10858,#10859,
#10860,#10861,#10862,#10863,#10864,#10865,#10866,#10867,#10868,#10869,#10870,
#10871,#10872));
#3393=EDGE_LOOP('',(#10873,#10874,#10875,#10876,#10877,#10878,#10879,#10880,
#10881,#10882,#10883,#10884,#10885,#10886,#10887,#10888,#10889,#10890,#10891,
#10892,#10893,#10894,#10895,#10896,#10897,#10898,#10899,#10900,#10901,#10902,
#10903,#10904,#10905,#10906,#10907,#10908,#10909,#10910,#10911,#10912,#10913,
#10914,#10915,#10916,#10917,#10918,#10919,#10920,#10921,#10922,#10923,#10924,
#10925,#10926));
#3394=EDGE_LOOP('',(#10927,#10928,#10929,#10930));
#3395=EDGE_LOOP('',(#10931));
#3396=EDGE_LOOP('',(#10932));
#3397=EDGE_LOOP('',(#10933,#10934,#10935,#10936));
#3398=EDGE_LOOP('',(#10937,#10938,#10939,#10940));
#3399=EDGE_LOOP('',(#10941,#10942,#10943,#10944,#10945,#10946,#10947,#10948,
#10949,#10950,#10951,#10952,#10953,#10954,#10955,#10956,#10957,#10958,#10959,
#10960,#10961,#10962,#10963,#10964,#10965,#10966,#10967,#10968,#10969,#10970,
#10971,#10972,#10973,#10974,#10975,#10976,#10977,#10978,#10979,#10980,#10981,
#10982,#10983,#10984,#10985,#10986,#10987,#10988,#10989,#10990,#10991,#10992,
#10993,#10994,#10995,#10996,#10997,#10998,#10999,#11000,#11001,#11002,#11003,
#11004,#11005,#11006,#11007,#11008,#11009,#11010,#11011,#11012));
#3400=EDGE_LOOP('',(#11013,#11014,#11015,#11016));
#3401=EDGE_LOOP('',(#11017));
#3402=EDGE_LOOP('',(#11018));
#3403=EDGE_LOOP('',(#11019));
#3404=EDGE_LOOP('',(#11020));
#3405=EDGE_LOOP('',(#11021,#11022,#11023,#11024));
#3406=EDGE_LOOP('',(#11025,#11026,#11027,#11028));
#3407=EDGE_LOOP('',(#11029,#11030,#11031,#11032));
#3408=EDGE_LOOP('',(#11033,#11034,#11035,#11036));
#3409=EDGE_LOOP('',(#11037,#11038,#11039,#11040));
#3410=EDGE_LOOP('',(#11041,#11042,#11043,#11044));
#3411=EDGE_LOOP('',(#11045,#11046,#11047,#11048));
#3412=EDGE_LOOP('',(#11049,#11050,#11051,#11052));
#3413=EDGE_LOOP('',(#11053,#11054,#11055,#11056));
#3414=EDGE_LOOP('',(#11057,#11058,#11059,#11060));
#3415=EDGE_LOOP('',(#11061,#11062,#11063,#11064));
#3416=EDGE_LOOP('',(#11065,#11066,#11067,#11068));
#3417=EDGE_LOOP('',(#11069,#11070,#11071,#11072));
#3418=EDGE_LOOP('',(#11073,#11074,#11075,#11076));
#3419=EDGE_LOOP('',(#11077,#11078,#11079,#11080));
#3420=EDGE_LOOP('',(#11081,#11082,#11083,#11084));
#3421=EDGE_LOOP('',(#11085,#11086,#11087,#11088));
#3422=EDGE_LOOP('',(#11089,#11090,#11091,#11092));
#3423=EDGE_LOOP('',(#11093,#11094,#11095,#11096));
#3424=EDGE_LOOP('',(#11097,#11098,#11099,#11100));
#3425=EDGE_LOOP('',(#11101,#11102,#11103,#11104));
#3426=EDGE_LOOP('',(#11105,#11106,#11107,#11108));
#3427=EDGE_LOOP('',(#11109,#11110,#11111,#11112));
#3428=EDGE_LOOP('',(#11113,#11114,#11115,#11116));
#3429=EDGE_LOOP('',(#11117,#11118,#11119,#11120));
#3430=EDGE_LOOP('',(#11121,#11122,#11123,#11124));
#3431=EDGE_LOOP('',(#11125,#11126,#11127,#11128));
#3432=EDGE_LOOP('',(#11129,#11130,#11131,#11132));
#3433=EDGE_LOOP('',(#11133,#11134,#11135,#11136));
#3434=EDGE_LOOP('',(#11137,#11138,#11139,#11140));
#3435=EDGE_LOOP('',(#11141,#11142,#11143,#11144));
#3436=EDGE_LOOP('',(#11145,#11146,#11147,#11148));
#3437=EDGE_LOOP('',(#11149,#11150,#11151,#11152));
#3438=EDGE_LOOP('',(#11153,#11154,#11155,#11156));
#3439=EDGE_LOOP('',(#11157,#11158,#11159,#11160));
#3440=EDGE_LOOP('',(#11161,#11162,#11163,#11164));
#3441=EDGE_LOOP('',(#11165,#11166,#11167,#11168));
#3442=EDGE_LOOP('',(#11169,#11170,#11171,#11172));
#3443=EDGE_LOOP('',(#11173,#11174,#11175,#11176));
#3444=EDGE_LOOP('',(#11177,#11178,#11179,#11180));
#3445=EDGE_LOOP('',(#11181,#11182,#11183,#11184));
#3446=EDGE_LOOP('',(#11185,#11186,#11187,#11188));
#3447=EDGE_LOOP('',(#11189,#11190,#11191,#11192));
#3448=EDGE_LOOP('',(#11193,#11194,#11195,#11196));
#3449=EDGE_LOOP('',(#11197,#11198,#11199,#11200));
#3450=EDGE_LOOP('',(#11201,#11202,#11203,#11204));
#3451=EDGE_LOOP('',(#11205,#11206,#11207,#11208));
#3452=EDGE_LOOP('',(#11209,#11210,#11211,#11212));
#3453=EDGE_LOOP('',(#11213,#11214,#11215,#11216));
#3454=EDGE_LOOP('',(#11217,#11218,#11219,#11220));
#3455=EDGE_LOOP('',(#11221,#11222,#11223,#11224));
#3456=EDGE_LOOP('',(#11225,#11226,#11227,#11228));
#3457=EDGE_LOOP('',(#11229,#11230,#11231,#11232));
#3458=EDGE_LOOP('',(#11233,#11234,#11235,#11236));
#3459=EDGE_LOOP('',(#11237,#11238,#11239,#11240));
#3460=EDGE_LOOP('',(#11241,#11242,#11243,#11244));
#3461=EDGE_LOOP('',(#11245,#11246,#11247,#11248));
#3462=EDGE_LOOP('',(#11249,#11250,#11251,#11252));
#3463=EDGE_LOOP('',(#11253,#11254,#11255,#11256));
#3464=EDGE_LOOP('',(#11257,#11258,#11259,#11260));
#3465=EDGE_LOOP('',(#11261,#11262,#11263,#11264));
#3466=EDGE_LOOP('',(#11265,#11266,#11267,#11268));
#3467=EDGE_LOOP('',(#11269,#11270,#11271,#11272));
#3468=EDGE_LOOP('',(#11273,#11274,#11275,#11276));
#3469=EDGE_LOOP('',(#11277,#11278,#11279,#11280));
#3470=EDGE_LOOP('',(#11281,#11282,#11283,#11284));
#3471=EDGE_LOOP('',(#11285,#11286,#11287,#11288));
#3472=EDGE_LOOP('',(#11289,#11290,#11291,#11292));
#3473=EDGE_LOOP('',(#11293,#11294,#11295,#11296));
#3474=EDGE_LOOP('',(#11297,#11298,#11299,#11300));
#3475=EDGE_LOOP('',(#11301,#11302,#11303,#11304));
#3476=EDGE_LOOP('',(#11305,#11306,#11307,#11308));
#3477=EDGE_LOOP('',(#11309,#11310,#11311,#11312));
#3478=EDGE_LOOP('',(#11313,#11314,#11315,#11316));
#3479=EDGE_LOOP('',(#11317,#11318,#11319,#11320));
#3480=EDGE_LOOP('',(#11321,#11322,#11323,#11324,#11325,#11326,#11327,#11328,
#11329,#11330,#11331,#11332,#11333,#11334,#11335,#11336,#11337,#11338,#11339,
#11340,#11341,#11342,#11343,#11344,#11345,#11346,#11347,#11348,#11349,#11350,
#11351,#11352,#11353,#11354,#11355,#11356,#11357,#11358,#11359,#11360,#11361,
#11362,#11363,#11364,#11365,#11366,#11367,#11368,#11369,#11370,#11371,#11372,
#11373,#11374,#11375,#11376,#11377,#11378,#11379,#11380,#11381,#11382,#11383,
#11384,#11385,#11386,#11387,#11388,#11389,#11390,#11391,#11392));
#3481=EDGE_LOOP('',(#11393,#11394,#11395,#11396));
#3482=EDGE_LOOP('',(#11397));
#3483=EDGE_LOOP('',(#11398));
#3484=EDGE_LOOP('',(#11399));
#3485=EDGE_LOOP('',(#11400));
#4080=LINE('',#28044,#4916);
#4081=LINE('',#28056,#4917);
#4082=LINE('',#28079,#4918);
#4083=LINE('',#28169,#4919);
#4084=LINE('',#28256,#4920);
#4085=LINE('',#28343,#4921);
#4086=LINE('',#28430,#4922);
#4087=LINE('',#28520,#4923);
#4088=LINE('',#28607,#4924);
#4089=LINE('',#28694,#4925);
#4090=LINE('',#28784,#4926);
#4091=LINE('',#28871,#4927);
#4092=LINE('',#28958,#4928);
#4093=LINE('',#29045,#4929);
#4094=LINE('',#29135,#4930);
#4095=LINE('',#29222,#4931);
#4096=LINE('',#29309,#4932);
#4097=LINE('',#29396,#4933);
#4098=LINE('',#29486,#4934);
#4099=LINE('',#29573,#4935);
#4100=LINE('',#29660,#4936);
#4101=LINE('',#29750,#4937);
#4102=LINE('',#29837,#4938);
#4103=LINE('',#29924,#4939);
#4104=LINE('',#30011,#4940);
#4105=LINE('',#30101,#4941);
#4106=LINE('',#30170,#4942);
#4107=LINE('',#30203,#4943);
#4108=LINE('',#30240,#4944);
#4109=LINE('',#30278,#4945);
#4110=LINE('',#30314,#4946);
#4111=LINE('',#30352,#4947);
#4112=LINE('',#30390,#4948);
#4113=LINE('',#30426,#4949);
#4114=LINE('',#30464,#4950);
#4115=LINE('',#30502,#4951);
#4116=LINE('',#30538,#4952);
#4117=LINE('',#30576,#4953);
#4118=LINE('',#30613,#4954);
#4119=LINE('',#30650,#4955);
#4120=LINE('',#30688,#4956);
#4121=LINE('',#30724,#4957);
#4122=LINE('',#30762,#4958);
#4123=LINE('',#30800,#4959);
#4124=LINE('',#30836,#4960);
#4125=LINE('',#30874,#4961);
#4126=LINE('',#30912,#4962);
#4127=LINE('',#30948,#4963);
#4128=LINE('',#30986,#4964);
#4129=LINE('',#31023,#4965);
#4130=LINE('',#31060,#4966);
#4131=LINE('',#31080,#4967);
#4132=LINE('',#31092,#4968);
#4133=LINE('',#31115,#4969);
#4134=LINE('',#31205,#4970);
#4135=LINE('',#31292,#4971);
#4136=LINE('',#31379,#4972);
#4137=LINE('',#31466,#4973);
#4138=LINE('',#31553,#4974);
#4139=LINE('',#31643,#4975);
#4140=LINE('',#31730,#4976);
#4141=LINE('',#31817,#4977);
#4142=LINE('',#31904,#4978);
#4143=LINE('',#31991,#4979);
#4144=LINE('',#32081,#4980);
#4145=LINE('',#32168,#4981);
#4146=LINE('',#32255,#4982);
#4147=LINE('',#32342,#4983);
#4148=LINE('',#32429,#4984);
#4149=LINE('',#32516,#4985);
#4150=LINE('',#32603,#4986);
#4151=LINE('',#32690,#4987);
#4152=LINE('',#32765,#4988);
#4153=LINE('',#32813,#4989);
#4154=LINE('',#32870,#4990);
#4155=LINE('',#32957,#4991);
#4156=LINE('',#33044,#4992);
#4157=LINE('',#33131,#4993);
#4158=LINE('',#33218,#4994);
#4159=LINE('',#33305,#4995);
#4160=LINE('',#33395,#4996);
#4161=LINE('',#33482,#4997);
#4162=LINE('',#33569,#4998);
#4163=LINE('',#33656,#4999);
#4164=LINE('',#33743,#5000);
#4165=LINE('',#33833,#5001);
#4166=LINE('',#33920,#5002);
#4167=LINE('',#34007,#5003);
#4168=LINE('',#34094,#5004);
#4169=LINE('',#34181,#5005);
#4170=LINE('',#34271,#5006);
#4171=LINE('',#34358,#5007);
#4172=LINE('',#34427,#5008);
#4173=LINE('',#34460,#5009);
#4174=LINE('',#34497,#5010);
#4175=LINE('',#34535,#5011);
#4176=LINE('',#34571,#5012);
#4177=LINE('',#34609,#5013);
#4178=LINE('',#34646,#5014);
#4179=LINE('',#34683,#5015);
#4180=LINE('',#34721,#5016);
#4181=LINE('',#34757,#5017);
#4182=LINE('',#34795,#5018);
#4183=LINE('',#34832,#5019);
#4184=LINE('',#34869,#5020);
#4185=LINE('',#34907,#5021);
#4186=LINE('',#34943,#5022);
#4187=LINE('',#34981,#5023);
#4188=LINE('',#35018,#5024);
#4189=LINE('',#35055,#5025);
#4190=LINE('',#35093,#5026);
#4191=LINE('',#35129,#5027);
#4192=LINE('',#35156,#5028);
#4193=LINE('',#35180,#5029);
#4194=LINE('',#35213,#5030);
#4195=LINE('',#35251,#5031);
#4196=LINE('',#35287,#5032);
#4197=LINE('',#35325,#5033);
#4198=LINE('',#35361,#5034);
#4199=LINE('',#35399,#5035);
#4200=LINE('',#35437,#5036);
#4201=LINE('',#35473,#5037);
#4202=LINE('',#35511,#5038);
#4203=LINE('',#35547,#5039);
#4204=LINE('',#35585,#5040);
#4205=LINE('',#35623,#5041);
#4206=LINE('',#35659,#5042);
#4207=LINE('',#35697,#5043);
#4208=LINE('',#35733,#5044);
#4209=LINE('',#35771,#5045);
#4210=LINE('',#35809,#5046);
#4211=LINE('',#35845,#5047);
#4212=LINE('',#43512,#5048);
#4213=LINE('',#43515,#5049);
#4214=LINE('',#43518,#5050);
#4215=LINE('',#43520,#5051);
#4216=LINE('',#43521,#5052);
#4217=LINE('',#43524,#5053);
#4218=LINE('',#43528,#5054);
#4219=LINE('',#43532,#5055);
#4220=LINE('',#43536,#5056);
#4221=LINE('',#43540,#5057);
#4222=LINE('',#43544,#5058);
#4223=LINE('',#43548,#5059);
#4224=LINE('',#43552,#5060);
#4225=LINE('',#43556,#5061);
#4226=LINE('',#43560,#5062);
#4227=LINE('',#43564,#5063);
#4228=LINE('',#43568,#5064);
#4229=LINE('',#43572,#5065);
#4230=LINE('',#43576,#5066);
#4231=LINE('',#43580,#5067);
#4232=LINE('',#43584,#5068);
#4233=LINE('',#43588,#5069);
#4234=LINE('',#43592,#5070);
#4235=LINE('',#43596,#5071);
#4236=LINE('',#43600,#5072);
#4237=LINE('',#43604,#5073);
#4238=LINE('',#43608,#5074);
#4239=LINE('',#43612,#5075);
#4240=LINE('',#43616,#5076);
#4241=LINE('',#43620,#5077);
#4242=LINE('',#43624,#5078);
#4243=LINE('',#43628,#5079);
#4244=LINE('',#43632,#5080);
#4245=LINE('',#43636,#5081);
#4246=LINE('',#43640,#5082);
#4247=LINE('',#43644,#5083);
#4248=LINE('',#43648,#5084);
#4249=LINE('',#43652,#5085);
#4250=LINE('',#43656,#5086);
#4251=LINE('',#43660,#5087);
#4252=LINE('',#43674,#5088);
#4253=LINE('',#43675,#5089);
#4254=LINE('',#43678,#5090);
#4255=LINE('',#43679,#5091);
#4256=LINE('',#43683,#5092);
#4257=LINE('',#43686,#5093);
#4258=LINE('',#43687,#5094);
#4259=LINE('',#43691,#5095);
#4260=LINE('',#43694,#5096);
#4261=LINE('',#43695,#5097);
#4262=LINE('',#43699,#5098);
#4263=LINE('',#43702,#5099);
#4264=LINE('',#43703,#5100);
#4265=LINE('',#43707,#5101);
#4266=LINE('',#43710,#5102);
#4267=LINE('',#43713,#5103);
#4268=LINE('',#43716,#5104);
#4269=LINE('',#43717,#5105);
#4270=LINE('',#43721,#5106);
#4271=LINE('',#43724,#5107);
#4272=LINE('',#43727,#5108);
#4273=LINE('',#43730,#5109);
#4274=LINE('',#43731,#5110);
#4275=LINE('',#43735,#5111);
#4276=LINE('',#43740,#5112);
#4277=LINE('',#43741,#5113);
#4278=LINE('',#43744,#5114);
#4279=LINE('',#43745,#5115);
#4280=LINE('',#43749,#5116);
#4281=LINE('',#43752,#5117);
#4282=LINE('',#43753,#5118);
#4283=LINE('',#43757,#5119);
#4284=LINE('',#43760,#5120);
#4285=LINE('',#43761,#5121);
#4286=LINE('',#43765,#5122);
#4287=LINE('',#43768,#5123);
#4288=LINE('',#43769,#5124);
#4289=LINE('',#43773,#5125);
#4290=LINE('',#43776,#5126);
#4291=LINE('',#43779,#5127);
#4292=LINE('',#43782,#5128);
#4293=LINE('',#43783,#5129);
#4294=LINE('',#43787,#5130);
#4295=LINE('',#43790,#5131);
#4296=LINE('',#43793,#5132);
#4297=LINE('',#43796,#5133);
#4298=LINE('',#43797,#5134);
#4299=LINE('',#43801,#5135);
#4300=LINE('',#43806,#5136);
#4301=LINE('',#43807,#5137);
#4302=LINE('',#43810,#5138);
#4303=LINE('',#43811,#5139);
#4304=LINE('',#43815,#5140);
#4305=LINE('',#43818,#5141);
#4306=LINE('',#43819,#5142);
#4307=LINE('',#43823,#5143);
#4308=LINE('',#43826,#5144);
#4309=LINE('',#43827,#5145);
#4310=LINE('',#43831,#5146);
#4311=LINE('',#43834,#5147);
#4312=LINE('',#43835,#5148);
#4313=LINE('',#43839,#5149);
#4314=LINE('',#43842,#5150);
#4315=LINE('',#43845,#5151);
#4316=LINE('',#43848,#5152);
#4317=LINE('',#43849,#5153);
#4318=LINE('',#43853,#5154);
#4319=LINE('',#43856,#5155);
#4320=LINE('',#43859,#5156);
#4321=LINE('',#43862,#5157);
#4322=LINE('',#43863,#5158);
#4323=LINE('',#43867,#5159);
#4324=LINE('',#43872,#5160);
#4325=LINE('',#43873,#5161);
#4326=LINE('',#43876,#5162);
#4327=LINE('',#43877,#5163);
#4328=LINE('',#43881,#5164);
#4329=LINE('',#43884,#5165);
#4330=LINE('',#43885,#5166);
#4331=LINE('',#43889,#5167);
#4332=LINE('',#43892,#5168);
#4333=LINE('',#43893,#5169);
#4334=LINE('',#43897,#5170);
#4335=LINE('',#43900,#5171);
#4336=LINE('',#43901,#5172);
#4337=LINE('',#43905,#5173);
#4338=LINE('',#43908,#5174);
#4339=LINE('',#43911,#5175);
#4340=LINE('',#43914,#5176);
#4341=LINE('',#43915,#5177);
#4342=LINE('',#43919,#5178);
#4343=LINE('',#43922,#5179);
#4344=LINE('',#43926,#5180);
#4345=LINE('',#43930,#5181);
#4346=LINE('',#43933,#5182);
#4347=LINE('',#43936,#5183);
#4348=LINE('',#43940,#5184);
#4349=LINE('',#43943,#5185);
#4350=LINE('',#43945,#5186);
#4351=LINE('',#43947,#5187);
#4352=LINE('',#43949,#5188);
#4353=LINE('',#43951,#5189);
#4354=LINE('',#43953,#5190);
#4355=LINE('',#43955,#5191);
#4356=LINE('',#43957,#5192);
#4357=LINE('',#43959,#5193);
#4358=LINE('',#43961,#5194);
#4359=LINE('',#43963,#5195);
#4360=LINE('',#43965,#5196);
#4916=VECTOR('',#16191,5.);
#4917=VECTOR('',#16194,5.);
#4918=VECTOR('',#16201,5.);
#4919=VECTOR('',#16204,5.);
#4920=VECTOR('',#16207,5.);
#4921=VECTOR('',#16210,5.);
#4922=VECTOR('',#16213,5.);
#4923=VECTOR('',#16216,5.);
#4924=VECTOR('',#16219,5.);
#4925=VECTOR('',#16222,5.);
#4926=VECTOR('',#16225,5.);
#4927=VECTOR('',#16228,5.);
#4928=VECTOR('',#16231,5.);
#4929=VECTOR('',#16234,5.);
#4930=VECTOR('',#16237,5.);
#4931=VECTOR('',#16240,5.);
#4932=VECTOR('',#16243,5.);
#4933=VECTOR('',#16246,5.);
#4934=VECTOR('',#16249,5.);
#4935=VECTOR('',#16252,5.);
#4936=VECTOR('',#16255,5.);
#4937=VECTOR('',#16258,5.);
#4938=VECTOR('',#16261,5.);
#4939=VECTOR('',#16264,5.);
#4940=VECTOR('',#16267,5.);
#4941=VECTOR('',#16270,5.);
#4942=VECTOR('',#16275,5.0736);
#4943=VECTOR('',#16280,5.0736);
#4944=VECTOR('',#16283,5.0736);
#4945=VECTOR('',#16286,5.0736);
#4946=VECTOR('',#16289,5.0736);
#4947=VECTOR('',#16292,5.0736);
#4948=VECTOR('',#16295,5.0736);
#4949=VECTOR('',#16298,5.0736);
#4950=VECTOR('',#16301,5.0736);
#4951=VECTOR('',#16304,5.0736);
#4952=VECTOR('',#16307,5.0736);
#4953=VECTOR('',#16310,5.0736);
#4954=VECTOR('',#16313,5.0736);
#4955=VECTOR('',#16316,5.0736);
#4956=VECTOR('',#16319,5.0736);
#4957=VECTOR('',#16322,5.0736);
#4958=VECTOR('',#16325,5.0736);
#4959=VECTOR('',#16328,5.0736);
#4960=VECTOR('',#16331,5.0736);
#4961=VECTOR('',#16334,5.0736);
#4962=VECTOR('',#16337,5.0736);
#4963=VECTOR('',#16340,5.0736);
#4964=VECTOR('',#16343,5.0736);
#4965=VECTOR('',#16346,5.0736);
#4966=VECTOR('',#16349,5.0736);
#4967=VECTOR('',#16354,5.);
#4968=VECTOR('',#16357,5.);
#4969=VECTOR('',#16364,5.);
#4970=VECTOR('',#16367,5.);
#4971=VECTOR('',#16370,5.);
#4972=VECTOR('',#16373,5.);
#4973=VECTOR('',#16376,5.);
#4974=VECTOR('',#16379,5.);
#4975=VECTOR('',#16382,5.);
#4976=VECTOR('',#16385,5.);
#4977=VECTOR('',#16388,5.);
#4978=VECTOR('',#16391,5.);
#4979=VECTOR('',#16394,5.);
#4980=VECTOR('',#16397,5.);
#4981=VECTOR('',#16400,5.);
#4982=VECTOR('',#16403,5.);
#4983=VECTOR('',#16406,5.);
#4984=VECTOR('',#16409,5.);
#4985=VECTOR('',#16412,5.);
#4986=VECTOR('',#16415,5.);
#4987=VECTOR('',#16418,5.);
#4988=VECTOR('',#16421,5.);
#4989=VECTOR('',#16424,5.);
#4990=VECTOR('',#16427,5.);
#4991=VECTOR('',#16430,5.);
#4992=VECTOR('',#16433,5.);
#4993=VECTOR('',#16436,5.);
#4994=VECTOR('',#16439,5.);
#4995=VECTOR('',#16442,5.);
#4996=VECTOR('',#16445,5.);
#4997=VECTOR('',#16448,5.);
#4998=VECTOR('',#16451,5.);
#4999=VECTOR('',#16454,5.);
#5000=VECTOR('',#16457,5.);
#5001=VECTOR('',#16460,5.);
#5002=VECTOR('',#16463,5.);
#5003=VECTOR('',#16466,5.);
#5004=VECTOR('',#16469,5.);
#5005=VECTOR('',#16472,5.);
#5006=VECTOR('',#16475,5.);
#5007=VECTOR('',#16478,5.);
#5008=VECTOR('',#16483,5.0736);
#5009=VECTOR('',#16488,5.0736);
#5010=VECTOR('',#16491,5.0736);
#5011=VECTOR('',#16494,5.0736);
#5012=VECTOR('',#16497,5.0736);
#5013=VECTOR('',#16500,5.0736);
#5014=VECTOR('',#16503,5.0736);
#5015=VECTOR('',#16506,5.0736);
#5016=VECTOR('',#16509,5.0736);
#5017=VECTOR('',#16512,5.0736);
#5018=VECTOR('',#16515,5.0736);
#5019=VECTOR('',#16518,5.0736);
#5020=VECTOR('',#16521,5.0736);
#5021=VECTOR('',#16524,5.0736);
#5022=VECTOR('',#16527,5.0736);
#5023=VECTOR('',#16530,5.0736);
#5024=VECTOR('',#16533,5.0736);
#5025=VECTOR('',#16536,5.0736);
#5026=VECTOR('',#16539,5.0736);
#5027=VECTOR('',#16542,5.0736);
#5028=VECTOR('',#16545,5.0736);
#5029=VECTOR('',#16548,5.0736);
#5030=VECTOR('',#16551,5.0736);
#5031=VECTOR('',#16554,5.0736);
#5032=VECTOR('',#16557,5.0736);
#5033=VECTOR('',#16560,5.0736);
#5034=VECTOR('',#16563,5.0736);
#5035=VECTOR('',#16566,5.0736);
#5036=VECTOR('',#16569,5.0736);
#5037=VECTOR('',#16572,5.0736);
#5038=VECTOR('',#16575,5.0736);
#5039=VECTOR('',#16578,5.0736);
#5040=VECTOR('',#16581,5.0736);
#5041=VECTOR('',#16584,5.0736);
#5042=VECTOR('',#16587,5.0736);
#5043=VECTOR('',#16590,5.0736);
#5044=VECTOR('',#16593,5.0736);
#5045=VECTOR('',#16596,5.0736);
#5046=VECTOR('',#16599,5.0736);
#5047=VECTOR('',#16602,5.0736);
#5048=VECTOR('',#16629,10.);
#5049=VECTOR('',#16632,10.);
#5050=VECTOR('',#16635,10.);
#5051=VECTOR('',#16636,10.);
#5052=VECTOR('',#16637,10.);
#5053=VECTOR('',#16640,10.);
#5054=VECTOR('',#16643,10.);
#5055=VECTOR('',#16646,10.);
#5056=VECTOR('',#16649,10.);
#5057=VECTOR('',#16652,10.);
#5058=VECTOR('',#16655,10.);
#5059=VECTOR('',#16658,10.);
#5060=VECTOR('',#16661,10.);
#5061=VECTOR('',#16664,10.);
#5062=VECTOR('',#16667,10.);
#5063=VECTOR('',#16670,10.);
#5064=VECTOR('',#16673,10.);
#5065=VECTOR('',#16676,10.);
#5066=VECTOR('',#16679,10.);
#5067=VECTOR('',#16682,10.);
#5068=VECTOR('',#16685,10.);
#5069=VECTOR('',#16688,10.);
#5070=VECTOR('',#16691,10.);
#5071=VECTOR('',#16694,10.);
#5072=VECTOR('',#16697,10.);
#5073=VECTOR('',#16700,10.);
#5074=VECTOR('',#16703,10.);
#5075=VECTOR('',#16706,10.);
#5076=VECTOR('',#16709,10.);
#5077=VECTOR('',#16712,10.);
#5078=VECTOR('',#16715,10.);
#5079=VECTOR('',#16718,10.);
#5080=VECTOR('',#16721,10.);
#5081=VECTOR('',#16724,10.);
#5082=VECTOR('',#16727,10.);
#5083=VECTOR('',#16730,10.);
#5084=VECTOR('',#16733,10.);
#5085=VECTOR('',#16736,10.);
#5086=VECTOR('',#16739,10.);
#5087=VECTOR('',#16742,10.);
#5088=VECTOR('',#16757,10.);
#5089=VECTOR('',#16758,10.);
#5090=VECTOR('',#16761,10.);
#5091=VECTOR('',#16762,10.);
#5092=VECTOR('',#16767,10.);
#5093=VECTOR('',#16770,10.);
#5094=VECTOR('',#16771,10.);
#5095=VECTOR('',#16776,10.);
#5096=VECTOR('',#16779,10.);
#5097=VECTOR('',#16780,10.);
#5098=VECTOR('',#16785,10.);
#5099=VECTOR('',#16788,10.);
#5100=VECTOR('',#16789,10.);
#5101=VECTOR('',#16794,10.);
#5102=VECTOR('',#16797,10.);
#5103=VECTOR('',#16800,10.);
#5104=VECTOR('',#16803,10.);
#5105=VECTOR('',#16804,10.);
#5106=VECTOR('',#16809,10.);
#5107=VECTOR('',#16812,10.);
#5108=VECTOR('',#16815,10.);
#5109=VECTOR('',#16818,10.);
#5110=VECTOR('',#16819,10.);
#5111=VECTOR('',#16824,10.);
#5112=VECTOR('',#16829,10.);
#5113=VECTOR('',#16830,10.);
#5114=VECTOR('',#16833,10.);
#5115=VECTOR('',#16834,10.);
#5116=VECTOR('',#16839,10.);
#5117=VECTOR('',#16842,10.);
#5118=VECTOR('',#16843,10.);
#5119=VECTOR('',#16848,10.);
#5120=VECTOR('',#16851,10.);
#5121=VECTOR('',#16852,10.);
#5122=VECTOR('',#16857,10.);
#5123=VECTOR('',#16860,10.);
#5124=VECTOR('',#16861,10.);
#5125=VECTOR('',#16866,10.);
#5126=VECTOR('',#16869,10.);
#5127=VECTOR('',#16872,10.);
#5128=VECTOR('',#16875,10.);
#5129=VECTOR('',#16876,10.);
#5130=VECTOR('',#16881,10.);
#5131=VECTOR('',#16884,10.);
#5132=VECTOR('',#16887,10.);
#5133=VECTOR('',#16890,10.);
#5134=VECTOR('',#16891,10.);
#5135=VECTOR('',#16896,10.);
#5136=VECTOR('',#16901,10.);
#5137=VECTOR('',#16902,10.);
#5138=VECTOR('',#16905,10.);
#5139=VECTOR('',#16906,10.);
#5140=VECTOR('',#16911,10.);
#5141=VECTOR('',#16914,10.);
#5142=VECTOR('',#16915,10.);
#5143=VECTOR('',#16920,10.);
#5144=VECTOR('',#16923,10.);
#5145=VECTOR('',#16924,10.);
#5146=VECTOR('',#16929,10.);
#5147=VECTOR('',#16932,10.);
#5148=VECTOR('',#16933,10.);
#5149=VECTOR('',#16938,10.);
#5150=VECTOR('',#16941,10.);
#5151=VECTOR('',#16944,10.);
#5152=VECTOR('',#16947,10.);
#5153=VECTOR('',#16948,10.);
#5154=VECTOR('',#16953,10.);
#5155=VECTOR('',#16956,10.);
#5156=VECTOR('',#16959,10.);
#5157=VECTOR('',#16962,10.);
#5158=VECTOR('',#16963,10.);
#5159=VECTOR('',#16968,10.);
#5160=VECTOR('',#16973,10.);
#5161=VECTOR('',#16974,10.);
#5162=VECTOR('',#16977,10.);
#5163=VECTOR('',#16978,10.);
#5164=VECTOR('',#16983,10.);
#5165=VECTOR('',#16986,10.);
#5166=VECTOR('',#16987,10.);
#5167=VECTOR('',#16992,10.);
#5168=VECTOR('',#16995,10.);
#5169=VECTOR('',#16996,10.);
#5170=VECTOR('',#17001,10.);
#5171=VECTOR('',#17004,10.);
#5172=VECTOR('',#17005,10.);
#5173=VECTOR('',#17010,10.);
#5174=VECTOR('',#17013,10.);
#5175=VECTOR('',#17016,10.);
#5176=VECTOR('',#17019,10.);
#5177=VECTOR('',#17020,10.);
#5178=VECTOR('',#17025,10.);
#5179=VECTOR('',#17028,10.);
#5180=VECTOR('',#17033,3.);
#5181=VECTOR('',#17038,3.);
#5182=VECTOR('',#17043,4.);
#5183=VECTOR('',#17046,3.);
#5184=VECTOR('',#17051,3.);
#5185=VECTOR('',#17056,10.);
#5186=VECTOR('',#17059,10.);
#5187=VECTOR('',#17062,10.);
#5188=VECTOR('',#17065,10.);
#5189=VECTOR('',#17068,10.);
#5190=VECTOR('',#17071,10.);
#5191=VECTOR('',#17074,10.);
#5192=VECTOR('',#17077,10.);
#5193=VECTOR('',#17080,10.);
#5194=VECTOR('',#17083,10.);
#5195=VECTOR('',#17086,10.);
#5196=VECTOR('',#17089,10.);
#5882=VERTEX_POINT('',#28042);
#5883=VERTEX_POINT('',#28043);
#5884=VERTEX_POINT('',#28045);
#5885=VERTEX_POINT('',#28053);
#5886=VERTEX_POINT('',#28055);
#5887=VERTEX_POINT('',#28058);
#5888=VERTEX_POINT('',#28077);
#5889=VERTEX_POINT('',#28078);
#5890=VERTEX_POINT('',#28167);
#5891=VERTEX_POINT('',#28168);
#5892=VERTEX_POINT('',#28254);
#5893=VERTEX_POINT('',#28255);
#5894=VERTEX_POINT('',#28341);
#5895=VERTEX_POINT('',#28342);
#5896=VERTEX_POINT('',#28428);
#5897=VERTEX_POINT('',#28429);
#5898=VERTEX_POINT('',#28518);
#5899=VERTEX_POINT('',#28519);
#5900=VERTEX_POINT('',#28605);
#5901=VERTEX_POINT('',#28606);
#5902=VERTEX_POINT('',#28692);
#5903=VERTEX_POINT('',#28693);
#5904=VERTEX_POINT('',#28782);
#5905=VERTEX_POINT('',#28783);
#5906=VERTEX_POINT('',#28869);
#5907=VERTEX_POINT('',#28870);
#5908=VERTEX_POINT('',#28956);
#5909=VERTEX_POINT('',#28957);
#5910=VERTEX_POINT('',#29043);
#5911=VERTEX_POINT('',#29044);
#5912=VERTEX_POINT('',#29133);
#5913=VERTEX_POINT('',#29134);
#5914=VERTEX_POINT('',#29220);
#5915=VERTEX_POINT('',#29221);
#5916=VERTEX_POINT('',#29307);
#5917=VERTEX_POINT('',#29308);
#5918=VERTEX_POINT('',#29394);
#5919=VERTEX_POINT('',#29395);
#5920=VERTEX_POINT('',#29484);
#5921=VERTEX_POINT('',#29485);
#5922=VERTEX_POINT('',#29571);
#5923=VERTEX_POINT('',#29572);
#5924=VERTEX_POINT('',#29658);
#5925=VERTEX_POINT('',#29659);
#5926=VERTEX_POINT('',#29748);
#5927=VERTEX_POINT('',#29749);
#5928=VERTEX_POINT('',#29835);
#5929=VERTEX_POINT('',#29836);
#5930=VERTEX_POINT('',#29922);
#5931=VERTEX_POINT('',#29923);
#5932=VERTEX_POINT('',#30009);
#5933=VERTEX_POINT('',#30010);
#5934=VERTEX_POINT('',#30099);
#5935=VERTEX_POINT('',#30100);
#5936=VERTEX_POINT('',#30102);
#5937=VERTEX_POINT('',#30128);
#5938=VERTEX_POINT('',#30168);
#5939=VERTEX_POINT('',#30169);
#5940=VERTEX_POINT('',#30171);
#5941=VERTEX_POINT('',#30184);
#5942=VERTEX_POINT('',#30201);
#5943=VERTEX_POINT('',#30202);
#5944=VERTEX_POINT('',#30238);
#5945=VERTEX_POINT('',#30239);
#5946=VERTEX_POINT('',#30276);
#5947=VERTEX_POINT('',#30277);
#5948=VERTEX_POINT('',#30312);
#5949=VERTEX_POINT('',#30313);
#5950=VERTEX_POINT('',#30350);
#5951=VERTEX_POINT('',#30351);
#5952=VERTEX_POINT('',#30388);
#5953=VERTEX_POINT('',#30389);
#5954=VERTEX_POINT('',#30424);
#5955=VERTEX_POINT('',#30425);
#5956=VERTEX_POINT('',#30462);
#5957=VERTEX_POINT('',#30463);
#5958=VERTEX_POINT('',#30500);
#5959=VERTEX_POINT('',#30501);
#5960=VERTEX_POINT('',#30536);
#5961=VERTEX_POINT('',#30537);
#5962=VERTEX_POINT('',#30574);
#5963=VERTEX_POINT('',#30575);
#5964=VERTEX_POINT('',#30611);
#5965=VERTEX_POINT('',#30612);
#5966=VERTEX_POINT('',#30648);
#5967=VERTEX_POINT('',#30649);
#5968=VERTEX_POINT('',#30686);
#5969=VERTEX_POINT('',#30687);
#5970=VERTEX_POINT('',#30722);
#5971=VERTEX_POINT('',#30723);
#5972=VERTEX_POINT('',#30760);
#5973=VERTEX_POINT('',#30761);
#5974=VERTEX_POINT('',#30798);
#5975=VERTEX_POINT('',#30799);
#5976=VERTEX_POINT('',#30834);
#5977=VERTEX_POINT('',#30835);
#5978=VERTEX_POINT('',#30872);
#5979=VERTEX_POINT('',#30873);
#5980=VERTEX_POINT('',#30910);
#5981=VERTEX_POINT('',#30911);
#5982=VERTEX_POINT('',#30946);
#5983=VERTEX_POINT('',#30947);
#5984=VERTEX_POINT('',#30984);
#5985=VERTEX_POINT('',#30985);
#5986=VERTEX_POINT('',#31021);
#5987=VERTEX_POINT('',#31022);
#5988=VERTEX_POINT('',#31058);
#5989=VERTEX_POINT('',#31059);
#5990=VERTEX_POINT('',#31061);
#5991=VERTEX_POINT('',#31068);
#5992=VERTEX_POINT('',#31078);
#5993=VERTEX_POINT('',#31079);
#5994=VERTEX_POINT('',#31081);
#5995=VERTEX_POINT('',#31089);
#5996=VERTEX_POINT('',#31091);
#5997=VERTEX_POINT('',#31094);
#5998=VERTEX_POINT('',#31113);
#5999=VERTEX_POINT('',#31114);
#6000=VERTEX_POINT('',#31203);
#6001=VERTEX_POINT('',#31204);
#6002=VERTEX_POINT('',#31290);
#6003=VERTEX_POINT('',#31291);
#6004=VERTEX_POINT('',#31377);
#6005=VERTEX_POINT('',#31378);
#6006=VERTEX_POINT('',#31464);
#6007=VERTEX_POINT('',#31465);
#6008=VERTEX_POINT('',#31551);
#6009=VERTEX_POINT('',#31552);
#6010=VERTEX_POINT('',#31641);
#6011=VERTEX_POINT('',#31642);
#6012=VERTEX_POINT('',#31728);
#6013=VERTEX_POINT('',#31729);
#6014=VERTEX_POINT('',#31815);
#6015=VERTEX_POINT('',#31816);
#6016=VERTEX_POINT('',#31902);
#6017=VERTEX_POINT('',#31903);
#6018=VERTEX_POINT('',#31989);
#6019=VERTEX_POINT('',#31990);
#6020=VERTEX_POINT('',#32079);
#6021=VERTEX_POINT('',#32080);
#6022=VERTEX_POINT('',#32166);
#6023=VERTEX_POINT('',#32167);
#6024=VERTEX_POINT('',#32253);
#6025=VERTEX_POINT('',#32254);
#6026=VERTEX_POINT('',#32340);
#6027=VERTEX_POINT('',#32341);
#6028=VERTEX_POINT('',#32427);
#6029=VERTEX_POINT('',#32428);
#6030=VERTEX_POINT('',#32514);
#6031=VERTEX_POINT('',#32515);
#6032=VERTEX_POINT('',#32601);
#6033=VERTEX_POINT('',#32602);
#6034=VERTEX_POINT('',#32688);
#6035=VERTEX_POINT('',#32689);
#6036=VERTEX_POINT('',#32763);
#6037=VERTEX_POINT('',#32764);
#6038=VERTEX_POINT('',#32811);
#6039=VERTEX_POINT('',#32812);
#6040=VERTEX_POINT('',#32868);
#6041=VERTEX_POINT('',#32869);
#6042=VERTEX_POINT('',#32955);
#6043=VERTEX_POINT('',#32956);
#6044=VERTEX_POINT('',#33042);
#6045=VERTEX_POINT('',#33043);
#6046=VERTEX_POINT('',#33129);
#6047=VERTEX_POINT('',#33130);
#6048=VERTEX_POINT('',#33216);
#6049=VERTEX_POINT('',#33217);
#6050=VERTEX_POINT('',#33303);
#6051=VERTEX_POINT('',#33304);
#6052=VERTEX_POINT('',#33393);
#6053=VERTEX_POINT('',#33394);
#6054=VERTEX_POINT('',#33480);
#6055=VERTEX_POINT('',#33481);
#6056=VERTEX_POINT('',#33567);
#6057=VERTEX_POINT('',#33568);
#6058=VERTEX_POINT('',#33654);
#6059=VERTEX_POINT('',#33655);
#6060=VERTEX_POINT('',#33741);
#6061=VERTEX_POINT('',#33742);
#6062=VERTEX_POINT('',#33831);
#6063=VERTEX_POINT('',#33832);
#6064=VERTEX_POINT('',#33918);
#6065=VERTEX_POINT('',#33919);
#6066=VERTEX_POINT('',#34005);
#6067=VERTEX_POINT('',#34006);
#6068=VERTEX_POINT('',#34092);
#6069=VERTEX_POINT('',#34093);
#6070=VERTEX_POINT('',#34179);
#6071=VERTEX_POINT('',#34180);
#6072=VERTEX_POINT('',#34269);
#6073=VERTEX_POINT('',#34270);
#6074=VERTEX_POINT('',#34356);
#6075=VERTEX_POINT('',#34357);
#6076=VERTEX_POINT('',#34359);
#6077=VERTEX_POINT('',#34385);
#6078=VERTEX_POINT('',#34425);
#6079=VERTEX_POINT('',#34426);
#6080=VERTEX_POINT('',#34428);
#6081=VERTEX_POINT('',#34441);
#6082=VERTEX_POINT('',#34458);
#6083=VERTEX_POINT('',#34459);
#6084=VERTEX_POINT('',#34495);
#6085=VERTEX_POINT('',#34496);
#6086=VERTEX_POINT('',#34533);
#6087=VERTEX_POINT('',#34534);
#6088=VERTEX_POINT('',#34569);
#6089=VERTEX_POINT('',#34570);
#6090=VERTEX_POINT('',#34607);
#6091=VERTEX_POINT('',#34608);
#6092=VERTEX_POINT('',#34644);
#6093=VERTEX_POINT('',#34645);
#6094=VERTEX_POINT('',#34681);
#6095=VERTEX_POINT('',#34682);
#6096=VERTEX_POINT('',#34719);
#6097=VERTEX_POINT('',#34720);
#6098=VERTEX_POINT('',#34755);
#6099=VERTEX_POINT('',#34756);
#6100=VERTEX_POINT('',#34793);
#6101=VERTEX_POINT('',#34794);
#6102=VERTEX_POINT('',#34830);
#6103=VERTEX_POINT('',#34831);
#6104=VERTEX_POINT('',#34867);
#6105=VERTEX_POINT('',#34868);
#6106=VERTEX_POINT('',#34905);
#6107=VERTEX_POINT('',#34906);
#6108=VERTEX_POINT('',#34941);
#6109=VERTEX_POINT('',#34942);
#6110=VERTEX_POINT('',#34979);
#6111=VERTEX_POINT('',#34980);
#6112=VERTEX_POINT('',#35016);
#6113=VERTEX_POINT('',#35017);
#6114=VERTEX_POINT('',#35053);
#6115=VERTEX_POINT('',#35054);
#6116=VERTEX_POINT('',#35091);
#6117=VERTEX_POINT('',#35092);
#6118=VERTEX_POINT('',#35127);
#6119=VERTEX_POINT('',#35128);
#6120=VERTEX_POINT('',#35154);
#6121=VERTEX_POINT('',#35155);
#6122=VERTEX_POINT('',#35178);
#6123=VERTEX_POINT('',#35179);
#6124=VERTEX_POINT('',#35211);
#6125=VERTEX_POINT('',#35212);
#6126=VERTEX_POINT('',#35249);
#6127=VERTEX_POINT('',#35250);
#6128=VERTEX_POINT('',#35285);
#6129=VERTEX_POINT('',#35286);
#6130=VERTEX_POINT('',#35323);
#6131=VERTEX_POINT('',#35324);
#6132=VERTEX_POINT('',#35359);
#6133=VERTEX_POINT('',#35360);
#6134=VERTEX_POINT('',#35397);
#6135=VERTEX_POINT('',#35398);
#6136=VERTEX_POINT('',#35435);
#6137=VERTEX_POINT('',#35436);
#6138=VERTEX_POINT('',#35471);
#6139=VERTEX_POINT('',#35472);
#6140=VERTEX_POINT('',#35509);
#6141=VERTEX_POINT('',#35510);
#6142=VERTEX_POINT('',#35545);
#6143=VERTEX_POINT('',#35546);
#6144=VERTEX_POINT('',#35583);
#6145=VERTEX_POINT('',#35584);
#6146=VERTEX_POINT('',#35621);
#6147=VERTEX_POINT('',#35622);
#6148=VERTEX_POINT('',#35657);
#6149=VERTEX_POINT('',#35658);
#6150=VERTEX_POINT('',#35695);
#6151=VERTEX_POINT('',#35696);
#6152=VERTEX_POINT('',#35731);
#6153=VERTEX_POINT('',#35732);
#6154=VERTEX_POINT('',#35769);
#6155=VERTEX_POINT('',#35770);
#6156=VERTEX_POINT('',#35807);
#6157=VERTEX_POINT('',#35808);
#6158=VERTEX_POINT('',#35843);
#6159=VERTEX_POINT('',#35844);
#6160=VERTEX_POINT('',#35846);
#6161=VERTEX_POINT('',#35853);
#6162=VERTEX_POINT('',#40380);
#6163=VERTEX_POINT('',#43505);
#6164=VERTEX_POINT('',#43508);
#6165=VERTEX_POINT('',#43509);
#6166=VERTEX_POINT('',#43511);
#6167=VERTEX_POINT('',#43513);
#6168=VERTEX_POINT('',#43517);
#6169=VERTEX_POINT('',#43519);
#6170=VERTEX_POINT('',#43523);
#6171=VERTEX_POINT('',#43525);
#6172=VERTEX_POINT('',#43527);
#6173=VERTEX_POINT('',#43529);
#6174=VERTEX_POINT('',#43531);
#6175=VERTEX_POINT('',#43533);
#6176=VERTEX_POINT('',#43535);
#6177=VERTEX_POINT('',#43537);
#6178=VERTEX_POINT('',#43539);
#6179=VERTEX_POINT('',#43541);
#6180=VERTEX_POINT('',#43543);
#6181=VERTEX_POINT('',#43545);
#6182=VERTEX_POINT('',#43547);
#6183=VERTEX_POINT('',#43549);
#6184=VERTEX_POINT('',#43551);
#6185=VERTEX_POINT('',#43553);
#6186=VERTEX_POINT('',#43555);
#6187=VERTEX_POINT('',#43557);
#6188=VERTEX_POINT('',#43559);
#6189=VERTEX_POINT('',#43561);
#6190=VERTEX_POINT('',#43563);
#6191=VERTEX_POINT('',#43565);
#6192=VERTEX_POINT('',#43567);
#6193=VERTEX_POINT('',#43569);
#6194=VERTEX_POINT('',#43571);
#6195=VERTEX_POINT('',#43573);
#6196=VERTEX_POINT('',#43575);
#6197=VERTEX_POINT('',#43577);
#6198=VERTEX_POINT('',#43579);
#6199=VERTEX_POINT('',#43581);
#6200=VERTEX_POINT('',#43583);
#6201=VERTEX_POINT('',#43585);
#6202=VERTEX_POINT('',#43587);
#6203=VERTEX_POINT('',#43589);
#6204=VERTEX_POINT('',#43591);
#6205=VERTEX_POINT('',#43593);
#6206=VERTEX_POINT('',#43595);
#6207=VERTEX_POINT('',#43597);
#6208=VERTEX_POINT('',#43599);
#6209=VERTEX_POINT('',#43601);
#6210=VERTEX_POINT('',#43603);
#6211=VERTEX_POINT('',#43605);
#6212=VERTEX_POINT('',#43607);
#6213=VERTEX_POINT('',#43609);
#6214=VERTEX_POINT('',#43611);
#6215=VERTEX_POINT('',#43613);
#6216=VERTEX_POINT('',#43615);
#6217=VERTEX_POINT('',#43617);
#6218=VERTEX_POINT('',#43619);
#6219=VERTEX_POINT('',#43621);
#6220=VERTEX_POINT('',#43623);
#6221=VERTEX_POINT('',#43625);
#6222=VERTEX_POINT('',#43627);
#6223=VERTEX_POINT('',#43629);
#6224=VERTEX_POINT('',#43631);
#6225=VERTEX_POINT('',#43633);
#6226=VERTEX_POINT('',#43635);
#6227=VERTEX_POINT('',#43637);
#6228=VERTEX_POINT('',#43639);
#6229=VERTEX_POINT('',#43641);
#6230=VERTEX_POINT('',#43643);
#6231=VERTEX_POINT('',#43645);
#6232=VERTEX_POINT('',#43647);
#6233=VERTEX_POINT('',#43649);
#6234=VERTEX_POINT('',#43651);
#6235=VERTEX_POINT('',#43653);
#6236=VERTEX_POINT('',#43655);
#6237=VERTEX_POINT('',#43657);
#6238=VERTEX_POINT('',#43659);
#6239=VERTEX_POINT('',#43662);
#6240=VERTEX_POINT('',#43664);
#6241=VERTEX_POINT('',#43666);
#6242=VERTEX_POINT('',#43668);
#6243=VERTEX_POINT('',#43671);
#6244=VERTEX_POINT('',#43672);
#6245=VERTEX_POINT('',#43677);
#6246=VERTEX_POINT('',#43681);
#6247=VERTEX_POINT('',#43685);
#6248=VERTEX_POINT('',#43689);
#6249=VERTEX_POINT('',#43693);
#6250=VERTEX_POINT('',#43697);
#6251=VERTEX_POINT('',#43701);
#6252=VERTEX_POINT('',#43705);
#6253=VERTEX_POINT('',#43709);
#6254=VERTEX_POINT('',#43711);
#6255=VERTEX_POINT('',#43715);
#6256=VERTEX_POINT('',#43719);
#6257=VERTEX_POINT('',#43723);
#6258=VERTEX_POINT('',#43725);
#6259=VERTEX_POINT('',#43729);
#6260=VERTEX_POINT('',#43733);
#6261=VERTEX_POINT('',#43737);
#6262=VERTEX_POINT('',#43738);
#6263=VERTEX_POINT('',#43743);
#6264=VERTEX_POINT('',#43747);
#6265=VERTEX_POINT('',#43751);
#6266=VERTEX_POINT('',#43755);
#6267=VERTEX_POINT('',#43759);
#6268=VERTEX_POINT('',#43763);
#6269=VERTEX_POINT('',#43767);
#6270=VERTEX_POINT('',#43771);
#6271=VERTEX_POINT('',#43775);
#6272=VERTEX_POINT('',#43777);
#6273=VERTEX_POINT('',#43781);
#6274=VERTEX_POINT('',#43785);
#6275=VERTEX_POINT('',#43789);
#6276=VERTEX_POINT('',#43791);
#6277=VERTEX_POINT('',#43795);
#6278=VERTEX_POINT('',#43799);
#6279=VERTEX_POINT('',#43803);
#6280=VERTEX_POINT('',#43804);
#6281=VERTEX_POINT('',#43809);
#6282=VERTEX_POINT('',#43813);
#6283=VERTEX_POINT('',#43817);
#6284=VERTEX_POINT('',#43821);
#6285=VERTEX_POINT('',#43825);
#6286=VERTEX_POINT('',#43829);
#6287=VERTEX_POINT('',#43833);
#6288=VERTEX_POINT('',#43837);
#6289=VERTEX_POINT('',#43841);
#6290=VERTEX_POINT('',#43843);
#6291=VERTEX_POINT('',#43847);
#6292=VERTEX_POINT('',#43851);
#6293=VERTEX_POINT('',#43855);
#6294=VERTEX_POINT('',#43857);
#6295=VERTEX_POINT('',#43861);
#6296=VERTEX_POINT('',#43865);
#6297=VERTEX_POINT('',#43869);
#6298=VERTEX_POINT('',#43870);
#6299=VERTEX_POINT('',#43875);
#6300=VERTEX_POINT('',#43879);
#6301=VERTEX_POINT('',#43883);
#6302=VERTEX_POINT('',#43887);
#6303=VERTEX_POINT('',#43891);
#6304=VERTEX_POINT('',#43895);
#6305=VERTEX_POINT('',#43899);
#6306=VERTEX_POINT('',#43903);
#6307=VERTEX_POINT('',#43907);
#6308=VERTEX_POINT('',#43909);
#6309=VERTEX_POINT('',#43913);
#6310=VERTEX_POINT('',#43917);
#6311=VERTEX_POINT('',#43921);
#6312=VERTEX_POINT('',#43925);
#6313=VERTEX_POINT('',#43929);
#6314=VERTEX_POINT('',#43935);
#6315=VERTEX_POINT('',#43939);
#7472=EDGE_CURVE('',#5882,#5883,#4080,.T.);
#7473=EDGE_CURVE('',#5883,#5884,#752,.T.);
#7474=EDGE_CURVE('',#5884,#5885,#312,.T.);
#7475=EDGE_CURVE('',#5885,#5886,#4081,.T.);
#7476=EDGE_CURVE('',#5886,#5886,#313,.F.);
#7477=EDGE_CURVE('',#5885,#5887,#314,.T.);
#7478=EDGE_CURVE('',#5887,#5882,#753,.T.);
#7479=EDGE_CURVE('',#5888,#5889,#4082,.T.);
#7480=EDGE_CURVE('',#5889,#5883,#754,.T.);
#7481=EDGE_CURVE('',#5882,#5888,#755,.T.);
#7482=EDGE_CURVE('',#5890,#5891,#4083,.T.);
#7483=EDGE_CURVE('',#5891,#5889,#756,.T.);
#7484=EDGE_CURVE('',#5888,#5890,#757,.T.);
#7485=EDGE_CURVE('',#5892,#5893,#4084,.T.);
#7486=EDGE_CURVE('',#5893,#5891,#758,.T.);
#7487=EDGE_CURVE('',#5890,#5892,#759,.T.);
#7488=EDGE_CURVE('',#5894,#5895,#4085,.T.);
#7489=EDGE_CURVE('',#5895,#5893,#760,.T.);
#7490=EDGE_CURVE('',#5892,#5894,#761,.T.);
#7491=EDGE_CURVE('',#5896,#5897,#4086,.T.);
#7492=EDGE_CURVE('',#5897,#5895,#762,.T.);
#7493=EDGE_CURVE('',#5894,#5896,#763,.T.);
#7494=EDGE_CURVE('',#5898,#5899,#4087,.T.);
#7495=EDGE_CURVE('',#5899,#5897,#764,.T.);
#7496=EDGE_CURVE('',#5896,#5898,#765,.T.);
#7497=EDGE_CURVE('',#5900,#5901,#4088,.T.);
#7498=EDGE_CURVE('',#5901,#5899,#766,.T.);
#7499=EDGE_CURVE('',#5898,#5900,#767,.T.);
#7500=EDGE_CURVE('',#5902,#5903,#4089,.T.);
#7501=EDGE_CURVE('',#5903,#5901,#768,.T.);
#7502=EDGE_CURVE('',#5900,#5902,#769,.T.);
#7503=EDGE_CURVE('',#5904,#5905,#4090,.T.);
#7504=EDGE_CURVE('',#5905,#5903,#770,.T.);
#7505=EDGE_CURVE('',#5902,#5904,#771,.T.);
#7506=EDGE_CURVE('',#5906,#5907,#4091,.T.);
#7507=EDGE_CURVE('',#5907,#5905,#772,.T.);
#7508=EDGE_CURVE('',#5904,#5906,#773,.T.);
#7509=EDGE_CURVE('',#5908,#5909,#4092,.T.);
#7510=EDGE_CURVE('',#5909,#5907,#774,.T.);
#7511=EDGE_CURVE('',#5906,#5908,#775,.T.);
#7512=EDGE_CURVE('',#5910,#5911,#4093,.T.);
#7513=EDGE_CURVE('',#5911,#5909,#776,.T.);
#7514=EDGE_CURVE('',#5908,#5910,#777,.T.);
#7515=EDGE_CURVE('',#5912,#5913,#4094,.T.);
#7516=EDGE_CURVE('',#5913,#5911,#778,.T.);
#7517=EDGE_CURVE('',#5910,#5912,#779,.T.);
#7518=EDGE_CURVE('',#5914,#5915,#4095,.T.);
#7519=EDGE_CURVE('',#5915,#5913,#780,.T.);
#7520=EDGE_CURVE('',#5912,#5914,#781,.T.);
#7521=EDGE_CURVE('',#5916,#5917,#4096,.T.);
#7522=EDGE_CURVE('',#5917,#5915,#782,.T.);
#7523=EDGE_CURVE('',#5914,#5916,#783,.T.);
#7524=EDGE_CURVE('',#5918,#5919,#4097,.T.);
#7525=EDGE_CURVE('',#5919,#5917,#784,.T.);
#7526=EDGE_CURVE('',#5916,#5918,#785,.T.);
#7527=EDGE_CURVE('',#5920,#5921,#4098,.T.);
#7528=EDGE_CURVE('',#5921,#5919,#786,.T.);
#7529=EDGE_CURVE('',#5918,#5920,#787,.T.);
#7530=EDGE_CURVE('',#5922,#5923,#4099,.T.);
#7531=EDGE_CURVE('',#5923,#5921,#788,.T.);
#7532=EDGE_CURVE('',#5920,#5922,#789,.T.);
#7533=EDGE_CURVE('',#5924,#5925,#4100,.T.);
#7534=EDGE_CURVE('',#5925,#5923,#790,.T.);
#7535=EDGE_CURVE('',#5922,#5924,#791,.T.);
#7536=EDGE_CURVE('',#5926,#5927,#4101,.T.);
#7537=EDGE_CURVE('',#5927,#5925,#792,.T.);
#7538=EDGE_CURVE('',#5924,#5926,#793,.T.);
#7539=EDGE_CURVE('',#5928,#5929,#4102,.T.);
#7540=EDGE_CURVE('',#5929,#5927,#794,.T.);
#7541=EDGE_CURVE('',#5926,#5928,#795,.T.);
#7542=EDGE_CURVE('',#5930,#5931,#4103,.T.);
#7543=EDGE_CURVE('',#5931,#5929,#796,.T.);
#7544=EDGE_CURVE('',#5928,#5930,#797,.T.);
#7545=EDGE_CURVE('',#5932,#5933,#4104,.T.);
#7546=EDGE_CURVE('',#5933,#5931,#798,.T.);
#7547=EDGE_CURVE('',#5930,#5932,#799,.T.);
#7548=EDGE_CURVE('',#5934,#5935,#4105,.T.);
#7549=EDGE_CURVE('',#5934,#5936,#800,.T.);
#7550=EDGE_CURVE('',#5937,#5936,#315,.T.);
#7551=EDGE_CURVE('',#5937,#5935,#801,.T.);
#7552=EDGE_CURVE('',#5938,#5939,#4106,.T.);
#7553=EDGE_CURVE('',#5939,#5940,#802,.T.);
#7554=EDGE_CURVE('',#5941,#5940,#316,.T.);
#7555=EDGE_CURVE('',#5938,#5941,#803,.T.);
#7556=EDGE_CURVE('',#5942,#5943,#4107,.T.);
#7557=EDGE_CURVE('',#5943,#5939,#804,.T.);
#7558=EDGE_CURVE('',#5942,#5938,#805,.T.);
#7559=EDGE_CURVE('',#5944,#5945,#4108,.T.);
#7560=EDGE_CURVE('',#5945,#5943,#806,.T.);
#7561=EDGE_CURVE('',#5944,#5942,#807,.T.);
#7562=EDGE_CURVE('',#5946,#5947,#4109,.T.);
#7563=EDGE_CURVE('',#5947,#5945,#808,.T.);
#7564=EDGE_CURVE('',#5946,#5944,#809,.T.);
#7565=EDGE_CURVE('',#5948,#5949,#4110,.T.);
#7566=EDGE_CURVE('',#5949,#5947,#810,.T.);
#7567=EDGE_CURVE('',#5948,#5946,#811,.T.);
#7568=EDGE_CURVE('',#5950,#5951,#4111,.T.);
#7569=EDGE_CURVE('',#5951,#5949,#812,.T.);
#7570=EDGE_CURVE('',#5950,#5948,#813,.T.);
#7571=EDGE_CURVE('',#5952,#5953,#4112,.T.);
#7572=EDGE_CURVE('',#5953,#5951,#814,.T.);
#7573=EDGE_CURVE('',#5952,#5950,#815,.T.);
#7574=EDGE_CURVE('',#5954,#5955,#4113,.T.);
#7575=EDGE_CURVE('',#5955,#5953,#816,.T.);
#7576=EDGE_CURVE('',#5954,#5952,#817,.T.);
#7577=EDGE_CURVE('',#5956,#5957,#4114,.T.);
#7578=EDGE_CURVE('',#5957,#5955,#818,.T.);
#7579=EDGE_CURVE('',#5956,#5954,#819,.T.);
#7580=EDGE_CURVE('',#5958,#5959,#4115,.T.);
#7581=EDGE_CURVE('',#5959,#5957,#820,.T.);
#7582=EDGE_CURVE('',#5958,#5956,#821,.T.);
#7583=EDGE_CURVE('',#5960,#5961,#4116,.T.);
#7584=EDGE_CURVE('',#5961,#5959,#822,.T.);
#7585=EDGE_CURVE('',#5960,#5958,#823,.T.);
#7586=EDGE_CURVE('',#5962,#5963,#4117,.T.);
#7587=EDGE_CURVE('',#5963,#5961,#824,.T.);
#7588=EDGE_CURVE('',#5962,#5960,#825,.T.);
#7589=EDGE_CURVE('',#5964,#5965,#4118,.T.);
#7590=EDGE_CURVE('',#5965,#5963,#826,.T.);
#7591=EDGE_CURVE('',#5964,#5962,#827,.T.);
#7592=EDGE_CURVE('',#5966,#5967,#4119,.T.);
#7593=EDGE_CURVE('',#5967,#5965,#828,.T.);
#7594=EDGE_CURVE('',#5966,#5964,#829,.T.);
#7595=EDGE_CURVE('',#5968,#5969,#4120,.T.);
#7596=EDGE_CURVE('',#5969,#5967,#830,.T.);
#7597=EDGE_CURVE('',#5968,#5966,#831,.T.);
#7598=EDGE_CURVE('',#5970,#5971,#4121,.T.);
#7599=EDGE_CURVE('',#5971,#5969,#832,.T.);
#7600=EDGE_CURVE('',#5970,#5968,#833,.T.);
#7601=EDGE_CURVE('',#5972,#5973,#4122,.T.);
#7602=EDGE_CURVE('',#5973,#5971,#834,.T.);
#7603=EDGE_CURVE('',#5972,#5970,#835,.T.);
#7604=EDGE_CURVE('',#5974,#5975,#4123,.T.);
#7605=EDGE_CURVE('',#5975,#5973,#836,.T.);
#7606=EDGE_CURVE('',#5974,#5972,#837,.T.);
#7607=EDGE_CURVE('',#5976,#5977,#4124,.T.);
#7608=EDGE_CURVE('',#5977,#5975,#838,.T.);
#7609=EDGE_CURVE('',#5976,#5974,#839,.T.);
#7610=EDGE_CURVE('',#5978,#5979,#4125,.T.);
#7611=EDGE_CURVE('',#5979,#5977,#840,.T.);
#7612=EDGE_CURVE('',#5978,#5976,#841,.T.);
#7613=EDGE_CURVE('',#5980,#5981,#4126,.T.);
#7614=EDGE_CURVE('',#5981,#5979,#842,.T.);
#7615=EDGE_CURVE('',#5980,#5978,#843,.T.);
#7616=EDGE_CURVE('',#5982,#5983,#4127,.T.);
#7617=EDGE_CURVE('',#5983,#5981,#844,.T.);
#7618=EDGE_CURVE('',#5982,#5980,#845,.T.);
#7619=EDGE_CURVE('',#5984,#5985,#4128,.T.);
#7620=EDGE_CURVE('',#5985,#5983,#846,.T.);
#7621=EDGE_CURVE('',#5984,#5982,#847,.T.);
#7622=EDGE_CURVE('',#5986,#5987,#4129,.T.);
#7623=EDGE_CURVE('',#5987,#5985,#848,.T.);
#7624=EDGE_CURVE('',#5986,#5984,#849,.T.);
#7625=EDGE_CURVE('',#5988,#5989,#4130,.T.);
#7626=EDGE_CURVE('',#5990,#5988,#850,.T.);
#7627=EDGE_CURVE('',#5991,#5990,#317,.T.);
#7628=EDGE_CURVE('',#5991,#5989,#851,.T.);
#7629=EDGE_CURVE('',#5992,#5993,#4131,.T.);
#7630=EDGE_CURVE('',#5993,#5994,#852,.T.);
#7631=EDGE_CURVE('',#5994,#5995,#318,.T.);
#7632=EDGE_CURVE('',#5995,#5996,#4132,.T.);
#7633=EDGE_CURVE('',#5996,#5996,#319,.F.);
#7634=EDGE_CURVE('',#5995,#5997,#320,.T.);
#7635=EDGE_CURVE('',#5997,#5992,#853,.T.);
#7636=EDGE_CURVE('',#5998,#5999,#4133,.T.);
#7637=EDGE_CURVE('',#5999,#5993,#854,.T.);
#7638=EDGE_CURVE('',#5992,#5998,#855,.T.);
#7639=EDGE_CURVE('',#6000,#6001,#4134,.T.);
#7640=EDGE_CURVE('',#6001,#5999,#856,.T.);
#7641=EDGE_CURVE('',#5998,#6000,#857,.T.);
#7642=EDGE_CURVE('',#6002,#6003,#4135,.T.);
#7643=EDGE_CURVE('',#6003,#6001,#858,.T.);
#7644=EDGE_CURVE('',#6000,#6002,#859,.T.);
#7645=EDGE_CURVE('',#6004,#6005,#4136,.T.);
#7646=EDGE_CURVE('',#6005,#6003,#860,.T.);
#7647=EDGE_CURVE('',#6002,#6004,#861,.T.);
#7648=EDGE_CURVE('',#6006,#6007,#4137,.T.);
#7649=EDGE_CURVE('',#6007,#6005,#862,.T.);
#7650=EDGE_CURVE('',#6004,#6006,#863,.T.);
#7651=EDGE_CURVE('',#6008,#6009,#4138,.T.);
#7652=EDGE_CURVE('',#6009,#6007,#864,.T.);
#7653=EDGE_CURVE('',#6006,#6008,#865,.T.);
#7654=EDGE_CURVE('',#6010,#6011,#4139,.T.);
#7655=EDGE_CURVE('',#6011,#6009,#866,.T.);
#7656=EDGE_CURVE('',#6008,#6010,#867,.T.);
#7657=EDGE_CURVE('',#6012,#6013,#4140,.T.);
#7658=EDGE_CURVE('',#6013,#6011,#868,.T.);
#7659=EDGE_CURVE('',#6010,#6012,#869,.T.);
#7660=EDGE_CURVE('',#6014,#6015,#4141,.T.);
#7661=EDGE_CURVE('',#6015,#6013,#870,.T.);
#7662=EDGE_CURVE('',#6012,#6014,#871,.T.);
#7663=EDGE_CURVE('',#6016,#6017,#4142,.T.);
#7664=EDGE_CURVE('',#6017,#6015,#872,.T.);
#7665=EDGE_CURVE('',#6014,#6016,#873,.T.);
#7666=EDGE_CURVE('',#6018,#6019,#4143,.T.);
#7667=EDGE_CURVE('',#6019,#6017,#874,.T.);
#7668=EDGE_CURVE('',#6016,#6018,#875,.T.);
#7669=EDGE_CURVE('',#6020,#6021,#4144,.T.);
#7670=EDGE_CURVE('',#6021,#6019,#876,.T.);
#7671=EDGE_CURVE('',#6018,#6020,#877,.T.);
#7672=EDGE_CURVE('',#6022,#6023,#4145,.T.);
#7673=EDGE_CURVE('',#6023,#6021,#878,.T.);
#7674=EDGE_CURVE('',#6020,#6022,#879,.T.);
#7675=EDGE_CURVE('',#6024,#6025,#4146,.T.);
#7676=EDGE_CURVE('',#6025,#6023,#880,.T.);
#7677=EDGE_CURVE('',#6022,#6024,#881,.T.);
#7678=EDGE_CURVE('',#6026,#6027,#4147,.T.);
#7679=EDGE_CURVE('',#6027,#6025,#882,.T.);
#7680=EDGE_CURVE('',#6024,#6026,#883,.T.);
#7681=EDGE_CURVE('',#6028,#6029,#4148,.T.);
#7682=EDGE_CURVE('',#6029,#6027,#884,.T.);
#7683=EDGE_CURVE('',#6026,#6028,#885,.T.);
#7684=EDGE_CURVE('',#6030,#6031,#4149,.T.);
#7685=EDGE_CURVE('',#6031,#6029,#886,.T.);
#7686=EDGE_CURVE('',#6028,#6030,#887,.T.);
#7687=EDGE_CURVE('',#6032,#6033,#4150,.T.);
#7688=EDGE_CURVE('',#6033,#6031,#888,.T.);
#7689=EDGE_CURVE('',#6030,#6032,#889,.T.);
#7690=EDGE_CURVE('',#6034,#6035,#4151,.T.);
#7691=EDGE_CURVE('',#6035,#6033,#890,.T.);
#7692=EDGE_CURVE('',#6032,#6034,#891,.T.);
#7693=EDGE_CURVE('',#6036,#6037,#4152,.T.);
#7694=EDGE_CURVE('',#6037,#6035,#892,.T.);
#7695=EDGE_CURVE('',#6034,#6036,#893,.T.);
#7696=EDGE_CURVE('',#6038,#6039,#4153,.T.);
#7697=EDGE_CURVE('',#6039,#6037,#894,.T.);
#7698=EDGE_CURVE('',#6036,#6038,#895,.T.);
#7699=EDGE_CURVE('',#6040,#6041,#4154,.T.);
#7700=EDGE_CURVE('',#6041,#6039,#896,.T.);
#7701=EDGE_CURVE('',#6038,#6040,#897,.T.);
#7702=EDGE_CURVE('',#6042,#6043,#4155,.T.);
#7703=EDGE_CURVE('',#6043,#6041,#898,.T.);
#7704=EDGE_CURVE('',#6040,#6042,#899,.T.);
#7705=EDGE_CURVE('',#6044,#6045,#4156,.T.);
#7706=EDGE_CURVE('',#6045,#6043,#900,.T.);
#7707=EDGE_CURVE('',#6042,#6044,#901,.T.);
#7708=EDGE_CURVE('',#6046,#6047,#4157,.T.);
#7709=EDGE_CURVE('',#6047,#6045,#902,.T.);
#7710=EDGE_CURVE('',#6044,#6046,#903,.T.);
#7711=EDGE_CURVE('',#6048,#6049,#4158,.T.);
#7712=EDGE_CURVE('',#6049,#6047,#904,.T.);
#7713=EDGE_CURVE('',#6046,#6048,#905,.T.);
#7714=EDGE_CURVE('',#6050,#6051,#4159,.T.);
#7715=EDGE_CURVE('',#6051,#6049,#906,.T.);
#7716=EDGE_CURVE('',#6048,#6050,#907,.T.);
#7717=EDGE_CURVE('',#6052,#6053,#4160,.T.);
#7718=EDGE_CURVE('',#6053,#6051,#908,.T.);
#7719=EDGE_CURVE('',#6050,#6052,#909,.T.);
#7720=EDGE_CURVE('',#6054,#6055,#4161,.T.);
#7721=EDGE_CURVE('',#6055,#6053,#910,.T.);
#7722=EDGE_CURVE('',#6052,#6054,#911,.T.);
#7723=EDGE_CURVE('',#6056,#6057,#4162,.T.);
#7724=EDGE_CURVE('',#6057,#6055,#912,.T.);
#7725=EDGE_CURVE('',#6054,#6056,#913,.T.);
#7726=EDGE_CURVE('',#6058,#6059,#4163,.T.);
#7727=EDGE_CURVE('',#6059,#6057,#914,.T.);
#7728=EDGE_CURVE('',#6056,#6058,#915,.T.);
#7729=EDGE_CURVE('',#6060,#6061,#4164,.T.);
#7730=EDGE_CURVE('',#6061,#6059,#916,.T.);
#7731=EDGE_CURVE('',#6058,#6060,#917,.T.);
#7732=EDGE_CURVE('',#6062,#6063,#4165,.T.);
#7733=EDGE_CURVE('',#6063,#6061,#918,.T.);
#7734=EDGE_CURVE('',#6060,#6062,#919,.T.);
#7735=EDGE_CURVE('',#6064,#6065,#4166,.T.);
#7736=EDGE_CURVE('',#6065,#6063,#920,.T.);
#7737=EDGE_CURVE('',#6062,#6064,#921,.T.);
#7738=EDGE_CURVE('',#6066,#6067,#4167,.T.);
#7739=EDGE_CURVE('',#6067,#6065,#922,.T.);
#7740=EDGE_CURVE('',#6064,#6066,#923,.T.);
#7741=EDGE_CURVE('',#6068,#6069,#4168,.T.);
#7742=EDGE_CURVE('',#6069,#6067,#924,.T.);
#7743=EDGE_CURVE('',#6066,#6068,#925,.T.);
#7744=EDGE_CURVE('',#6070,#6071,#4169,.T.);
#7745=EDGE_CURVE('',#6071,#6069,#926,.T.);
#7746=EDGE_CURVE('',#6068,#6070,#927,.T.);
#7747=EDGE_CURVE('',#6072,#6073,#4170,.T.);
#7748=EDGE_CURVE('',#6073,#6071,#928,.T.);
#7749=EDGE_CURVE('',#6070,#6072,#929,.T.);
#7750=EDGE_CURVE('',#6074,#6075,#4171,.T.);
#7751=EDGE_CURVE('',#6074,#6076,#930,.T.);
#7752=EDGE_CURVE('',#6077,#6076,#321,.F.);
#7753=EDGE_CURVE('',#6077,#6075,#931,.T.);
#7754=EDGE_CURVE('',#6078,#6079,#4172,.T.);
#7755=EDGE_CURVE('',#6079,#6080,#932,.T.);
#7756=EDGE_CURVE('',#6081,#6080,#322,.T.);
#7757=EDGE_CURVE('',#6078,#6081,#933,.T.);
#7758=EDGE_CURVE('',#6082,#6083,#4173,.T.);
#7759=EDGE_CURVE('',#6083,#6079,#934,.T.);
#7760=EDGE_CURVE('',#6082,#6078,#935,.T.);
#7761=EDGE_CURVE('',#6084,#6085,#4174,.T.);
#7762=EDGE_CURVE('',#6085,#6083,#936,.T.);
#7763=EDGE_CURVE('',#6084,#6082,#937,.T.);
#7764=EDGE_CURVE('',#6086,#6087,#4175,.T.);
#7765=EDGE_CURVE('',#6087,#6085,#938,.T.);
#7766=EDGE_CURVE('',#6086,#6084,#939,.T.);
#7767=EDGE_CURVE('',#6088,#6089,#4176,.T.);
#7768=EDGE_CURVE('',#6089,#6087,#940,.T.);
#7769=EDGE_CURVE('',#6088,#6086,#941,.T.);
#7770=EDGE_CURVE('',#6090,#6091,#4177,.T.);
#7771=EDGE_CURVE('',#6091,#6089,#942,.T.);
#7772=EDGE_CURVE('',#6090,#6088,#943,.T.);
#7773=EDGE_CURVE('',#6092,#6093,#4178,.T.);
#7774=EDGE_CURVE('',#6093,#6091,#944,.T.);
#7775=EDGE_CURVE('',#6092,#6090,#945,.T.);
#7776=EDGE_CURVE('',#6094,#6095,#4179,.T.);
#7777=EDGE_CURVE('',#6095,#6093,#946,.T.);
#7778=EDGE_CURVE('',#6094,#6092,#947,.T.);
#7779=EDGE_CURVE('',#6096,#6097,#4180,.T.);
#7780=EDGE_CURVE('',#6097,#6095,#948,.T.);
#7781=EDGE_CURVE('',#6096,#6094,#949,.T.);
#7782=EDGE_CURVE('',#6098,#6099,#4181,.T.);
#7783=EDGE_CURVE('',#6099,#6097,#950,.T.);
#7784=EDGE_CURVE('',#6098,#6096,#951,.T.);
#7785=EDGE_CURVE('',#6100,#6101,#4182,.T.);
#7786=EDGE_CURVE('',#6101,#6099,#952,.T.);
#7787=EDGE_CURVE('',#6100,#6098,#953,.T.);
#7788=EDGE_CURVE('',#6102,#6103,#4183,.T.);
#7789=EDGE_CURVE('',#6103,#6101,#954,.T.);
#7790=EDGE_CURVE('',#6102,#6100,#955,.T.);
#7791=EDGE_CURVE('',#6104,#6105,#4184,.T.);
#7792=EDGE_CURVE('',#6105,#6103,#956,.T.);
#7793=EDGE_CURVE('',#6104,#6102,#957,.T.);
#7794=EDGE_CURVE('',#6106,#6107,#4185,.T.);
#7795=EDGE_CURVE('',#6107,#6105,#958,.T.);
#7796=EDGE_CURVE('',#6106,#6104,#959,.T.);
#7797=EDGE_CURVE('',#6108,#6109,#4186,.T.);
#7798=EDGE_CURVE('',#6109,#6107,#960,.T.);
#7799=EDGE_CURVE('',#6108,#6106,#961,.T.);
#7800=EDGE_CURVE('',#6110,#6111,#4187,.T.);
#7801=EDGE_CURVE('',#6111,#6109,#962,.T.);
#7802=EDGE_CURVE('',#6110,#6108,#963,.T.);
#7803=EDGE_CURVE('',#6112,#6113,#4188,.T.);
#7804=EDGE_CURVE('',#6113,#6111,#964,.T.);
#7805=EDGE_CURVE('',#6112,#6110,#965,.T.);
#7806=EDGE_CURVE('',#6114,#6115,#4189,.T.);
#7807=EDGE_CURVE('',#6115,#6113,#966,.T.);
#7808=EDGE_CURVE('',#6114,#6112,#967,.T.);
#7809=EDGE_CURVE('',#6116,#6117,#4190,.T.);
#7810=EDGE_CURVE('',#6117,#6115,#968,.T.);
#7811=EDGE_CURVE('',#6116,#6114,#969,.T.);
#7812=EDGE_CURVE('',#6118,#6119,#4191,.T.);
#7813=EDGE_CURVE('',#6119,#6117,#970,.T.);
#7814=EDGE_CURVE('',#6118,#6116,#971,.T.);
#7815=EDGE_CURVE('',#6120,#6121,#4192,.T.);
#7816=EDGE_CURVE('',#6121,#6119,#972,.T.);
#7817=EDGE_CURVE('',#6120,#6118,#973,.T.);
#7818=EDGE_CURVE('',#6122,#6123,#4193,.T.);
#7819=EDGE_CURVE('',#6123,#6121,#974,.T.);
#7820=EDGE_CURVE('',#6122,#6120,#975,.T.);
#7821=EDGE_CURVE('',#6124,#6125,#4194,.T.);
#7822=EDGE_CURVE('',#6125,#6123,#976,.T.);
#7823=EDGE_CURVE('',#6124,#6122,#977,.T.);
#7824=EDGE_CURVE('',#6126,#6127,#4195,.T.);
#7825=EDGE_CURVE('',#6127,#6125,#978,.T.);
#7826=EDGE_CURVE('',#6126,#6124,#979,.T.);
#7827=EDGE_CURVE('',#6128,#6129,#4196,.T.);
#7828=EDGE_CURVE('',#6129,#6127,#980,.T.);
#7829=EDGE_CURVE('',#6128,#6126,#981,.T.);
#7830=EDGE_CURVE('',#6130,#6131,#4197,.T.);
#7831=EDGE_CURVE('',#6131,#6129,#982,.T.);
#7832=EDGE_CURVE('',#6130,#6128,#983,.T.);
#7833=EDGE_CURVE('',#6132,#6133,#4198,.T.);
#7834=EDGE_CURVE('',#6133,#6131,#984,.T.);
#7835=EDGE_CURVE('',#6132,#6130,#985,.T.);
#7836=EDGE_CURVE('',#6134,#6135,#4199,.T.);
#7837=EDGE_CURVE('',#6135,#6133,#986,.T.);
#7838=EDGE_CURVE('',#6134,#6132,#987,.T.);
#7839=EDGE_CURVE('',#6136,#6137,#4200,.T.);
#7840=EDGE_CURVE('',#6137,#6135,#988,.T.);
#7841=EDGE_CURVE('',#6136,#6134,#989,.T.);
#7842=EDGE_CURVE('',#6138,#6139,#4201,.T.);
#7843=EDGE_CURVE('',#6139,#6137,#990,.T.);
#7844=EDGE_CURVE('',#6138,#6136,#991,.T.);
#7845=EDGE_CURVE('',#6140,#6141,#4202,.T.);
#7846=EDGE_CURVE('',#6141,#6139,#992,.T.);
#7847=EDGE_CURVE('',#6140,#6138,#993,.T.);
#7848=EDGE_CURVE('',#6142,#6143,#4203,.T.);
#7849=EDGE_CURVE('',#6143,#6141,#994,.T.);
#7850=EDGE_CURVE('',#6142,#6140,#995,.T.);
#7851=EDGE_CURVE('',#6144,#6145,#4204,.T.);
#7852=EDGE_CURVE('',#6145,#6143,#996,.T.);
#7853=EDGE_CURVE('',#6144,#6142,#997,.T.);
#7854=EDGE_CURVE('',#6146,#6147,#4205,.T.);
#7855=EDGE_CURVE('',#6147,#6145,#998,.T.);
#7856=EDGE_CURVE('',#6146,#6144,#999,.T.);
#7857=EDGE_CURVE('',#6148,#6149,#4206,.T.);
#7858=EDGE_CURVE('',#6149,#6147,#1000,.T.);
#7859=EDGE_CURVE('',#6148,#6146,#1001,.T.);
#7860=EDGE_CURVE('',#6150,#6151,#4207,.T.);
#7861=EDGE_CURVE('',#6151,#6149,#1002,.T.);
#7862=EDGE_CURVE('',#6150,#6148,#1003,.T.);
#7863=EDGE_CURVE('',#6152,#6153,#4208,.T.);
#7864=EDGE_CURVE('',#6153,#6151,#1004,.T.);
#7865=EDGE_CURVE('',#6152,#6150,#1005,.T.);
#7866=EDGE_CURVE('',#6154,#6155,#4209,.T.);
#7867=EDGE_CURVE('',#6155,#6153,#1006,.T.);
#7868=EDGE_CURVE('',#6154,#6152,#1007,.T.);
#7869=EDGE_CURVE('',#6156,#6157,#4210,.T.);
#7870=EDGE_CURVE('',#6157,#6155,#1008,.T.);
#7871=EDGE_CURVE('',#6156,#6154,#1009,.T.);
#7872=EDGE_CURVE('',#6158,#6159,#4211,.T.);
#7873=EDGE_CURVE('',#6160,#6158,#1010,.T.);
#7874=EDGE_CURVE('',#6161,#6160,#323,.T.);
#7875=EDGE_CURVE('',#6161,#6159,#1011,.T.);
#7876=EDGE_CURVE('',#5994,#6081,#1012,.T.);
#7877=EDGE_CURVE('',#6080,#5997,#1013,.T.);
#7878=EDGE_CURVE('',#6159,#6157,#1014,.T.);
#7879=EDGE_CURVE('',#6158,#6156,#1015,.T.);
#7880=EDGE_CURVE('',#6076,#6161,#1016,.T.);
#7881=EDGE_CURVE('',#6072,#6074,#1017,.T.);
#7882=EDGE_CURVE('',#6075,#6073,#1018,.T.);
#7883=EDGE_CURVE('',#6160,#6077,#1019,.T.);
#7884=EDGE_CURVE('',#6162,#6162,#324,.T.);
#7885=EDGE_CURVE('',#5884,#5941,#1020,.T.);
#7886=EDGE_CURVE('',#5940,#5887,#1021,.T.);
#7887=EDGE_CURVE('',#5989,#5987,#1022,.T.);
#7888=EDGE_CURVE('',#5988,#5986,#1023,.T.);
#7889=EDGE_CURVE('',#5936,#5991,#1024,.T.);
#7890=EDGE_CURVE('',#5932,#5934,#1025,.T.);
#7891=EDGE_CURVE('',#5935,#5933,#1026,.T.);
#7892=EDGE_CURVE('',#5990,#5937,#1027,.T.);
#7893=EDGE_CURVE('',#6163,#6163,#325,.T.);
#7894=EDGE_CURVE('',#6164,#6165,#326,.T.);
#7895=EDGE_CURVE('',#6165,#6166,#4212,.T.);
#7896=EDGE_CURVE('',#6166,#6167,#327,.T.);
#7897=EDGE_CURVE('',#6167,#6164,#4213,.T.);
#7898=EDGE_CURVE('',#6168,#6165,#4214,.T.);
#7899=EDGE_CURVE('',#6169,#6168,#4215,.T.);
#7900=EDGE_CURVE('',#6166,#6169,#4216,.T.);
#7901=EDGE_CURVE('',#6164,#6170,#4217,.T.);
#7902=EDGE_CURVE('',#6171,#6170,#328,.T.);
#7903=EDGE_CURVE('',#6171,#6172,#4218,.T.);
#7904=EDGE_CURVE('',#6173,#6172,#329,.T.);
#7905=EDGE_CURVE('',#6173,#6174,#4219,.T.);
#7906=EDGE_CURVE('',#6175,#6174,#330,.T.);
#7907=EDGE_CURVE('',#6175,#6176,#4220,.T.);
#7908=EDGE_CURVE('',#6177,#6176,#331,.T.);
#7909=EDGE_CURVE('',#6177,#6178,#4221,.T.);
#7910=EDGE_CURVE('',#6179,#6178,#332,.T.);
#7911=EDGE_CURVE('',#6179,#6180,#4222,.T.);
#7912=EDGE_CURVE('',#6181,#6180,#333,.T.);
#7913=EDGE_CURVE('',#6181,#6182,#4223,.T.);
#7914=EDGE_CURVE('',#6183,#6182,#334,.T.);
#7915=EDGE_CURVE('',#6183,#6184,#4224,.T.);
#7916=EDGE_CURVE('',#6185,#6184,#335,.T.);
#7917=EDGE_CURVE('',#6185,#6186,#4225,.T.);
#7918=EDGE_CURVE('',#6187,#6186,#336,.T.);
#7919=EDGE_CURVE('',#6187,#6188,#4226,.T.);
#7920=EDGE_CURVE('',#6189,#6188,#337,.T.);
#7921=EDGE_CURVE('',#6189,#6190,#4227,.T.);
#7922=EDGE_CURVE('',#6191,#6190,#338,.T.);
#7923=EDGE_CURVE('',#6191,#6192,#4228,.T.);
#7924=EDGE_CURVE('',#6193,#6192,#339,.T.);
#7925=EDGE_CURVE('',#6193,#6194,#4229,.T.);
#7926=EDGE_CURVE('',#6195,#6194,#340,.T.);
#7927=EDGE_CURVE('',#6195,#6196,#4230,.T.);
#7928=EDGE_CURVE('',#6197,#6196,#341,.T.);
#7929=EDGE_CURVE('',#6197,#6198,#4231,.T.);
#7930=EDGE_CURVE('',#6199,#6198,#342,.T.);
#7931=EDGE_CURVE('',#6199,#6200,#4232,.T.);
#7932=EDGE_CURVE('',#6201,#6200,#343,.T.);
#7933=EDGE_CURVE('',#6201,#6202,#4233,.T.);
#7934=EDGE_CURVE('',#6203,#6202,#344,.T.);
#7935=EDGE_CURVE('',#6203,#6204,#4234,.T.);
#7936=EDGE_CURVE('',#6205,#6204,#345,.T.);
#7937=EDGE_CURVE('',#6205,#6206,#4235,.T.);
#7938=EDGE_CURVE('',#6207,#6206,#346,.T.);
#7939=EDGE_CURVE('',#6207,#6208,#4236,.T.);
#7940=EDGE_CURVE('',#6209,#6208,#347,.T.);
#7941=EDGE_CURVE('',#6209,#6210,#4237,.T.);
#7942=EDGE_CURVE('',#6211,#6210,#348,.T.);
#7943=EDGE_CURVE('',#6211,#6212,#4238,.T.);
#7944=EDGE_CURVE('',#6213,#6212,#349,.T.);
#7945=EDGE_CURVE('',#6213,#6214,#4239,.T.);
#7946=EDGE_CURVE('',#6215,#6214,#350,.T.);
#7947=EDGE_CURVE('',#6215,#6216,#4240,.T.);
#7948=EDGE_CURVE('',#6217,#6216,#351,.T.);
#7949=EDGE_CURVE('',#6217,#6218,#4241,.T.);
#7950=EDGE_CURVE('',#6219,#6218,#352,.T.);
#7951=EDGE_CURVE('',#6219,#6220,#4242,.T.);
#7952=EDGE_CURVE('',#6221,#6220,#353,.T.);
#7953=EDGE_CURVE('',#6221,#6222,#4243,.T.);
#7954=EDGE_CURVE('',#6223,#6222,#354,.T.);
#7955=EDGE_CURVE('',#6223,#6224,#4244,.T.);
#7956=EDGE_CURVE('',#6225,#6224,#355,.T.);
#7957=EDGE_CURVE('',#6225,#6226,#4245,.T.);
#7958=EDGE_CURVE('',#6227,#6226,#356,.T.);
#7959=EDGE_CURVE('',#6227,#6228,#4246,.T.);
#7960=EDGE_CURVE('',#6229,#6228,#357,.T.);
#7961=EDGE_CURVE('',#6229,#6230,#4247,.T.);
#7962=EDGE_CURVE('',#6231,#6230,#358,.T.);
#7963=EDGE_CURVE('',#6231,#6232,#4248,.T.);
#7964=EDGE_CURVE('',#6233,#6232,#359,.T.);
#7965=EDGE_CURVE('',#6233,#6234,#4249,.T.);
#7966=EDGE_CURVE('',#6235,#6234,#360,.T.);
#7967=EDGE_CURVE('',#6235,#6236,#4250,.T.);
#7968=EDGE_CURVE('',#6237,#6236,#361,.T.);
#7969=EDGE_CURVE('',#6237,#6238,#4251,.T.);
#7970=EDGE_CURVE('',#6168,#6238,#362,.T.);
#7971=EDGE_CURVE('',#6239,#6239,#363,.T.);
#7972=EDGE_CURVE('',#6240,#6240,#364,.T.);
#7973=EDGE_CURVE('',#6241,#6241,#365,.T.);
#7974=EDGE_CURVE('',#6242,#6242,#366,.T.);
#7975=EDGE_CURVE('',#6243,#6244,#367,.T.);
#7976=EDGE_CURVE('',#6244,#6171,#4252,.T.);
#7977=EDGE_CURVE('',#6170,#6243,#4253,.T.);
#7978=EDGE_CURVE('',#6245,#6244,#4254,.T.);
#7979=EDGE_CURVE('',#6172,#6245,#4255,.T.);
#7980=EDGE_CURVE('',#6245,#6246,#368,.T.);
#7981=EDGE_CURVE('',#6246,#6173,#4256,.T.);
#7982=EDGE_CURVE('',#6247,#6246,#4257,.T.);
#7983=EDGE_CURVE('',#6174,#6247,#4258,.T.);
#7984=EDGE_CURVE('',#6247,#6248,#369,.T.);
#7985=EDGE_CURVE('',#6248,#6175,#4259,.T.);
#7986=EDGE_CURVE('',#6249,#6248,#4260,.T.);
#7987=EDGE_CURVE('',#6176,#6249,#4261,.T.);
#7988=EDGE_CURVE('',#6249,#6250,#370,.T.);
#7989=EDGE_CURVE('',#6250,#6177,#4262,.T.);
#7990=EDGE_CURVE('',#6251,#6250,#4263,.T.);
#7991=EDGE_CURVE('',#6178,#6251,#4264,.T.);
#7992=EDGE_CURVE('',#6251,#6252,#371,.T.);
#7993=EDGE_CURVE('',#6252,#6179,#4265,.T.);
#7994=EDGE_CURVE('',#6180,#6253,#4266,.T.);
#7995=EDGE_CURVE('',#6253,#6254,#372,.T.);
#7996=EDGE_CURVE('',#6254,#6181,#4267,.T.);
#7997=EDGE_CURVE('',#6255,#6254,#4268,.T.);
#7998=EDGE_CURVE('',#6182,#6255,#4269,.T.);
#7999=EDGE_CURVE('',#6255,#6256,#373,.T.);
#8000=EDGE_CURVE('',#6256,#6183,#4270,.T.);
#8001=EDGE_CURVE('',#6184,#6257,#4271,.T.);
#8002=EDGE_CURVE('',#6257,#6258,#374,.T.);
#8003=EDGE_CURVE('',#6258,#6185,#4272,.T.);
#8004=EDGE_CURVE('',#6259,#6258,#4273,.T.);
#8005=EDGE_CURVE('',#6186,#6259,#4274,.T.);
#8006=EDGE_CURVE('',#6259,#6260,#375,.T.);
#8007=EDGE_CURVE('',#6260,#6187,#4275,.T.);
#8008=EDGE_CURVE('',#6261,#6262,#376,.T.);
#8009=EDGE_CURVE('',#6262,#6189,#4276,.T.);
#8010=EDGE_CURVE('',#6188,#6261,#4277,.T.);
#8011=EDGE_CURVE('',#6263,#6262,#4278,.T.);
#8012=EDGE_CURVE('',#6190,#6263,#4279,.T.);
#8013=EDGE_CURVE('',#6263,#6264,#377,.T.);
#8014=EDGE_CURVE('',#6264,#6191,#4280,.T.);
#8015=EDGE_CURVE('',#6265,#6264,#4281,.T.);
#8016=EDGE_CURVE('',#6192,#6265,#4282,.T.);
#8017=EDGE_CURVE('',#6265,#6266,#378,.T.);
#8018=EDGE_CURVE('',#6266,#6193,#4283,.T.);
#8019=EDGE_CURVE('',#6267,#6266,#4284,.T.);
#8020=EDGE_CURVE('',#6194,#6267,#4285,.T.);
#8021=EDGE_CURVE('',#6267,#6268,#379,.T.);
#8022=EDGE_CURVE('',#6268,#6195,#4286,.T.);
#8023=EDGE_CURVE('',#6269,#6268,#4287,.T.);
#8024=EDGE_CURVE('',#6196,#6269,#4288,.T.);
#8025=EDGE_CURVE('',#6269,#6270,#380,.T.);
#8026=EDGE_CURVE('',#6270,#6197,#4289,.T.);
#8027=EDGE_CURVE('',#6198,#6271,#4290,.T.);
#8028=EDGE_CURVE('',#6271,#6272,#381,.T.);
#8029=EDGE_CURVE('',#6272,#6199,#4291,.T.);
#8030=EDGE_CURVE('',#6273,#6272,#4292,.T.);
#8031=EDGE_CURVE('',#6200,#6273,#4293,.T.);
#8032=EDGE_CURVE('',#6273,#6274,#382,.T.);
#8033=EDGE_CURVE('',#6274,#6201,#4294,.T.);
#8034=EDGE_CURVE('',#6202,#6275,#4295,.T.);
#8035=EDGE_CURVE('',#6275,#6276,#383,.T.);
#8036=EDGE_CURVE('',#6276,#6203,#4296,.T.);
#8037=EDGE_CURVE('',#6277,#6276,#4297,.T.);
#8038=EDGE_CURVE('',#6204,#6277,#4298,.T.);
#8039=EDGE_CURVE('',#6277,#6278,#384,.T.);
#8040=EDGE_CURVE('',#6278,#6205,#4299,.T.);
#8041=EDGE_CURVE('',#6279,#6280,#385,.T.);
#8042=EDGE_CURVE('',#6280,#6207,#4300,.T.);
#8043=EDGE_CURVE('',#6206,#6279,#4301,.T.);
#8044=EDGE_CURVE('',#6281,#6280,#4302,.T.);
#8045=EDGE_CURVE('',#6208,#6281,#4303,.T.);
#8046=EDGE_CURVE('',#6281,#6282,#386,.T.);
#8047=EDGE_CURVE('',#6282,#6209,#4304,.T.);
#8048=EDGE_CURVE('',#6283,#6282,#4305,.T.);
#8049=EDGE_CURVE('',#6210,#6283,#4306,.T.);
#8050=EDGE_CURVE('',#6283,#6284,#387,.T.);
#8051=EDGE_CURVE('',#6284,#6211,#4307,.T.);
#8052=EDGE_CURVE('',#6285,#6284,#4308,.T.);
#8053=EDGE_CURVE('',#6212,#6285,#4309,.T.);
#8054=EDGE_CURVE('',#6285,#6286,#388,.T.);
#8055=EDGE_CURVE('',#6286,#6213,#4310,.T.);
#8056=EDGE_CURVE('',#6287,#6286,#4311,.T.);
#8057=EDGE_CURVE('',#6214,#6287,#4312,.T.);
#8058=EDGE_CURVE('',#6287,#6288,#389,.T.);
#8059=EDGE_CURVE('',#6288,#6215,#4313,.T.);
#8060=EDGE_CURVE('',#6216,#6289,#4314,.T.);
#8061=EDGE_CURVE('',#6289,#6290,#390,.T.);
#8062=EDGE_CURVE('',#6290,#6217,#4315,.T.);
#8063=EDGE_CURVE('',#6291,#6290,#4316,.T.);
#8064=EDGE_CURVE('',#6218,#6291,#4317,.T.);
#8065=EDGE_CURVE('',#6291,#6292,#391,.T.);
#8066=EDGE_CURVE('',#6292,#6219,#4318,.T.);
#8067=EDGE_CURVE('',#6220,#6293,#4319,.T.);
#8068=EDGE_CURVE('',#6293,#6294,#392,.T.);
#8069=EDGE_CURVE('',#6294,#6221,#4320,.T.);
#8070=EDGE_CURVE('',#6295,#6294,#4321,.T.);
#8071=EDGE_CURVE('',#6222,#6295,#4322,.T.);
#8072=EDGE_CURVE('',#6295,#6296,#393,.T.);
#8073=EDGE_CURVE('',#6296,#6223,#4323,.T.);
#8074=EDGE_CURVE('',#6297,#6298,#394,.T.);
#8075=EDGE_CURVE('',#6298,#6225,#4324,.T.);
#8076=EDGE_CURVE('',#6224,#6297,#4325,.T.);
#8077=EDGE_CURVE('',#6299,#6298,#4326,.T.);
#8078=EDGE_CURVE('',#6226,#6299,#4327,.T.);
#8079=EDGE_CURVE('',#6299,#6300,#395,.T.);
#8080=EDGE_CURVE('',#6300,#6227,#4328,.T.);
#8081=EDGE_CURVE('',#6301,#6300,#4329,.T.);
#8082=EDGE_CURVE('',#6228,#6301,#4330,.T.);
#8083=EDGE_CURVE('',#6301,#6302,#396,.T.);
#8084=EDGE_CURVE('',#6302,#6229,#4331,.T.);
#8085=EDGE_CURVE('',#6303,#6302,#4332,.T.);
#8086=EDGE_CURVE('',#6230,#6303,#4333,.T.);
#8087=EDGE_CURVE('',#6303,#6304,#397,.T.);
#8088=EDGE_CURVE('',#6304,#6231,#4334,.T.);
#8089=EDGE_CURVE('',#6305,#6304,#4335,.T.);
#8090=EDGE_CURVE('',#6232,#6305,#4336,.T.);
#8091=EDGE_CURVE('',#6305,#6306,#398,.T.);
#8092=EDGE_CURVE('',#6306,#6233,#4337,.T.);
#8093=EDGE_CURVE('',#6234,#6307,#4338,.T.);
#8094=EDGE_CURVE('',#6307,#6308,#399,.T.);
#8095=EDGE_CURVE('',#6308,#6235,#4339,.T.);
#8096=EDGE_CURVE('',#6309,#6308,#4340,.T.);
#8097=EDGE_CURVE('',#6236,#6309,#4341,.T.);
#8098=EDGE_CURVE('',#6309,#6310,#400,.T.);
#8099=EDGE_CURVE('',#6310,#6237,#4342,.T.);
#8100=EDGE_CURVE('',#6238,#6311,#4343,.T.);
#8101=EDGE_CURVE('',#6311,#6169,#401,.T.);
#8102=EDGE_CURVE('',#6242,#6312,#4344,.T.);
#8103=EDGE_CURVE('',#6312,#6312,#402,.T.);
#8104=EDGE_CURVE('',#6241,#6313,#4345,.T.);
#8105=EDGE_CURVE('',#6313,#6313,#403,.T.);
#8106=EDGE_CURVE('',#6163,#6162,#4346,.T.);
#8107=EDGE_CURVE('',#6240,#6314,#4347,.T.);
#8108=EDGE_CURVE('',#6314,#6314,#404,.T.);
#8109=EDGE_CURVE('',#6239,#6315,#4348,.T.);
#8110=EDGE_CURVE('',#6315,#6315,#405,.T.);
#8111=EDGE_CURVE('',#6311,#6310,#4349,.T.);
#8112=EDGE_CURVE('',#6307,#6306,#4350,.T.);
#8113=EDGE_CURVE('',#6297,#6296,#4351,.T.);
#8114=EDGE_CURVE('',#6293,#6292,#4352,.T.);
#8115=EDGE_CURVE('',#6289,#6288,#4353,.T.);
#8116=EDGE_CURVE('',#6279,#6278,#4354,.T.);
#8117=EDGE_CURVE('',#6275,#6274,#4355,.T.);
#8118=EDGE_CURVE('',#6271,#6270,#4356,.T.);
#8119=EDGE_CURVE('',#6261,#6260,#4357,.T.);
#8120=EDGE_CURVE('',#6257,#6256,#4358,.T.);
#8121=EDGE_CURVE('',#6253,#6252,#4359,.T.);
#8122=EDGE_CURVE('',#6243,#6167,#4360,.T.);
#10099=ORIENTED_EDGE('',*,*,#7472,.T.);
#10100=ORIENTED_EDGE('',*,*,#7473,.T.);
#10101=ORIENTED_EDGE('',*,*,#7474,.T.);
#10102=ORIENTED_EDGE('',*,*,#7475,.T.);
#10103=ORIENTED_EDGE('',*,*,#7476,.T.);
#10104=ORIENTED_EDGE('',*,*,#7475,.F.);
#10105=ORIENTED_EDGE('',*,*,#7477,.T.);
#10106=ORIENTED_EDGE('',*,*,#7478,.T.);
#10107=ORIENTED_EDGE('',*,*,#7479,.T.);
#10108=ORIENTED_EDGE('',*,*,#7480,.T.);
#10109=ORIENTED_EDGE('',*,*,#7472,.F.);
#10110=ORIENTED_EDGE('',*,*,#7481,.T.);
#10111=ORIENTED_EDGE('',*,*,#7482,.T.);
#10112=ORIENTED_EDGE('',*,*,#7483,.T.);
#10113=ORIENTED_EDGE('',*,*,#7479,.F.);
#10114=ORIENTED_EDGE('',*,*,#7484,.T.);
#10115=ORIENTED_EDGE('',*,*,#7485,.T.);
#10116=ORIENTED_EDGE('',*,*,#7486,.T.);
#10117=ORIENTED_EDGE('',*,*,#7482,.F.);
#10118=ORIENTED_EDGE('',*,*,#7487,.T.);
#10119=ORIENTED_EDGE('',*,*,#7488,.T.);
#10120=ORIENTED_EDGE('',*,*,#7489,.T.);
#10121=ORIENTED_EDGE('',*,*,#7485,.F.);
#10122=ORIENTED_EDGE('',*,*,#7490,.T.);
#10123=ORIENTED_EDGE('',*,*,#7491,.T.);
#10124=ORIENTED_EDGE('',*,*,#7492,.T.);
#10125=ORIENTED_EDGE('',*,*,#7488,.F.);
#10126=ORIENTED_EDGE('',*,*,#7493,.T.);
#10127=ORIENTED_EDGE('',*,*,#7494,.T.);
#10128=ORIENTED_EDGE('',*,*,#7495,.T.);
#10129=ORIENTED_EDGE('',*,*,#7491,.F.);
#10130=ORIENTED_EDGE('',*,*,#7496,.T.);
#10131=ORIENTED_EDGE('',*,*,#7497,.T.);
#10132=ORIENTED_EDGE('',*,*,#7498,.T.);
#10133=ORIENTED_EDGE('',*,*,#7494,.F.);
#10134=ORIENTED_EDGE('',*,*,#7499,.T.);
#10135=ORIENTED_EDGE('',*,*,#7500,.T.);
#10136=ORIENTED_EDGE('',*,*,#7501,.T.);
#10137=ORIENTED_EDGE('',*,*,#7497,.F.);
#10138=ORIENTED_EDGE('',*,*,#7502,.T.);
#10139=ORIENTED_EDGE('',*,*,#7503,.T.);
#10140=ORIENTED_EDGE('',*,*,#7504,.T.);
#10141=ORIENTED_EDGE('',*,*,#7500,.F.);
#10142=ORIENTED_EDGE('',*,*,#7505,.T.);
#10143=ORIENTED_EDGE('',*,*,#7506,.T.);
#10144=ORIENTED_EDGE('',*,*,#7507,.T.);
#10145=ORIENTED_EDGE('',*,*,#7503,.F.);
#10146=ORIENTED_EDGE('',*,*,#7508,.T.);
#10147=ORIENTED_EDGE('',*,*,#7509,.T.);
#10148=ORIENTED_EDGE('',*,*,#7510,.T.);
#10149=ORIENTED_EDGE('',*,*,#7506,.F.);
#10150=ORIENTED_EDGE('',*,*,#7511,.T.);
#10151=ORIENTED_EDGE('',*,*,#7512,.T.);
#10152=ORIENTED_EDGE('',*,*,#7513,.T.);
#10153=ORIENTED_EDGE('',*,*,#7509,.F.);
#10154=ORIENTED_EDGE('',*,*,#7514,.T.);
#10155=ORIENTED_EDGE('',*,*,#7515,.T.);
#10156=ORIENTED_EDGE('',*,*,#7516,.T.);
#10157=ORIENTED_EDGE('',*,*,#7512,.F.);
#10158=ORIENTED_EDGE('',*,*,#7517,.T.);
#10159=ORIENTED_EDGE('',*,*,#7518,.T.);
#10160=ORIENTED_EDGE('',*,*,#7519,.T.);
#10161=ORIENTED_EDGE('',*,*,#7515,.F.);
#10162=ORIENTED_EDGE('',*,*,#7520,.T.);
#10163=ORIENTED_EDGE('',*,*,#7521,.T.);
#10164=ORIENTED_EDGE('',*,*,#7522,.T.);
#10165=ORIENTED_EDGE('',*,*,#7518,.F.);
#10166=ORIENTED_EDGE('',*,*,#7523,.T.);
#10167=ORIENTED_EDGE('',*,*,#7524,.T.);
#10168=ORIENTED_EDGE('',*,*,#7525,.T.);
#10169=ORIENTED_EDGE('',*,*,#7521,.F.);
#10170=ORIENTED_EDGE('',*,*,#7526,.T.);
#10171=ORIENTED_EDGE('',*,*,#7527,.T.);
#10172=ORIENTED_EDGE('',*,*,#7528,.T.);
#10173=ORIENTED_EDGE('',*,*,#7524,.F.);
#10174=ORIENTED_EDGE('',*,*,#7529,.T.);
#10175=ORIENTED_EDGE('',*,*,#7530,.T.);
#10176=ORIENTED_EDGE('',*,*,#7531,.T.);
#10177=ORIENTED_EDGE('',*,*,#7527,.F.);
#10178=ORIENTED_EDGE('',*,*,#7532,.T.);
#10179=ORIENTED_EDGE('',*,*,#7533,.T.);
#10180=ORIENTED_EDGE('',*,*,#7534,.T.);
#10181=ORIENTED_EDGE('',*,*,#7530,.F.);
#10182=ORIENTED_EDGE('',*,*,#7535,.T.);
#10183=ORIENTED_EDGE('',*,*,#7536,.T.);
#10184=ORIENTED_EDGE('',*,*,#7537,.T.);
#10185=ORIENTED_EDGE('',*,*,#7533,.F.);
#10186=ORIENTED_EDGE('',*,*,#7538,.T.);
#10187=ORIENTED_EDGE('',*,*,#7539,.T.);
#10188=ORIENTED_EDGE('',*,*,#7540,.T.);
#10189=ORIENTED_EDGE('',*,*,#7536,.F.);
#10190=ORIENTED_EDGE('',*,*,#7541,.T.);
#10191=ORIENTED_EDGE('',*,*,#7542,.T.);
#10192=ORIENTED_EDGE('',*,*,#7543,.T.);
#10193=ORIENTED_EDGE('',*,*,#7539,.F.);
#10194=ORIENTED_EDGE('',*,*,#7544,.T.);
#10195=ORIENTED_EDGE('',*,*,#7545,.T.);
#10196=ORIENTED_EDGE('',*,*,#7546,.T.);
#10197=ORIENTED_EDGE('',*,*,#7542,.F.);
#10198=ORIENTED_EDGE('',*,*,#7547,.T.);
#10199=ORIENTED_EDGE('',*,*,#7548,.F.);
#10200=ORIENTED_EDGE('',*,*,#7549,.T.);
#10201=ORIENTED_EDGE('',*,*,#7550,.F.);
#10202=ORIENTED_EDGE('',*,*,#7551,.T.);
#10203=ORIENTED_EDGE('',*,*,#7552,.T.);
#10204=ORIENTED_EDGE('',*,*,#7553,.T.);
#10205=ORIENTED_EDGE('',*,*,#7554,.F.);
#10206=ORIENTED_EDGE('',*,*,#7555,.F.);
#10207=ORIENTED_EDGE('',*,*,#7556,.T.);
#10208=ORIENTED_EDGE('',*,*,#7557,.T.);
#10209=ORIENTED_EDGE('',*,*,#7552,.F.);
#10210=ORIENTED_EDGE('',*,*,#7558,.F.);
#10211=ORIENTED_EDGE('',*,*,#7559,.T.);
#10212=ORIENTED_EDGE('',*,*,#7560,.T.);
#10213=ORIENTED_EDGE('',*,*,#7556,.F.);
#10214=ORIENTED_EDGE('',*,*,#7561,.F.);
#10215=ORIENTED_EDGE('',*,*,#7562,.T.);
#10216=ORIENTED_EDGE('',*,*,#7563,.T.);
#10217=ORIENTED_EDGE('',*,*,#7559,.F.);
#10218=ORIENTED_EDGE('',*,*,#7564,.F.);
#10219=ORIENTED_EDGE('',*,*,#7565,.T.);
#10220=ORIENTED_EDGE('',*,*,#7566,.T.);
#10221=ORIENTED_EDGE('',*,*,#7562,.F.);
#10222=ORIENTED_EDGE('',*,*,#7567,.F.);
#10223=ORIENTED_EDGE('',*,*,#7568,.T.);
#10224=ORIENTED_EDGE('',*,*,#7569,.T.);
#10225=ORIENTED_EDGE('',*,*,#7565,.F.);
#10226=ORIENTED_EDGE('',*,*,#7570,.F.);
#10227=ORIENTED_EDGE('',*,*,#7571,.T.);
#10228=ORIENTED_EDGE('',*,*,#7572,.T.);
#10229=ORIENTED_EDGE('',*,*,#7568,.F.);
#10230=ORIENTED_EDGE('',*,*,#7573,.F.);
#10231=ORIENTED_EDGE('',*,*,#7574,.T.);
#10232=ORIENTED_EDGE('',*,*,#7575,.T.);
#10233=ORIENTED_EDGE('',*,*,#7571,.F.);
#10234=ORIENTED_EDGE('',*,*,#7576,.F.);
#10235=ORIENTED_EDGE('',*,*,#7577,.T.);
#10236=ORIENTED_EDGE('',*,*,#7578,.T.);
#10237=ORIENTED_EDGE('',*,*,#7574,.F.);
#10238=ORIENTED_EDGE('',*,*,#7579,.F.);
#10239=ORIENTED_EDGE('',*,*,#7580,.T.);
#10240=ORIENTED_EDGE('',*,*,#7581,.T.);
#10241=ORIENTED_EDGE('',*,*,#7577,.F.);
#10242=ORIENTED_EDGE('',*,*,#7582,.F.);
#10243=ORIENTED_EDGE('',*,*,#7583,.T.);
#10244=ORIENTED_EDGE('',*,*,#7584,.T.);
#10245=ORIENTED_EDGE('',*,*,#7580,.F.);
#10246=ORIENTED_EDGE('',*,*,#7585,.F.);
#10247=ORIENTED_EDGE('',*,*,#7586,.T.);
#10248=ORIENTED_EDGE('',*,*,#7587,.T.);
#10249=ORIENTED_EDGE('',*,*,#7583,.F.);
#10250=ORIENTED_EDGE('',*,*,#7588,.F.);
#10251=ORIENTED_EDGE('',*,*,#7589,.T.);
#10252=ORIENTED_EDGE('',*,*,#7590,.T.);
#10253=ORIENTED_EDGE('',*,*,#7586,.F.);
#10254=ORIENTED_EDGE('',*,*,#7591,.F.);
#10255=ORIENTED_EDGE('',*,*,#7592,.T.);
#10256=ORIENTED_EDGE('',*,*,#7593,.T.);
#10257=ORIENTED_EDGE('',*,*,#7589,.F.);
#10258=ORIENTED_EDGE('',*,*,#7594,.F.);
#10259=ORIENTED_EDGE('',*,*,#7595,.T.);
#10260=ORIENTED_EDGE('',*,*,#7596,.T.);
#10261=ORIENTED_EDGE('',*,*,#7592,.F.);
#10262=ORIENTED_EDGE('',*,*,#7597,.F.);
#10263=ORIENTED_EDGE('',*,*,#7598,.T.);
#10264=ORIENTED_EDGE('',*,*,#7599,.T.);
#10265=ORIENTED_EDGE('',*,*,#7595,.F.);
#10266=ORIENTED_EDGE('',*,*,#7600,.F.);
#10267=ORIENTED_EDGE('',*,*,#7601,.T.);
#10268=ORIENTED_EDGE('',*,*,#7602,.T.);
#10269=ORIENTED_EDGE('',*,*,#7598,.F.);
#10270=ORIENTED_EDGE('',*,*,#7603,.F.);
#10271=ORIENTED_EDGE('',*,*,#7604,.T.);
#10272=ORIENTED_EDGE('',*,*,#7605,.T.);
#10273=ORIENTED_EDGE('',*,*,#7601,.F.);
#10274=ORIENTED_EDGE('',*,*,#7606,.F.);
#10275=ORIENTED_EDGE('',*,*,#7607,.T.);
#10276=ORIENTED_EDGE('',*,*,#7608,.T.);
#10277=ORIENTED_EDGE('',*,*,#7604,.F.);
#10278=ORIENTED_EDGE('',*,*,#7609,.F.);
#10279=ORIENTED_EDGE('',*,*,#7610,.T.);
#10280=ORIENTED_EDGE('',*,*,#7611,.T.);
#10281=ORIENTED_EDGE('',*,*,#7607,.F.);
#10282=ORIENTED_EDGE('',*,*,#7612,.F.);
#10283=ORIENTED_EDGE('',*,*,#7613,.T.);
#10284=ORIENTED_EDGE('',*,*,#7614,.T.);
#10285=ORIENTED_EDGE('',*,*,#7610,.F.);
#10286=ORIENTED_EDGE('',*,*,#7615,.F.);
#10287=ORIENTED_EDGE('',*,*,#7616,.T.);
#10288=ORIENTED_EDGE('',*,*,#7617,.T.);
#10289=ORIENTED_EDGE('',*,*,#7613,.F.);
#10290=ORIENTED_EDGE('',*,*,#7618,.F.);
#10291=ORIENTED_EDGE('',*,*,#7619,.T.);
#10292=ORIENTED_EDGE('',*,*,#7620,.T.);
#10293=ORIENTED_EDGE('',*,*,#7616,.F.);
#10294=ORIENTED_EDGE('',*,*,#7621,.F.);
#10295=ORIENTED_EDGE('',*,*,#7622,.T.);
#10296=ORIENTED_EDGE('',*,*,#7623,.T.);
#10297=ORIENTED_EDGE('',*,*,#7619,.F.);
#10298=ORIENTED_EDGE('',*,*,#7624,.F.);
#10299=ORIENTED_EDGE('',*,*,#7625,.F.);
#10300=ORIENTED_EDGE('',*,*,#7626,.F.);
#10301=ORIENTED_EDGE('',*,*,#7627,.F.);
#10302=ORIENTED_EDGE('',*,*,#7628,.T.);
#10303=ORIENTED_EDGE('',*,*,#7629,.T.);
#10304=ORIENTED_EDGE('',*,*,#7630,.T.);
#10305=ORIENTED_EDGE('',*,*,#7631,.T.);
#10306=ORIENTED_EDGE('',*,*,#7632,.T.);
#10307=ORIENTED_EDGE('',*,*,#7633,.T.);
#10308=ORIENTED_EDGE('',*,*,#7632,.F.);
#10309=ORIENTED_EDGE('',*,*,#7634,.T.);
#10310=ORIENTED_EDGE('',*,*,#7635,.T.);
#10311=ORIENTED_EDGE('',*,*,#7636,.T.);
#10312=ORIENTED_EDGE('',*,*,#7637,.T.);
#10313=ORIENTED_EDGE('',*,*,#7629,.F.);
#10314=ORIENTED_EDGE('',*,*,#7638,.T.);
#10315=ORIENTED_EDGE('',*,*,#7639,.T.);
#10316=ORIENTED_EDGE('',*,*,#7640,.T.);
#10317=ORIENTED_EDGE('',*,*,#7636,.F.);
#10318=ORIENTED_EDGE('',*,*,#7641,.T.);
#10319=ORIENTED_EDGE('',*,*,#7642,.T.);
#10320=ORIENTED_EDGE('',*,*,#7643,.T.);
#10321=ORIENTED_EDGE('',*,*,#7639,.F.);
#10322=ORIENTED_EDGE('',*,*,#7644,.T.);
#10323=ORIENTED_EDGE('',*,*,#7645,.T.);
#10324=ORIENTED_EDGE('',*,*,#7646,.T.);
#10325=ORIENTED_EDGE('',*,*,#7642,.F.);
#10326=ORIENTED_EDGE('',*,*,#7647,.T.);
#10327=ORIENTED_EDGE('',*,*,#7648,.T.);
#10328=ORIENTED_EDGE('',*,*,#7649,.T.);
#10329=ORIENTED_EDGE('',*,*,#7645,.F.);
#10330=ORIENTED_EDGE('',*,*,#7650,.T.);
#10331=ORIENTED_EDGE('',*,*,#7651,.T.);
#10332=ORIENTED_EDGE('',*,*,#7652,.T.);
#10333=ORIENTED_EDGE('',*,*,#7648,.F.);
#10334=ORIENTED_EDGE('',*,*,#7653,.T.);
#10335=ORIENTED_EDGE('',*,*,#7654,.T.);
#10336=ORIENTED_EDGE('',*,*,#7655,.T.);
#10337=ORIENTED_EDGE('',*,*,#7651,.F.);
#10338=ORIENTED_EDGE('',*,*,#7656,.T.);
#10339=ORIENTED_EDGE('',*,*,#7657,.T.);
#10340=ORIENTED_EDGE('',*,*,#7658,.T.);
#10341=ORIENTED_EDGE('',*,*,#7654,.F.);
#10342=ORIENTED_EDGE('',*,*,#7659,.T.);
#10343=ORIENTED_EDGE('',*,*,#7660,.T.);
#10344=ORIENTED_EDGE('',*,*,#7661,.T.);
#10345=ORIENTED_EDGE('',*,*,#7657,.F.);
#10346=ORIENTED_EDGE('',*,*,#7662,.T.);
#10347=ORIENTED_EDGE('',*,*,#7663,.T.);
#10348=ORIENTED_EDGE('',*,*,#7664,.T.);
#10349=ORIENTED_EDGE('',*,*,#7660,.F.);
#10350=ORIENTED_EDGE('',*,*,#7665,.T.);
#10351=ORIENTED_EDGE('',*,*,#7666,.T.);
#10352=ORIENTED_EDGE('',*,*,#7667,.T.);
#10353=ORIENTED_EDGE('',*,*,#7663,.F.);
#10354=ORIENTED_EDGE('',*,*,#7668,.T.);
#10355=ORIENTED_EDGE('',*,*,#7669,.T.);
#10356=ORIENTED_EDGE('',*,*,#7670,.T.);
#10357=ORIENTED_EDGE('',*,*,#7666,.F.);
#10358=ORIENTED_EDGE('',*,*,#7671,.T.);
#10359=ORIENTED_EDGE('',*,*,#7672,.T.);
#10360=ORIENTED_EDGE('',*,*,#7673,.T.);
#10361=ORIENTED_EDGE('',*,*,#7669,.F.);
#10362=ORIENTED_EDGE('',*,*,#7674,.T.);
#10363=ORIENTED_EDGE('',*,*,#7675,.T.);
#10364=ORIENTED_EDGE('',*,*,#7676,.T.);
#10365=ORIENTED_EDGE('',*,*,#7672,.F.);
#10366=ORIENTED_EDGE('',*,*,#7677,.T.);
#10367=ORIENTED_EDGE('',*,*,#7678,.T.);
#10368=ORIENTED_EDGE('',*,*,#7679,.T.);
#10369=ORIENTED_EDGE('',*,*,#7675,.F.);
#10370=ORIENTED_EDGE('',*,*,#7680,.T.);
#10371=ORIENTED_EDGE('',*,*,#7681,.T.);
#10372=ORIENTED_EDGE('',*,*,#7682,.T.);
#10373=ORIENTED_EDGE('',*,*,#7678,.F.);
#10374=ORIENTED_EDGE('',*,*,#7683,.T.);
#10375=ORIENTED_EDGE('',*,*,#7684,.T.);
#10376=ORIENTED_EDGE('',*,*,#7685,.T.);
#10377=ORIENTED_EDGE('',*,*,#7681,.F.);
#10378=ORIENTED_EDGE('',*,*,#7686,.T.);
#10379=ORIENTED_EDGE('',*,*,#7687,.T.);
#10380=ORIENTED_EDGE('',*,*,#7688,.T.);
#10381=ORIENTED_EDGE('',*,*,#7684,.F.);
#10382=ORIENTED_EDGE('',*,*,#7689,.T.);
#10383=ORIENTED_EDGE('',*,*,#7690,.T.);
#10384=ORIENTED_EDGE('',*,*,#7691,.T.);
#10385=ORIENTED_EDGE('',*,*,#7687,.F.);
#10386=ORIENTED_EDGE('',*,*,#7692,.T.);
#10387=ORIENTED_EDGE('',*,*,#7693,.T.);
#10388=ORIENTED_EDGE('',*,*,#7694,.T.);
#10389=ORIENTED_EDGE('',*,*,#7690,.F.);
#10390=ORIENTED_EDGE('',*,*,#7695,.T.);
#10391=ORIENTED_EDGE('',*,*,#7696,.T.);
#10392=ORIENTED_EDGE('',*,*,#7697,.T.);
#10393=ORIENTED_EDGE('',*,*,#7693,.F.);
#10394=ORIENTED_EDGE('',*,*,#7698,.T.);
#10395=ORIENTED_EDGE('',*,*,#7699,.T.);
#10396=ORIENTED_EDGE('',*,*,#7700,.T.);
#10397=ORIENTED_EDGE('',*,*,#7696,.F.);
#10398=ORIENTED_EDGE('',*,*,#7701,.T.);
#10399=ORIENTED_EDGE('',*,*,#7702,.T.);
#10400=ORIENTED_EDGE('',*,*,#7703,.T.);
#10401=ORIENTED_EDGE('',*,*,#7699,.F.);
#10402=ORIENTED_EDGE('',*,*,#7704,.T.);
#10403=ORIENTED_EDGE('',*,*,#7705,.T.);
#10404=ORIENTED_EDGE('',*,*,#7706,.T.);
#10405=ORIENTED_EDGE('',*,*,#7702,.F.);
#10406=ORIENTED_EDGE('',*,*,#7707,.T.);
#10407=ORIENTED_EDGE('',*,*,#7708,.T.);
#10408=ORIENTED_EDGE('',*,*,#7709,.T.);
#10409=ORIENTED_EDGE('',*,*,#7705,.F.);
#10410=ORIENTED_EDGE('',*,*,#7710,.T.);
#10411=ORIENTED_EDGE('',*,*,#7711,.T.);
#10412=ORIENTED_EDGE('',*,*,#7712,.T.);
#10413=ORIENTED_EDGE('',*,*,#7708,.F.);
#10414=ORIENTED_EDGE('',*,*,#7713,.T.);
#10415=ORIENTED_EDGE('',*,*,#7714,.T.);
#10416=ORIENTED_EDGE('',*,*,#7715,.T.);
#10417=ORIENTED_EDGE('',*,*,#7711,.F.);
#10418=ORIENTED_EDGE('',*,*,#7716,.T.);
#10419=ORIENTED_EDGE('',*,*,#7717,.T.);
#10420=ORIENTED_EDGE('',*,*,#7718,.T.);
#10421=ORIENTED_EDGE('',*,*,#7714,.F.);
#10422=ORIENTED_EDGE('',*,*,#7719,.T.);
#10423=ORIENTED_EDGE('',*,*,#7720,.T.);
#10424=ORIENTED_EDGE('',*,*,#7721,.T.);
#10425=ORIENTED_EDGE('',*,*,#7717,.F.);
#10426=ORIENTED_EDGE('',*,*,#7722,.T.);
#10427=ORIENTED_EDGE('',*,*,#7723,.T.);
#10428=ORIENTED_EDGE('',*,*,#7724,.T.);
#10429=ORIENTED_EDGE('',*,*,#7720,.F.);
#10430=ORIENTED_EDGE('',*,*,#7725,.T.);
#10431=ORIENTED_EDGE('',*,*,#7726,.T.);
#10432=ORIENTED_EDGE('',*,*,#7727,.T.);
#10433=ORIENTED_EDGE('',*,*,#7723,.F.);
#10434=ORIENTED_EDGE('',*,*,#7728,.T.);
#10435=ORIENTED_EDGE('',*,*,#7729,.T.);
#10436=ORIENTED_EDGE('',*,*,#7730,.T.);
#10437=ORIENTED_EDGE('',*,*,#7726,.F.);
#10438=ORIENTED_EDGE('',*,*,#7731,.T.);
#10439=ORIENTED_EDGE('',*,*,#7732,.T.);
#10440=ORIENTED_EDGE('',*,*,#7733,.T.);
#10441=ORIENTED_EDGE('',*,*,#7729,.F.);
#10442=ORIENTED_EDGE('',*,*,#7734,.T.);
#10443=ORIENTED_EDGE('',*,*,#7735,.T.);
#10444=ORIENTED_EDGE('',*,*,#7736,.T.);
#10445=ORIENTED_EDGE('',*,*,#7732,.F.);
#10446=ORIENTED_EDGE('',*,*,#7737,.T.);
#10447=ORIENTED_EDGE('',*,*,#7738,.T.);
#10448=ORIENTED_EDGE('',*,*,#7739,.T.);
#10449=ORIENTED_EDGE('',*,*,#7735,.F.);
#10450=ORIENTED_EDGE('',*,*,#7740,.T.);
#10451=ORIENTED_EDGE('',*,*,#7741,.T.);
#10452=ORIENTED_EDGE('',*,*,#7742,.T.);
#10453=ORIENTED_EDGE('',*,*,#7738,.F.);
#10454=ORIENTED_EDGE('',*,*,#7743,.T.);
#10455=ORIENTED_EDGE('',*,*,#7744,.T.);
#10456=ORIENTED_EDGE('',*,*,#7745,.T.);
#10457=ORIENTED_EDGE('',*,*,#7741,.F.);
#10458=ORIENTED_EDGE('',*,*,#7746,.T.);
#10459=ORIENTED_EDGE('',*,*,#7747,.T.);
#10460=ORIENTED_EDGE('',*,*,#7748,.T.);
#10461=ORIENTED_EDGE('',*,*,#7744,.F.);
#10462=ORIENTED_EDGE('',*,*,#7749,.T.);
#10463=ORIENTED_EDGE('',*,*,#7750,.F.);
#10464=ORIENTED_EDGE('',*,*,#7751,.T.);
#10465=ORIENTED_EDGE('',*,*,#7752,.F.);
#10466=ORIENTED_EDGE('',*,*,#7753,.T.);
#10467=ORIENTED_EDGE('',*,*,#7754,.T.);
#10468=ORIENTED_EDGE('',*,*,#7755,.T.);
#10469=ORIENTED_EDGE('',*,*,#7756,.F.);
#10470=ORIENTED_EDGE('',*,*,#7757,.F.);
#10471=ORIENTED_EDGE('',*,*,#7758,.T.);
#10472=ORIENTED_EDGE('',*,*,#7759,.T.);
#10473=ORIENTED_EDGE('',*,*,#7754,.F.);
#10474=ORIENTED_EDGE('',*,*,#7760,.F.);
#10475=ORIENTED_EDGE('',*,*,#7761,.T.);
#10476=ORIENTED_EDGE('',*,*,#7762,.T.);
#10477=ORIENTED_EDGE('',*,*,#7758,.F.);
#10478=ORIENTED_EDGE('',*,*,#7763,.F.);
#10479=ORIENTED_EDGE('',*,*,#7764,.T.);
#10480=ORIENTED_EDGE('',*,*,#7765,.T.);
#10481=ORIENTED_EDGE('',*,*,#7761,.F.);
#10482=ORIENTED_EDGE('',*,*,#7766,.F.);
#10483=ORIENTED_EDGE('',*,*,#7767,.T.);
#10484=ORIENTED_EDGE('',*,*,#7768,.T.);
#10485=ORIENTED_EDGE('',*,*,#7764,.F.);
#10486=ORIENTED_EDGE('',*,*,#7769,.F.);
#10487=ORIENTED_EDGE('',*,*,#7770,.T.);
#10488=ORIENTED_EDGE('',*,*,#7771,.T.);
#10489=ORIENTED_EDGE('',*,*,#7767,.F.);
#10490=ORIENTED_EDGE('',*,*,#7772,.F.);
#10491=ORIENTED_EDGE('',*,*,#7773,.T.);
#10492=ORIENTED_EDGE('',*,*,#7774,.T.);
#10493=ORIENTED_EDGE('',*,*,#7770,.F.);
#10494=ORIENTED_EDGE('',*,*,#7775,.F.);
#10495=ORIENTED_EDGE('',*,*,#7776,.T.);
#10496=ORIENTED_EDGE('',*,*,#7777,.T.);
#10497=ORIENTED_EDGE('',*,*,#7773,.F.);
#10498=ORIENTED_EDGE('',*,*,#7778,.F.);
#10499=ORIENTED_EDGE('',*,*,#7779,.T.);
#10500=ORIENTED_EDGE('',*,*,#7780,.T.);
#10501=ORIENTED_EDGE('',*,*,#7776,.F.);
#10502=ORIENTED_EDGE('',*,*,#7781,.F.);
#10503=ORIENTED_EDGE('',*,*,#7782,.T.);
#10504=ORIENTED_EDGE('',*,*,#7783,.T.);
#10505=ORIENTED_EDGE('',*,*,#7779,.F.);
#10506=ORIENTED_EDGE('',*,*,#7784,.F.);
#10507=ORIENTED_EDGE('',*,*,#7785,.T.);
#10508=ORIENTED_EDGE('',*,*,#7786,.T.);
#10509=ORIENTED_EDGE('',*,*,#7782,.F.);
#10510=ORIENTED_EDGE('',*,*,#7787,.F.);
#10511=ORIENTED_EDGE('',*,*,#7788,.T.);
#10512=ORIENTED_EDGE('',*,*,#7789,.T.);
#10513=ORIENTED_EDGE('',*,*,#7785,.F.);
#10514=ORIENTED_EDGE('',*,*,#7790,.F.);
#10515=ORIENTED_EDGE('',*,*,#7791,.T.);
#10516=ORIENTED_EDGE('',*,*,#7792,.T.);
#10517=ORIENTED_EDGE('',*,*,#7788,.F.);
#10518=ORIENTED_EDGE('',*,*,#7793,.F.);
#10519=ORIENTED_EDGE('',*,*,#7794,.T.);
#10520=ORIENTED_EDGE('',*,*,#7795,.T.);
#10521=ORIENTED_EDGE('',*,*,#7791,.F.);
#10522=ORIENTED_EDGE('',*,*,#7796,.F.);
#10523=ORIENTED_EDGE('',*,*,#7797,.T.);
#10524=ORIENTED_EDGE('',*,*,#7798,.T.);
#10525=ORIENTED_EDGE('',*,*,#7794,.F.);
#10526=ORIENTED_EDGE('',*,*,#7799,.F.);
#10527=ORIENTED_EDGE('',*,*,#7800,.T.);
#10528=ORIENTED_EDGE('',*,*,#7801,.T.);
#10529=ORIENTED_EDGE('',*,*,#7797,.F.);
#10530=ORIENTED_EDGE('',*,*,#7802,.F.);
#10531=ORIENTED_EDGE('',*,*,#7803,.T.);
#10532=ORIENTED_EDGE('',*,*,#7804,.T.);
#10533=ORIENTED_EDGE('',*,*,#7800,.F.);
#10534=ORIENTED_EDGE('',*,*,#7805,.F.);
#10535=ORIENTED_EDGE('',*,*,#7806,.T.);
#10536=ORIENTED_EDGE('',*,*,#7807,.T.);
#10537=ORIENTED_EDGE('',*,*,#7803,.F.);
#10538=ORIENTED_EDGE('',*,*,#7808,.F.);
#10539=ORIENTED_EDGE('',*,*,#7809,.T.);
#10540=ORIENTED_EDGE('',*,*,#7810,.T.);
#10541=ORIENTED_EDGE('',*,*,#7806,.F.);
#10542=ORIENTED_EDGE('',*,*,#7811,.F.);
#10543=ORIENTED_EDGE('',*,*,#7812,.T.);
#10544=ORIENTED_EDGE('',*,*,#7813,.T.);
#10545=ORIENTED_EDGE('',*,*,#7809,.F.);
#10546=ORIENTED_EDGE('',*,*,#7814,.F.);
#10547=ORIENTED_EDGE('',*,*,#7815,.T.);
#10548=ORIENTED_EDGE('',*,*,#7816,.T.);
#10549=ORIENTED_EDGE('',*,*,#7812,.F.);
#10550=ORIENTED_EDGE('',*,*,#7817,.F.);
#10551=ORIENTED_EDGE('',*,*,#7818,.T.);
#10552=ORIENTED_EDGE('',*,*,#7819,.T.);
#10553=ORIENTED_EDGE('',*,*,#7815,.F.);
#10554=ORIENTED_EDGE('',*,*,#7820,.F.);
#10555=ORIENTED_EDGE('',*,*,#7821,.T.);
#10556=ORIENTED_EDGE('',*,*,#7822,.T.);
#10557=ORIENTED_EDGE('',*,*,#7818,.F.);
#10558=ORIENTED_EDGE('',*,*,#7823,.F.);
#10559=ORIENTED_EDGE('',*,*,#7824,.T.);
#10560=ORIENTED_EDGE('',*,*,#7825,.T.);
#10561=ORIENTED_EDGE('',*,*,#7821,.F.);
#10562=ORIENTED_EDGE('',*,*,#7826,.F.);
#10563=ORIENTED_EDGE('',*,*,#7827,.T.);
#10564=ORIENTED_EDGE('',*,*,#7828,.T.);
#10565=ORIENTED_EDGE('',*,*,#7824,.F.);
#10566=ORIENTED_EDGE('',*,*,#7829,.F.);
#10567=ORIENTED_EDGE('',*,*,#7830,.T.);
#10568=ORIENTED_EDGE('',*,*,#7831,.T.);
#10569=ORIENTED_EDGE('',*,*,#7827,.F.);
#10570=ORIENTED_EDGE('',*,*,#7832,.F.);
#10571=ORIENTED_EDGE('',*,*,#7833,.T.);
#10572=ORIENTED_EDGE('',*,*,#7834,.T.);
#10573=ORIENTED_EDGE('',*,*,#7830,.F.);
#10574=ORIENTED_EDGE('',*,*,#7835,.F.);
#10575=ORIENTED_EDGE('',*,*,#7836,.T.);
#10576=ORIENTED_EDGE('',*,*,#7837,.T.);
#10577=ORIENTED_EDGE('',*,*,#7833,.F.);
#10578=ORIENTED_EDGE('',*,*,#7838,.F.);
#10579=ORIENTED_EDGE('',*,*,#7839,.T.);
#10580=ORIENTED_EDGE('',*,*,#7840,.T.);
#10581=ORIENTED_EDGE('',*,*,#7836,.F.);
#10582=ORIENTED_EDGE('',*,*,#7841,.F.);
#10583=ORIENTED_EDGE('',*,*,#7842,.T.);
#10584=ORIENTED_EDGE('',*,*,#7843,.T.);
#10585=ORIENTED_EDGE('',*,*,#7839,.F.);
#10586=ORIENTED_EDGE('',*,*,#7844,.F.);
#10587=ORIENTED_EDGE('',*,*,#7845,.T.);
#10588=ORIENTED_EDGE('',*,*,#7846,.T.);
#10589=ORIENTED_EDGE('',*,*,#7842,.F.);
#10590=ORIENTED_EDGE('',*,*,#7847,.F.);
#10591=ORIENTED_EDGE('',*,*,#7848,.T.);
#10592=ORIENTED_EDGE('',*,*,#7849,.T.);
#10593=ORIENTED_EDGE('',*,*,#7845,.F.);
#10594=ORIENTED_EDGE('',*,*,#7850,.F.);
#10595=ORIENTED_EDGE('',*,*,#7851,.T.);
#10596=ORIENTED_EDGE('',*,*,#7852,.T.);
#10597=ORIENTED_EDGE('',*,*,#7848,.F.);
#10598=ORIENTED_EDGE('',*,*,#7853,.F.);
#10599=ORIENTED_EDGE('',*,*,#7854,.T.);
#10600=ORIENTED_EDGE('',*,*,#7855,.T.);
#10601=ORIENTED_EDGE('',*,*,#7851,.F.);
#10602=ORIENTED_EDGE('',*,*,#7856,.F.);
#10603=ORIENTED_EDGE('',*,*,#7857,.T.);
#10604=ORIENTED_EDGE('',*,*,#7858,.T.);
#10605=ORIENTED_EDGE('',*,*,#7854,.F.);
#10606=ORIENTED_EDGE('',*,*,#7859,.F.);
#10607=ORIENTED_EDGE('',*,*,#7860,.T.);
#10608=ORIENTED_EDGE('',*,*,#7861,.T.);
#10609=ORIENTED_EDGE('',*,*,#7857,.F.);
#10610=ORIENTED_EDGE('',*,*,#7862,.F.);
#10611=ORIENTED_EDGE('',*,*,#7863,.T.);
#10612=ORIENTED_EDGE('',*,*,#7864,.T.);
#10613=ORIENTED_EDGE('',*,*,#7860,.F.);
#10614=ORIENTED_EDGE('',*,*,#7865,.F.);
#10615=ORIENTED_EDGE('',*,*,#7866,.T.);
#10616=ORIENTED_EDGE('',*,*,#7867,.T.);
#10617=ORIENTED_EDGE('',*,*,#7863,.F.);
#10618=ORIENTED_EDGE('',*,*,#7868,.F.);
#10619=ORIENTED_EDGE('',*,*,#7869,.T.);
#10620=ORIENTED_EDGE('',*,*,#7870,.T.);
#10621=ORIENTED_EDGE('',*,*,#7866,.F.);
#10622=ORIENTED_EDGE('',*,*,#7871,.F.);
#10623=ORIENTED_EDGE('',*,*,#7872,.F.);
#10624=ORIENTED_EDGE('',*,*,#7873,.F.);
#10625=ORIENTED_EDGE('',*,*,#7874,.F.);
#10626=ORIENTED_EDGE('',*,*,#7875,.T.);
#10627=ORIENTED_EDGE('',*,*,#7631,.F.);
#10628=ORIENTED_EDGE('',*,*,#7876,.T.);
#10629=ORIENTED_EDGE('',*,*,#7756,.T.);
#10630=ORIENTED_EDGE('',*,*,#7877,.T.);
#10631=ORIENTED_EDGE('',*,*,#7634,.F.);
#10632=ORIENTED_EDGE('',*,*,#7872,.T.);
#10633=ORIENTED_EDGE('',*,*,#7878,.T.);
#10634=ORIENTED_EDGE('',*,*,#7869,.F.);
#10635=ORIENTED_EDGE('',*,*,#7879,.F.);
#10636=ORIENTED_EDGE('',*,*,#7877,.F.);
#10637=ORIENTED_EDGE('',*,*,#7755,.F.);
#10638=ORIENTED_EDGE('',*,*,#7759,.F.);
#10639=ORIENTED_EDGE('',*,*,#7762,.F.);
#10640=ORIENTED_EDGE('',*,*,#7765,.F.);
#10641=ORIENTED_EDGE('',*,*,#7768,.F.);
#10642=ORIENTED_EDGE('',*,*,#7771,.F.);
#10643=ORIENTED_EDGE('',*,*,#7774,.F.);
#10644=ORIENTED_EDGE('',*,*,#7777,.F.);
#10645=ORIENTED_EDGE('',*,*,#7780,.F.);
#10646=ORIENTED_EDGE('',*,*,#7783,.F.);
#10647=ORIENTED_EDGE('',*,*,#7786,.F.);
#10648=ORIENTED_EDGE('',*,*,#7789,.F.);
#10649=ORIENTED_EDGE('',*,*,#7792,.F.);
#10650=ORIENTED_EDGE('',*,*,#7795,.F.);
#10651=ORIENTED_EDGE('',*,*,#7798,.F.);
#10652=ORIENTED_EDGE('',*,*,#7801,.F.);
#10653=ORIENTED_EDGE('',*,*,#7804,.F.);
#10654=ORIENTED_EDGE('',*,*,#7807,.F.);
#10655=ORIENTED_EDGE('',*,*,#7810,.F.);
#10656=ORIENTED_EDGE('',*,*,#7813,.F.);
#10657=ORIENTED_EDGE('',*,*,#7816,.F.);
#10658=ORIENTED_EDGE('',*,*,#7819,.F.);
#10659=ORIENTED_EDGE('',*,*,#7822,.F.);
#10660=ORIENTED_EDGE('',*,*,#7825,.F.);
#10661=ORIENTED_EDGE('',*,*,#7828,.F.);
#10662=ORIENTED_EDGE('',*,*,#7831,.F.);
#10663=ORIENTED_EDGE('',*,*,#7834,.F.);
#10664=ORIENTED_EDGE('',*,*,#7837,.F.);
#10665=ORIENTED_EDGE('',*,*,#7840,.F.);
#10666=ORIENTED_EDGE('',*,*,#7843,.F.);
#10667=ORIENTED_EDGE('',*,*,#7846,.F.);
#10668=ORIENTED_EDGE('',*,*,#7849,.F.);
#10669=ORIENTED_EDGE('',*,*,#7852,.F.);
#10670=ORIENTED_EDGE('',*,*,#7855,.F.);
#10671=ORIENTED_EDGE('',*,*,#7858,.F.);
#10672=ORIENTED_EDGE('',*,*,#7861,.F.);
#10673=ORIENTED_EDGE('',*,*,#7864,.F.);
#10674=ORIENTED_EDGE('',*,*,#7867,.F.);
#10675=ORIENTED_EDGE('',*,*,#7870,.F.);
#10676=ORIENTED_EDGE('',*,*,#7878,.F.);
#10677=ORIENTED_EDGE('',*,*,#7875,.F.);
#10678=ORIENTED_EDGE('',*,*,#7880,.F.);
#10679=ORIENTED_EDGE('',*,*,#7751,.F.);
#10680=ORIENTED_EDGE('',*,*,#7881,.F.);
#10681=ORIENTED_EDGE('',*,*,#7749,.F.);
#10682=ORIENTED_EDGE('',*,*,#7746,.F.);
#10683=ORIENTED_EDGE('',*,*,#7743,.F.);
#10684=ORIENTED_EDGE('',*,*,#7740,.F.);
#10685=ORIENTED_EDGE('',*,*,#7737,.F.);
#10686=ORIENTED_EDGE('',*,*,#7734,.F.);
#10687=ORIENTED_EDGE('',*,*,#7731,.F.);
#10688=ORIENTED_EDGE('',*,*,#7728,.F.);
#10689=ORIENTED_EDGE('',*,*,#7725,.F.);
#10690=ORIENTED_EDGE('',*,*,#7722,.F.);
#10691=ORIENTED_EDGE('',*,*,#7719,.F.);
#10692=ORIENTED_EDGE('',*,*,#7716,.F.);
#10693=ORIENTED_EDGE('',*,*,#7713,.F.);
#10694=ORIENTED_EDGE('',*,*,#7710,.F.);
#10695=ORIENTED_EDGE('',*,*,#7707,.F.);
#10696=ORIENTED_EDGE('',*,*,#7704,.F.);
#10697=ORIENTED_EDGE('',*,*,#7701,.F.);
#10698=ORIENTED_EDGE('',*,*,#7698,.F.);
#10699=ORIENTED_EDGE('',*,*,#7695,.F.);
#10700=ORIENTED_EDGE('',*,*,#7692,.F.);
#10701=ORIENTED_EDGE('',*,*,#7689,.F.);
#10702=ORIENTED_EDGE('',*,*,#7686,.F.);
#10703=ORIENTED_EDGE('',*,*,#7683,.F.);
#10704=ORIENTED_EDGE('',*,*,#7680,.F.);
#10705=ORIENTED_EDGE('',*,*,#7677,.F.);
#10706=ORIENTED_EDGE('',*,*,#7674,.F.);
#10707=ORIENTED_EDGE('',*,*,#7671,.F.);
#10708=ORIENTED_EDGE('',*,*,#7668,.F.);
#10709=ORIENTED_EDGE('',*,*,#7665,.F.);
#10710=ORIENTED_EDGE('',*,*,#7662,.F.);
#10711=ORIENTED_EDGE('',*,*,#7659,.F.);
#10712=ORIENTED_EDGE('',*,*,#7656,.F.);
#10713=ORIENTED_EDGE('',*,*,#7653,.F.);
#10714=ORIENTED_EDGE('',*,*,#7650,.F.);
#10715=ORIENTED_EDGE('',*,*,#7647,.F.);
#10716=ORIENTED_EDGE('',*,*,#7644,.F.);
#10717=ORIENTED_EDGE('',*,*,#7641,.F.);
#10718=ORIENTED_EDGE('',*,*,#7638,.F.);
#10719=ORIENTED_EDGE('',*,*,#7635,.F.);
#10720=ORIENTED_EDGE('',*,*,#7876,.F.);
#10721=ORIENTED_EDGE('',*,*,#7630,.F.);
#10722=ORIENTED_EDGE('',*,*,#7637,.F.);
#10723=ORIENTED_EDGE('',*,*,#7640,.F.);
#10724=ORIENTED_EDGE('',*,*,#7643,.F.);
#10725=ORIENTED_EDGE('',*,*,#7646,.F.);
#10726=ORIENTED_EDGE('',*,*,#7649,.F.);
#10727=ORIENTED_EDGE('',*,*,#7652,.F.);
#10728=ORIENTED_EDGE('',*,*,#7655,.F.);
#10729=ORIENTED_EDGE('',*,*,#7658,.F.);
#10730=ORIENTED_EDGE('',*,*,#7661,.F.);
#10731=ORIENTED_EDGE('',*,*,#7664,.F.);
#10732=ORIENTED_EDGE('',*,*,#7667,.F.);
#10733=ORIENTED_EDGE('',*,*,#7670,.F.);
#10734=ORIENTED_EDGE('',*,*,#7673,.F.);
#10735=ORIENTED_EDGE('',*,*,#7676,.F.);
#10736=ORIENTED_EDGE('',*,*,#7679,.F.);
#10737=ORIENTED_EDGE('',*,*,#7682,.F.);
#10738=ORIENTED_EDGE('',*,*,#7685,.F.);
#10739=ORIENTED_EDGE('',*,*,#7688,.F.);
#10740=ORIENTED_EDGE('',*,*,#7691,.F.);
#10741=ORIENTED_EDGE('',*,*,#7694,.F.);
#10742=ORIENTED_EDGE('',*,*,#7697,.F.);
#10743=ORIENTED_EDGE('',*,*,#7700,.F.);
#10744=ORIENTED_EDGE('',*,*,#7703,.F.);
#10745=ORIENTED_EDGE('',*,*,#7706,.F.);
#10746=ORIENTED_EDGE('',*,*,#7709,.F.);
#10747=ORIENTED_EDGE('',*,*,#7712,.F.);
#10748=ORIENTED_EDGE('',*,*,#7715,.F.);
#10749=ORIENTED_EDGE('',*,*,#7718,.F.);
#10750=ORIENTED_EDGE('',*,*,#7721,.F.);
#10751=ORIENTED_EDGE('',*,*,#7724,.F.);
#10752=ORIENTED_EDGE('',*,*,#7727,.F.);
#10753=ORIENTED_EDGE('',*,*,#7730,.F.);
#10754=ORIENTED_EDGE('',*,*,#7733,.F.);
#10755=ORIENTED_EDGE('',*,*,#7736,.F.);
#10756=ORIENTED_EDGE('',*,*,#7739,.F.);
#10757=ORIENTED_EDGE('',*,*,#7742,.F.);
#10758=ORIENTED_EDGE('',*,*,#7745,.F.);
#10759=ORIENTED_EDGE('',*,*,#7748,.F.);
#10760=ORIENTED_EDGE('',*,*,#7882,.F.);
#10761=ORIENTED_EDGE('',*,*,#7753,.F.);
#10762=ORIENTED_EDGE('',*,*,#7883,.F.);
#10763=ORIENTED_EDGE('',*,*,#7873,.T.);
#10764=ORIENTED_EDGE('',*,*,#7879,.T.);
#10765=ORIENTED_EDGE('',*,*,#7871,.T.);
#10766=ORIENTED_EDGE('',*,*,#7868,.T.);
#10767=ORIENTED_EDGE('',*,*,#7865,.T.);
#10768=ORIENTED_EDGE('',*,*,#7862,.T.);
#10769=ORIENTED_EDGE('',*,*,#7859,.T.);
#10770=ORIENTED_EDGE('',*,*,#7856,.T.);
#10771=ORIENTED_EDGE('',*,*,#7853,.T.);
#10772=ORIENTED_EDGE('',*,*,#7850,.T.);
#10773=ORIENTED_EDGE('',*,*,#7847,.T.);
#10774=ORIENTED_EDGE('',*,*,#7844,.T.);
#10775=ORIENTED_EDGE('',*,*,#7841,.T.);
#10776=ORIENTED_EDGE('',*,*,#7838,.T.);
#10777=ORIENTED_EDGE('',*,*,#7835,.T.);
#10778=ORIENTED_EDGE('',*,*,#7832,.T.);
#10779=ORIENTED_EDGE('',*,*,#7829,.T.);
#10780=ORIENTED_EDGE('',*,*,#7826,.T.);
#10781=ORIENTED_EDGE('',*,*,#7823,.T.);
#10782=ORIENTED_EDGE('',*,*,#7820,.T.);
#10783=ORIENTED_EDGE('',*,*,#7817,.T.);
#10784=ORIENTED_EDGE('',*,*,#7814,.T.);
#10785=ORIENTED_EDGE('',*,*,#7811,.T.);
#10786=ORIENTED_EDGE('',*,*,#7808,.T.);
#10787=ORIENTED_EDGE('',*,*,#7805,.T.);
#10788=ORIENTED_EDGE('',*,*,#7802,.T.);
#10789=ORIENTED_EDGE('',*,*,#7799,.T.);
#10790=ORIENTED_EDGE('',*,*,#7796,.T.);
#10791=ORIENTED_EDGE('',*,*,#7793,.T.);
#10792=ORIENTED_EDGE('',*,*,#7790,.T.);
#10793=ORIENTED_EDGE('',*,*,#7787,.T.);
#10794=ORIENTED_EDGE('',*,*,#7784,.T.);
#10795=ORIENTED_EDGE('',*,*,#7781,.T.);
#10796=ORIENTED_EDGE('',*,*,#7778,.T.);
#10797=ORIENTED_EDGE('',*,*,#7775,.T.);
#10798=ORIENTED_EDGE('',*,*,#7772,.T.);
#10799=ORIENTED_EDGE('',*,*,#7769,.T.);
#10800=ORIENTED_EDGE('',*,*,#7766,.T.);
#10801=ORIENTED_EDGE('',*,*,#7763,.T.);
#10802=ORIENTED_EDGE('',*,*,#7760,.T.);
#10803=ORIENTED_EDGE('',*,*,#7757,.T.);
#10804=ORIENTED_EDGE('',*,*,#7750,.T.);
#10805=ORIENTED_EDGE('',*,*,#7882,.T.);
#10806=ORIENTED_EDGE('',*,*,#7747,.F.);
#10807=ORIENTED_EDGE('',*,*,#7881,.T.);
#10808=ORIENTED_EDGE('',*,*,#7633,.F.);
#10809=ORIENTED_EDGE('',*,*,#7884,.F.);
#10810=ORIENTED_EDGE('',*,*,#7474,.F.);
#10811=ORIENTED_EDGE('',*,*,#7885,.T.);
#10812=ORIENTED_EDGE('',*,*,#7554,.T.);
#10813=ORIENTED_EDGE('',*,*,#7886,.T.);
#10814=ORIENTED_EDGE('',*,*,#7477,.F.);
#10815=ORIENTED_EDGE('',*,*,#7625,.T.);
#10816=ORIENTED_EDGE('',*,*,#7887,.T.);
#10817=ORIENTED_EDGE('',*,*,#7622,.F.);
#10818=ORIENTED_EDGE('',*,*,#7888,.F.);
#10819=ORIENTED_EDGE('',*,*,#7886,.F.);
#10820=ORIENTED_EDGE('',*,*,#7553,.F.);
#10821=ORIENTED_EDGE('',*,*,#7557,.F.);
#10822=ORIENTED_EDGE('',*,*,#7560,.F.);
#10823=ORIENTED_EDGE('',*,*,#7563,.F.);
#10824=ORIENTED_EDGE('',*,*,#7566,.F.);
#10825=ORIENTED_EDGE('',*,*,#7569,.F.);
#10826=ORIENTED_EDGE('',*,*,#7572,.F.);
#10827=ORIENTED_EDGE('',*,*,#7575,.F.);
#10828=ORIENTED_EDGE('',*,*,#7578,.F.);
#10829=ORIENTED_EDGE('',*,*,#7581,.F.);
#10830=ORIENTED_EDGE('',*,*,#7584,.F.);
#10831=ORIENTED_EDGE('',*,*,#7587,.F.);
#10832=ORIENTED_EDGE('',*,*,#7590,.F.);
#10833=ORIENTED_EDGE('',*,*,#7593,.F.);
#10834=ORIENTED_EDGE('',*,*,#7596,.F.);
#10835=ORIENTED_EDGE('',*,*,#7599,.F.);
#10836=ORIENTED_EDGE('',*,*,#7602,.F.);
#10837=ORIENTED_EDGE('',*,*,#7605,.F.);
#10838=ORIENTED_EDGE('',*,*,#7608,.F.);
#10839=ORIENTED_EDGE('',*,*,#7611,.F.);
#10840=ORIENTED_EDGE('',*,*,#7614,.F.);
#10841=ORIENTED_EDGE('',*,*,#7617,.F.);
#10842=ORIENTED_EDGE('',*,*,#7620,.F.);
#10843=ORIENTED_EDGE('',*,*,#7623,.F.);
#10844=ORIENTED_EDGE('',*,*,#7887,.F.);
#10845=ORIENTED_EDGE('',*,*,#7628,.F.);
#10846=ORIENTED_EDGE('',*,*,#7889,.F.);
#10847=ORIENTED_EDGE('',*,*,#7549,.F.);
#10848=ORIENTED_EDGE('',*,*,#7890,.F.);
#10849=ORIENTED_EDGE('',*,*,#7547,.F.);
#10850=ORIENTED_EDGE('',*,*,#7544,.F.);
#10851=ORIENTED_EDGE('',*,*,#7541,.F.);
#10852=ORIENTED_EDGE('',*,*,#7538,.F.);
#10853=ORIENTED_EDGE('',*,*,#7535,.F.);
#10854=ORIENTED_EDGE('',*,*,#7532,.F.);
#10855=ORIENTED_EDGE('',*,*,#7529,.F.);
#10856=ORIENTED_EDGE('',*,*,#7526,.F.);
#10857=ORIENTED_EDGE('',*,*,#7523,.F.);
#10858=ORIENTED_EDGE('',*,*,#7520,.F.);
#10859=ORIENTED_EDGE('',*,*,#7517,.F.);
#10860=ORIENTED_EDGE('',*,*,#7514,.F.);
#10861=ORIENTED_EDGE('',*,*,#7511,.F.);
#10862=ORIENTED_EDGE('',*,*,#7508,.F.);
#10863=ORIENTED_EDGE('',*,*,#7505,.F.);
#10864=ORIENTED_EDGE('',*,*,#7502,.F.);
#10865=ORIENTED_EDGE('',*,*,#7499,.F.);
#10866=ORIENTED_EDGE('',*,*,#7496,.F.);
#10867=ORIENTED_EDGE('',*,*,#7493,.F.);
#10868=ORIENTED_EDGE('',*,*,#7490,.F.);
#10869=ORIENTED_EDGE('',*,*,#7487,.F.);
#10870=ORIENTED_EDGE('',*,*,#7484,.F.);
#10871=ORIENTED_EDGE('',*,*,#7481,.F.);
#10872=ORIENTED_EDGE('',*,*,#7478,.F.);
#10873=ORIENTED_EDGE('',*,*,#7885,.F.);
#10874=ORIENTED_EDGE('',*,*,#7473,.F.);
#10875=ORIENTED_EDGE('',*,*,#7480,.F.);
#10876=ORIENTED_EDGE('',*,*,#7483,.F.);
#10877=ORIENTED_EDGE('',*,*,#7486,.F.);
#10878=ORIENTED_EDGE('',*,*,#7489,.F.);
#10879=ORIENTED_EDGE('',*,*,#7492,.F.);
#10880=ORIENTED_EDGE('',*,*,#7495,.F.);
#10881=ORIENTED_EDGE('',*,*,#7498,.F.);
#10882=ORIENTED_EDGE('',*,*,#7501,.F.);
#10883=ORIENTED_EDGE('',*,*,#7504,.F.);
#10884=ORIENTED_EDGE('',*,*,#7507,.F.);
#10885=ORIENTED_EDGE('',*,*,#7510,.F.);
#10886=ORIENTED_EDGE('',*,*,#7513,.F.);
#10887=ORIENTED_EDGE('',*,*,#7516,.F.);
#10888=ORIENTED_EDGE('',*,*,#7519,.F.);
#10889=ORIENTED_EDGE('',*,*,#7522,.F.);
#10890=ORIENTED_EDGE('',*,*,#7525,.F.);
#10891=ORIENTED_EDGE('',*,*,#7528,.F.);
#10892=ORIENTED_EDGE('',*,*,#7531,.F.);
#10893=ORIENTED_EDGE('',*,*,#7534,.F.);
#10894=ORIENTED_EDGE('',*,*,#7537,.F.);
#10895=ORIENTED_EDGE('',*,*,#7540,.F.);
#10896=ORIENTED_EDGE('',*,*,#7543,.F.);
#10897=ORIENTED_EDGE('',*,*,#7546,.F.);
#10898=ORIENTED_EDGE('',*,*,#7891,.F.);
#10899=ORIENTED_EDGE('',*,*,#7551,.F.);
#10900=ORIENTED_EDGE('',*,*,#7892,.F.);
#10901=ORIENTED_EDGE('',*,*,#7626,.T.);
#10902=ORIENTED_EDGE('',*,*,#7888,.T.);
#10903=ORIENTED_EDGE('',*,*,#7624,.T.);
#10904=ORIENTED_EDGE('',*,*,#7621,.T.);
#10905=ORIENTED_EDGE('',*,*,#7618,.T.);
#10906=ORIENTED_EDGE('',*,*,#7615,.T.);
#10907=ORIENTED_EDGE('',*,*,#7612,.T.);
#10908=ORIENTED_EDGE('',*,*,#7609,.T.);
#10909=ORIENTED_EDGE('',*,*,#7606,.T.);
#10910=ORIENTED_EDGE('',*,*,#7603,.T.);
#10911=ORIENTED_EDGE('',*,*,#7600,.T.);
#10912=ORIENTED_EDGE('',*,*,#7597,.T.);
#10913=ORIENTED_EDGE('',*,*,#7594,.T.);
#10914=ORIENTED_EDGE('',*,*,#7591,.T.);
#10915=ORIENTED_EDGE('',*,*,#7588,.T.);
#10916=ORIENTED_EDGE('',*,*,#7585,.T.);
#10917=ORIENTED_EDGE('',*,*,#7582,.T.);
#10918=ORIENTED_EDGE('',*,*,#7579,.T.);
#10919=ORIENTED_EDGE('',*,*,#7576,.T.);
#10920=ORIENTED_EDGE('',*,*,#7573,.T.);
#10921=ORIENTED_EDGE('',*,*,#7570,.T.);
#10922=ORIENTED_EDGE('',*,*,#7567,.T.);
#10923=ORIENTED_EDGE('',*,*,#7564,.T.);
#10924=ORIENTED_EDGE('',*,*,#7561,.T.);
#10925=ORIENTED_EDGE('',*,*,#7558,.T.);
#10926=ORIENTED_EDGE('',*,*,#7555,.T.);
#10927=ORIENTED_EDGE('',*,*,#7548,.T.);
#10928=ORIENTED_EDGE('',*,*,#7891,.T.);
#10929=ORIENTED_EDGE('',*,*,#7545,.F.);
#10930=ORIENTED_EDGE('',*,*,#7890,.T.);
#10931=ORIENTED_EDGE('',*,*,#7476,.F.);
#10932=ORIENTED_EDGE('',*,*,#7893,.F.);
#10933=ORIENTED_EDGE('',*,*,#7894,.T.);
#10934=ORIENTED_EDGE('',*,*,#7895,.T.);
#10935=ORIENTED_EDGE('',*,*,#7896,.T.);
#10936=ORIENTED_EDGE('',*,*,#7897,.T.);
#10937=ORIENTED_EDGE('',*,*,#7895,.F.);
#10938=ORIENTED_EDGE('',*,*,#7898,.F.);
#10939=ORIENTED_EDGE('',*,*,#7899,.F.);
#10940=ORIENTED_EDGE('',*,*,#7900,.F.);
#10941=ORIENTED_EDGE('',*,*,#7894,.F.);
#10942=ORIENTED_EDGE('',*,*,#7901,.T.);
#10943=ORIENTED_EDGE('',*,*,#7902,.F.);
#10944=ORIENTED_EDGE('',*,*,#7903,.T.);
#10945=ORIENTED_EDGE('',*,*,#7904,.F.);
#10946=ORIENTED_EDGE('',*,*,#7905,.T.);
#10947=ORIENTED_EDGE('',*,*,#7906,.F.);
#10948=ORIENTED_EDGE('',*,*,#7907,.T.);
#10949=ORIENTED_EDGE('',*,*,#7908,.F.);
#10950=ORIENTED_EDGE('',*,*,#7909,.T.);
#10951=ORIENTED_EDGE('',*,*,#7910,.F.);
#10952=ORIENTED_EDGE('',*,*,#7911,.T.);
#10953=ORIENTED_EDGE('',*,*,#7912,.F.);
#10954=ORIENTED_EDGE('',*,*,#7913,.T.);
#10955=ORIENTED_EDGE('',*,*,#7914,.F.);
#10956=ORIENTED_EDGE('',*,*,#7915,.T.);
#10957=ORIENTED_EDGE('',*,*,#7916,.F.);
#10958=ORIENTED_EDGE('',*,*,#7917,.T.);
#10959=ORIENTED_EDGE('',*,*,#7918,.F.);
#10960=ORIENTED_EDGE('',*,*,#7919,.T.);
#10961=ORIENTED_EDGE('',*,*,#7920,.F.);
#10962=ORIENTED_EDGE('',*,*,#7921,.T.);
#10963=ORIENTED_EDGE('',*,*,#7922,.F.);
#10964=ORIENTED_EDGE('',*,*,#7923,.T.);
#10965=ORIENTED_EDGE('',*,*,#7924,.F.);
#10966=ORIENTED_EDGE('',*,*,#7925,.T.);
#10967=ORIENTED_EDGE('',*,*,#7926,.F.);
#10968=ORIENTED_EDGE('',*,*,#7927,.T.);
#10969=ORIENTED_EDGE('',*,*,#7928,.F.);
#10970=ORIENTED_EDGE('',*,*,#7929,.T.);
#10971=ORIENTED_EDGE('',*,*,#7930,.F.);
#10972=ORIENTED_EDGE('',*,*,#7931,.T.);
#10973=ORIENTED_EDGE('',*,*,#7932,.F.);
#10974=ORIENTED_EDGE('',*,*,#7933,.T.);
#10975=ORIENTED_EDGE('',*,*,#7934,.F.);
#10976=ORIENTED_EDGE('',*,*,#7935,.T.);
#10977=ORIENTED_EDGE('',*,*,#7936,.F.);
#10978=ORIENTED_EDGE('',*,*,#7937,.T.);
#10979=ORIENTED_EDGE('',*,*,#7938,.F.);
#10980=ORIENTED_EDGE('',*,*,#7939,.T.);
#10981=ORIENTED_EDGE('',*,*,#7940,.F.);
#10982=ORIENTED_EDGE('',*,*,#7941,.T.);
#10983=ORIENTED_EDGE('',*,*,#7942,.F.);
#10984=ORIENTED_EDGE('',*,*,#7943,.T.);
#10985=ORIENTED_EDGE('',*,*,#7944,.F.);
#10986=ORIENTED_EDGE('',*,*,#7945,.T.);
#10987=ORIENTED_EDGE('',*,*,#7946,.F.);
#10988=ORIENTED_EDGE('',*,*,#7947,.T.);
#10989=ORIENTED_EDGE('',*,*,#7948,.F.);
#10990=ORIENTED_EDGE('',*,*,#7949,.T.);
#10991=ORIENTED_EDGE('',*,*,#7950,.F.);
#10992=ORIENTED_EDGE('',*,*,#7951,.T.);
#10993=ORIENTED_EDGE('',*,*,#7952,.F.);
#10994=ORIENTED_EDGE('',*,*,#7953,.T.);
#10995=ORIENTED_EDGE('',*,*,#7954,.F.);
#10996=ORIENTED_EDGE('',*,*,#7955,.T.);
#10997=ORIENTED_EDGE('',*,*,#7956,.F.);
#10998=ORIENTED_EDGE('',*,*,#7957,.T.);
#10999=ORIENTED_EDGE('',*,*,#7958,.F.);
#11000=ORIENTED_EDGE('',*,*,#7959,.T.);
#11001=ORIENTED_EDGE('',*,*,#7960,.F.);
#11002=ORIENTED_EDGE('',*,*,#7961,.T.);
#11003=ORIENTED_EDGE('',*,*,#7962,.F.);
#11004=ORIENTED_EDGE('',*,*,#7963,.T.);
#11005=ORIENTED_EDGE('',*,*,#7964,.F.);
#11006=ORIENTED_EDGE('',*,*,#7965,.T.);
#11007=ORIENTED_EDGE('',*,*,#7966,.F.);
#11008=ORIENTED_EDGE('',*,*,#7967,.T.);
#11009=ORIENTED_EDGE('',*,*,#7968,.F.);
#11010=ORIENTED_EDGE('',*,*,#7969,.T.);
#11011=ORIENTED_EDGE('',*,*,#7970,.F.);
#11012=ORIENTED_EDGE('',*,*,#7898,.T.);
#11013=ORIENTED_EDGE('',*,*,#7892,.T.);
#11014=ORIENTED_EDGE('',*,*,#7550,.T.);
#11015=ORIENTED_EDGE('',*,*,#7889,.T.);
#11016=ORIENTED_EDGE('',*,*,#7627,.T.);
#11017=ORIENTED_EDGE('',*,*,#7971,.T.);
#11018=ORIENTED_EDGE('',*,*,#7972,.T.);
#11019=ORIENTED_EDGE('',*,*,#7973,.T.);
#11020=ORIENTED_EDGE('',*,*,#7974,.T.);
#11021=ORIENTED_EDGE('',*,*,#7975,.T.);
#11022=ORIENTED_EDGE('',*,*,#7976,.T.);
#11023=ORIENTED_EDGE('',*,*,#7902,.T.);
#11024=ORIENTED_EDGE('',*,*,#7977,.T.);
#11025=ORIENTED_EDGE('',*,*,#7976,.F.);
#11026=ORIENTED_EDGE('',*,*,#7978,.F.);
#11027=ORIENTED_EDGE('',*,*,#7979,.F.);
#11028=ORIENTED_EDGE('',*,*,#7903,.F.);
#11029=ORIENTED_EDGE('',*,*,#7980,.T.);
#11030=ORIENTED_EDGE('',*,*,#7981,.T.);
#11031=ORIENTED_EDGE('',*,*,#7904,.T.);
#11032=ORIENTED_EDGE('',*,*,#7979,.T.);
#11033=ORIENTED_EDGE('',*,*,#7981,.F.);
#11034=ORIENTED_EDGE('',*,*,#7982,.F.);
#11035=ORIENTED_EDGE('',*,*,#7983,.F.);
#11036=ORIENTED_EDGE('',*,*,#7905,.F.);
#11037=ORIENTED_EDGE('',*,*,#7984,.T.);
#11038=ORIENTED_EDGE('',*,*,#7985,.T.);
#11039=ORIENTED_EDGE('',*,*,#7906,.T.);
#11040=ORIENTED_EDGE('',*,*,#7983,.T.);
#11041=ORIENTED_EDGE('',*,*,#7985,.F.);
#11042=ORIENTED_EDGE('',*,*,#7986,.F.);
#11043=ORIENTED_EDGE('',*,*,#7987,.F.);
#11044=ORIENTED_EDGE('',*,*,#7907,.F.);
#11045=ORIENTED_EDGE('',*,*,#7988,.T.);
#11046=ORIENTED_EDGE('',*,*,#7989,.T.);
#11047=ORIENTED_EDGE('',*,*,#7908,.T.);
#11048=ORIENTED_EDGE('',*,*,#7987,.T.);
#11049=ORIENTED_EDGE('',*,*,#7989,.F.);
#11050=ORIENTED_EDGE('',*,*,#7990,.F.);
#11051=ORIENTED_EDGE('',*,*,#7991,.F.);
#11052=ORIENTED_EDGE('',*,*,#7909,.F.);
#11053=ORIENTED_EDGE('',*,*,#7910,.T.);
#11054=ORIENTED_EDGE('',*,*,#7991,.T.);
#11055=ORIENTED_EDGE('',*,*,#7992,.T.);
#11056=ORIENTED_EDGE('',*,*,#7993,.T.);
#11057=ORIENTED_EDGE('',*,*,#7912,.T.);
#11058=ORIENTED_EDGE('',*,*,#7994,.T.);
#11059=ORIENTED_EDGE('',*,*,#7995,.T.);
#11060=ORIENTED_EDGE('',*,*,#7996,.T.);
#11061=ORIENTED_EDGE('',*,*,#7996,.F.);
#11062=ORIENTED_EDGE('',*,*,#7997,.F.);
#11063=ORIENTED_EDGE('',*,*,#7998,.F.);
#11064=ORIENTED_EDGE('',*,*,#7913,.F.);
#11065=ORIENTED_EDGE('',*,*,#7914,.T.);
#11066=ORIENTED_EDGE('',*,*,#7998,.T.);
#11067=ORIENTED_EDGE('',*,*,#7999,.T.);
#11068=ORIENTED_EDGE('',*,*,#8000,.T.);
#11069=ORIENTED_EDGE('',*,*,#7916,.T.);
#11070=ORIENTED_EDGE('',*,*,#8001,.T.);
#11071=ORIENTED_EDGE('',*,*,#8002,.T.);
#11072=ORIENTED_EDGE('',*,*,#8003,.T.);
#11073=ORIENTED_EDGE('',*,*,#8003,.F.);
#11074=ORIENTED_EDGE('',*,*,#8004,.F.);
#11075=ORIENTED_EDGE('',*,*,#8005,.F.);
#11076=ORIENTED_EDGE('',*,*,#7917,.F.);
#11077=ORIENTED_EDGE('',*,*,#7918,.T.);
#11078=ORIENTED_EDGE('',*,*,#8005,.T.);
#11079=ORIENTED_EDGE('',*,*,#8006,.T.);
#11080=ORIENTED_EDGE('',*,*,#8007,.T.);
#11081=ORIENTED_EDGE('',*,*,#8008,.T.);
#11082=ORIENTED_EDGE('',*,*,#8009,.T.);
#11083=ORIENTED_EDGE('',*,*,#7920,.T.);
#11084=ORIENTED_EDGE('',*,*,#8010,.T.);
#11085=ORIENTED_EDGE('',*,*,#8009,.F.);
#11086=ORIENTED_EDGE('',*,*,#8011,.F.);
#11087=ORIENTED_EDGE('',*,*,#8012,.F.);
#11088=ORIENTED_EDGE('',*,*,#7921,.F.);
#11089=ORIENTED_EDGE('',*,*,#8013,.T.);
#11090=ORIENTED_EDGE('',*,*,#8014,.T.);
#11091=ORIENTED_EDGE('',*,*,#7922,.T.);
#11092=ORIENTED_EDGE('',*,*,#8012,.T.);
#11093=ORIENTED_EDGE('',*,*,#8014,.F.);
#11094=ORIENTED_EDGE('',*,*,#8015,.F.);
#11095=ORIENTED_EDGE('',*,*,#8016,.F.);
#11096=ORIENTED_EDGE('',*,*,#7923,.F.);
#11097=ORIENTED_EDGE('',*,*,#8017,.T.);
#11098=ORIENTED_EDGE('',*,*,#8018,.T.);
#11099=ORIENTED_EDGE('',*,*,#7924,.T.);
#11100=ORIENTED_EDGE('',*,*,#8016,.T.);
#11101=ORIENTED_EDGE('',*,*,#8018,.F.);
#11102=ORIENTED_EDGE('',*,*,#8019,.F.);
#11103=ORIENTED_EDGE('',*,*,#8020,.F.);
#11104=ORIENTED_EDGE('',*,*,#7925,.F.);
#11105=ORIENTED_EDGE('',*,*,#8021,.T.);
#11106=ORIENTED_EDGE('',*,*,#8022,.T.);
#11107=ORIENTED_EDGE('',*,*,#7926,.T.);
#11108=ORIENTED_EDGE('',*,*,#8020,.T.);
#11109=ORIENTED_EDGE('',*,*,#8022,.F.);
#11110=ORIENTED_EDGE('',*,*,#8023,.F.);
#11111=ORIENTED_EDGE('',*,*,#8024,.F.);
#11112=ORIENTED_EDGE('',*,*,#7927,.F.);
#11113=ORIENTED_EDGE('',*,*,#7928,.T.);
#11114=ORIENTED_EDGE('',*,*,#8024,.T.);
#11115=ORIENTED_EDGE('',*,*,#8025,.T.);
#11116=ORIENTED_EDGE('',*,*,#8026,.T.);
#11117=ORIENTED_EDGE('',*,*,#7930,.T.);
#11118=ORIENTED_EDGE('',*,*,#8027,.T.);
#11119=ORIENTED_EDGE('',*,*,#8028,.T.);
#11120=ORIENTED_EDGE('',*,*,#8029,.T.);
#11121=ORIENTED_EDGE('',*,*,#8029,.F.);
#11122=ORIENTED_EDGE('',*,*,#8030,.F.);
#11123=ORIENTED_EDGE('',*,*,#8031,.F.);
#11124=ORIENTED_EDGE('',*,*,#7931,.F.);
#11125=ORIENTED_EDGE('',*,*,#7932,.T.);
#11126=ORIENTED_EDGE('',*,*,#8031,.T.);
#11127=ORIENTED_EDGE('',*,*,#8032,.T.);
#11128=ORIENTED_EDGE('',*,*,#8033,.T.);
#11129=ORIENTED_EDGE('',*,*,#7934,.T.);
#11130=ORIENTED_EDGE('',*,*,#8034,.T.);
#11131=ORIENTED_EDGE('',*,*,#8035,.T.);
#11132=ORIENTED_EDGE('',*,*,#8036,.T.);
#11133=ORIENTED_EDGE('',*,*,#8036,.F.);
#11134=ORIENTED_EDGE('',*,*,#8037,.F.);
#11135=ORIENTED_EDGE('',*,*,#8038,.F.);
#11136=ORIENTED_EDGE('',*,*,#7935,.F.);
#11137=ORIENTED_EDGE('',*,*,#7936,.T.);
#11138=ORIENTED_EDGE('',*,*,#8038,.T.);
#11139=ORIENTED_EDGE('',*,*,#8039,.T.);
#11140=ORIENTED_EDGE('',*,*,#8040,.T.);
#11141=ORIENTED_EDGE('',*,*,#8041,.T.);
#11142=ORIENTED_EDGE('',*,*,#8042,.T.);
#11143=ORIENTED_EDGE('',*,*,#7938,.T.);
#11144=ORIENTED_EDGE('',*,*,#8043,.T.);
#11145=ORIENTED_EDGE('',*,*,#8042,.F.);
#11146=ORIENTED_EDGE('',*,*,#8044,.F.);
#11147=ORIENTED_EDGE('',*,*,#8045,.F.);
#11148=ORIENTED_EDGE('',*,*,#7939,.F.);
#11149=ORIENTED_EDGE('',*,*,#8046,.T.);
#11150=ORIENTED_EDGE('',*,*,#8047,.T.);
#11151=ORIENTED_EDGE('',*,*,#7940,.T.);
#11152=ORIENTED_EDGE('',*,*,#8045,.T.);
#11153=ORIENTED_EDGE('',*,*,#8047,.F.);
#11154=ORIENTED_EDGE('',*,*,#8048,.F.);
#11155=ORIENTED_EDGE('',*,*,#8049,.F.);
#11156=ORIENTED_EDGE('',*,*,#7941,.F.);
#11157=ORIENTED_EDGE('',*,*,#8050,.T.);
#11158=ORIENTED_EDGE('',*,*,#8051,.T.);
#11159=ORIENTED_EDGE('',*,*,#7942,.T.);
#11160=ORIENTED_EDGE('',*,*,#8049,.T.);
#11161=ORIENTED_EDGE('',*,*,#8051,.F.);
#11162=ORIENTED_EDGE('',*,*,#8052,.F.);
#11163=ORIENTED_EDGE('',*,*,#8053,.F.);
#11164=ORIENTED_EDGE('',*,*,#7943,.F.);
#11165=ORIENTED_EDGE('',*,*,#8054,.T.);
#11166=ORIENTED_EDGE('',*,*,#8055,.T.);
#11167=ORIENTED_EDGE('',*,*,#7944,.T.);
#11168=ORIENTED_EDGE('',*,*,#8053,.T.);
#11169=ORIENTED_EDGE('',*,*,#8055,.F.);
#11170=ORIENTED_EDGE('',*,*,#8056,.F.);
#11171=ORIENTED_EDGE('',*,*,#8057,.F.);
#11172=ORIENTED_EDGE('',*,*,#7945,.F.);
#11173=ORIENTED_EDGE('',*,*,#7946,.T.);
#11174=ORIENTED_EDGE('',*,*,#8057,.T.);
#11175=ORIENTED_EDGE('',*,*,#8058,.T.);
#11176=ORIENTED_EDGE('',*,*,#8059,.T.);
#11177=ORIENTED_EDGE('',*,*,#7948,.T.);
#11178=ORIENTED_EDGE('',*,*,#8060,.T.);
#11179=ORIENTED_EDGE('',*,*,#8061,.T.);
#11180=ORIENTED_EDGE('',*,*,#8062,.T.);
#11181=ORIENTED_EDGE('',*,*,#8062,.F.);
#11182=ORIENTED_EDGE('',*,*,#8063,.F.);
#11183=ORIENTED_EDGE('',*,*,#8064,.F.);
#11184=ORIENTED_EDGE('',*,*,#7949,.F.);
#11185=ORIENTED_EDGE('',*,*,#7950,.T.);
#11186=ORIENTED_EDGE('',*,*,#8064,.T.);
#11187=ORIENTED_EDGE('',*,*,#8065,.T.);
#11188=ORIENTED_EDGE('',*,*,#8066,.T.);
#11189=ORIENTED_EDGE('',*,*,#7952,.T.);
#11190=ORIENTED_EDGE('',*,*,#8067,.T.);
#11191=ORIENTED_EDGE('',*,*,#8068,.T.);
#11192=ORIENTED_EDGE('',*,*,#8069,.T.);
#11193=ORIENTED_EDGE('',*,*,#8069,.F.);
#11194=ORIENTED_EDGE('',*,*,#8070,.F.);
#11195=ORIENTED_EDGE('',*,*,#8071,.F.);
#11196=ORIENTED_EDGE('',*,*,#7953,.F.);
#11197=ORIENTED_EDGE('',*,*,#7954,.T.);
#11198=ORIENTED_EDGE('',*,*,#8071,.T.);
#11199=ORIENTED_EDGE('',*,*,#8072,.T.);
#11200=ORIENTED_EDGE('',*,*,#8073,.T.);
#11201=ORIENTED_EDGE('',*,*,#8074,.T.);
#11202=ORIENTED_EDGE('',*,*,#8075,.T.);
#11203=ORIENTED_EDGE('',*,*,#7956,.T.);
#11204=ORIENTED_EDGE('',*,*,#8076,.T.);
#11205=ORIENTED_EDGE('',*,*,#8075,.F.);
#11206=ORIENTED_EDGE('',*,*,#8077,.F.);
#11207=ORIENTED_EDGE('',*,*,#8078,.F.);
#11208=ORIENTED_EDGE('',*,*,#7957,.F.);
#11209=ORIENTED_EDGE('',*,*,#8079,.T.);
#11210=ORIENTED_EDGE('',*,*,#8080,.T.);
#11211=ORIENTED_EDGE('',*,*,#7958,.T.);
#11212=ORIENTED_EDGE('',*,*,#8078,.T.);
#11213=ORIENTED_EDGE('',*,*,#8080,.F.);
#11214=ORIENTED_EDGE('',*,*,#8081,.F.);
#11215=ORIENTED_EDGE('',*,*,#8082,.F.);
#11216=ORIENTED_EDGE('',*,*,#7959,.F.);
#11217=ORIENTED_EDGE('',*,*,#8083,.T.);
#11218=ORIENTED_EDGE('',*,*,#8084,.T.);
#11219=ORIENTED_EDGE('',*,*,#7960,.T.);
#11220=ORIENTED_EDGE('',*,*,#8082,.T.);
#11221=ORIENTED_EDGE('',*,*,#8084,.F.);
#11222=ORIENTED_EDGE('',*,*,#8085,.F.);
#11223=ORIENTED_EDGE('',*,*,#8086,.F.);
#11224=ORIENTED_EDGE('',*,*,#7961,.F.);
#11225=ORIENTED_EDGE('',*,*,#8087,.T.);
#11226=ORIENTED_EDGE('',*,*,#8088,.T.);
#11227=ORIENTED_EDGE('',*,*,#7962,.T.);
#11228=ORIENTED_EDGE('',*,*,#8086,.T.);
#11229=ORIENTED_EDGE('',*,*,#8088,.F.);
#11230=ORIENTED_EDGE('',*,*,#8089,.F.);
#11231=ORIENTED_EDGE('',*,*,#8090,.F.);
#11232=ORIENTED_EDGE('',*,*,#7963,.F.);
#11233=ORIENTED_EDGE('',*,*,#7964,.T.);
#11234=ORIENTED_EDGE('',*,*,#8090,.T.);
#11235=ORIENTED_EDGE('',*,*,#8091,.T.);
#11236=ORIENTED_EDGE('',*,*,#8092,.T.);
#11237=ORIENTED_EDGE('',*,*,#7966,.T.);
#11238=ORIENTED_EDGE('',*,*,#8093,.T.);
#11239=ORIENTED_EDGE('',*,*,#8094,.T.);
#11240=ORIENTED_EDGE('',*,*,#8095,.T.);
#11241=ORIENTED_EDGE('',*,*,#8095,.F.);
#11242=ORIENTED_EDGE('',*,*,#8096,.F.);
#11243=ORIENTED_EDGE('',*,*,#8097,.F.);
#11244=ORIENTED_EDGE('',*,*,#7967,.F.);
#11245=ORIENTED_EDGE('',*,*,#7968,.T.);
#11246=ORIENTED_EDGE('',*,*,#8097,.T.);
#11247=ORIENTED_EDGE('',*,*,#8098,.T.);
#11248=ORIENTED_EDGE('',*,*,#8099,.T.);
#11249=ORIENTED_EDGE('',*,*,#7970,.T.);
#11250=ORIENTED_EDGE('',*,*,#8100,.T.);
#11251=ORIENTED_EDGE('',*,*,#8101,.T.);
#11252=ORIENTED_EDGE('',*,*,#7899,.T.);
#11253=ORIENTED_EDGE('',*,*,#7974,.F.);
#11254=ORIENTED_EDGE('',*,*,#8102,.T.);
#11255=ORIENTED_EDGE('',*,*,#8103,.T.);
#11256=ORIENTED_EDGE('',*,*,#8102,.F.);
#11257=ORIENTED_EDGE('',*,*,#7973,.F.);
#11258=ORIENTED_EDGE('',*,*,#8104,.T.);
#11259=ORIENTED_EDGE('',*,*,#8105,.T.);
#11260=ORIENTED_EDGE('',*,*,#8104,.F.);
#11261=ORIENTED_EDGE('',*,*,#7893,.T.);
#11262=ORIENTED_EDGE('',*,*,#8106,.T.);
#11263=ORIENTED_EDGE('',*,*,#7884,.T.);
#11264=ORIENTED_EDGE('',*,*,#8106,.F.);
#11265=ORIENTED_EDGE('',*,*,#7972,.F.);
#11266=ORIENTED_EDGE('',*,*,#8107,.T.);
#11267=ORIENTED_EDGE('',*,*,#8108,.T.);
#11268=ORIENTED_EDGE('',*,*,#8107,.F.);
#11269=ORIENTED_EDGE('',*,*,#7971,.F.);
#11270=ORIENTED_EDGE('',*,*,#8109,.T.);
#11271=ORIENTED_EDGE('',*,*,#8110,.T.);
#11272=ORIENTED_EDGE('',*,*,#8109,.F.);
#11273=ORIENTED_EDGE('',*,*,#8099,.F.);
#11274=ORIENTED_EDGE('',*,*,#8111,.F.);
#11275=ORIENTED_EDGE('',*,*,#8100,.F.);
#11276=ORIENTED_EDGE('',*,*,#7969,.F.);
#11277=ORIENTED_EDGE('',*,*,#8092,.F.);
#11278=ORIENTED_EDGE('',*,*,#8112,.F.);
#11279=ORIENTED_EDGE('',*,*,#8093,.F.);
#11280=ORIENTED_EDGE('',*,*,#7965,.F.);
#11281=ORIENTED_EDGE('',*,*,#8073,.F.);
#11282=ORIENTED_EDGE('',*,*,#8113,.F.);
#11283=ORIENTED_EDGE('',*,*,#8076,.F.);
#11284=ORIENTED_EDGE('',*,*,#7955,.F.);
#11285=ORIENTED_EDGE('',*,*,#8066,.F.);
#11286=ORIENTED_EDGE('',*,*,#8114,.F.);
#11287=ORIENTED_EDGE('',*,*,#8067,.F.);
#11288=ORIENTED_EDGE('',*,*,#7951,.F.);
#11289=ORIENTED_EDGE('',*,*,#8059,.F.);
#11290=ORIENTED_EDGE('',*,*,#8115,.F.);
#11291=ORIENTED_EDGE('',*,*,#8060,.F.);
#11292=ORIENTED_EDGE('',*,*,#7947,.F.);
#11293=ORIENTED_EDGE('',*,*,#8040,.F.);
#11294=ORIENTED_EDGE('',*,*,#8116,.F.);
#11295=ORIENTED_EDGE('',*,*,#8043,.F.);
#11296=ORIENTED_EDGE('',*,*,#7937,.F.);
#11297=ORIENTED_EDGE('',*,*,#8033,.F.);
#11298=ORIENTED_EDGE('',*,*,#8117,.F.);
#11299=ORIENTED_EDGE('',*,*,#8034,.F.);
#11300=ORIENTED_EDGE('',*,*,#7933,.F.);
#11301=ORIENTED_EDGE('',*,*,#8026,.F.);
#11302=ORIENTED_EDGE('',*,*,#8118,.F.);
#11303=ORIENTED_EDGE('',*,*,#8027,.F.);
#11304=ORIENTED_EDGE('',*,*,#7929,.F.);
#11305=ORIENTED_EDGE('',*,*,#8007,.F.);
#11306=ORIENTED_EDGE('',*,*,#8119,.F.);
#11307=ORIENTED_EDGE('',*,*,#8010,.F.);
#11308=ORIENTED_EDGE('',*,*,#7919,.F.);
#11309=ORIENTED_EDGE('',*,*,#8000,.F.);
#11310=ORIENTED_EDGE('',*,*,#8120,.F.);
#11311=ORIENTED_EDGE('',*,*,#8001,.F.);
#11312=ORIENTED_EDGE('',*,*,#7915,.F.);
#11313=ORIENTED_EDGE('',*,*,#7993,.F.);
#11314=ORIENTED_EDGE('',*,*,#8121,.F.);
#11315=ORIENTED_EDGE('',*,*,#7994,.F.);
#11316=ORIENTED_EDGE('',*,*,#7911,.F.);
#11317=ORIENTED_EDGE('',*,*,#7897,.F.);
#11318=ORIENTED_EDGE('',*,*,#8122,.F.);
#11319=ORIENTED_EDGE('',*,*,#7977,.F.);
#11320=ORIENTED_EDGE('',*,*,#7901,.F.);
#11321=ORIENTED_EDGE('',*,*,#7896,.F.);
#11322=ORIENTED_EDGE('',*,*,#7900,.T.);
#11323=ORIENTED_EDGE('',*,*,#8101,.F.);
#11324=ORIENTED_EDGE('',*,*,#8111,.T.);
#11325=ORIENTED_EDGE('',*,*,#8098,.F.);
#11326=ORIENTED_EDGE('',*,*,#8096,.T.);
#11327=ORIENTED_EDGE('',*,*,#8094,.F.);
#11328=ORIENTED_EDGE('',*,*,#8112,.T.);
#11329=ORIENTED_EDGE('',*,*,#8091,.F.);
#11330=ORIENTED_EDGE('',*,*,#8089,.T.);
#11331=ORIENTED_EDGE('',*,*,#8087,.F.);
#11332=ORIENTED_EDGE('',*,*,#8085,.T.);
#11333=ORIENTED_EDGE('',*,*,#8083,.F.);
#11334=ORIENTED_EDGE('',*,*,#8081,.T.);
#11335=ORIENTED_EDGE('',*,*,#8079,.F.);
#11336=ORIENTED_EDGE('',*,*,#8077,.T.);
#11337=ORIENTED_EDGE('',*,*,#8074,.F.);
#11338=ORIENTED_EDGE('',*,*,#8113,.T.);
#11339=ORIENTED_EDGE('',*,*,#8072,.F.);
#11340=ORIENTED_EDGE('',*,*,#8070,.T.);
#11341=ORIENTED_EDGE('',*,*,#8068,.F.);
#11342=ORIENTED_EDGE('',*,*,#8114,.T.);
#11343=ORIENTED_EDGE('',*,*,#8065,.F.);
#11344=ORIENTED_EDGE('',*,*,#8063,.T.);
#11345=ORIENTED_EDGE('',*,*,#8061,.F.);
#11346=ORIENTED_EDGE('',*,*,#8115,.T.);
#11347=ORIENTED_EDGE('',*,*,#8058,.F.);
#11348=ORIENTED_EDGE('',*,*,#8056,.T.);
#11349=ORIENTED_EDGE('',*,*,#8054,.F.);
#11350=ORIENTED_EDGE('',*,*,#8052,.T.);
#11351=ORIENTED_EDGE('',*,*,#8050,.F.);
#11352=ORIENTED_EDGE('',*,*,#8048,.T.);
#11353=ORIENTED_EDGE('',*,*,#8046,.F.);
#11354=ORIENTED_EDGE('',*,*,#8044,.T.);
#11355=ORIENTED_EDGE('',*,*,#8041,.F.);
#11356=ORIENTED_EDGE('',*,*,#8116,.T.);
#11357=ORIENTED_EDGE('',*,*,#8039,.F.);
#11358=ORIENTED_EDGE('',*,*,#8037,.T.);
#11359=ORIENTED_EDGE('',*,*,#8035,.F.);
#11360=ORIENTED_EDGE('',*,*,#8117,.T.);
#11361=ORIENTED_EDGE('',*,*,#8032,.F.);
#11362=ORIENTED_EDGE('',*,*,#8030,.T.);
#11363=ORIENTED_EDGE('',*,*,#8028,.F.);
#11364=ORIENTED_EDGE('',*,*,#8118,.T.);
#11365=ORIENTED_EDGE('',*,*,#8025,.F.);
#11366=ORIENTED_EDGE('',*,*,#8023,.T.);
#11367=ORIENTED_EDGE('',*,*,#8021,.F.);
#11368=ORIENTED_EDGE('',*,*,#8019,.T.);
#11369=ORIENTED_EDGE('',*,*,#8017,.F.);
#11370=ORIENTED_EDGE('',*,*,#8015,.T.);
#11371=ORIENTED_EDGE('',*,*,#8013,.F.);
#11372=ORIENTED_EDGE('',*,*,#8011,.T.);
#11373=ORIENTED_EDGE('',*,*,#8008,.F.);
#11374=ORIENTED_EDGE('',*,*,#8119,.T.);
#11375=ORIENTED_EDGE('',*,*,#8006,.F.);
#11376=ORIENTED_EDGE('',*,*,#8004,.T.);
#11377=ORIENTED_EDGE('',*,*,#8002,.F.);
#11378=ORIENTED_EDGE('',*,*,#8120,.T.);
#11379=ORIENTED_EDGE('',*,*,#7999,.F.);
#11380=ORIENTED_EDGE('',*,*,#7997,.T.);
#11381=ORIENTED_EDGE('',*,*,#7995,.F.);
#11382=ORIENTED_EDGE('',*,*,#8121,.T.);
#11383=ORIENTED_EDGE('',*,*,#7992,.F.);
#11384=ORIENTED_EDGE('',*,*,#7990,.T.);
#11385=ORIENTED_EDGE('',*,*,#7988,.F.);
#11386=ORIENTED_EDGE('',*,*,#7986,.T.);
#11387=ORIENTED_EDGE('',*,*,#7984,.F.);
#11388=ORIENTED_EDGE('',*,*,#7982,.T.);
#11389=ORIENTED_EDGE('',*,*,#7980,.F.);
#11390=ORIENTED_EDGE('',*,*,#7978,.T.);
#11391=ORIENTED_EDGE('',*,*,#7975,.F.);
#11392=ORIENTED_EDGE('',*,*,#8122,.T.);
#11393=ORIENTED_EDGE('',*,*,#7883,.T.);
#11394=ORIENTED_EDGE('',*,*,#7752,.T.);
#11395=ORIENTED_EDGE('',*,*,#7880,.T.);
#11396=ORIENTED_EDGE('',*,*,#7874,.T.);
#11397=ORIENTED_EDGE('',*,*,#8110,.F.);
#11398=ORIENTED_EDGE('',*,*,#8108,.F.);
#11399=ORIENTED_EDGE('',*,*,#8105,.F.);
#11400=ORIENTED_EDGE('',*,*,#8103,.F.);
#13447=PLANE('',#14884);
#13448=PLANE('',#14887);
#13449=PLANE('',#14889);
#13450=PLANE('',#14892);
#13451=PLANE('',#14897);
#13452=PLANE('',#14898);
#13453=PLANE('',#14940);
#13454=PLANE('',#14943);
#13455=PLANE('',#14946);
#13456=PLANE('',#14949);
#13457=PLANE('',#14954);
#13458=PLANE('',#14959);
#13459=PLANE('',#14964);
#13460=PLANE('',#14967);
#13461=PLANE('',#14970);
#13462=PLANE('',#14973);
#13463=PLANE('',#14978);
#13464=PLANE('',#14983);
#13465=PLANE('',#14988);
#13466=PLANE('',#14991);
#13467=PLANE('',#14994);
#13468=PLANE('',#14997);
#13469=PLANE('',#15002);
#13470=PLANE('',#15007);
#13471=PLANE('',#15012);
#13472=PLANE('',#15015);
#13473=PLANE('',#15018);
#13474=PLANE('',#15021);
#13475=PLANE('',#15026);
#13476=PLANE('',#15040);
#13477=PLANE('',#15041);
#13478=PLANE('',#15042);
#13479=PLANE('',#15043);
#13480=PLANE('',#15044);
#13481=PLANE('',#15045);
#13482=PLANE('',#15046);
#13483=PLANE('',#15047);
#13484=PLANE('',#15048);
#13485=PLANE('',#15049);
#13486=PLANE('',#15050);
#13487=PLANE('',#15051);
#13488=PLANE('',#15052);
#13723=ADVANCED_FACE('',(#2477),#1715,.F.);
#13724=ADVANCED_FACE('',(#2478),#1716,.F.);
#13725=ADVANCED_FACE('',(#2479),#1717,.F.);
#13726=ADVANCED_FACE('',(#2480),#1718,.F.);
#13727=ADVANCED_FACE('',(#2481),#1719,.F.);
#13728=ADVANCED_FACE('',(#2482),#1720,.F.);
#13729=ADVANCED_FACE('',(#2483),#1721,.F.);
#13730=ADVANCED_FACE('',(#2484),#1722,.F.);
#13731=ADVANCED_FACE('',(#2485),#1723,.F.);
#13732=ADVANCED_FACE('',(#2486),#1724,.F.);
#13733=ADVANCED_FACE('',(#2487),#1725,.F.);
#13734=ADVANCED_FACE('',(#2488),#1726,.F.);
#13735=ADVANCED_FACE('',(#2489),#1727,.F.);
#13736=ADVANCED_FACE('',(#2490),#1728,.F.);
#13737=ADVANCED_FACE('',(#2491),#1729,.F.);
#13738=ADVANCED_FACE('',(#2492),#1730,.F.);
#13739=ADVANCED_FACE('',(#2493),#1731,.F.);
#13740=ADVANCED_FACE('',(#2494),#1732,.F.);
#13741=ADVANCED_FACE('',(#2495),#1733,.F.);
#13742=ADVANCED_FACE('',(#2496),#1734,.F.);
#13743=ADVANCED_FACE('',(#2497),#1735,.F.);
#13744=ADVANCED_FACE('',(#2498),#1736,.F.);
#13745=ADVANCED_FACE('',(#2499),#1737,.F.);
#13746=ADVANCED_FACE('',(#2500),#1738,.F.);
#13747=ADVANCED_FACE('',(#2501),#1739,.F.);
#13748=ADVANCED_FACE('',(#2502),#1740,.F.);
#13749=ADVANCED_FACE('',(#2503),#1741,.F.);
#13750=ADVANCED_FACE('',(#2504),#1742,.F.);
#13751=ADVANCED_FACE('',(#2505),#1743,.F.);
#13752=ADVANCED_FACE('',(#2506),#1744,.F.);
#13753=ADVANCED_FACE('',(#2507),#1745,.F.);
#13754=ADVANCED_FACE('',(#2508),#1746,.F.);
#13755=ADVANCED_FACE('',(#2509),#1747,.F.);
#13756=ADVANCED_FACE('',(#2510),#1748,.F.);
#13757=ADVANCED_FACE('',(#2511),#1749,.F.);
#13758=ADVANCED_FACE('',(#2512),#1750,.F.);
#13759=ADVANCED_FACE('',(#2513),#1751,.F.);
#13760=ADVANCED_FACE('',(#2514),#1752,.F.);
#13761=ADVANCED_FACE('',(#2515),#1753,.F.);
#13762=ADVANCED_FACE('',(#2516),#1754,.F.);
#13763=ADVANCED_FACE('',(#2517),#1755,.F.);
#13764=ADVANCED_FACE('',(#2518),#1756,.F.);
#13765=ADVANCED_FACE('',(#2519),#1757,.F.);
#13766=ADVANCED_FACE('',(#2520),#1758,.F.);
#13767=ADVANCED_FACE('',(#2521),#1759,.F.);
#13768=ADVANCED_FACE('',(#2522),#1760,.F.);
#13769=ADVANCED_FACE('',(#2523),#1761,.F.);
#13770=ADVANCED_FACE('',(#2524),#1762,.F.);
#13771=ADVANCED_FACE('',(#2525),#1763,.F.);
#13772=ADVANCED_FACE('',(#2526),#1764,.F.);
#13773=ADVANCED_FACE('',(#2527),#1765,.F.);
#13774=ADVANCED_FACE('',(#2528),#1766,.F.);
#13775=ADVANCED_FACE('',(#2529),#1767,.F.);
#13776=ADVANCED_FACE('',(#2530),#1768,.F.);
#13777=ADVANCED_FACE('',(#2531),#1769,.F.);
#13778=ADVANCED_FACE('',(#2532),#1770,.F.);
#13779=ADVANCED_FACE('',(#2533),#1771,.F.);
#13780=ADVANCED_FACE('',(#2534),#1772,.F.);
#13781=ADVANCED_FACE('',(#2535),#1773,.F.);
#13782=ADVANCED_FACE('',(#2536),#1774,.F.);
#13783=ADVANCED_FACE('',(#2537),#1775,.F.);
#13784=ADVANCED_FACE('',(#2538),#1776,.F.);
#13785=ADVANCED_FACE('',(#2539),#1777,.F.);
#13786=ADVANCED_FACE('',(#2540),#1778,.F.);
#13787=ADVANCED_FACE('',(#2541),#1779,.F.);
#13788=ADVANCED_FACE('',(#2542),#1780,.F.);
#13789=ADVANCED_FACE('',(#2543),#1781,.F.);
#13790=ADVANCED_FACE('',(#2544),#1782,.F.);
#13791=ADVANCED_FACE('',(#2545),#1783,.F.);
#13792=ADVANCED_FACE('',(#2546),#1784,.F.);
#13793=ADVANCED_FACE('',(#2547),#1785,.F.);
#13794=ADVANCED_FACE('',(#2548),#1786,.F.);
#13795=ADVANCED_FACE('',(#2549),#1787,.F.);
#13796=ADVANCED_FACE('',(#2550),#1788,.F.);
#13797=ADVANCED_FACE('',(#2551),#1789,.F.);
#13798=ADVANCED_FACE('',(#2552),#1790,.F.);
#13799=ADVANCED_FACE('',(#2553),#1791,.F.);
#13800=ADVANCED_FACE('',(#2554),#1792,.F.);
#13801=ADVANCED_FACE('',(#2555),#1793,.F.);
#13802=ADVANCED_FACE('',(#2556),#1794,.F.);
#13803=ADVANCED_FACE('',(#2557),#1795,.F.);
#13804=ADVANCED_FACE('',(#2558),#1796,.F.);
#13805=ADVANCED_FACE('',(#2559),#1797,.F.);
#13806=ADVANCED_FACE('',(#2560),#1798,.F.);
#13807=ADVANCED_FACE('',(#2561),#1799,.F.);
#13808=ADVANCED_FACE('',(#2562),#1800,.F.);
#13809=ADVANCED_FACE('',(#2563),#1801,.F.);
#13810=ADVANCED_FACE('',(#2564),#1802,.F.);
#13811=ADVANCED_FACE('',(#2565),#1803,.F.);
#13812=ADVANCED_FACE('',(#2566),#1804,.F.);
#13813=ADVANCED_FACE('',(#2567),#1805,.F.);
#13814=ADVANCED_FACE('',(#2568),#1806,.F.);
#13815=ADVANCED_FACE('',(#2569),#1807,.F.);
#13816=ADVANCED_FACE('',(#2570),#1808,.F.);
#13817=ADVANCED_FACE('',(#2571),#1809,.F.);
#13818=ADVANCED_FACE('',(#2572),#1810,.F.);
#13819=ADVANCED_FACE('',(#2573),#1811,.F.);
#13820=ADVANCED_FACE('',(#2574),#1812,.F.);
#13821=ADVANCED_FACE('',(#2575),#1813,.F.);
#13822=ADVANCED_FACE('',(#2576),#1814,.F.);
#13823=ADVANCED_FACE('',(#2577),#1815,.F.);
#13824=ADVANCED_FACE('',(#2578),#1816,.F.);
#13825=ADVANCED_FACE('',(#2579),#1817,.F.);
#13826=ADVANCED_FACE('',(#2580),#1818,.F.);
#13827=ADVANCED_FACE('',(#2581),#1819,.F.);
#13828=ADVANCED_FACE('',(#2582),#1820,.F.);
#13829=ADVANCED_FACE('',(#2583),#1821,.F.);
#13830=ADVANCED_FACE('',(#2584),#1822,.F.);
#13831=ADVANCED_FACE('',(#2585),#1823,.F.);
#13832=ADVANCED_FACE('',(#2586),#1824,.F.);
#13833=ADVANCED_FACE('',(#2587),#1825,.F.);
#13834=ADVANCED_FACE('',(#2588),#1826,.F.);
#13835=ADVANCED_FACE('',(#2589),#1827,.F.);
#13836=ADVANCED_FACE('',(#2590),#1828,.F.);
#13837=ADVANCED_FACE('',(#2591),#1829,.F.);
#13838=ADVANCED_FACE('',(#2592),#1830,.F.);
#13839=ADVANCED_FACE('',(#2593),#1831,.F.);
#13840=ADVANCED_FACE('',(#2594),#1832,.F.);
#13841=ADVANCED_FACE('',(#2595),#1833,.F.);
#13842=ADVANCED_FACE('',(#2596),#1834,.F.);
#13843=ADVANCED_FACE('',(#2597),#1835,.F.);
#13844=ADVANCED_FACE('',(#2598),#1836,.F.);
#13845=ADVANCED_FACE('',(#2599),#1837,.F.);
#13846=ADVANCED_FACE('',(#2600),#1838,.F.);
#13847=ADVANCED_FACE('',(#2601),#1839,.F.);
#13848=ADVANCED_FACE('',(#2602),#1840,.F.);
#13849=ADVANCED_FACE('',(#2603),#1841,.F.);
#13850=ADVANCED_FACE('',(#2604),#1842,.F.);
#13851=ADVANCED_FACE('',(#2605),#1843,.F.);
#13852=ADVANCED_FACE('',(#2606),#1844,.F.);
#13853=ADVANCED_FACE('',(#2607),#13447,.F.);
#13854=ADVANCED_FACE('',(#2608),#1845,.F.);
#13855=ADVANCED_FACE('',(#2609),#267,.F.);
#13856=ADVANCED_FACE('',(#2610),#268,.F.);
#13857=ADVANCED_FACE('',(#2611),#1846,.F.);
#13858=ADVANCED_FACE('',(#2612,#2256),#13448,.F.);
#13859=ADVANCED_FACE('',(#2613),#13449,.T.);
#13860=ADVANCED_FACE('',(#2614),#1847,.F.);
#13861=ADVANCED_FACE('',(#2615),#269,.F.);
#13862=ADVANCED_FACE('',(#2616),#270,.F.);
#13863=ADVANCED_FACE('',(#2617),#1848,.F.);
#13864=ADVANCED_FACE('',(#2618,#2257),#13450,.F.);
#13865=ADVANCED_FACE('',(#2619),#1849,.T.);
#13866=ADVANCED_FACE('',(#2620),#13451,.T.);
#13867=ADVANCED_FACE('',(#2621,#2258,#2259,#2260,#2261,#2262),#13452,.T.);
#13868=ADVANCED_FACE('',(#2622),#1850,.F.);
#13869=ADVANCED_FACE('',(#2623),#13453,.T.);
#13870=ADVANCED_FACE('',(#2624),#1851,.F.);
#13871=ADVANCED_FACE('',(#2625),#13454,.T.);
#13872=ADVANCED_FACE('',(#2626),#1852,.F.);
#13873=ADVANCED_FACE('',(#2627),#13455,.T.);
#13874=ADVANCED_FACE('',(#2628),#1853,.F.);
#13875=ADVANCED_FACE('',(#2629),#13456,.T.);
#13876=ADVANCED_FACE('',(#2630),#1854,.T.);
#13877=ADVANCED_FACE('',(#2631),#1855,.T.);
#13878=ADVANCED_FACE('',(#2632),#13457,.T.);
#13879=ADVANCED_FACE('',(#2633),#1856,.T.);
#13880=ADVANCED_FACE('',(#2634),#1857,.T.);
#13881=ADVANCED_FACE('',(#2635),#13458,.T.);
#13882=ADVANCED_FACE('',(#2636),#1858,.T.);
#13883=ADVANCED_FACE('',(#2637),#1859,.F.);
#13884=ADVANCED_FACE('',(#2638),#13459,.T.);
#13885=ADVANCED_FACE('',(#2639),#1860,.F.);
#13886=ADVANCED_FACE('',(#2640),#13460,.T.);
#13887=ADVANCED_FACE('',(#2641),#1861,.F.);
#13888=ADVANCED_FACE('',(#2642),#13461,.T.);
#13889=ADVANCED_FACE('',(#2643),#1862,.F.);
#13890=ADVANCED_FACE('',(#2644),#13462,.T.);
#13891=ADVANCED_FACE('',(#2645),#1863,.T.);
#13892=ADVANCED_FACE('',(#2646),#1864,.T.);
#13893=ADVANCED_FACE('',(#2647),#13463,.T.);
#13894=ADVANCED_FACE('',(#2648),#1865,.T.);
#13895=ADVANCED_FACE('',(#2649),#1866,.T.);
#13896=ADVANCED_FACE('',(#2650),#13464,.T.);
#13897=ADVANCED_FACE('',(#2651),#1867,.T.);
#13898=ADVANCED_FACE('',(#2652),#1868,.F.);
#13899=ADVANCED_FACE('',(#2653),#13465,.T.);
#13900=ADVANCED_FACE('',(#2654),#1869,.F.);
#13901=ADVANCED_FACE('',(#2655),#13466,.T.);
#13902=ADVANCED_FACE('',(#2656),#1870,.F.);
#13903=ADVANCED_FACE('',(#2657),#13467,.T.);
#13904=ADVANCED_FACE('',(#2658),#1871,.F.);
#13905=ADVANCED_FACE('',(#2659),#13468,.T.);
#13906=ADVANCED_FACE('',(#2660),#1872,.T.);
#13907=ADVANCED_FACE('',(#2661),#1873,.T.);
#13908=ADVANCED_FACE('',(#2662),#13469,.T.);
#13909=ADVANCED_FACE('',(#2663),#1874,.T.);
#13910=ADVANCED_FACE('',(#2664),#1875,.T.);
#13911=ADVANCED_FACE('',(#2665),#13470,.T.);
#13912=ADVANCED_FACE('',(#2666),#1876,.T.);
#13913=ADVANCED_FACE('',(#2667),#1877,.F.);
#13914=ADVANCED_FACE('',(#2668),#13471,.T.);
#13915=ADVANCED_FACE('',(#2669),#1878,.F.);
#13916=ADVANCED_FACE('',(#2670),#13472,.T.);
#13917=ADVANCED_FACE('',(#2671),#1879,.F.);
#13918=ADVANCED_FACE('',(#2672),#13473,.T.);
#13919=ADVANCED_FACE('',(#2673),#1880,.F.);
#13920=ADVANCED_FACE('',(#2674),#13474,.T.);
#13921=ADVANCED_FACE('',(#2675),#1881,.T.);
#13922=ADVANCED_FACE('',(#2676),#1882,.T.);
#13923=ADVANCED_FACE('',(#2677),#13475,.T.);
#13924=ADVANCED_FACE('',(#2678),#1883,.T.);
#13925=ADVANCED_FACE('',(#2679),#1884,.T.);
#13926=ADVANCED_FACE('',(#2680),#1885,.F.);
#13927=ADVANCED_FACE('',(#2681),#1886,.F.);
#13928=ADVANCED_FACE('',(#2682),#1887,.F.);
#13929=ADVANCED_FACE('',(#2683),#1888,.F.);
#13930=ADVANCED_FACE('',(#2684),#1889,.F.);
#13931=ADVANCED_FACE('',(#2685),#13476,.T.);
#13932=ADVANCED_FACE('',(#2686),#13477,.T.);
#13933=ADVANCED_FACE('',(#2687),#13478,.T.);
#13934=ADVANCED_FACE('',(#2688),#13479,.T.);
#13935=ADVANCED_FACE('',(#2689),#13480,.T.);
#13936=ADVANCED_FACE('',(#2690),#13481,.T.);
#13937=ADVANCED_FACE('',(#2691),#13482,.T.);
#13938=ADVANCED_FACE('',(#2692),#13483,.T.);
#13939=ADVANCED_FACE('',(#2693),#13484,.T.);
#13940=ADVANCED_FACE('',(#2694),#13485,.T.);
#13941=ADVANCED_FACE('',(#2695),#13486,.T.);
#13942=ADVANCED_FACE('',(#2696),#13487,.T.);
#13943=ADVANCED_FACE('',(#2697,#2263,#2264,#2265,#2266,#2267),#13488,.F.);
#14314=CLOSED_SHELL('',(#13723,#13724,#13725,#13726,#13727,#13728,#13729,
#13730,#13731,#13732,#13733,#13734,#13735,#13736,#13737,#13738,#13739,#13740,
#13741,#13742,#13743,#13744,#13745,#13746,#13747,#13748,#13749,#13750,#13751,
#13752,#13753,#13754,#13755,#13756,#13757,#13758,#13759,#13760,#13761,#13762,
#13763,#13764,#13765,#13766,#13767,#13768,#13769,#13770,#13771,#13772,#13773,
#13774,#13775,#13776,#13777,#13778,#13779,#13780,#13781,#13782,#13783,#13784,
#13785,#13786,#13787,#13788,#13789,#13790,#13791,#13792,#13793,#13794,#13795,
#13796,#13797,#13798,#13799,#13800,#13801,#13802,#13803,#13804,#13805,#13806,
#13807,#13808,#13809,#13810,#13811,#13812,#13813,#13814,#13815,#13816,#13817,
#13818,#13819,#13820,#13821,#13822,#13823,#13824,#13825,#13826,#13827,#13828,
#13829,#13830,#13831,#13832,#13833,#13834,#13835,#13836,#13837,#13838,#13839,
#13840,#13841,#13842,#13843,#13844,#13845,#13846,#13847,#13848,#13849,#13850,
#13851,#13852,#13853,#13854,#13855,#13856,#13857,#13858,#13859,#13860,#13861,
#13862,#13863,#13864,#13865,#13866,#13867,#13868,#13869,#13870,#13871,#13872,
#13873,#13874,#13875,#13876,#13877,#13878,#13879,#13880,#13881,#13882,#13883,
#13884,#13885,#13886,#13887,#13888,#13889,#13890,#13891,#13892,#13893,#13894,
#13895,#13896,#13897,#13898,#13899,#13900,#13901,#13902,#13903,#13904,#13905,
#13906,#13907,#13908,#13909,#13910,#13911,#13912,#13913,#13914,#13915,#13916,
#13917,#13918,#13919,#13920,#13921,#13922,#13923,#13924,#13925,#13926,#13927,
#13928,#13929,#13930,#13931,#13932,#13933,#13934,#13935,#13936,#13937,#13938,
#13939,#13940,#13941,#13942,#13943));
#14741=AXIS2_PLACEMENT_3D('',#28040,#16187,#16188);
#14742=AXIS2_PLACEMENT_3D('',#28041,#16189,#16190);
#14743=AXIS2_PLACEMENT_3D('',#28054,#16192,#16193);
#14744=AXIS2_PLACEMENT_3D('',#28057,#16195,#16196);
#14745=AXIS2_PLACEMENT_3D('',#28059,#16197,#16198);
#14746=AXIS2_PLACEMENT_3D('',#28076,#16199,#16200);
#14747=AXIS2_PLACEMENT_3D('',#28166,#16202,#16203);
#14748=AXIS2_PLACEMENT_3D('',#28253,#16205,#16206);
#14749=AXIS2_PLACEMENT_3D('',#28340,#16208,#16209);
#14750=AXIS2_PLACEMENT_3D('',#28427,#16211,#16212);
#14751=AXIS2_PLACEMENT_3D('',#28517,#16214,#16215);
#14752=AXIS2_PLACEMENT_3D('',#28604,#16217,#16218);
#14753=AXIS2_PLACEMENT_3D('',#28691,#16220,#16221);
#14754=AXIS2_PLACEMENT_3D('',#28781,#16223,#16224);
#14755=AXIS2_PLACEMENT_3D('',#28868,#16226,#16227);
#14756=AXIS2_PLACEMENT_3D('',#28955,#16229,#16230);
#14757=AXIS2_PLACEMENT_3D('',#29042,#16232,#16233);
#14758=AXIS2_PLACEMENT_3D('',#29132,#16235,#16236);
#14759=AXIS2_PLACEMENT_3D('',#29219,#16238,#16239);
#14760=AXIS2_PLACEMENT_3D('',#29306,#16241,#16242);
#14761=AXIS2_PLACEMENT_3D('',#29393,#16244,#16245);
#14762=AXIS2_PLACEMENT_3D('',#29483,#16247,#16248);
#14763=AXIS2_PLACEMENT_3D('',#29570,#16250,#16251);
#14764=AXIS2_PLACEMENT_3D('',#29657,#16253,#16254);
#14765=AXIS2_PLACEMENT_3D('',#29747,#16256,#16257);
#14766=AXIS2_PLACEMENT_3D('',#29834,#16259,#16260);
#14767=AXIS2_PLACEMENT_3D('',#29921,#16262,#16263);
#14768=AXIS2_PLACEMENT_3D('',#30008,#16265,#16266);
#14769=AXIS2_PLACEMENT_3D('',#30098,#16268,#16269);
#14770=AXIS2_PLACEMENT_3D('',#30129,#16271,#16272);
#14771=AXIS2_PLACEMENT_3D('',#30167,#16273,#16274);
#14772=AXIS2_PLACEMENT_3D('',#30185,#16276,#16277);
#14773=AXIS2_PLACEMENT_3D('',#30200,#16278,#16279);
#14774=AXIS2_PLACEMENT_3D('',#30237,#16281,#16282);
#14775=AXIS2_PLACEMENT_3D('',#30275,#16284,#16285);
#14776=AXIS2_PLACEMENT_3D('',#30311,#16287,#16288);
#14777=AXIS2_PLACEMENT_3D('',#30349,#16290,#16291);
#14778=AXIS2_PLACEMENT_3D('',#30387,#16293,#16294);
#14779=AXIS2_PLACEMENT_3D('',#30423,#16296,#16297);
#14780=AXIS2_PLACEMENT_3D('',#30461,#16299,#16300);
#14781=AXIS2_PLACEMENT_3D('',#30499,#16302,#16303);
#14782=AXIS2_PLACEMENT_3D('',#30535,#16305,#16306);
#14783=AXIS2_PLACEMENT_3D('',#30573,#16308,#16309);
#14784=AXIS2_PLACEMENT_3D('',#30610,#16311,#16312);
#14785=AXIS2_PLACEMENT_3D('',#30647,#16314,#16315);
#14786=AXIS2_PLACEMENT_3D('',#30685,#16317,#16318);
#14787=AXIS2_PLACEMENT_3D('',#30721,#16320,#16321);
#14788=AXIS2_PLACEMENT_3D('',#30759,#16323,#16324);
#14789=AXIS2_PLACEMENT_3D('',#30797,#16326,#16327);
#14790=AXIS2_PLACEMENT_3D('',#30833,#16329,#16330);
#14791=AXIS2_PLACEMENT_3D('',#30871,#16332,#16333);
#14792=AXIS2_PLACEMENT_3D('',#30909,#16335,#16336);
#14793=AXIS2_PLACEMENT_3D('',#30945,#16338,#16339);
#14794=AXIS2_PLACEMENT_3D('',#30983,#16341,#16342);
#14795=AXIS2_PLACEMENT_3D('',#31020,#16344,#16345);
#14796=AXIS2_PLACEMENT_3D('',#31057,#16347,#16348);
#14797=AXIS2_PLACEMENT_3D('',#31069,#16350,#16351);
#14798=AXIS2_PLACEMENT_3D('',#31077,#16352,#16353);
#14799=AXIS2_PLACEMENT_3D('',#31090,#16355,#16356);
#14800=AXIS2_PLACEMENT_3D('',#31093,#16358,#16359);
#14801=AXIS2_PLACEMENT_3D('',#31095,#16360,#16361);
#14802=AXIS2_PLACEMENT_3D('',#31112,#16362,#16363);
#14803=AXIS2_PLACEMENT_3D('',#31202,#16365,#16366);
#14804=AXIS2_PLACEMENT_3D('',#31289,#16368,#16369);
#14805=AXIS2_PLACEMENT_3D('',#31376,#16371,#16372);
#14806=AXIS2_PLACEMENT_3D('',#31463,#16374,#16375);
#14807=AXIS2_PLACEMENT_3D('',#31550,#16377,#16378);
#14808=AXIS2_PLACEMENT_3D('',#31640,#16380,#16381);
#14809=AXIS2_PLACEMENT_3D('',#31727,#16383,#16384);
#14810=AXIS2_PLACEMENT_3D('',#31814,#16386,#16387);
#14811=AXIS2_PLACEMENT_3D('',#31901,#16389,#16390);
#14812=AXIS2_PLACEMENT_3D('',#31988,#16392,#16393);
#14813=AXIS2_PLACEMENT_3D('',#32078,#16395,#16396);
#14814=AXIS2_PLACEMENT_3D('',#32165,#16398,#16399);
#14815=AXIS2_PLACEMENT_3D('',#32252,#16401,#16402);
#14816=AXIS2_PLACEMENT_3D('',#32339,#16404,#16405);
#14817=AXIS2_PLACEMENT_3D('',#32426,#16407,#16408);
#14818=AXIS2_PLACEMENT_3D('',#32513,#16410,#16411);
#14819=AXIS2_PLACEMENT_3D('',#32600,#16413,#16414);
#14820=AXIS2_PLACEMENT_3D('',#32687,#16416,#16417);
#14821=AXIS2_PLACEMENT_3D('',#32762,#16419,#16420);
#14822=AXIS2_PLACEMENT_3D('',#32810,#16422,#16423);
#14823=AXIS2_PLACEMENT_3D('',#32867,#16425,#16426);
#14824=AXIS2_PLACEMENT_3D('',#32954,#16428,#16429);
#14825=AXIS2_PLACEMENT_3D('',#33041,#16431,#16432);
#14826=AXIS2_PLACEMENT_3D('',#33128,#16434,#16435);
#14827=AXIS2_PLACEMENT_3D('',#33215,#16437,#16438);
#14828=AXIS2_PLACEMENT_3D('',#33302,#16440,#16441);
#14829=AXIS2_PLACEMENT_3D('',#33392,#16443,#16444);
#14830=AXIS2_PLACEMENT_3D('',#33479,#16446,#16447);
#14831=AXIS2_PLACEMENT_3D('',#33566,#16449,#16450);
#14832=AXIS2_PLACEMENT_3D('',#33653,#16452,#16453);
#14833=AXIS2_PLACEMENT_3D('',#33740,#16455,#16456);
#14834=AXIS2_PLACEMENT_3D('',#33830,#16458,#16459);
#14835=AXIS2_PLACEMENT_3D('',#33917,#16461,#16462);
#14836=AXIS2_PLACEMENT_3D('',#34004,#16464,#16465);
#14837=AXIS2_PLACEMENT_3D('',#34091,#16467,#16468);
#14838=AXIS2_PLACEMENT_3D('',#34178,#16470,#16471);
#14839=AXIS2_PLACEMENT_3D('',#34268,#16473,#16474);
#14840=AXIS2_PLACEMENT_3D('',#34355,#16476,#16477);
#14841=AXIS2_PLACEMENT_3D('',#34386,#16479,#16480);
#14842=AXIS2_PLACEMENT_3D('',#34424,#16481,#16482);
#14843=AXIS2_PLACEMENT_3D('',#34442,#16484,#16485);
#14844=AXIS2_PLACEMENT_3D('',#34457,#16486,#16487);
#14845=AXIS2_PLACEMENT_3D('',#34494,#16489,#16490);
#14846=AXIS2_PLACEMENT_3D('',#34532,#16492,#16493);
#14847=AXIS2_PLACEMENT_3D('',#34568,#16495,#16496);
#14848=AXIS2_PLACEMENT_3D('',#34606,#16498,#16499);
#14849=AXIS2_PLACEMENT_3D('',#34643,#16501,#16502);
#14850=AXIS2_PLACEMENT_3D('',#34680,#16504,#16505);
#14851=AXIS2_PLACEMENT_3D('',#34718,#16507,#16508);
#14852=AXIS2_PLACEMENT_3D('',#34754,#16510,#16511);
#14853=AXIS2_PLACEMENT_3D('',#34792,#16513,#16514);
#14854=AXIS2_PLACEMENT_3D('',#34829,#16516,#16517);
#14855=AXIS2_PLACEMENT_3D('',#34866,#16519,#16520);
#14856=AXIS2_PLACEMENT_3D('',#34904,#16522,#16523);
#14857=AXIS2_PLACEMENT_3D('',#34940,#16525,#16526);
#14858=AXIS2_PLACEMENT_3D('',#34978,#16528,#16529);
#14859=AXIS2_PLACEMENT_3D('',#35015,#16531,#16532);
#14860=AXIS2_PLACEMENT_3D('',#35052,#16534,#16535);
#14861=AXIS2_PLACEMENT_3D('',#35090,#16537,#16538);
#14862=AXIS2_PLACEMENT_3D('',#35126,#16540,#16541);
#14863=AXIS2_PLACEMENT_3D('',#35153,#16543,#16544);
#14864=AXIS2_PLACEMENT_3D('',#35177,#16546,#16547);
#14865=AXIS2_PLACEMENT_3D('',#35210,#16549,#16550);
#14866=AXIS2_PLACEMENT_3D('',#35248,#16552,#16553);
#14867=AXIS2_PLACEMENT_3D('',#35284,#16555,#16556);
#14868=AXIS2_PLACEMENT_3D('',#35322,#16558,#16559);
#14869=AXIS2_PLACEMENT_3D('',#35358,#16561,#16562);
#14870=AXIS2_PLACEMENT_3D('',#35396,#16564,#16565);
#14871=AXIS2_PLACEMENT_3D('',#35434,#16567,#16568);
#14872=AXIS2_PLACEMENT_3D('',#35470,#16570,#16571);
#14873=AXIS2_PLACEMENT_3D('',#35508,#16573,#16574);
#14874=AXIS2_PLACEMENT_3D('',#35544,#16576,#16577);
#14875=AXIS2_PLACEMENT_3D('',#35582,#16579,#16580);
#14876=AXIS2_PLACEMENT_3D('',#35620,#16582,#16583);
#14877=AXIS2_PLACEMENT_3D('',#35656,#16585,#16586);
#14878=AXIS2_PLACEMENT_3D('',#35694,#16588,#16589);
#14879=AXIS2_PLACEMENT_3D('',#35730,#16591,#16592);
#14880=AXIS2_PLACEMENT_3D('',#35768,#16594,#16595);
#14881=AXIS2_PLACEMENT_3D('',#35806,#16597,#16598);
#14882=AXIS2_PLACEMENT_3D('',#35842,#16600,#16601);
#14883=AXIS2_PLACEMENT_3D('',#35854,#16603,#16604);
#14884=AXIS2_PLACEMENT_3D('',#35862,#16605,#16606);
#14885=AXIS2_PLACEMENT_3D('',#36072,#16607,#16608);
#14886=AXIS2_PLACEMENT_3D('',#40378,#16609,#16610);
#14887=AXIS2_PLACEMENT_3D('',#40379,#16611,#16612);
#14888=AXIS2_PLACEMENT_3D('',#40381,#16613,#16614);
#14889=AXIS2_PLACEMENT_3D('',#40382,#16615,#16616);
#14890=AXIS2_PLACEMENT_3D('',#40589,#16617,#16618);
#14891=AXIS2_PLACEMENT_3D('',#43503,#16619,#16620);
#14892=AXIS2_PLACEMENT_3D('',#43504,#16621,#16622);
#14893=AXIS2_PLACEMENT_3D('',#43506,#16623,#16624);
#14894=AXIS2_PLACEMENT_3D('',#43507,#16625,#16626);
#14895=AXIS2_PLACEMENT_3D('',#43510,#16627,#16628);
#14896=AXIS2_PLACEMENT_3D('',#43514,#16630,#16631);
#14897=AXIS2_PLACEMENT_3D('',#43516,#16633,#16634);
#14898=AXIS2_PLACEMENT_3D('',#43522,#16638,#16639);
#14899=AXIS2_PLACEMENT_3D('',#43526,#16641,#16642);
#14900=AXIS2_PLACEMENT_3D('',#43530,#16644,#16645);
#14901=AXIS2_PLACEMENT_3D('',#43534,#16647,#16648);
#14902=AXIS2_PLACEMENT_3D('',#43538,#16650,#16651);
#14903=AXIS2_PLACEMENT_3D('',#43542,#16653,#16654);
#14904=AXIS2_PLACEMENT_3D('',#43546,#16656,#16657);
#14905=AXIS2_PLACEMENT_3D('',#43550,#16659,#16660);
#14906=AXIS2_PLACEMENT_3D('',#43554,#16662,#16663);
#14907=AXIS2_PLACEMENT_3D('',#43558,#16665,#16666);
#14908=AXIS2_PLACEMENT_3D('',#43562,#16668,#16669);
#14909=AXIS2_PLACEMENT_3D('',#43566,#16671,#16672);
#14910=AXIS2_PLACEMENT_3D('',#43570,#16674,#16675);
#14911=AXIS2_PLACEMENT_3D('',#43574,#16677,#16678);
#14912=AXIS2_PLACEMENT_3D('',#43578,#16680,#16681);
#14913=AXIS2_PLACEMENT_3D('',#43582,#16683,#16684);
#14914=AXIS2_PLACEMENT_3D('',#43586,#16686,#16687);
#14915=AXIS2_PLACEMENT_3D('',#43590,#16689,#16690);
#14916=AXIS2_PLACEMENT_3D('',#43594,#16692,#16693);
#14917=AXIS2_PLACEMENT_3D('',#43598,#16695,#16696);
#14918=AXIS2_PLACEMENT_3D('',#43602,#16698,#16699);
#14919=AXIS2_PLACEMENT_3D('',#43606,#16701,#16702);
#14920=AXIS2_PLACEMENT_3D('',#43610,#16704,#16705);
#14921=AXIS2_PLACEMENT_3D('',#43614,#16707,#16708);
#14922=AXIS2_PLACEMENT_3D('',#43618,#16710,#16711);
#14923=AXIS2_PLACEMENT_3D('',#43622,#16713,#16714);
#14924=AXIS2_PLACEMENT_3D('',#43626,#16716,#16717);
#14925=AXIS2_PLACEMENT_3D('',#43630,#16719,#16720);
#14926=AXIS2_PLACEMENT_3D('',#43634,#16722,#16723);
#14927=AXIS2_PLACEMENT_3D('',#43638,#16725,#16726);
#14928=AXIS2_PLACEMENT_3D('',#43642,#16728,#16729);
#14929=AXIS2_PLACEMENT_3D('',#43646,#16731,#16732);
#14930=AXIS2_PLACEMENT_3D('',#43650,#16734,#16735);
#14931=AXIS2_PLACEMENT_3D('',#43654,#16737,#16738);
#14932=AXIS2_PLACEMENT_3D('',#43658,#16740,#16741);
#14933=AXIS2_PLACEMENT_3D('',#43661,#16743,#16744);
#14934=AXIS2_PLACEMENT_3D('',#43663,#16745,#16746);
#14935=AXIS2_PLACEMENT_3D('',#43665,#16747,#16748);
#14936=AXIS2_PLACEMENT_3D('',#43667,#16749,#16750);
#14937=AXIS2_PLACEMENT_3D('',#43669,#16751,#16752);
#14938=AXIS2_PLACEMENT_3D('',#43670,#16753,#16754);
#14939=AXIS2_PLACEMENT_3D('',#43673,#16755,#16756);
#14940=AXIS2_PLACEMENT_3D('',#43676,#16759,#16760);
#14941=AXIS2_PLACEMENT_3D('',#43680,#16763,#16764);
#14942=AXIS2_PLACEMENT_3D('',#43682,#16765,#16766);
#14943=AXIS2_PLACEMENT_3D('',#43684,#16768,#16769);
#14944=AXIS2_PLACEMENT_3D('',#43688,#16772,#16773);
#14945=AXIS2_PLACEMENT_3D('',#43690,#16774,#16775);
#14946=AXIS2_PLACEMENT_3D('',#43692,#16777,#16778);
#14947=AXIS2_PLACEMENT_3D('',#43696,#16781,#16782);
#14948=AXIS2_PLACEMENT_3D('',#43698,#16783,#16784);
#14949=AXIS2_PLACEMENT_3D('',#43700,#16786,#16787);
#14950=AXIS2_PLACEMENT_3D('',#43704,#16790,#16791);
#14951=AXIS2_PLACEMENT_3D('',#43706,#16792,#16793);
#14952=AXIS2_PLACEMENT_3D('',#43708,#16795,#16796);
#14953=AXIS2_PLACEMENT_3D('',#43712,#16798,#16799);
#14954=AXIS2_PLACEMENT_3D('',#43714,#16801,#16802);
#14955=AXIS2_PLACEMENT_3D('',#43718,#16805,#16806);
#14956=AXIS2_PLACEMENT_3D('',#43720,#16807,#16808);
#14957=AXIS2_PLACEMENT_3D('',#43722,#16810,#16811);
#14958=AXIS2_PLACEMENT_3D('',#43726,#16813,#16814);
#14959=AXIS2_PLACEMENT_3D('',#43728,#16816,#16817);
#14960=AXIS2_PLACEMENT_3D('',#43732,#16820,#16821);
#14961=AXIS2_PLACEMENT_3D('',#43734,#16822,#16823);
#14962=AXIS2_PLACEMENT_3D('',#43736,#16825,#16826);
#14963=AXIS2_PLACEMENT_3D('',#43739,#16827,#16828);
#14964=AXIS2_PLACEMENT_3D('',#43742,#16831,#16832);
#14965=AXIS2_PLACEMENT_3D('',#43746,#16835,#16836);
#14966=AXIS2_PLACEMENT_3D('',#43748,#16837,#16838);
#14967=AXIS2_PLACEMENT_3D('',#43750,#16840,#16841);
#14968=AXIS2_PLACEMENT_3D('',#43754,#16844,#16845);
#14969=AXIS2_PLACEMENT_3D('',#43756,#16846,#16847);
#14970=AXIS2_PLACEMENT_3D('',#43758,#16849,#16850);
#14971=AXIS2_PLACEMENT_3D('',#43762,#16853,#16854);
#14972=AXIS2_PLACEMENT_3D('',#43764,#16855,#16856);
#14973=AXIS2_PLACEMENT_3D('',#43766,#16858,#16859);
#14974=AXIS2_PLACEMENT_3D('',#43770,#16862,#16863);
#14975=AXIS2_PLACEMENT_3D('',#43772,#16864,#16865);
#14976=AXIS2_PLACEMENT_3D('',#43774,#16867,#16868);
#14977=AXIS2_PLACEMENT_3D('',#43778,#16870,#16871);
#14978=AXIS2_PLACEMENT_3D('',#43780,#16873,#16874);
#14979=AXIS2_PLACEMENT_3D('',#43784,#16877,#16878);
#14980=AXIS2_PLACEMENT_3D('',#43786,#16879,#16880);
#14981=AXIS2_PLACEMENT_3D('',#43788,#16882,#16883);
#14982=AXIS2_PLACEMENT_3D('',#43792,#16885,#16886);
#14983=AXIS2_PLACEMENT_3D('',#43794,#16888,#16889);
#14984=AXIS2_PLACEMENT_3D('',#43798,#16892,#16893);
#14985=AXIS2_PLACEMENT_3D('',#43800,#16894,#16895);
#14986=AXIS2_PLACEMENT_3D('',#43802,#16897,#16898);
#14987=AXIS2_PLACEMENT_3D('',#43805,#16899,#16900);
#14988=AXIS2_PLACEMENT_3D('',#43808,#16903,#16904);
#14989=AXIS2_PLACEMENT_3D('',#43812,#16907,#16908);
#14990=AXIS2_PLACEMENT_3D('',#43814,#16909,#16910);
#14991=AXIS2_PLACEMENT_3D('',#43816,#16912,#16913);
#14992=AXIS2_PLACEMENT_3D('',#43820,#16916,#16917);
#14993=AXIS2_PLACEMENT_3D('',#43822,#16918,#16919);
#14994=AXIS2_PLACEMENT_3D('',#43824,#16921,#16922);
#14995=AXIS2_PLACEMENT_3D('',#43828,#16925,#16926);
#14996=AXIS2_PLACEMENT_3D('',#43830,#16927,#16928);
#14997=AXIS2_PLACEMENT_3D('',#43832,#16930,#16931);
#14998=AXIS2_PLACEMENT_3D('',#43836,#16934,#16935);
#14999=AXIS2_PLACEMENT_3D('',#43838,#16936,#16937);
#15000=AXIS2_PLACEMENT_3D('',#43840,#16939,#16940);
#15001=AXIS2_PLACEMENT_3D('',#43844,#16942,#16943);
#15002=AXIS2_PLACEMENT_3D('',#43846,#16945,#16946);
#15003=AXIS2_PLACEMENT_3D('',#43850,#16949,#16950);
#15004=AXIS2_PLACEMENT_3D('',#43852,#16951,#16952);
#15005=AXIS2_PLACEMENT_3D('',#43854,#16954,#16955);
#15006=AXIS2_PLACEMENT_3D('',#43858,#16957,#16958);
#15007=AXIS2_PLACEMENT_3D('',#43860,#16960,#16961);
#15008=AXIS2_PLACEMENT_3D('',#43864,#16964,#16965);
#15009=AXIS2_PLACEMENT_3D('',#43866,#16966,#16967);
#15010=AXIS2_PLACEMENT_3D('',#43868,#16969,#16970);
#15011=AXIS2_PLACEMENT_3D('',#43871,#16971,#16972);
#15012=AXIS2_PLACEMENT_3D('',#43874,#16975,#16976);
#15013=AXIS2_PLACEMENT_3D('',#43878,#16979,#16980);
#15014=AXIS2_PLACEMENT_3D('',#43880,#16981,#16982);
#15015=AXIS2_PLACEMENT_3D('',#43882,#16984,#16985);
#15016=AXIS2_PLACEMENT_3D('',#43886,#16988,#16989);
#15017=AXIS2_PLACEMENT_3D('',#43888,#16990,#16991);
#15018=AXIS2_PLACEMENT_3D('',#43890,#16993,#16994);
#15019=AXIS2_PLACEMENT_3D('',#43894,#16997,#16998);
#15020=AXIS2_PLACEMENT_3D('',#43896,#16999,#17000);
#15021=AXIS2_PLACEMENT_3D('',#43898,#17002,#17003);
#15022=AXIS2_PLACEMENT_3D('',#43902,#17006,#17007);
#15023=AXIS2_PLACEMENT_3D('',#43904,#17008,#17009);
#15024=AXIS2_PLACEMENT_3D('',#43906,#17011,#17012);
#15025=AXIS2_PLACEMENT_3D('',#43910,#17014,#17015);
#15026=AXIS2_PLACEMENT_3D('',#43912,#17017,#17018);
#15027=AXIS2_PLACEMENT_3D('',#43916,#17021,#17022);
#15028=AXIS2_PLACEMENT_3D('',#43918,#17023,#17024);
#15029=AXIS2_PLACEMENT_3D('',#43920,#17026,#17027);
#15030=AXIS2_PLACEMENT_3D('',#43923,#17029,#17030);
#15031=AXIS2_PLACEMENT_3D('',#43924,#17031,#17032);
#15032=AXIS2_PLACEMENT_3D('',#43927,#17034,#17035);
#15033=AXIS2_PLACEMENT_3D('',#43928,#17036,#17037);
#15034=AXIS2_PLACEMENT_3D('',#43931,#17039,#17040);
#15035=AXIS2_PLACEMENT_3D('',#43932,#17041,#17042);
#15036=AXIS2_PLACEMENT_3D('',#43934,#17044,#17045);
#15037=AXIS2_PLACEMENT_3D('',#43937,#17047,#17048);
#15038=AXIS2_PLACEMENT_3D('',#43938,#17049,#17050);
#15039=AXIS2_PLACEMENT_3D('',#43941,#17052,#17053);
#15040=AXIS2_PLACEMENT_3D('',#43942,#17054,#17055);
#15041=AXIS2_PLACEMENT_3D('',#43944,#17057,#17058);
#15042=AXIS2_PLACEMENT_3D('',#43946,#17060,#17061);
#15043=AXIS2_PLACEMENT_3D('',#43948,#17063,#17064);
#15044=AXIS2_PLACEMENT_3D('',#43950,#17066,#17067);
#15045=AXIS2_PLACEMENT_3D('',#43952,#17069,#17070);
#15046=AXIS2_PLACEMENT_3D('',#43954,#17072,#17073);
#15047=AXIS2_PLACEMENT_3D('',#43956,#17075,#17076);
#15048=AXIS2_PLACEMENT_3D('',#43958,#17078,#17079);
#15049=AXIS2_PLACEMENT_3D('',#43960,#17081,#17082);
#15050=AXIS2_PLACEMENT_3D('',#43962,#17084,#17085);
#15051=AXIS2_PLACEMENT_3D('',#43964,#17087,#17088);
#15052=AXIS2_PLACEMENT_3D('',#43966,#17090,#17091);
#16187=DIRECTION('axis',(0.,0.,1.));
#16188=DIRECTION('refdir',(1.,0.,0.));
#16189=DIRECTION('center_axis',(0.,0.,-1.));
#16190=DIRECTION('ref_axis',(1.,0.,0.));
#16191=DIRECTION('',(0.,0.,-1.));
#16192=DIRECTION('center_axis',(0.,0.,1.));
#16193=DIRECTION('ref_axis',(1.,0.,0.));
#16194=DIRECTION('',(0.,0.,-1.));
#16195=DIRECTION('center_axis',(0.,0.,1.));
#16196=DIRECTION('ref_axis',(1.,0.,0.));
#16197=DIRECTION('center_axis',(0.,0.,1.));
#16198=DIRECTION('ref_axis',(1.,0.,0.));
#16199=DIRECTION('center_axis',(0.,0.,-1.));
#16200=DIRECTION('ref_axis',(1.,0.,0.));
#16201=DIRECTION('',(0.,0.,-1.));
#16202=DIRECTION('center_axis',(0.,0.,-1.));
#16203=DIRECTION('ref_axis',(1.,0.,0.));
#16204=DIRECTION('',(0.,0.,-1.));
#16205=DIRECTION('center_axis',(0.,0.,-1.));
#16206=DIRECTION('ref_axis',(1.,0.,0.));
#16207=DIRECTION('',(0.,0.,-1.));
#16208=DIRECTION('center_axis',(0.,0.,-1.));
#16209=DIRECTION('ref_axis',(1.,0.,0.));
#16210=DIRECTION('',(0.,0.,-1.));
#16211=DIRECTION('center_axis',(0.,0.,-1.));
#16212=DIRECTION('ref_axis',(1.,0.,0.));
#16213=DIRECTION('',(0.,0.,-1.));
#16214=DIRECTION('center_axis',(0.,0.,-1.));
#16215=DIRECTION('ref_axis',(1.,0.,0.));
#16216=DIRECTION('',(0.,0.,-1.));
#16217=DIRECTION('center_axis',(0.,0.,-1.));
#16218=DIRECTION('ref_axis',(1.,0.,0.));
#16219=DIRECTION('',(0.,0.,-1.));
#16220=DIRECTION('center_axis',(0.,0.,-1.));
#16221=DIRECTION('ref_axis',(1.,0.,0.));
#16222=DIRECTION('',(0.,0.,-1.));
#16223=DIRECTION('center_axis',(0.,0.,-1.));
#16224=DIRECTION('ref_axis',(1.,0.,0.));
#16225=DIRECTION('',(0.,0.,-1.));
#16226=DIRECTION('center_axis',(0.,0.,-1.));
#16227=DIRECTION('ref_axis',(1.,0.,0.));
#16228=DIRECTION('',(0.,0.,-1.));
#16229=DIRECTION('center_axis',(0.,0.,-1.));
#16230=DIRECTION('ref_axis',(1.,0.,0.));
#16231=DIRECTION('',(0.,0.,-1.));
#16232=DIRECTION('center_axis',(0.,0.,-1.));
#16233=DIRECTION('ref_axis',(1.,0.,0.));
#16234=DIRECTION('',(0.,0.,-1.));
#16235=DIRECTION('center_axis',(0.,0.,-1.));
#16236=DIRECTION('ref_axis',(1.,0.,0.));
#16237=DIRECTION('',(0.,0.,-1.));
#16238=DIRECTION('center_axis',(0.,0.,-1.));
#16239=DIRECTION('ref_axis',(1.,0.,0.));
#16240=DIRECTION('',(0.,0.,-1.));
#16241=DIRECTION('center_axis',(0.,0.,-1.));
#16242=DIRECTION('ref_axis',(1.,0.,0.));
#16243=DIRECTION('',(0.,0.,-1.));
#16244=DIRECTION('center_axis',(0.,0.,-1.));
#16245=DIRECTION('ref_axis',(1.,0.,0.));
#16246=DIRECTION('',(0.,0.,-1.));
#16247=DIRECTION('center_axis',(0.,0.,-1.));
#16248=DIRECTION('ref_axis',(1.,0.,0.));
#16249=DIRECTION('',(0.,0.,-1.));
#16250=DIRECTION('center_axis',(0.,0.,-1.));
#16251=DIRECTION('ref_axis',(1.,0.,0.));
#16252=DIRECTION('',(0.,0.,-1.));
#16253=DIRECTION('center_axis',(0.,0.,-1.));
#16254=DIRECTION('ref_axis',(1.,0.,0.));
#16255=DIRECTION('',(0.,0.,-1.));
#16256=DIRECTION('center_axis',(0.,0.,-1.));
#16257=DIRECTION('ref_axis',(1.,0.,0.));
#16258=DIRECTION('',(0.,0.,-1.));
#16259=DIRECTION('center_axis',(0.,0.,-1.));
#16260=DIRECTION('ref_axis',(1.,0.,0.));
#16261=DIRECTION('',(0.,0.,-1.));
#16262=DIRECTION('center_axis',(0.,0.,-1.));
#16263=DIRECTION('ref_axis',(1.,0.,0.));
#16264=DIRECTION('',(0.,0.,-1.));
#16265=DIRECTION('center_axis',(0.,0.,-1.));
#16266=DIRECTION('ref_axis',(1.,0.,0.));
#16267=DIRECTION('',(0.,0.,-1.));
#16268=DIRECTION('center_axis',(0.,0.,-1.));
#16269=DIRECTION('ref_axis',(0.938097899428847,-0.346370222575766,0.));
#16270=DIRECTION('',(0.,0.,-1.));
#16271=DIRECTION('center_axis',(0.,0.,-1.));
#16272=DIRECTION('ref_axis',(1.,0.,0.));
#16273=DIRECTION('center_axis',(0.,0.,-1.));
#16274=DIRECTION('ref_axis',(0.793346897669268,0.608769825105144,0.));
#16275=DIRECTION('',(1.22464679914735E-16,3.85574710022057E-30,-1.));
#16276=DIRECTION('center_axis',(0.,0.,1.));
#16277=DIRECTION('ref_axis',(1.,3.16070290694603E-14,0.));
#16278=DIRECTION('center_axis',(0.,0.,-1.));
#16279=DIRECTION('ref_axis',(1.,3.16070290694603E-14,0.));
#16280=DIRECTION('',(1.22464679914735E-16,3.85574710022057E-30,-1.));
#16281=DIRECTION('center_axis',(0.,0.,-1.));
#16282=DIRECTION('ref_axis',(1.,3.16070290694603E-14,0.));
#16283=DIRECTION('',(1.22464679914735E-16,3.85574710022057E-30,-1.));
#16284=DIRECTION('center_axis',(0.,0.,-1.));
#16285=DIRECTION('ref_axis',(1.,3.16070290694603E-14,0.));
#16286=DIRECTION('',(1.22464679914735E-16,3.85574710022057E-30,-1.));
#16287=DIRECTION('center_axis',(0.,0.,-1.));
#16288=DIRECTION('ref_axis',(1.,3.16070290694603E-14,0.));
#16289=DIRECTION('',(1.22464679914735E-16,3.85574710022057E-30,-1.));
#16290=DIRECTION('center_axis',(0.,0.,-1.));
#16291=DIRECTION('ref_axis',(1.,3.16070290694603E-14,0.));
#16292=DIRECTION('',(1.22464679914735E-16,3.85574710022057E-30,-1.));
#16293=DIRECTION('center_axis',(0.,0.,-1.));
#16294=DIRECTION('ref_axis',(1.,3.16070290694603E-14,0.));
#16295=DIRECTION('',(1.22464679914735E-16,3.85574710022057E-30,-1.));
#16296=DIRECTION('center_axis',(0.,0.,-1.));
#16297=DIRECTION('ref_axis',(1.,3.16070290694603E-14,0.));
#16298=DIRECTION('',(1.22464679914735E-16,3.85574710022057E-30,-1.));
#16299=DIRECTION('center_axis',(0.,0.,-1.));
#16300=DIRECTION('ref_axis',(1.,3.16070290694603E-14,0.));
#16301=DIRECTION('',(1.22464679914735E-16,3.85574710022057E-30,-1.));
#16302=DIRECTION('center_axis',(0.,0.,-1.));
#16303=DIRECTION('ref_axis',(1.,3.16070290694603E-14,0.));
#16304=DIRECTION('',(1.22464679914735E-16,3.85574710022057E-30,-1.));
#16305=DIRECTION('center_axis',(0.,0.,-1.));
#16306=DIRECTION('ref_axis',(1.,3.16070290694603E-14,0.));
#16307=DIRECTION('',(1.22464679914735E-16,3.85574710022057E-30,-1.));
#16308=DIRECTION('center_axis',(0.,0.,-1.));
#16309=DIRECTION('ref_axis',(1.,3.16070290694603E-14,0.));
#16310=DIRECTION('',(1.22464679914735E-16,3.85574710022057E-30,-1.));
#16311=DIRECTION('center_axis',(0.,0.,-1.));
#16312=DIRECTION('ref_axis',(1.,3.16070290694603E-14,0.));
#16313=DIRECTION('',(1.22464679914735E-16,3.85574710022057E-30,-1.));
#16314=DIRECTION('center_axis',(0.,0.,-1.));
#16315=DIRECTION('ref_axis',(1.,3.16070290694603E-14,0.));
#16316=DIRECTION('',(1.22464679914735E-16,3.85574710022057E-30,-1.));
#16317=DIRECTION('center_axis',(0.,0.,-1.));
#16318=DIRECTION('ref_axis',(1.,3.16070290694603E-14,0.));
#16319=DIRECTION('',(1.22464679914735E-16,3.85574710022057E-30,-1.));
#16320=DIRECTION('center_axis',(0.,0.,-1.));
#16321=DIRECTION('ref_axis',(1.,3.16070290694603E-14,0.));
#16322=DIRECTION('',(1.22464679914735E-16,3.85574710022057E-30,-1.));
#16323=DIRECTION('center_axis',(0.,0.,-1.));
#16324=DIRECTION('ref_axis',(1.,3.16070290694603E-14,0.));
#16325=DIRECTION('',(1.22464679914735E-16,3.85574710022057E-30,-1.));
#16326=DIRECTION('center_axis',(0.,0.,-1.));
#16327=DIRECTION('ref_axis',(1.,3.16070290694603E-14,0.));
#16328=DIRECTION('',(1.22464679914735E-16,3.85574710022057E-30,-1.));
#16329=DIRECTION('center_axis',(0.,0.,-1.));
#16330=DIRECTION('ref_axis',(1.,3.16070290694603E-14,0.));
#16331=DIRECTION('',(1.22464679914735E-16,3.85574710022057E-30,-1.));
#16332=DIRECTION('center_axis',(0.,0.,-1.));
#16333=DIRECTION('ref_axis',(1.,3.16070290694603E-14,0.));
#16334=DIRECTION('',(1.22464679914735E-16,3.85574710022057E-30,-1.));
#16335=DIRECTION('center_axis',(0.,0.,-1.));
#16336=DIRECTION('ref_axis',(1.,3.16070290694603E-14,0.));
#16337=DIRECTION('',(1.22464679914735E-16,3.85574710022057E-30,-1.));
#16338=DIRECTION('center_axis',(0.,0.,-1.));
#16339=DIRECTION('ref_axis',(1.,3.16070290694603E-14,0.));
#16340=DIRECTION('',(1.22464679914735E-16,3.85574710022057E-30,-1.));
#16341=DIRECTION('center_axis',(0.,0.,-1.));
#16342=DIRECTION('ref_axis',(1.,3.16070290694603E-14,0.));
#16343=DIRECTION('',(1.22464679914735E-16,3.85574710022057E-30,-1.));
#16344=DIRECTION('center_axis',(0.,0.,-1.));
#16345=DIRECTION('ref_axis',(1.,3.16070290694603E-14,0.));
#16346=DIRECTION('',(1.22464679914735E-16,3.85574710022057E-30,-1.));
#16347=DIRECTION('center_axis',(0.,0.,-1.));
#16348=DIRECTION('ref_axis',(-0.6087766502803,-0.793341660366766,0.));
#16349=DIRECTION('',(1.22464679914735E-16,3.85574710022057E-30,-1.));
#16350=DIRECTION('center_axis',(0.,0.,-1.));
#16351=DIRECTION('ref_axis',(1.,3.16070290694603E-14,0.));
#16352=DIRECTION('center_axis',(0.,0.,1.));
#16353=DIRECTION('ref_axis',(-1.,0.,0.));
#16354=DIRECTION('',(0.,0.,1.));
#16355=DIRECTION('center_axis',(0.,0.,-1.));
#16356=DIRECTION('ref_axis',(-1.,0.,0.));
#16357=DIRECTION('',(0.,0.,1.));
#16358=DIRECTION('center_axis',(0.,0.,-1.));
#16359=DIRECTION('ref_axis',(-1.,0.,0.));
#16360=DIRECTION('center_axis',(0.,0.,-1.));
#16361=DIRECTION('ref_axis',(-1.,0.,0.));
#16362=DIRECTION('center_axis',(0.,0.,1.));
#16363=DIRECTION('ref_axis',(-1.,0.,0.));
#16364=DIRECTION('',(0.,0.,1.));
#16365=DIRECTION('center_axis',(0.,0.,1.));
#16366=DIRECTION('ref_axis',(-1.,0.,0.));
#16367=DIRECTION('',(0.,0.,1.));
#16368=DIRECTION('center_axis',(0.,0.,1.));
#16369=DIRECTION('ref_axis',(-1.,0.,0.));
#16370=DIRECTION('',(0.,0.,1.));
#16371=DIRECTION('center_axis',(0.,0.,1.));
#16372=DIRECTION('ref_axis',(-1.,0.,0.));
#16373=DIRECTION('',(0.,0.,1.));
#16374=DIRECTION('center_axis',(0.,0.,1.));
#16375=DIRECTION('ref_axis',(-1.,0.,0.));
#16376=DIRECTION('',(0.,0.,1.));
#16377=DIRECTION('center_axis',(0.,0.,1.));
#16378=DIRECTION('ref_axis',(-1.,0.,0.));
#16379=DIRECTION('',(0.,0.,1.));
#16380=DIRECTION('center_axis',(0.,0.,1.));
#16381=DIRECTION('ref_axis',(-1.,0.,0.));
#16382=DIRECTION('',(0.,0.,1.));
#16383=DIRECTION('center_axis',(0.,0.,1.));
#16384=DIRECTION('ref_axis',(-1.,0.,0.));
#16385=DIRECTION('',(0.,0.,1.));
#16386=DIRECTION('center_axis',(0.,0.,1.));
#16387=DIRECTION('ref_axis',(-1.,0.,0.));
#16388=DIRECTION('',(0.,0.,1.));
#16389=DIRECTION('center_axis',(0.,0.,1.));
#16390=DIRECTION('ref_axis',(-1.,0.,0.));
#16391=DIRECTION('',(0.,0.,1.));
#16392=DIRECTION('center_axis',(0.,0.,1.));
#16393=DIRECTION('ref_axis',(-1.,0.,0.));
#16394=DIRECTION('',(0.,0.,1.));
#16395=DIRECTION('center_axis',(0.,0.,1.));
#16396=DIRECTION('ref_axis',(-1.,0.,0.));
#16397=DIRECTION('',(0.,0.,1.));
#16398=DIRECTION('center_axis',(0.,0.,1.));
#16399=DIRECTION('ref_axis',(-1.,0.,0.));
#16400=DIRECTION('',(0.,0.,1.));
#16401=DIRECTION('center_axis',(0.,0.,1.));
#16402=DIRECTION('ref_axis',(-1.,0.,0.));
#16403=DIRECTION('',(0.,0.,1.));
#16404=DIRECTION('center_axis',(0.,0.,1.));
#16405=DIRECTION('ref_axis',(-1.,0.,0.));
#16406=DIRECTION('',(0.,0.,1.));
#16407=DIRECTION('center_axis',(0.,0.,1.));
#16408=DIRECTION('ref_axis',(-1.,0.,0.));
#16409=DIRECTION('',(0.,0.,1.));
#16410=DIRECTION('center_axis',(0.,0.,1.));
#16411=DIRECTION('ref_axis',(-1.,0.,0.));
#16412=DIRECTION('',(0.,0.,1.));
#16413=DIRECTION('center_axis',(0.,0.,1.));
#16414=DIRECTION('ref_axis',(-1.,0.,0.));
#16415=DIRECTION('',(0.,0.,1.));
#16416=DIRECTION('center_axis',(0.,0.,1.));
#16417=DIRECTION('ref_axis',(-1.,0.,0.));
#16418=DIRECTION('',(0.,0.,1.));
#16419=DIRECTION('center_axis',(0.,0.,1.));
#16420=DIRECTION('ref_axis',(-1.,0.,0.));
#16421=DIRECTION('',(0.,0.,1.));
#16422=DIRECTION('center_axis',(0.,0.,1.));
#16423=DIRECTION('ref_axis',(-1.,0.,0.));
#16424=DIRECTION('',(0.,0.,1.));
#16425=DIRECTION('center_axis',(0.,0.,1.));
#16426=DIRECTION('ref_axis',(-1.,0.,0.));
#16427=DIRECTION('',(0.,0.,1.));
#16428=DIRECTION('center_axis',(0.,0.,1.));
#16429=DIRECTION('ref_axis',(-1.,0.,0.));
#16430=DIRECTION('',(0.,0.,1.));
#16431=DIRECTION('center_axis',(0.,0.,1.));
#16432=DIRECTION('ref_axis',(-1.,0.,0.));
#16433=DIRECTION('',(0.,0.,1.));
#16434=DIRECTION('center_axis',(0.,0.,1.));
#16435=DIRECTION('ref_axis',(-1.,0.,0.));
#16436=DIRECTION('',(0.,0.,1.));
#16437=DIRECTION('center_axis',(0.,0.,1.));
#16438=DIRECTION('ref_axis',(-1.,0.,0.));
#16439=DIRECTION('',(0.,0.,1.));
#16440=DIRECTION('center_axis',(0.,0.,1.));
#16441=DIRECTION('ref_axis',(-1.,0.,0.));
#16442=DIRECTION('',(0.,0.,1.));
#16443=DIRECTION('center_axis',(0.,0.,1.));
#16444=DIRECTION('ref_axis',(-1.,0.,0.));
#16445=DIRECTION('',(0.,0.,1.));
#16446=DIRECTION('center_axis',(0.,0.,1.));
#16447=DIRECTION('ref_axis',(-1.,0.,0.));
#16448=DIRECTION('',(0.,0.,1.));
#16449=DIRECTION('center_axis',(0.,0.,1.));
#16450=DIRECTION('ref_axis',(-1.,0.,0.));
#16451=DIRECTION('',(0.,0.,1.));
#16452=DIRECTION('center_axis',(0.,0.,1.));
#16453=DIRECTION('ref_axis',(-1.,0.,0.));
#16454=DIRECTION('',(0.,0.,1.));
#16455=DIRECTION('center_axis',(0.,0.,1.));
#16456=DIRECTION('ref_axis',(-1.,0.,0.));
#16457=DIRECTION('',(0.,0.,1.));
#16458=DIRECTION('center_axis',(0.,0.,1.));
#16459=DIRECTION('ref_axis',(-1.,0.,0.));
#16460=DIRECTION('',(0.,0.,1.));
#16461=DIRECTION('center_axis',(0.,0.,1.));
#16462=DIRECTION('ref_axis',(-1.,0.,0.));
#16463=DIRECTION('',(0.,0.,1.));
#16464=DIRECTION('center_axis',(0.,0.,1.));
#16465=DIRECTION('ref_axis',(-1.,0.,0.));
#16466=DIRECTION('',(0.,0.,1.));
#16467=DIRECTION('center_axis',(0.,0.,1.));
#16468=DIRECTION('ref_axis',(-1.,0.,0.));
#16469=DIRECTION('',(0.,0.,1.));
#16470=DIRECTION('center_axis',(0.,0.,1.));
#16471=DIRECTION('ref_axis',(-1.,0.,0.));
#16472=DIRECTION('',(0.,0.,1.));
#16473=DIRECTION('center_axis',(0.,0.,1.));
#16474=DIRECTION('ref_axis',(-1.,0.,0.));
#16475=DIRECTION('',(0.,0.,1.));
#16476=DIRECTION('center_axis',(0.,0.,1.));
#16477=DIRECTION('ref_axis',(-0.938097369934915,-0.346371656636617,0.));
#16478=DIRECTION('',(0.,0.,1.));
#16479=DIRECTION('center_axis',(0.,0.,-1.));
#16480=DIRECTION('ref_axis',(-1.,0.,0.));
#16481=DIRECTION('center_axis',(0.,0.,1.));
#16482=DIRECTION('ref_axis',(-0.793344496203991,0.608772954674266,0.));
#16483=DIRECTION('',(-1.22464679914735E-16,4.47534497895031E-29,1.));
#16484=DIRECTION('center_axis',(0.,0.,-1.));
#16485=DIRECTION('ref_axis',(-1.,3.65562114876707E-13,0.));
#16486=DIRECTION('center_axis',(0.,0.,1.));
#16487=DIRECTION('ref_axis',(-1.,3.65562114876707E-13,0.));
#16488=DIRECTION('',(-1.22464679914735E-16,4.47534497895031E-29,1.));
#16489=DIRECTION('center_axis',(0.,0.,1.));
#16490=DIRECTION('ref_axis',(-1.,3.65562114876707E-13,0.));
#16491=DIRECTION('',(-1.22464679914735E-16,4.47534497895031E-29,1.));
#16492=DIRECTION('center_axis',(0.,0.,1.));
#16493=DIRECTION('ref_axis',(-1.,3.65562114876707E-13,0.));
#16494=DIRECTION('',(-1.22464679914735E-16,4.47534497895031E-29,1.));
#16495=DIRECTION('center_axis',(0.,0.,1.));
#16496=DIRECTION('ref_axis',(-1.,3.65562114876707E-13,0.));
#16497=DIRECTION('',(-1.22464679914735E-16,4.47534497895031E-29,1.));
#16498=DIRECTION('center_axis',(0.,0.,1.));
#16499=DIRECTION('ref_axis',(-1.,3.65562114876707E-13,0.));
#16500=DIRECTION('',(-1.22464679914735E-16,4.47534497895031E-29,1.));
#16501=DIRECTION('center_axis',(0.,0.,1.));
#16502=DIRECTION('ref_axis',(-1.,3.65562114876707E-13,0.));
#16503=DIRECTION('',(-1.22464679914735E-16,4.47534497895031E-29,1.));
#16504=DIRECTION('center_axis',(0.,0.,1.));
#16505=DIRECTION('ref_axis',(-1.,3.65562114876707E-13,0.));
#16506=DIRECTION('',(-1.22464679914735E-16,4.47534497895031E-29,1.));
#16507=DIRECTION('center_axis',(0.,0.,1.));
#16508=DIRECTION('ref_axis',(-1.,3.65562114876707E-13,0.));
#16509=DIRECTION('',(-1.22464679914735E-16,4.47534497895031E-29,1.));
#16510=DIRECTION('center_axis',(0.,0.,1.));
#16511=DIRECTION('ref_axis',(-1.,3.65562114876707E-13,0.));
#16512=DIRECTION('',(-1.22464679914735E-16,4.47534497895031E-29,1.));
#16513=DIRECTION('center_axis',(0.,0.,1.));
#16514=DIRECTION('ref_axis',(-1.,3.65562114876707E-13,0.));
#16515=DIRECTION('',(-1.22464679914735E-16,4.47534497895031E-29,1.));
#16516=DIRECTION('center_axis',(0.,0.,1.));
#16517=DIRECTION('ref_axis',(-1.,3.65562114876707E-13,0.));
#16518=DIRECTION('',(-1.22464679914735E-16,4.47534497895031E-29,1.));
#16519=DIRECTION('center_axis',(0.,0.,1.));
#16520=DIRECTION('ref_axis',(-1.,3.65562114876707E-13,0.));
#16521=DIRECTION('',(-1.22464679914735E-16,4.47534497895031E-29,1.));
#16522=DIRECTION('center_axis',(0.,0.,1.));
#16523=DIRECTION('ref_axis',(-1.,3.65562114876707E-13,0.));
#16524=DIRECTION('',(-1.22464679914735E-16,4.47534497895031E-29,1.));
#16525=DIRECTION('center_axis',(0.,0.,1.));
#16526=DIRECTION('ref_axis',(-1.,3.65562114876707E-13,0.));
#16527=DIRECTION('',(-1.22464679914735E-16,4.47534497895031E-29,1.));
#16528=DIRECTION('center_axis',(0.,0.,1.));
#16529=DIRECTION('ref_axis',(-1.,3.65562114876707E-13,0.));
#16530=DIRECTION('',(-1.22464679914735E-16,4.47534497895031E-29,1.));
#16531=DIRECTION('center_axis',(0.,0.,1.));
#16532=DIRECTION('ref_axis',(-1.,3.65562114876707E-13,0.));
#16533=DIRECTION('',(-1.22464679914735E-16,4.47534497895031E-29,1.));
#16534=DIRECTION('center_axis',(0.,0.,1.));
#16535=DIRECTION('ref_axis',(-1.,3.65562114876707E-13,0.));
#16536=DIRECTION('',(-1.22464679914735E-16,4.47534497895031E-29,1.));
#16537=DIRECTION('center_axis',(0.,0.,1.));
#16538=DIRECTION('ref_axis',(-1.,3.65562114876707E-13,0.));
#16539=DIRECTION('',(-1.22464679914735E-16,4.47534497895031E-29,1.));
#16540=DIRECTION('center_axis',(0.,0.,1.));
#16541=DIRECTION('ref_axis',(-1.,3.65562114876707E-13,0.));
#16542=DIRECTION('',(-1.22464679914735E-16,4.47534497895031E-29,1.));
#16543=DIRECTION('center_axis',(0.,0.,1.));
#16544=DIRECTION('ref_axis',(-1.,3.65562114876707E-13,0.));
#16545=DIRECTION('',(-1.22464679914735E-16,4.47534497895031E-29,1.));
#16546=DIRECTION('center_axis',(0.,0.,1.));
#16547=DIRECTION('ref_axis',(-1.,3.65562114876707E-13,0.));
#16548=DIRECTION('',(-1.22464679914735E-16,4.47534497895031E-29,1.));
#16549=DIRECTION('center_axis',(0.,0.,1.));
#16550=DIRECTION('ref_axis',(-1.,3.65562114876707E-13,0.));
#16551=DIRECTION('',(-1.22464679914735E-16,4.47534497895031E-29,1.));
#16552=DIRECTION('center_axis',(0.,0.,1.));
#16553=DIRECTION('ref_axis',(-1.,3.65562114876707E-13,0.));
#16554=DIRECTION('',(-1.22464679914735E-16,4.47534497895031E-29,1.));
#16555=DIRECTION('center_axis',(0.,0.,1.));
#16556=DIRECTION('ref_axis',(-1.,3.65562114876707E-13,0.));
#16557=DIRECTION('',(-1.22464679914735E-16,4.47534497895031E-29,1.));
#16558=DIRECTION('center_axis',(0.,0.,1.));
#16559=DIRECTION('ref_axis',(-1.,3.65562114876707E-13,0.));
#16560=DIRECTION('',(-1.22464679914735E-16,4.47534497895031E-29,1.));
#16561=DIRECTION('center_axis',(0.,0.,1.));
#16562=DIRECTION('ref_axis',(-1.,3.65562114876707E-13,0.));
#16563=DIRECTION('',(-1.22464679914735E-16,4.47534497895031E-29,1.));
#16564=DIRECTION('center_axis',(0.,0.,1.));
#16565=DIRECTION('ref_axis',(-1.,3.65562114876707E-13,0.));
#16566=DIRECTION('',(-1.22464679914735E-16,4.47534497895031E-29,1.));
#16567=DIRECTION('center_axis',(0.,0.,1.));
#16568=DIRECTION('ref_axis',(-1.,3.65562114876707E-13,0.));
#16569=DIRECTION('',(-1.22464679914735E-16,4.47534497895031E-29,1.));
#16570=DIRECTION('center_axis',(0.,0.,1.));
#16571=DIRECTION('ref_axis',(-1.,3.65562114876707E-13,0.));
#16572=DIRECTION('',(-1.22464679914735E-16,4.47534497895031E-29,1.));
#16573=DIRECTION('center_axis',(0.,0.,1.));
#16574=DIRECTION('ref_axis',(-1.,3.65562114876707E-13,0.));
#16575=DIRECTION('',(-1.22464679914735E-16,4.47534497895031E-29,1.));
#16576=DIRECTION('center_axis',(0.,0.,1.));
#16577=DIRECTION('ref_axis',(-1.,3.65562114876707E-13,0.));
#16578=DIRECTION('',(-1.22464679914735E-16,4.47534497895031E-29,1.));
#16579=DIRECTION('center_axis',(0.,0.,1.));
#16580=DIRECTION('ref_axis',(-1.,3.65562114876707E-13,0.));
#16581=DIRECTION('',(-1.22464679914735E-16,4.47534497895031E-29,1.));
#16582=DIRECTION('center_axis',(0.,0.,1.));
#16583=DIRECTION('ref_axis',(-1.,3.65562114876707E-13,0.));
#16584=DIRECTION('',(-1.22464679914735E-16,4.47534497895031E-29,1.));
#16585=DIRECTION('center_axis',(0.,0.,1.));
#16586=DIRECTION('ref_axis',(-1.,3.65562114876707E-13,0.));
#16587=DIRECTION('',(-1.22464679914735E-16,4.47534497895031E-29,1.));
#16588=DIRECTION('center_axis',(0.,0.,1.));
#16589=DIRECTION('ref_axis',(-1.,3.65562114876707E-13,0.));
#16590=DIRECTION('',(-1.22464679914735E-16,4.47534497895031E-29,1.));
#16591=DIRECTION('center_axis',(0.,0.,1.));
#16592=DIRECTION('ref_axis',(-1.,3.65562114876707E-13,0.));
#16593=DIRECTION('',(-1.22464679914735E-16,4.47534497895031E-29,1.));
#16594=DIRECTION('center_axis',(0.,0.,1.));
#16595=DIRECTION('ref_axis',(-1.,3.65562114876707E-13,0.));
#16596=DIRECTION('',(-1.22464679914735E-16,4.47534497895031E-29,1.));
#16597=DIRECTION('center_axis',(0.,0.,1.));
#16598=DIRECTION('ref_axis',(-1.,3.65562114876707E-13,0.));
#16599=DIRECTION('',(-1.22464679914735E-16,4.47534497895031E-29,1.));
#16600=DIRECTION('center_axis',(0.,0.,1.));
#16601=DIRECTION('ref_axis',(0.608777863132373,-0.793340729674193,0.));
#16602=DIRECTION('',(-1.22464679914735E-16,4.47534497895031E-29,1.));
#16603=DIRECTION('center_axis',(0.,0.,1.));
#16604=DIRECTION('ref_axis',(-1.,3.65562114876707E-13,0.));
#16605=DIRECTION('center_axis',(0.,0.,1.));
#16606=DIRECTION('ref_axis',(1.,0.,0.));
#16607=DIRECTION('center_axis',(0.,0.,1.));
#16608=DIRECTION('ref_axis',(-1.,3.65562114876707E-13,0.));
#16609=DIRECTION('center_axis',(0.,0.,1.));
#16610=DIRECTION('ref_axis',(-1.,0.,0.));
#16611=DIRECTION('center_axis',(0.,0.,1.));
#16612=DIRECTION('ref_axis',(-1.,0.,0.));
#16613=DIRECTION('center_axis',(0.,0.,-1.));
#16614=DIRECTION('ref_axis',(1.,0.,0.));
#16615=DIRECTION('center_axis',(0.,0.,1.));
#16616=DIRECTION('ref_axis',(1.,0.,0.));
#16617=DIRECTION('center_axis',(0.,0.,-1.));
#16618=DIRECTION('ref_axis',(1.,3.16070290694603E-14,0.));
#16619=DIRECTION('center_axis',(0.,0.,-1.));
#16620=DIRECTION('ref_axis',(1.,0.,0.));
#16621=DIRECTION('center_axis',(0.,0.,-1.));
#16622=DIRECTION('ref_axis',(1.,0.,0.));
#16623=DIRECTION('center_axis',(0.,0.,1.));
#16624=DIRECTION('ref_axis',(1.,0.,0.));
#16625=DIRECTION('center_axis',(0.,0.,1.));
#16626=DIRECTION('ref_axis',(0.707106781186548,-0.707106781186547,0.));
#16627=DIRECTION('center_axis',(0.,0.,-1.));
#16628=DIRECTION('ref_axis',(0.707106781186548,-0.707106781186547,0.));
#16629=DIRECTION('',(0.,0.,-1.));
#16630=DIRECTION('center_axis',(0.,0.,1.));
#16631=DIRECTION('ref_axis',(0.707106781186548,-0.707106781186547,0.));
#16632=DIRECTION('',(0.,0.,1.));
#16633=DIRECTION('center_axis',(0.,-1.,0.));
#16634=DIRECTION('ref_axis',(1.,0.,0.));
#16635=DIRECTION('',(1.,0.,0.));
#16636=DIRECTION('',(0.,0.,1.));
#16637=DIRECTION('',(-1.,0.,0.));
#16638=DIRECTION('center_axis',(0.,0.,1.));
#16639=DIRECTION('ref_axis',(1.,0.,0.));
#16640=DIRECTION('',(0.,1.,0.));
#16641=DIRECTION('center_axis',(0.,0.,1.));
#16642=DIRECTION('ref_axis',(-0.707106781186548,0.707106781186547,0.));
#16643=DIRECTION('',(1.,0.,0.));
#16644=DIRECTION('center_axis',(0.,0.,1.));
#16645=DIRECTION('ref_axis',(0.707106781186547,0.707106781186548,0.));
#16646=DIRECTION('',(0.,-1.,0.));
#16647=DIRECTION('center_axis',(0.,0.,1.));
#16648=DIRECTION('ref_axis',(0.707106781186548,-0.707106781186548,0.));
#16649=DIRECTION('',(-1.,0.,0.));
#16650=DIRECTION('center_axis',(0.,0.,1.));
#16651=DIRECTION('ref_axis',(-0.707106781186548,-0.707106781186548,0.));
#16652=DIRECTION('',(0.,1.,0.));
#16653=DIRECTION('center_axis',(0.,0.,-1.));
#16654=DIRECTION('ref_axis',(0.707106781186548,0.707106781186547,0.));
#16655=DIRECTION('',(-1.,0.,0.));
#16656=DIRECTION('center_axis',(0.,0.,-1.));
#16657=DIRECTION('ref_axis',(-0.707106781186548,0.707106781186547,0.));
#16658=DIRECTION('',(0.,-1.,0.));
#16659=DIRECTION('center_axis',(0.,0.,-1.));
#16660=DIRECTION('ref_axis',(-0.707106781186548,-0.707106781186548,0.));
#16661=DIRECTION('',(1.,0.,0.));
#16662=DIRECTION('center_axis',(0.,0.,-1.));
#16663=DIRECTION('ref_axis',(0.707106781186547,-0.707106781186548,0.));
#16664=DIRECTION('',(0.,1.,0.));
#16665=DIRECTION('center_axis',(0.,0.,-1.));
#16666=DIRECTION('ref_axis',(0.707106781186547,0.707106781186548,0.));
#16667=DIRECTION('',(-1.,0.,0.));
#16668=DIRECTION('center_axis',(0.,0.,1.));
#16669=DIRECTION('ref_axis',(-0.707106781186547,-0.707106781186548,0.));
#16670=DIRECTION('',(0.,1.,0.));
#16671=DIRECTION('center_axis',(0.,0.,1.));
#16672=DIRECTION('ref_axis',(-0.707106781186548,0.707106781186547,0.));
#16673=DIRECTION('',(1.,0.,0.));
#16674=DIRECTION('center_axis',(0.,0.,1.));
#16675=DIRECTION('ref_axis',(0.707106781186548,0.707106781186548,0.));
#16676=DIRECTION('',(0.,-1.,0.));
#16677=DIRECTION('center_axis',(0.,0.,1.));
#16678=DIRECTION('ref_axis',(0.707106781186548,-0.707106781186548,0.));
#16679=DIRECTION('',(-1.,0.,0.));
#16680=DIRECTION('center_axis',(0.,0.,-1.));
#16681=DIRECTION('ref_axis',(-0.707106781186547,0.707106781186548,0.));
#16682=DIRECTION('',(0.,-1.,0.));
#16683=DIRECTION('center_axis',(0.,0.,-1.));
#16684=DIRECTION('ref_axis',(-0.707106781186547,-0.707106781186548,0.));
#16685=DIRECTION('',(1.,0.,0.));
#16686=DIRECTION('center_axis',(0.,0.,-1.));
#16687=DIRECTION('ref_axis',(0.707106781186548,-0.707106781186548,0.));
#16688=DIRECTION('',(0.,1.,0.));
#16689=DIRECTION('center_axis',(0.,0.,-1.));
#16690=DIRECTION('ref_axis',(0.707106781186548,0.707106781186547,0.));
#16691=DIRECTION('',(-1.,0.,0.));
#16692=DIRECTION('center_axis',(0.,0.,-1.));
#16693=DIRECTION('ref_axis',(-0.707106781186548,0.707106781186547,0.));
#16694=DIRECTION('',(0.,-1.,0.));
#16695=DIRECTION('center_axis',(0.,0.,1.));
#16696=DIRECTION('ref_axis',(0.707106781186548,-0.707106781186547,0.));
#16697=DIRECTION('',(-1.,0.,0.));
#16698=DIRECTION('center_axis',(0.,0.,1.));
#16699=DIRECTION('ref_axis',(-0.707106781186547,-0.707106781186548,0.));
#16700=DIRECTION('',(0.,1.,0.));
#16701=DIRECTION('center_axis',(0.,0.,1.));
#16702=DIRECTION('ref_axis',(-0.707106781186548,0.707106781186548,0.));
#16703=DIRECTION('',(1.,0.,0.));
#16704=DIRECTION('center_axis',(0.,0.,1.));
#16705=DIRECTION('ref_axis',(0.707106781186548,0.707106781186548,0.));
#16706=DIRECTION('',(0.,-1.,0.));
#16707=DIRECTION('center_axis',(0.,0.,-1.));
#16708=DIRECTION('ref_axis',(-0.707106781186548,-0.707106781186547,0.));
#16709=DIRECTION('',(1.,0.,0.));
#16710=DIRECTION('center_axis',(0.,0.,-1.));
#16711=DIRECTION('ref_axis',(0.707106781186548,-0.707106781186547,0.));
#16712=DIRECTION('',(0.,1.,0.));
#16713=DIRECTION('center_axis',(0.,0.,-1.));
#16714=DIRECTION('ref_axis',(0.707106781186548,0.707106781186548,0.));
#16715=DIRECTION('',(-1.,0.,0.));
#16716=DIRECTION('center_axis',(0.,0.,-1.));
#16717=DIRECTION('ref_axis',(-0.707106781186547,0.707106781186548,0.));
#16718=DIRECTION('',(0.,-1.,0.));
#16719=DIRECTION('center_axis',(0.,0.,-1.));
#16720=DIRECTION('ref_axis',(-0.707106781186547,-0.707106781186548,0.));
#16721=DIRECTION('',(1.,0.,0.));
#16722=DIRECTION('center_axis',(0.,0.,1.));
#16723=DIRECTION('ref_axis',(0.707106781186547,0.707106781186548,0.));
#16724=DIRECTION('',(0.,-1.,0.));
#16725=DIRECTION('center_axis',(0.,0.,1.));
#16726=DIRECTION('ref_axis',(0.707106781186548,-0.707106781186547,0.));
#16727=DIRECTION('',(-1.,0.,0.));
#16728=DIRECTION('center_axis',(0.,0.,1.));
#16729=DIRECTION('ref_axis',(-0.707106781186548,-0.707106781186548,0.));
#16730=DIRECTION('',(0.,1.,0.));
#16731=DIRECTION('center_axis',(0.,0.,1.));
#16732=DIRECTION('ref_axis',(-0.707106781186548,0.707106781186548,0.));
#16733=DIRECTION('',(1.,0.,0.));
#16734=DIRECTION('center_axis',(0.,0.,-1.));
#16735=DIRECTION('ref_axis',(0.707106781186547,-0.707106781186548,0.));
#16736=DIRECTION('',(0.,1.,0.));
#16737=DIRECTION('center_axis',(0.,0.,-1.));
#16738=DIRECTION('ref_axis',(0.707106781186547,0.707106781186548,0.));
#16739=DIRECTION('',(-1.,0.,0.));
#16740=DIRECTION('center_axis',(0.,0.,-1.));
#16741=DIRECTION('ref_axis',(-0.707106781186548,0.707106781186548,0.));
#16742=DIRECTION('',(0.,-1.,0.));
#16743=DIRECTION('center_axis',(0.,0.,-1.));
#16744=DIRECTION('ref_axis',(-0.707106781186548,-0.707106781186547,0.));
#16745=DIRECTION('center_axis',(0.,0.,-1.));
#16746=DIRECTION('ref_axis',(1.,0.,0.));
#16747=DIRECTION('center_axis',(0.,0.,-1.));
#16748=DIRECTION('ref_axis',(1.,0.,0.));
#16749=DIRECTION('center_axis',(0.,0.,-1.));
#16750=DIRECTION('ref_axis',(1.,0.,0.));
#16751=DIRECTION('center_axis',(0.,0.,-1.));
#16752=DIRECTION('ref_axis',(1.,0.,0.));
#16753=DIRECTION('center_axis',(0.,0.,1.));
#16754=DIRECTION('ref_axis',(-0.707106781186548,0.707106781186547,0.));
#16755=DIRECTION('center_axis',(0.,0.,-1.));
#16756=DIRECTION('ref_axis',(-0.707106781186548,0.707106781186547,0.));
#16757=DIRECTION('',(0.,0.,1.));
#16758=DIRECTION('',(0.,0.,-1.));
#16759=DIRECTION('center_axis',(0.,-1.,0.));
#16760=DIRECTION('ref_axis',(1.,0.,0.));
#16761=DIRECTION('',(-1.,0.,0.));
#16762=DIRECTION('',(0.,0.,-1.));
#16763=DIRECTION('center_axis',(0.,0.,1.));
#16764=DIRECTION('ref_axis',(0.707106781186547,0.707106781186548,0.));
#16765=DIRECTION('center_axis',(0.,0.,-1.));
#16766=DIRECTION('ref_axis',(0.707106781186547,0.707106781186548,0.));
#16767=DIRECTION('',(0.,0.,1.));
#16768=DIRECTION('center_axis',(-1.,0.,0.));
#16769=DIRECTION('ref_axis',(0.,-1.,0.));
#16770=DIRECTION('',(0.,1.,0.));
#16771=DIRECTION('',(0.,0.,-1.));
#16772=DIRECTION('center_axis',(0.,0.,1.));
#16773=DIRECTION('ref_axis',(0.707106781186548,-0.707106781186548,0.));
#16774=DIRECTION('center_axis',(0.,0.,-1.));
#16775=DIRECTION('ref_axis',(0.707106781186548,-0.707106781186548,0.));
#16776=DIRECTION('',(0.,0.,1.));
#16777=DIRECTION('center_axis',(0.,1.,0.));
#16778=DIRECTION('ref_axis',(-1.,0.,0.));
#16779=DIRECTION('',(1.,0.,0.));
#16780=DIRECTION('',(0.,0.,-1.));
#16781=DIRECTION('center_axis',(0.,0.,1.));
#16782=DIRECTION('ref_axis',(-0.707106781186548,-0.707106781186548,0.));
#16783=DIRECTION('center_axis',(0.,0.,-1.));
#16784=DIRECTION('ref_axis',(-0.707106781186548,-0.707106781186548,0.));
#16785=DIRECTION('',(0.,0.,1.));
#16786=DIRECTION('center_axis',(1.,0.,0.));
#16787=DIRECTION('ref_axis',(0.,1.,0.));
#16788=DIRECTION('',(0.,-1.,0.));
#16789=DIRECTION('',(0.,0.,-1.));
#16790=DIRECTION('center_axis',(0.,0.,1.));
#16791=DIRECTION('ref_axis',(0.707106781186548,0.707106781186547,0.));
#16792=DIRECTION('center_axis',(0.,0.,1.));
#16793=DIRECTION('ref_axis',(0.707106781186548,0.707106781186547,0.));
#16794=DIRECTION('',(0.,0.,1.));
#16795=DIRECTION('center_axis',(0.,0.,1.));
#16796=DIRECTION('ref_axis',(-0.707106781186548,0.707106781186547,0.));
#16797=DIRECTION('',(0.,0.,-1.));
#16798=DIRECTION('center_axis',(0.,0.,1.));
#16799=DIRECTION('ref_axis',(-0.707106781186548,0.707106781186547,0.));
#16800=DIRECTION('',(0.,0.,1.));
#16801=DIRECTION('center_axis',(-1.,0.,0.));
#16802=DIRECTION('ref_axis',(0.,-1.,0.));
#16803=DIRECTION('',(0.,1.,0.));
#16804=DIRECTION('',(0.,0.,-1.));
#16805=DIRECTION('center_axis',(0.,0.,1.));
#16806=DIRECTION('ref_axis',(-0.707106781186548,-0.707106781186548,0.));
#16807=DIRECTION('center_axis',(0.,0.,1.));
#16808=DIRECTION('ref_axis',(-0.707106781186548,-0.707106781186548,0.));
#16809=DIRECTION('',(0.,0.,1.));
#16810=DIRECTION('center_axis',(0.,0.,1.));
#16811=DIRECTION('ref_axis',(0.707106781186547,-0.707106781186548,0.));
#16812=DIRECTION('',(0.,0.,-1.));
#16813=DIRECTION('center_axis',(0.,0.,1.));
#16814=DIRECTION('ref_axis',(0.707106781186547,-0.707106781186548,0.));
#16815=DIRECTION('',(0.,0.,1.));
#16816=DIRECTION('center_axis',(1.,0.,0.));
#16817=DIRECTION('ref_axis',(0.,1.,0.));
#16818=DIRECTION('',(0.,-1.,0.));
#16819=DIRECTION('',(0.,0.,-1.));
#16820=DIRECTION('center_axis',(0.,0.,1.));
#16821=DIRECTION('ref_axis',(0.707106781186547,0.707106781186548,0.));
#16822=DIRECTION('center_axis',(0.,0.,1.));
#16823=DIRECTION('ref_axis',(0.707106781186547,0.707106781186548,0.));
#16824=DIRECTION('',(0.,0.,1.));
#16825=DIRECTION('center_axis',(0.,0.,1.));
#16826=DIRECTION('ref_axis',(-0.707106781186547,-0.707106781186548,0.));
#16827=DIRECTION('center_axis',(0.,0.,-1.));
#16828=DIRECTION('ref_axis',(-0.707106781186547,-0.707106781186548,0.));
#16829=DIRECTION('',(0.,0.,1.));
#16830=DIRECTION('',(0.,0.,-1.));
#16831=DIRECTION('center_axis',(1.,0.,0.));
#16832=DIRECTION('ref_axis',(0.,1.,0.));
#16833=DIRECTION('',(0.,-1.,0.));
#16834=DIRECTION('',(0.,0.,-1.));
#16835=DIRECTION('center_axis',(0.,0.,1.));
#16836=DIRECTION('ref_axis',(-0.707106781186548,0.707106781186547,0.));
#16837=DIRECTION('center_axis',(0.,0.,-1.));
#16838=DIRECTION('ref_axis',(-0.707106781186548,0.707106781186547,0.));
#16839=DIRECTION('',(0.,0.,1.));
#16840=DIRECTION('center_axis',(0.,-1.,0.));
#16841=DIRECTION('ref_axis',(1.,0.,0.));
#16842=DIRECTION('',(-1.,0.,0.));
#16843=DIRECTION('',(0.,0.,-1.));
#16844=DIRECTION('center_axis',(0.,0.,1.));
#16845=DIRECTION('ref_axis',(0.707106781186548,0.707106781186548,0.));
#16846=DIRECTION('center_axis',(0.,0.,-1.));
#16847=DIRECTION('ref_axis',(0.707106781186548,0.707106781186548,0.));
#16848=DIRECTION('',(0.,0.,1.));
#16849=DIRECTION('center_axis',(-1.,0.,0.));
#16850=DIRECTION('ref_axis',(0.,-1.,0.));
#16851=DIRECTION('',(0.,1.,0.));
#16852=DIRECTION('',(0.,0.,-1.));
#16853=DIRECTION('center_axis',(0.,0.,1.));
#16854=DIRECTION('ref_axis',(0.707106781186548,-0.707106781186548,0.));
#16855=DIRECTION('center_axis',(0.,0.,-1.));
#16856=DIRECTION('ref_axis',(0.707106781186548,-0.707106781186548,0.));
#16857=DIRECTION('',(0.,0.,1.));
#16858=DIRECTION('center_axis',(0.,1.,0.));
#16859=DIRECTION('ref_axis',(-1.,0.,0.));
#16860=DIRECTION('',(1.,0.,0.));
#16861=DIRECTION('',(0.,0.,-1.));
#16862=DIRECTION('center_axis',(0.,0.,1.));
#16863=DIRECTION('ref_axis',(-0.707106781186547,0.707106781186548,0.));
#16864=DIRECTION('center_axis',(0.,0.,1.));
#16865=DIRECTION('ref_axis',(-0.707106781186547,0.707106781186548,0.));
#16866=DIRECTION('',(0.,0.,1.));
#16867=DIRECTION('center_axis',(0.,0.,1.));
#16868=DIRECTION('ref_axis',(-0.707106781186547,-0.707106781186548,0.));
#16869=DIRECTION('',(0.,0.,-1.));
#16870=DIRECTION('center_axis',(0.,0.,1.));
#16871=DIRECTION('ref_axis',(-0.707106781186547,-0.707106781186548,0.));
#16872=DIRECTION('',(0.,0.,1.));
#16873=DIRECTION('center_axis',(0.,-1.,0.));
#16874=DIRECTION('ref_axis',(1.,0.,0.));
#16875=DIRECTION('',(-1.,0.,0.));
#16876=DIRECTION('',(0.,0.,-1.));
#16877=DIRECTION('center_axis',(0.,0.,1.));
#16878=DIRECTION('ref_axis',(0.707106781186548,-0.707106781186548,0.));
#16879=DIRECTION('center_axis',(0.,0.,1.));
#16880=DIRECTION('ref_axis',(0.707106781186548,-0.707106781186548,0.));
#16881=DIRECTION('',(0.,0.,1.));
#16882=DIRECTION('center_axis',(0.,0.,1.));
#16883=DIRECTION('ref_axis',(0.707106781186548,0.707106781186547,0.));
#16884=DIRECTION('',(0.,0.,-1.));
#16885=DIRECTION('center_axis',(0.,0.,1.));
#16886=DIRECTION('ref_axis',(0.707106781186548,0.707106781186547,0.));
#16887=DIRECTION('',(0.,0.,1.));
#16888=DIRECTION('center_axis',(0.,1.,0.));
#16889=DIRECTION('ref_axis',(-1.,0.,0.));
#16890=DIRECTION('',(1.,0.,0.));
#16891=DIRECTION('',(0.,0.,-1.));
#16892=DIRECTION('center_axis',(0.,0.,1.));
#16893=DIRECTION('ref_axis',(-0.707106781186548,0.707106781186547,0.));
#16894=DIRECTION('center_axis',(0.,0.,1.));
#16895=DIRECTION('ref_axis',(-0.707106781186548,0.707106781186547,0.));
#16896=DIRECTION('',(0.,0.,1.));
#16897=DIRECTION('center_axis',(0.,0.,1.));
#16898=DIRECTION('ref_axis',(0.707106781186548,-0.707106781186547,0.));
#16899=DIRECTION('center_axis',(0.,0.,-1.));
#16900=DIRECTION('ref_axis',(0.707106781186548,-0.707106781186547,0.));
#16901=DIRECTION('',(0.,0.,1.));
#16902=DIRECTION('',(0.,0.,-1.));
#16903=DIRECTION('center_axis',(0.,1.,0.));
#16904=DIRECTION('ref_axis',(-1.,0.,0.));
#16905=DIRECTION('',(1.,0.,0.));
#16906=DIRECTION('',(0.,0.,-1.));
#16907=DIRECTION('center_axis',(0.,0.,1.));
#16908=DIRECTION('ref_axis',(-0.707106781186547,-0.707106781186548,0.));
#16909=DIRECTION('center_axis',(0.,0.,-1.));
#16910=DIRECTION('ref_axis',(-0.707106781186547,-0.707106781186548,0.));
#16911=DIRECTION('',(0.,0.,1.));
#16912=DIRECTION('center_axis',(1.,0.,0.));
#16913=DIRECTION('ref_axis',(0.,1.,0.));
#16914=DIRECTION('',(0.,-1.,0.));
#16915=DIRECTION('',(0.,0.,-1.));
#16916=DIRECTION('center_axis',(0.,0.,1.));
#16917=DIRECTION('ref_axis',(-0.707106781186548,0.707106781186548,0.));
#16918=DIRECTION('center_axis',(0.,0.,-1.));
#16919=DIRECTION('ref_axis',(-0.707106781186548,0.707106781186548,0.));
#16920=DIRECTION('',(0.,0.,1.));
#16921=DIRECTION('center_axis',(0.,-1.,0.));
#16922=DIRECTION('ref_axis',(1.,0.,0.));
#16923=DIRECTION('',(-1.,0.,0.));
#16924=DIRECTION('',(0.,0.,-1.));
#16925=DIRECTION('center_axis',(0.,0.,1.));
#16926=DIRECTION('ref_axis',(0.707106781186548,0.707106781186548,0.));
#16927=DIRECTION('center_axis',(0.,0.,-1.));
#16928=DIRECTION('ref_axis',(0.707106781186548,0.707106781186548,0.));
#16929=DIRECTION('',(0.,0.,1.));
#16930=DIRECTION('center_axis',(-1.,0.,0.));
#16931=DIRECTION('ref_axis',(0.,-1.,0.));
#16932=DIRECTION('',(0.,1.,0.));
#16933=DIRECTION('',(0.,0.,-1.));
#16934=DIRECTION('center_axis',(0.,0.,1.));
#16935=DIRECTION('ref_axis',(-0.707106781186548,-0.707106781186547,0.));
#16936=DIRECTION('center_axis',(0.,0.,1.));
#16937=DIRECTION('ref_axis',(-0.707106781186548,-0.707106781186547,0.));
#16938=DIRECTION('',(0.,0.,1.));
#16939=DIRECTION('center_axis',(0.,0.,1.));
#16940=DIRECTION('ref_axis',(0.707106781186548,-0.707106781186547,0.));
#16941=DIRECTION('',(0.,0.,-1.));
#16942=DIRECTION('center_axis',(0.,0.,1.));
#16943=DIRECTION('ref_axis',(0.707106781186548,-0.707106781186547,0.));
#16944=DIRECTION('',(0.,0.,1.));
#16945=DIRECTION('center_axis',(1.,0.,0.));
#16946=DIRECTION('ref_axis',(0.,1.,0.));
#16947=DIRECTION('',(0.,-1.,0.));
#16948=DIRECTION('',(0.,0.,-1.));
#16949=DIRECTION('center_axis',(0.,0.,1.));
#16950=DIRECTION('ref_axis',(0.707106781186548,0.707106781186548,0.));
#16951=DIRECTION('center_axis',(0.,0.,1.));
#16952=DIRECTION('ref_axis',(0.707106781186548,0.707106781186548,0.));
#16953=DIRECTION('',(0.,0.,1.));
#16954=DIRECTION('center_axis',(0.,0.,1.));
#16955=DIRECTION('ref_axis',(-0.707106781186547,0.707106781186548,0.));
#16956=DIRECTION('',(0.,0.,-1.));
#16957=DIRECTION('center_axis',(0.,0.,1.));
#16958=DIRECTION('ref_axis',(-0.707106781186547,0.707106781186548,0.));
#16959=DIRECTION('',(0.,0.,1.));
#16960=DIRECTION('center_axis',(-1.,0.,0.));
#16961=DIRECTION('ref_axis',(0.,-1.,0.));
#16962=DIRECTION('',(0.,1.,0.));
#16963=DIRECTION('',(0.,0.,-1.));
#16964=DIRECTION('center_axis',(0.,0.,1.));
#16965=DIRECTION('ref_axis',(-0.707106781186547,-0.707106781186548,0.));
#16966=DIRECTION('center_axis',(0.,0.,1.));
#16967=DIRECTION('ref_axis',(-0.707106781186547,-0.707106781186548,0.));
#16968=DIRECTION('',(0.,0.,1.));
#16969=DIRECTION('center_axis',(0.,0.,1.));
#16970=DIRECTION('ref_axis',(0.707106781186547,0.707106781186548,0.));
#16971=DIRECTION('center_axis',(0.,0.,-1.));
#16972=DIRECTION('ref_axis',(0.707106781186547,0.707106781186548,0.));
#16973=DIRECTION('',(0.,0.,1.));
#16974=DIRECTION('',(0.,0.,-1.));
#16975=DIRECTION('center_axis',(-1.,0.,0.));
#16976=DIRECTION('ref_axis',(0.,-1.,0.));
#16977=DIRECTION('',(0.,1.,0.));
#16978=DIRECTION('',(0.,0.,-1.));
#16979=DIRECTION('center_axis',(0.,0.,1.));
#16980=DIRECTION('ref_axis',(0.707106781186548,-0.707106781186547,0.));
#16981=DIRECTION('center_axis',(0.,0.,-1.));
#16982=DIRECTION('ref_axis',(0.707106781186548,-0.707106781186547,0.));
#16983=DIRECTION('',(0.,0.,1.));
#16984=DIRECTION('center_axis',(0.,1.,0.));
#16985=DIRECTION('ref_axis',(-1.,0.,0.));
#16986=DIRECTION('',(1.,0.,0.));
#16987=DIRECTION('',(0.,0.,-1.));
#16988=DIRECTION('center_axis',(0.,0.,1.));
#16989=DIRECTION('ref_axis',(-0.707106781186548,-0.707106781186548,0.));
#16990=DIRECTION('center_axis',(0.,0.,-1.));
#16991=DIRECTION('ref_axis',(-0.707106781186548,-0.707106781186548,0.));
#16992=DIRECTION('',(0.,0.,1.));
#16993=DIRECTION('center_axis',(1.,0.,0.));
#16994=DIRECTION('ref_axis',(0.,1.,0.));
#16995=DIRECTION('',(0.,-1.,0.));
#16996=DIRECTION('',(0.,0.,-1.));
#16997=DIRECTION('center_axis',(0.,0.,1.));
#16998=DIRECTION('ref_axis',(-0.707106781186548,0.707106781186548,0.));
#16999=DIRECTION('center_axis',(0.,0.,-1.));
#17000=DIRECTION('ref_axis',(-0.707106781186548,0.707106781186548,0.));
#17001=DIRECTION('',(0.,0.,1.));
#17002=DIRECTION('center_axis',(0.,-1.,0.));
#17003=DIRECTION('ref_axis',(1.,0.,0.));
#17004=DIRECTION('',(-1.,0.,0.));
#17005=DIRECTION('',(0.,0.,-1.));
#17006=DIRECTION('center_axis',(0.,0.,1.));
#17007=DIRECTION('ref_axis',(0.707106781186547,-0.707106781186548,0.));
#17008=DIRECTION('center_axis',(0.,0.,1.));
#17009=DIRECTION('ref_axis',(0.707106781186547,-0.707106781186548,0.));
#17010=DIRECTION('',(0.,0.,1.));
#17011=DIRECTION('center_axis',(0.,0.,1.));
#17012=DIRECTION('ref_axis',(0.707106781186547,0.707106781186548,0.));
#17013=DIRECTION('',(0.,0.,-1.));
#17014=DIRECTION('center_axis',(0.,0.,1.));
#17015=DIRECTION('ref_axis',(0.707106781186547,0.707106781186548,0.));
#17016=DIRECTION('',(0.,0.,1.));
#17017=DIRECTION('center_axis',(0.,1.,0.));
#17018=DIRECTION('ref_axis',(-1.,0.,0.));
#17019=DIRECTION('',(1.,0.,0.));
#17020=DIRECTION('',(0.,0.,-1.));
#17021=DIRECTION('center_axis',(0.,0.,1.));
#17022=DIRECTION('ref_axis',(-0.707106781186548,0.707106781186548,0.));
#17023=DIRECTION('center_axis',(0.,0.,1.));
#17024=DIRECTION('ref_axis',(-0.707106781186548,0.707106781186548,0.));
#17025=DIRECTION('',(0.,0.,1.));
#17026=DIRECTION('center_axis',(0.,0.,1.));
#17027=DIRECTION('ref_axis',(-0.707106781186548,-0.707106781186547,0.));
#17028=DIRECTION('',(0.,0.,-1.));
#17029=DIRECTION('center_axis',(0.,0.,1.));
#17030=DIRECTION('ref_axis',(-0.707106781186548,-0.707106781186547,0.));
#17031=DIRECTION('center_axis',(0.,0.,1.));
#17032=DIRECTION('ref_axis',(1.,0.,0.));
#17033=DIRECTION('',(0.,0.,-1.));
#17034=DIRECTION('center_axis',(0.,0.,-1.));
#17035=DIRECTION('ref_axis',(1.,0.,0.));
#17036=DIRECTION('center_axis',(0.,0.,1.));
#17037=DIRECTION('ref_axis',(1.,0.,0.));
#17038=DIRECTION('',(0.,0.,-1.));
#17039=DIRECTION('center_axis',(0.,0.,-1.));
#17040=DIRECTION('ref_axis',(1.,0.,0.));
#17041=DIRECTION('center_axis',(0.,0.,1.));
#17042=DIRECTION('ref_axis',(1.,0.,0.));
#17043=DIRECTION('',(0.,0.,-1.));
#17044=DIRECTION('center_axis',(0.,0.,1.));
#17045=DIRECTION('ref_axis',(1.,0.,0.));
#17046=DIRECTION('',(0.,0.,-1.));
#17047=DIRECTION('center_axis',(0.,0.,-1.));
#17048=DIRECTION('ref_axis',(1.,0.,0.));
#17049=DIRECTION('center_axis',(0.,0.,1.));
#17050=DIRECTION('ref_axis',(1.,0.,0.));
#17051=DIRECTION('',(0.,0.,-1.));
#17052=DIRECTION('center_axis',(0.,0.,-1.));
#17053=DIRECTION('ref_axis',(1.,0.,0.));
#17054=DIRECTION('center_axis',(-1.,0.,0.));
#17055=DIRECTION('ref_axis',(0.,-1.,0.));
#17056=DIRECTION('',(0.,1.,0.));
#17057=DIRECTION('center_axis',(1.,0.,0.));
#17058=DIRECTION('ref_axis',(0.,1.,0.));
#17059=DIRECTION('',(0.,-1.,0.));
#17060=DIRECTION('center_axis',(0.,-1.,0.));
#17061=DIRECTION('ref_axis',(1.,0.,0.));
#17062=DIRECTION('',(-1.,0.,0.));
#17063=DIRECTION('center_axis',(0.,1.,0.));
#17064=DIRECTION('ref_axis',(-1.,0.,0.));
#17065=DIRECTION('',(1.,0.,0.));
#17066=DIRECTION('center_axis',(0.,-1.,0.));
#17067=DIRECTION('ref_axis',(1.,0.,0.));
#17068=DIRECTION('',(-1.,0.,0.));
#17069=DIRECTION('center_axis',(-1.,0.,0.));
#17070=DIRECTION('ref_axis',(0.,-1.,0.));
#17071=DIRECTION('',(0.,1.,0.));
#17072=DIRECTION('center_axis',(1.,0.,0.));
#17073=DIRECTION('ref_axis',(0.,1.,0.));
#17074=DIRECTION('',(0.,-1.,0.));
#17075=DIRECTION('center_axis',(-1.,0.,0.));
#17076=DIRECTION('ref_axis',(0.,-1.,0.));
#17077=DIRECTION('',(0.,1.,0.));
#17078=DIRECTION('center_axis',(0.,1.,0.));
#17079=DIRECTION('ref_axis',(-1.,0.,0.));
#17080=DIRECTION('',(1.,0.,0.));
#17081=DIRECTION('center_axis',(0.,-1.,0.));
#17082=DIRECTION('ref_axis',(1.,0.,0.));
#17083=DIRECTION('',(-1.,0.,0.));
#17084=DIRECTION('center_axis',(0.,1.,0.));
#17085=DIRECTION('ref_axis',(-1.,0.,0.));
#17086=DIRECTION('',(1.,0.,0.));
#17087=DIRECTION('center_axis',(1.,0.,0.));
#17088=DIRECTION('ref_axis',(0.,1.,0.));
#17089=DIRECTION('',(0.,-1.,0.));
#17090=DIRECTION('center_axis',(0.,0.,1.));
#17091=DIRECTION('ref_axis',(1.,0.,0.));
#28040=CARTESIAN_POINT('',(0.,0.,0.));
#28041=CARTESIAN_POINT('Origin',(0.,0.,387.));
#28042=CARTESIAN_POINT('',(-4.51811257745934,-3.71096681342671E-5,375.387416697508));
#28043=CARTESIAN_POINT('',(-4.51738402494857,7.56118822245166E-5,375.112583302492));
#28044=CARTESIAN_POINT('',(-4.51775,5.53264807684796E-16,387.));
#28045=CARTESIAN_POINT('',(-3.43378788736318,2.93584158412846,375.));
#28046=CARTESIAN_POINT('Ctrl Pts',(-4.51738402494857,7.56118822245166E-5,
375.112583302492));
#28047=CARTESIAN_POINT('Ctrl Pts',(-4.51750331650906,0.316697913039608,
375.101431493481));
#28048=CARTESIAN_POINT('Ctrl Pts',(-4.4846735281982,0.633280120229468,375.09027968447));
#28049=CARTESIAN_POINT('Ctrl Pts',(-4.41862189351514,0.942742403897512,
375.07912787546));
#28050=CARTESIAN_POINT('Ctrl Pts',(-4.26239834514751,1.67467426709133,375.052751916973));
#28051=CARTESIAN_POINT('Ctrl Pts',(-3.92033033613571,2.36677696691102,375.026375958487));
#28052=CARTESIAN_POINT('Ctrl Pts',(-3.43378788736318,2.93584158412846,375.));
#28053=CARTESIAN_POINT('',(-4.51775,5.53264807684796E-16,375.));
#28054=CARTESIAN_POINT('Origin',(0.,0.,375.));
#28055=CARTESIAN_POINT('',(-4.51775,-5.53264807684796E-16,374.));
#28056=CARTESIAN_POINT('',(-4.51775,5.53264807684796E-16,387.));
#28057=CARTESIAN_POINT('Origin',(0.,0.,374.));
#28058=CARTESIAN_POINT('',(3.43408816985915,2.93604417002329,375.));
#28059=CARTESIAN_POINT('Origin',(0.,0.,375.));
#28060=CARTESIAN_POINT('Ctrl Pts',(3.43408816985915,2.93604417002329,375.));
#28061=CARTESIAN_POINT('Ctrl Pts',(2.97450239048794,3.47304931219374,375.024906410057));
#28062=CARTESIAN_POINT('Ctrl Pts',(2.38685944123298,3.90077491345638,375.049812820113));
#28063=CARTESIAN_POINT('Ctrl Pts',(1.73419289985632,4.17206490566361,375.07471923017));
#28064=CARTESIAN_POINT('Ctrl Pts',(1.04301719200363,4.45936177245515,375.101095188656));
#28065=CARTESIAN_POINT('Ctrl Pts',(0.278918372660684,4.57121814160633,375.127471147143));
#28066=CARTESIAN_POINT('Ctrl Pts',(-0.465602633695269,4.49408396451439,
375.153847105629));
#28067=CARTESIAN_POINT('Ctrl Pts',(-1.21012364005122,4.41694978742245,375.180223064116));
#28068=CARTESIAN_POINT('Ctrl Pts',(-1.93506683342019,4.15082506408738,375.206599022603));
#28069=CARTESIAN_POINT('Ctrl Pts',(-2.55266299064051,3.7279323762134,375.232974981089));
#28070=CARTESIAN_POINT('Ctrl Pts',(-3.17025914786083,3.30503968833942,375.259350939576));
#28071=CARTESIAN_POINT('Ctrl Pts',(-3.68050826893252,2.72537903592653,375.285726898063));
#28072=CARTESIAN_POINT('Ctrl Pts',(-4.02163754569994,2.05912619262106,375.312102856549));
#28073=CARTESIAN_POINT('Ctrl Pts',(-4.346324085653,1.4249873333691,375.337207470202));
#28074=CARTESIAN_POINT('Ctrl Pts',(-4.51780131678173,0.712402743689628,
375.362312083855));
#28075=CARTESIAN_POINT('Ctrl Pts',(-4.51811257745934,-3.71096681342671E-5,
375.387416697508));
#28076=CARTESIAN_POINT('Origin',(0.,0.,387.));
#28077=CARTESIAN_POINT('',(-4.51742232703027,-5.89235854892012E-5,376.387416697508));
#28078=CARTESIAN_POINT('',(-4.51809885152616,4.59828434581654E-5,376.112583302492));
#28079=CARTESIAN_POINT('',(-4.51775,5.53264807684796E-16,387.));
#28080=CARTESIAN_POINT('Ctrl Pts',(-4.51809885152616,4.59828434581654E-5,
376.112583302492));
#28081=CARTESIAN_POINT('Ctrl Pts',(-4.51812276106344,0.0453867389231147,
376.110985620474));
#28082=CARTESIAN_POINT('Ctrl Pts',(-4.51745435602182,0.090726788718723,
376.109387938455));
#28083=CARTESIAN_POINT('Ctrl Pts',(-4.51608913278767,0.136045847103087,
376.107790256437));
#28084=CARTESIAN_POINT('Ctrl Pts',(-4.49355081105947,0.884213247670103,
376.08141429795));
#28085=CARTESIAN_POINT('Ctrl Pts',(-4.28109923000243,1.62665957583979,376.055038339464));
#28086=CARTESIAN_POINT('Ctrl Pts',(-3.90445518421615,2.27349934356334,376.028662380977));
#28087=CARTESIAN_POINT('Ctrl Pts',(-3.52781113842983,2.92033911128693,376.002286422491));
#28088=CARTESIAN_POINT('Ctrl Pts',(-2.98697462791424,3.47157231856439,375.975910464004));
#28089=CARTESIAN_POINT('Ctrl Pts',(-2.3474228959368,3.86046307951571,375.949534505517));
#28090=CARTESIAN_POINT('Ctrl Pts',(-1.70787116395944,4.24935384046699,375.923158547031));
#28091=CARTESIAN_POINT('Ctrl Pts',(-0.969604210520236,4.47590215509218,
375.896782588544));
#28092=CARTESIAN_POINT('Ctrl Pts',(-0.222001520476049,4.51268047531198,
375.870406630058));
#28093=CARTESIAN_POINT('Ctrl Pts',(0.525601169568224,4.54945879553177,375.844030671571));
#28094=CARTESIAN_POINT('Ctrl Pts',(1.28253959621751,4.39646712134613,375.817654713084));
#28095=CARTESIAN_POINT('Ctrl Pts',(1.95717379585807,4.07222787085974,375.791278754598));
#28096=CARTESIAN_POINT('Ctrl Pts',(2.63180799549863,3.74798862037335,375.764902796111));
#28097=CARTESIAN_POINT('Ctrl Pts',(3.2241379681305,3.25250179358621,375.738526837624));
#28098=CARTESIAN_POINT('Ctrl Pts',(3.66245231025333,2.64575380780901,375.712150879138));
#28099=CARTESIAN_POINT('Ctrl Pts',(4.10076665237614,2.03900582203184,375.685774920651));
#28100=CARTESIAN_POINT('Ctrl Pts',(4.38506536398996,1.3209966772646,375.659398962165));
#28101=CARTESIAN_POINT('Ctrl Pts',(4.48092940302618,0.578654357786939,375.633023003678));
#28102=CARTESIAN_POINT('Ctrl Pts',(4.57679344206242,-0.163687961690764,
375.606647045192));
#28103=CARTESIAN_POINT('Ctrl Pts',(4.48422280852107,-0.930363455878798,
375.580271086705));
#28104=CARTESIAN_POINT('Ctrl Pts',(4.21442463026058,-1.62855553605874,375.553895128218));
#28105=CARTESIAN_POINT('Ctrl Pts',(3.9446264520001,-2.32674761623864,375.527519169732));
#28106=CARTESIAN_POINT('Ctrl Pts',(3.49760072902049,-2.95645628241037,375.501143211245));
#28107=CARTESIAN_POINT('Ctrl Pts',(2.92746753425598,-3.44144014717816,375.474767252759));
#28108=CARTESIAN_POINT('Ctrl Pts',(2.35733433949146,-3.92642401194595,375.448391294272));
#28109=CARTESIAN_POINT('Ctrl Pts',(1.66409367294202,-4.26668307530983,375.422015335785));
#28110=CARTESIAN_POINT('Ctrl Pts',(0.931673460847324,-4.42103326145621,
375.395639377299));
#28111=CARTESIAN_POINT('Ctrl Pts',(0.199253248752631,-4.57538344760259,
375.369263418812));
#28112=CARTESIAN_POINT('Ctrl Pts',(-0.572346508887337,-4.54382475653147,
375.342887460326));
#28113=CARTESIAN_POINT('Ctrl Pts',(-1.28970997066769,-4.33015694226547,
375.316511501839));
#28114=CARTESIAN_POINT('Ctrl Pts',(-2.00707343244804,-4.11648912799948,
375.290135543353));
#28115=CARTESIAN_POINT('Ctrl Pts',(-2.67020059836879,-3.72071219053859,
375.263759584866));
#28116=CARTESIAN_POINT('Ctrl Pts',(-3.19881015683584,-3.19078643170059,
375.237383626379));
#28117=CARTESIAN_POINT('Ctrl Pts',(-3.72741971530293,-2.66086067286256,
375.211007667893));
#28118=CARTESIAN_POINT('Ctrl Pts',(-4.12151166631632,-1.99678609264739,
375.184631709406));
#28119=CARTESIAN_POINT('Ctrl Pts',(-4.33336809796127,-1.27886828925581,
375.158255750919));
#28120=CARTESIAN_POINT('Ctrl Pts',(-4.45565119847602,-0.864487596482785,
375.143031601444));
#28121=CARTESIAN_POINT('Ctrl Pts',(-4.51722117132128,-0.432168630785926,
375.127807451968));
#28122=CARTESIAN_POINT('Ctrl Pts',(-4.51738402494857,7.56118822245166E-5,
375.112583302492));
#28123=CARTESIAN_POINT('Ctrl Pts',(-4.51811257745934,-3.71096681342671E-5,
375.387416697508));
#28124=CARTESIAN_POINT('Ctrl Pts',(-4.51812834028524,-0.0361164032740072,
375.388688042342));
#28125=CARTESIAN_POINT('Ctrl Pts',(-4.51770513086054,-0.072195325689107,
375.389959387175));
#28126=CARTESIAN_POINT('Ctrl Pts',(-4.51684061704284,-0.108263669884894,
375.391230732009));
#28127=CARTESIAN_POINT('Ctrl Pts',(-4.49890497915514,-0.856555654887204,
375.417606690495));
#28128=CARTESIAN_POINT('Ctrl Pts',(-4.29102427091659,-1.60029459069377,
375.443982648982));
#28129=CARTESIAN_POINT('Ctrl Pts',(-3.91836620190419,-2.24943891961304,
375.470358607469));
#28130=CARTESIAN_POINT('Ctrl Pts',(-3.54570813289175,-2.89858324853235,
375.496734565955));
#28131=CARTESIAN_POINT('Ctrl Pts',(-3.00827270310544,-3.45313297056435,
375.523110524442));
#28132=CARTESIAN_POINT('Ctrl Pts',(-2.37112526060116,-3.84595044058964,
375.549486482929));
#28133=CARTESIAN_POINT('Ctrl Pts',(-1.73397781809692,-4.2387679106149,375.575862441415));
#28134=CARTESIAN_POINT('Ctrl Pts',(-0.997118362874728,-4.46985312863346,
375.602238399902));
#28135=CARTESIAN_POINT('Ctrl Pts',(-0.249756040595646,-4.5112294783827,
375.628614358388));
#28136=CARTESIAN_POINT('Ctrl Pts',(0.497606281683436,-4.55260582813195,
375.654990316875));
#28137=CARTESIAN_POINT('Ctrl Pts',(1.25547147101941,-4.40427330961188,375.681366275361));
#28138=CARTESIAN_POINT('Ctrl Pts',(1.93208738599618,-4.08418999671804,375.707742233848));
#28139=CARTESIAN_POINT('Ctrl Pts',(2.60870330097296,-3.76410668382419,375.734118192335));
#28140=CARTESIAN_POINT('Ctrl Pts',(3.20406994159053,-3.27227257655657,375.760494150821));
#28141=CARTESIAN_POINT('Ctrl Pts',(3.64610826956487,-2.66823238495421,375.786870109308));
#28142=CARTESIAN_POINT('Ctrl Pts',(4.0881465975392,-2.06419219335185,375.813246067794));
#28143=CARTESIAN_POINT('Ctrl Pts',(4.37685661287028,-1.34794591741475,375.839622026281));
#28144=CARTESIAN_POINT('Ctrl Pts',(4.47728517843054,-0.606207059497561,
375.865997984767));
#28145=CARTESIAN_POINT('Ctrl Pts',(4.57771374399081,0.135531798419669,375.892373943254));
#28146=CARTESIAN_POINT('Ctrl Pts',(4.48986085978024,0.902763238316989,375.918749901741));
#28147=CARTESIAN_POINT('Ctrl Pts',(4.22436257375966,1.6026011428634,375.945125860228));
#28148=CARTESIAN_POINT('Ctrl Pts',(3.95886428773907,2.30243904740981,375.971501818714));
#28149=CARTESIAN_POINT('Ctrl Pts',(3.51572059990846,2.93488341660531,375.9978777772));
#28150=CARTESIAN_POINT('Ctrl Pts',(2.9485814178138,3.42336635395337,376.024253735687));
#28151=CARTESIAN_POINT('Ctrl Pts',(2.38144223571922,3.91184929130138,376.050629694174));
#28152=CARTESIAN_POINT('Ctrl Pts',(1.69030755936062,4.25637079680199,376.07700565266));
#28153=CARTESIAN_POINT('Ctrl Pts',(0.958850723376994,4.41522081720076,376.103381611147));
#28154=CARTESIAN_POINT('Ctrl Pts',(0.227393887393287,4.57407083759954,376.129757569634));
#28155=CARTESIAN_POINT('Ctrl Pts',(-0.544385108215453,4.54724937289643,
376.15613352812));
#28156=CARTESIAN_POINT('Ctrl Pts',(-1.26304959302181,4.33800360748393,376.182509486607));
#28157=CARTESIAN_POINT('Ctrl Pts',(-1.98171407782812,4.12875784207144,376.208885445093));
#28158=CARTESIAN_POINT('Ctrl Pts',(-2.64726405183205,3.73708777594958,376.23526140358));
#28159=CARTESIAN_POINT('Ctrl Pts',(-3.17912363311765,3.21041157777291,376.261637362067));
#28160=CARTESIAN_POINT('Ctrl Pts',(-3.71098321440328,2.68373537959622,376.288013320553));
#28161=CARTESIAN_POINT('Ctrl Pts',(-4.10915240297055,2.0220530493647,376.31438927904));
#28162=CARTESIAN_POINT('Ctrl Pts',(-4.32542620311525,1.30547222672582,376.340765237526));
#28163=CARTESIAN_POINT('Ctrl Pts',(-4.45293485255022,0.882997322948535,
376.356315724187));
#28164=CARTESIAN_POINT('Ctrl Pts',(-4.51721787315074,0.44144006785591,376.371866210847));
#28165=CARTESIAN_POINT('Ctrl Pts',(-4.51742232703027,-5.89235854892012E-5,
376.387416697508));
#28166=CARTESIAN_POINT('Origin',(0.,0.,387.));
#28167=CARTESIAN_POINT('',(-4.51776278108284,0.000115059314115817,377.387416697508));
#28168=CARTESIAN_POINT('',(-4.51759690135649,-0.00010734614409786,377.112583302492));
#28169=CARTESIAN_POINT('',(-4.51775,5.53264807684796E-16,387.));
#28170=CARTESIAN_POINT('Ctrl Pts',(-4.51759690135649,-0.00010734614409786,
377.112583302492));
#28171=CARTESIAN_POINT('Ctrl Pts',(-4.51713109747156,0.522789201244633,
377.094163788979));
#28172=CARTESIAN_POINT('Ctrl Pts',(-4.42639959069602,1.04584321668838,377.075744275467));
#28173=CARTESIAN_POINT('Ctrl Pts',(-4.24853722021895,1.53736821094173,377.057324761954));
#28174=CARTESIAN_POINT('Ctrl Pts',(-3.99384588448772,2.24121105862155,377.030948803468));
#28175=CARTESIAN_POINT('Ctrl Pts',(-3.56049254147675,2.88040358637871,377.004572844981));
#28176=CARTESIAN_POINT('Ctrl Pts',(-3.00094181327236,3.37756091891157,376.978196886494));
#28177=CARTESIAN_POINT('Ctrl Pts',(-2.44139108506791,3.87471825144449,376.951820928008));
#28178=CARTESIAN_POINT('Ctrl Pts',(-1.75564297167002,4.22984038875309,376.925444969521));
#28179=CARTESIAN_POINT('Ctrl Pts',(-1.02671867551292,4.39993389597404,376.899069011035));
#28180=CARTESIAN_POINT('Ctrl Pts',(-0.297794379355856,4.57002740319499,
376.872693052548));
#28181=CARTESIAN_POINT('Ctrl Pts',(0.474306099560417,4.55509228032832,376.846317094061));
#28182=CARTESIAN_POINT('Ctrl Pts',(1.19610717026038,4.35693667212173,376.819941135575));
#28183=CARTESIAN_POINT('Ctrl Pts',(1.91790824096034,4.15878106391514,376.793565177088));
#28184=CARTESIAN_POINT('Ctrl Pts',(2.58940990344398,3.77740497036863,376.767189218602));
#28185=CARTESIAN_POINT('Ctrl Pts',(3.12931572485767,3.25898030397792,376.740813260115));
#28186=CARTESIAN_POINT('Ctrl Pts',(3.66922154627136,2.74055563758721,376.714437301628));
#28187=CARTESIAN_POINT('Ctrl Pts',(4.07753152661508,2.0850823983523,376.688061343142));
#28188=CARTESIAN_POINT('Ctrl Pts',(4.30481295893208,1.37191651212926,376.661685384655));
#28189=CARTESIAN_POINT('Ctrl Pts',(4.53209439124908,0.658750625906209,376.635309426169));
#28190=CARTESIAN_POINT('Ctrl Pts',(4.57834727553935,-0.112107907304984,
376.608933467682));
#28191=CARTESIAN_POINT('Ctrl Pts',(4.4379719316997,-0.847333854561028,376.582557509196));
#28192=CARTESIAN_POINT('Ctrl Pts',(4.29759658786004,-1.58255980181707,376.556181550709));
#28193=CARTESIAN_POINT('Ctrl Pts',(3.97059301589046,-2.28215316311797,376.529805592222));
#28194=CARTESIAN_POINT('Ctrl Pts',(3.49655043114217,-2.86141653901512,376.503429633736));
#28195=CARTESIAN_POINT('Ctrl Pts',(3.02250784639385,-3.4406799149123,376.477053675249));
#28196=CARTESIAN_POINT('Ctrl Pts',(2.40142624886681,-3.89961330540572,376.450677716762));
#28197=CARTESIAN_POINT('Ctrl Pts',(1.7084978848751,-4.18265519808121,376.424301758276));
#28198=CARTESIAN_POINT('Ctrl Pts',(1.01556952088344,-4.46569709075668,376.397925799789));
#28199=CARTESIAN_POINT('Ctrl Pts',(0.250794390427128,-4.57284748561423,
376.371549841303));
#28200=CARTESIAN_POINT('Ctrl Pts',(-0.493238770703864,-4.4911340483472,
376.345173882816));
#28201=CARTESIAN_POINT('Ctrl Pts',(-1.2372719318349,-4.40942061108017,376.31879792433));
#28202=CARTESIAN_POINT('Ctrl Pts',(-1.96056312364061,-4.13884334168854,
376.292421965843));
#28203=CARTESIAN_POINT('Ctrl Pts',(-2.5755459301882,-3.71216011150867,376.266046007356));
#28204=CARTESIAN_POINT('Ctrl Pts',(-3.19052873673575,-3.28547688132881,
376.23967004887));
#28205=CARTESIAN_POINT('Ctrl Pts',(-3.69720315802519,-2.70268769036073,
376.213294090383));
#28206=CARTESIAN_POINT('Ctrl Pts',(-4.03422783747023,-2.03434885839451,
376.186918131897));
#28207=CARTESIAN_POINT('Ctrl Pts',(-4.350837779367,-1.40649359537751,376.162139855428));
#28208=CARTESIAN_POINT('Ctrl Pts',(-4.51772804111577,-0.703138866533066,
376.13736157896));
#28209=CARTESIAN_POINT('Ctrl Pts',(-4.51809885152616,4.59828434581654E-5,
376.112583302492));
#28210=CARTESIAN_POINT('Ctrl Pts',(-4.51742232703027,-5.89235854892012E-5,
376.387416697508));
#28211=CARTESIAN_POINT('Ctrl Pts',(-4.51756465760558,-0.307408461731671,
376.398242169334));
#28212=CARTESIAN_POINT('Ctrl Pts',(-4.48665292107515,-0.614729763863418,
376.40906764116));
#28213=CARTESIAN_POINT('Ctrl Pts',(-4.42439936040209,-0.915565329693696,
376.419893112986));
#28214=CARTESIAN_POINT('Ctrl Pts',(-4.27272030582208,-1.64854274842831,
376.446269071473));
#28215=CARTESIAN_POINT('Ctrl Pts',(-3.9349837849399,-2.34301827085134,376.472645029959));
#28216=CARTESIAN_POINT('Ctrl Pts',(-3.45207841488762,-2.91491409664169,
376.499020988446));
#28217=CARTESIAN_POINT('Ctrl Pts',(-2.96917304483534,-3.48680992243204,
376.525396946932));
#28218=CARTESIAN_POINT('Ctrl Pts',(-2.34109882561295,-3.93612605158971,
376.551772905419));
#28219=CARTESIAN_POINT('Ctrl Pts',(-1.64389457655484,-4.20846530156397,
376.578148863906));
#28220=CARTESIAN_POINT('Ctrl Pts',(-0.946690327496738,-4.48080455153823,
376.604524822392));
#28221=CARTESIAN_POINT('Ctrl Pts',(-0.180356048602913,-4.57616692232909,
376.630900780879));
#28222=CARTESIAN_POINT('Ctrl Pts',(0.562330763470305,-4.48300721455655,
376.657276739365));
#28223=CARTESIAN_POINT('Ctrl Pts',(1.30501757554357,-4.38984750678402,376.683652697852));
#28224=CARTESIAN_POINT('Ctrl Pts',(2.02405692079622,-4.10816572044807,376.710028656339));
#28225=CARTESIAN_POINT('Ctrl Pts',(2.6323971400614,-3.67206411576684,376.736404614825));
#28226=CARTESIAN_POINT('Ctrl Pts',(3.24073735932655,-3.23596251108564,376.762780573312));
#28227=CARTESIAN_POINT('Ctrl Pts',(3.73837845260424,-2.64544108805917,376.789156531798));
#28228=CARTESIAN_POINT('Ctrl Pts',(4.0650726975356,-1.97199227611499,376.815532490285));
#28229=CARTESIAN_POINT('Ctrl Pts',(4.39176694246694,-1.29854346417084,376.841908448771));
#28230=CARTESIAN_POINT('Ctrl Pts',(4.54751433905197,-0.542167263308996,
376.868284407258));
#28231=CARTESIAN_POINT('Ctrl Pts',(4.51345907728089,0.205564420603285,376.894660365745));
#28232=CARTESIAN_POINT('Ctrl Pts',(4.4794038155098,0.953296104515694,376.921036324231));
#28233=CARTESIAN_POINT('Ctrl Pts',(4.25554589538254,1.69238327147853,376.947412282718));
#28234=CARTESIAN_POINT('Ctrl Pts',(3.86898703740037,2.33334714042606,376.973788241204));
#28235=CARTESIAN_POINT('Ctrl Pts',(3.48242817941824,2.97431100937351,377.000164199691));
#28236=CARTESIAN_POINT('Ctrl Pts',(2.93316838358124,3.51715158030568,377.026540158178));
#28237=CARTESIAN_POINT('Ctrl Pts',(2.28770467380867,3.89614898312949,377.052916116664));
#28238=CARTESIAN_POINT('Ctrl Pts',(1.6422409640361,4.27514638595329,377.079292075151));
#28239=CARTESIAN_POINT('Ctrl Pts',(0.900573340327957,4.49030062066872,377.105668033637));
#28240=CARTESIAN_POINT('Ctrl Pts',(0.152492990912077,4.51556369250058,377.132043992124));
#28241=CARTESIAN_POINT('Ctrl Pts',(-0.595587358503804,4.54082676433243,
377.158419950611));
#28242=CARTESIAN_POINT('Ctrl Pts',(-1.35008043362742,4.3761986732807,377.184795909097));
#28243=CARTESIAN_POINT('Ctrl Pts',(-2.01964231224972,4.04161038496754,377.211171867584));
#28244=CARTESIAN_POINT('Ctrl Pts',(-2.68920419087202,3.70702209665437,377.23754782607));
#28245=CARTESIAN_POINT('Ctrl Pts',(-3.27383487299299,3.20247361107977,377.263923784557));
#28246=CARTESIAN_POINT('Ctrl Pts',(-3.70275510124179,2.58904890520336,377.290299743043));
#28247=CARTESIAN_POINT('Ctrl Pts',(-4.13167532949061,1.97562419932691,377.31667570153));
#28248=CARTESIAN_POINT('Ctrl Pts',(-4.40488510386723,1.25332327314864,377.343051660017));
#28249=CARTESIAN_POINT('Ctrl Pts',(-4.48930784196123,0.509592654393879,
377.369427618503));
#28250=CARTESIAN_POINT('Ctrl Pts',(-4.50850066492699,0.340511546362542,
377.375423978172));
#28251=CARTESIAN_POINT('Ctrl Pts',(-4.51793615737842,0.170322859138234,
377.38142033784));
#28252=CARTESIAN_POINT('Ctrl Pts',(-4.51776278108284,0.000115059314115817,
377.387416697508));
#28253=CARTESIAN_POINT('Origin',(0.,0.,387.));
#28254=CARTESIAN_POINT('',(-4.51797310231548,-9.04168125550817E-5,378.387416697508));
#28255=CARTESIAN_POINT('',(-4.51753028950122,9.61292306860575E-5,378.112583302492));
#28256=CARTESIAN_POINT('',(-4.51775,5.53264807684796E-16,387.));
#28257=CARTESIAN_POINT('Ctrl Pts',(-4.51753028950122,9.61292306860575E-5,
378.112583302492));
#28258=CARTESIAN_POINT('Ctrl Pts',(-4.51772668562278,0.251779003793691,
378.103717915972));
#28259=CARTESIAN_POINT('Ctrl Pts',(-4.49704602585537,0.503429942291254,
378.094852529451));
#28260=CARTESIAN_POINT('Ctrl Pts',(-4.4551993669653,0.751510564258943,378.085987142931));
#28261=CARTESIAN_POINT('Ctrl Pts',(-4.33069878989798,1.48959053081815,378.059611184445));
#28262=CARTESIAN_POINT('Ctrl Pts',(-4.01884552637064,2.19606752935734,378.033235225958));
#28263=CARTESIAN_POINT('Ctrl Pts',(-3.55739459519457,2.78541078149727,378.006859267472));
#28264=CARTESIAN_POINT('Ctrl Pts',(-3.09594366401851,3.3747540336372,377.980483308985));
#28265=CARTESIAN_POINT('Ctrl Pts',(-2.48489506519372,3.84696353937788,377.954107350499));
#28266=CARTESIAN_POINT('Ctrl Pts',(-1.79822638382644,4.14487049256201,377.927731392012));
#28267=CARTESIAN_POINT('Ctrl Pts',(-1.11155770245912,4.44277744574616,377.901355433525));
#28268=CARTESIAN_POINT('Ctrl Pts',(-0.349268938549303,4.56638184637374,
377.874979475039));
#28269=CARTESIAN_POINT('Ctrl Pts',(0.396352188045507,4.50071932813326,377.848603516552));
#28270=CARTESIAN_POINT('Ctrl Pts',(1.14197331464023,4.43505680989279,377.822227558065));
#28271=CARTESIAN_POINT('Ctrl Pts',(1.87092680391995,4.18012737278432,377.795851599579));
#28272=CARTESIAN_POINT('Ctrl Pts',(2.49496072486742,3.76679446067473,377.769475641092));
#28273=CARTESIAN_POINT('Ctrl Pts',(3.11899464581496,3.35346154856509,377.743099682606));
#28274=CARTESIAN_POINT('Ctrl Pts',(3.63810899843023,2.7817251614543,377.716723724119));
#28275=CARTESIAN_POINT('Ctrl Pts',(3.98945636554489,2.120803488071,377.690347765632));
#28276=CARTESIAN_POINT('Ctrl Pts',(4.34080373265956,1.45988181468769,377.663971807146));
#28277=CARTESIAN_POINT('Ctrl Pts',(4.52438411427362,0.709774855031875,377.637595848659));
#28278=CARTESIAN_POINT('Ctrl Pts',(4.517972055111,-0.0387044808375217,377.611219890173));
#28279=CARTESIAN_POINT('Ctrl Pts',(4.51155999594838,-0.787183816706875,
377.584843931686));
#28280=CARTESIAN_POINT('Ctrl Pts',(4.3151554960091,-1.53403552878981,377.558467973199));
#28281=CARTESIAN_POINT('Ctrl Pts',(3.9525365831578,-2.18884080883012,377.532092014713));
#28282=CARTESIAN_POINT('Ctrl Pts',(3.5899176703065,-2.84364608887043,377.505716056226));
#28283=CARTESIAN_POINT('Ctrl Pts',(3.06108434454318,-3.40640493686811,377.47934009774));
#28284=CARTESIAN_POINT('Ctrl Pts',(2.43006066621085,-3.80898604436084,377.452964139253));
#28285=CARTESIAN_POINT('Ctrl Pts',(1.79903698787851,-4.21156715185356,377.426588180766));
#28286=CARTESIAN_POINT('Ctrl Pts',(1.06582295697716,-4.45397051884133,377.40021222228));
#28287=CARTESIAN_POINT('Ctrl Pts',(0.319186313873781,-4.50684919035867,
377.373836263793));
#28288=CARTESIAN_POINT('Ctrl Pts',(-0.427450329229602,-4.55972786187601,
377.347460305307));
#28289=CARTESIAN_POINT('Ctrl Pts',(-1.18750958453502,-4.42308183792293,
377.32108434682));
#28290=CARTESIAN_POINT('Ctrl Pts',(-1.86897365124353,-4.11345438999364,
377.294708388334));
#28291=CARTESIAN_POINT('Ctrl Pts',(-2.55043771795204,-3.80382694206434,
377.268332429847));
#28292=CARTESIAN_POINT('Ctrl Pts',(-3.15330659606364,-3.32121807015883,
377.24195647136));
#28293=CARTESIAN_POINT('Ctrl Pts',(-3.60459299156575,-2.72405559648777,
377.215580512874));
#28294=CARTESIAN_POINT('Ctrl Pts',(-4.05587938706785,-2.1268931228167,377.189204554387));
#28295=CARTESIAN_POINT('Ctrl Pts',(-4.35558329996046,-1.41517704738009,
377.162828595901));
#28296=CARTESIAN_POINT('Ctrl Pts',(-4.46742059218106,-0.675072425860511,
377.136452637414));
#28297=CARTESIAN_POINT('Ctrl Pts',(-4.50115689268563,-0.451816019874252,
377.12849619244));
#28298=CARTESIAN_POINT('Ctrl Pts',(-4.51779810878667,-0.225976373769842,
377.120539747466));
#28299=CARTESIAN_POINT('Ctrl Pts',(-4.51759690135649,-0.00010734614409786,
377.112583302492));
#28300=CARTESIAN_POINT('Ctrl Pts',(-4.51776278108284,0.000115059314115817,
377.387416697508));
#28301=CARTESIAN_POINT('Ctrl Pts',(-4.51717353368206,-0.578363695817441,
377.407796296326));
#28302=CARTESIAN_POINT('Ctrl Pts',(-4.40559318176197,-1.15706321872293,
377.428175895145));
#28303=CARTESIAN_POINT('Ctrl Pts',(-4.18884997964351,-1.69325291121775,
377.448555493963));
#28304=CARTESIAN_POINT('Ctrl Pts',(-3.90833367742039,-2.38720754674346,
377.47493145245));
#28305=CARTESIAN_POINT('Ctrl Pts',(-3.45166537116277,-3.0099565064637,377.501307410936));
#28306=CARTESIAN_POINT('Ctrl Pts',(-2.87413234662247,-3.48610568219112,
377.527683369423));
#28307=CARTESIAN_POINT('Ctrl Pts',(-2.29659932208215,-3.96225485791856,
377.55405932791));
#28308=CARTESIAN_POINT('Ctrl Pts',(-1.59820157925914,-4.29180424965317,
377.580435286396));
#28309=CARTESIAN_POINT('Ctrl Pts',(-0.863491768396101,-4.43485642825323,
377.606811244883));
#28310=CARTESIAN_POINT('Ctrl Pts',(-0.128781957533104,-4.57790860685328,
377.633187203369));
#28311=CARTESIAN_POINT('Ctrl Pts',(0.642239921369918,-4.5344635723188,377.659563161856));
#28312=CARTESIAN_POINT('Ctrl Pts',(1.35622885978989,-4.30978106789426,377.685939120342));
#28313=CARTESIAN_POINT('Ctrl Pts',(2.07021779820986,-4.08509856346973,377.712315078829));
#28314=CARTESIAN_POINT('Ctrl Pts',(2.72717379614679,-3.67917858915515,377.738691037316));
#28315=CARTESIAN_POINT('Ctrl Pts',(3.24756141510707,-3.14116450196653,377.765066995802));
#28316=CARTESIAN_POINT('Ctrl Pts',(3.76794903406735,-2.6031504147779,377.791442954289));
#28317=CARTESIAN_POINT('Ctrl Pts',(4.15176827405098,-1.93304221471522,377.817818912776));
#28318=CARTESIAN_POINT('Ctrl Pts',(4.35255143912362,-1.21196763285564,377.844194871262));
#28319=CARTESIAN_POINT('Ctrl Pts',(4.55333460419626,-0.49089305099606,377.870570829749));
#28320=CARTESIAN_POINT('Ctrl Pts',(4.57108169435792,0.28114791266043,377.896946788235));
#28321=CARTESIAN_POINT('Ctrl Pts',(4.40364412948689,1.01068687244984,377.923322746722));
#28322=CARTESIAN_POINT('Ctrl Pts',(4.23620656461585,1.7402258322393,377.949698705208));
#28323=CARTESIAN_POINT('Ctrl Pts',(3.88358434471212,2.42726278816168,377.976074663695));
#28324=CARTESIAN_POINT('Ctrl Pts',(3.38846824810894,2.98862050198153,378.002450622182));
#28325=CARTESIAN_POINT('Ctrl Pts',(2.89335215150579,3.54997821580136,378.028826580668));
#28326=CARTESIAN_POINT('Ctrl Pts',(2.25574217820322,3.98565668751868,378.055202539155));
#28327=CARTESIAN_POINT('Ctrl Pts',(1.55283160898984,4.2429097995867,378.081578497641));
#28328=CARTESIAN_POINT('Ctrl Pts',(0.849921039776497,4.5001629116547,378.107954456128));
#28329=CARTESIAN_POINT('Ctrl Pts',(0.0817098746523573,4.57899066407343,
378.134330414615));
#28330=CARTESIAN_POINT('Ctrl Pts',(-0.658797161460833,4.46984964773514,
378.160706373101));
#28331=CARTESIAN_POINT('Ctrl Pts',(-1.39930419757415,4.36070863139684,378.187082331588));
#28332=CARTESIAN_POINT('Ctrl Pts',(-2.11210710467651,4.06359884630146,378.213458290074));
#28333=CARTESIAN_POINT('Ctrl Pts',(-2.71090924805577,3.61449036824177,378.239834248561));
#28334=CARTESIAN_POINT('Ctrl Pts',(-3.309711391435,3.16538189018211,378.266210207048));
#28335=CARTESIAN_POINT('Ctrl Pts',(-3.79451277109115,2.56427471915816,378.292586165534));
#28336=CARTESIAN_POINT('Ctrl Pts',(-4.10662012532275,1.8839428652698,378.318962124021));
#28337=CARTESIAN_POINT('Ctrl Pts',(-4.37662833282249,1.29537876422316,378.341780315183));
#28338=CARTESIAN_POINT('Ctrl Pts',(-4.5173887163544,0.647521251956349,378.364598506346));
#28339=CARTESIAN_POINT('Ctrl Pts',(-4.51797310231548,-9.04168125550817E-5,
378.387416697508));
#28340=CARTESIAN_POINT('Origin',(0.,0.,387.));
#28341=CARTESIAN_POINT('',(-4.51737365644452,-1.98811769755447E-6,379.387416697508));
#28342=CARTESIAN_POINT('',(-4.51813007169143,-2.03714566067892E-5,379.112583302492));
#28343=CARTESIAN_POINT('',(-4.51775,5.53264807684796E-16,387.));
#28344=CARTESIAN_POINT('Ctrl Pts',(-4.51813007169143,-2.03714566067892E-5,
379.112583302492));
#28345=CARTESIAN_POINT('Ctrl Pts',(-4.517945231463,0.728944748987095,379.086896084477));
#28346=CARTESIAN_POINT('Ctrl Pts',(-4.33810981632971,1.45799779441603,379.061208866463));
#28347=CARTESIAN_POINT('Ctrl Pts',(-3.99878265125311,2.10316590777759,379.035521648449));
#28348=CARTESIAN_POINT('Ctrl Pts',(-3.65035725094643,2.76563263988363,379.009145689962));
#28349=CARTESIAN_POINT('Ctrl Pts',(-3.13377267064052,3.33965579170571,378.982769731476));
#28350=CARTESIAN_POINT('Ctrl Pts',(-2.51157005653494,3.75574032365363,378.956393772989));
#28351=CARTESIAN_POINT('Ctrl Pts',(-1.88936744242933,4.17182485560157,378.930017814502));
#28352=CARTESIAN_POINT('Ctrl Pts',(-1.16154679452404,4.42997076767533,378.903641856016));
#28353=CARTESIAN_POINT('Ctrl Pts',(-0.416222894566461,4.49892520827358,
378.877265897529));
#28354=CARTESIAN_POINT('Ctrl Pts',(0.329101005391076,4.56787964887184,378.850889939042));
#28355=CARTESIAN_POINT('Ctrl Pts',(1.0919281574009,4.44764261799461,378.824513980556));
#28356=CARTESIAN_POINT('Ctrl Pts',(1.779905660781,4.15277080589822,378.798138022069));
#28357=CARTESIAN_POINT('Ctrl Pts',(2.46788316416111,3.85789899380182,378.771762063583));
#28358=CARTESIAN_POINT('Ctrl Pts',(3.08101101891148,3.38839240048625,378.745386105096));
#28359=CARTESIAN_POINT('Ctrl Pts',(3.54505991145048,2.80109259965241,378.71901014661));
#28360=CARTESIAN_POINT('Ctrl Pts',(4.00910880398948,2.21379279881858,378.692634188123));
#28361=CARTESIAN_POINT('Ctrl Pts',(4.3240787343171,1.50869979046648,378.666258229636));
#28362=CARTESIAN_POINT('Ctrl Pts',(4.45183735932425,0.771176797969019,378.63988227115));
#28363=CARTESIAN_POINT('Ctrl Pts',(4.57959598433139,0.0336538054715552,
378.613506312663));
#28364=CARTESIAN_POINT('Ctrl Pts',(4.52014330401807,-0.736299171171277,
378.587130354177));
#28365=CARTESIAN_POINT('Ctrl Pts',(4.28067705310806,-1.44546653181419,378.56075439569));
#28366=CARTESIAN_POINT('Ctrl Pts',(4.04121080219804,-2.1546338924571,378.534378437203));
#28367=CARTESIAN_POINT('Ctrl Pts',(3.62173098069132,-2.80301563710009,378.508002478717));
#28368=CARTESIAN_POINT('Ctrl Pts',(3.07302259039553,-3.31211438306704,378.48162652023));
#28369=CARTESIAN_POINT('Ctrl Pts',(2.5243142000997,-3.82121312903403,378.455250561744));
#28370=CARTESIAN_POINT('Ctrl Pts',(1.84637724101477,-4.19102887632496,378.428874603257));
#28371=CARTESIAN_POINT('Ctrl Pts',(1.12128724556784,-4.37678928445587,378.40249864477));
#28372=CARTESIAN_POINT('Ctrl Pts',(0.396197250120947,-4.56254969258676,
378.376122686284));
#28373=CARTESIAN_POINT('Ctrl Pts',(-0.37604578168795,-4.56425476155764,
378.349746727797));
#28374=CARTESIAN_POINT('Ctrl Pts',(-1.10194900048777,-4.38169806444086,
378.323370769311));
#28375=CARTESIAN_POINT('Ctrl Pts',(-1.82785221928764,-4.19914136732407,
378.296994810824));
#28376=CARTESIAN_POINT('Ctrl Pts',(-2.50741562507842,-3.83232290411959,
378.270618852338));
#28377=CARTESIAN_POINT('Ctrl Pts',(-3.05836677703682,-3.32565214427459,
378.244242893851));
#28378=CARTESIAN_POINT('Ctrl Pts',(-3.60931792899519,-2.81898138442963,
378.217866935364));
#28379=CARTESIAN_POINT('Ctrl Pts',(-4.0316568271212,-2.17245832794416,378.191490976878));
#28380=CARTESIAN_POINT('Ctrl Pts',(-4.27425233088056,-1.46435533241182,
378.165115018391));
#28381=CARTESIAN_POINT('Ctrl Pts',(-4.435307559621,-0.99425721373283,378.147604446425));
#28382=CARTESIAN_POINT('Ctrl Pts',(-4.51714237540265,-0.497018246743604,
378.130093874458));
#28383=CARTESIAN_POINT('Ctrl Pts',(-4.51753028950122,9.61292306860575E-5,
378.112583302492));
#28384=CARTESIAN_POINT('Ctrl Pts',(-4.51797310231548,-9.04168125550817E-5,
378.387416697508));
#28385=CARTESIAN_POINT('Ctrl Pts',(-4.51806421862098,-0.101064749856769,
378.390974464832));
#28386=CARTESIAN_POINT('Ctrl Pts',(-4.51474759603089,-0.202033106339626,
378.394532232156));
#28387=CARTESIAN_POINT('Ctrl Pts',(-4.50798181202017,-0.302769806622464,
378.398089999481));
#28388=CARTESIAN_POINT('Ctrl Pts',(-4.45782281567894,-1.04959408787382,
378.424465957967));
#28389=CARTESIAN_POINT('Ctrl Pts',(-4.2180914941894,-1.78368611362381,378.450841916454));
#28390=CARTESIAN_POINT('Ctrl Pts',(-3.81781130701489,-2.41617184764166,
378.47721787494));
#28391=CARTESIAN_POINT('Ctrl Pts',(-3.41753111984037,-3.04865758165951,
378.503593833427));
#28392=CARTESIAN_POINT('Ctrl Pts',(-2.85670206698089,-3.57953702394521,
378.529969791913));
#28393=CARTESIAN_POINT('Ctrl Pts',(-2.20322182313489,-3.94453839775569,
378.5563457504));
#28394=CARTESIAN_POINT('Ctrl Pts',(-1.54974157928885,-4.30953977156619,
378.582721708887));
#28395=CARTESIAN_POINT('Ctrl Pts',(-0.803610144456304,-4.50866307690144,
378.609097667373));
#28396=CARTESIAN_POINT('Ctrl Pts',(-0.0551591253652737,-4.51780112933225,
378.63547362586));
#28397=CARTESIAN_POINT('Ctrl Pts',(0.693291893725671,-4.52693918176306,
378.661849584346));
#28398=CARTESIAN_POINT('Ctrl Pts',(1.44406249707508,-4.34609198128947,378.688225542833));
#28399=CARTESIAN_POINT('Ctrl Pts',(2.10625942952888,-3.99715408620027,378.71460150132));
#28400=CARTESIAN_POINT('Ctrl Pts',(2.76845636198275,-3.64821619111103,378.740977459806));
#28401=CARTESIAN_POINT('Ctrl Pts',(3.34207962354098,-3.13118760140616,378.767353418293));
#28402=CARTESIAN_POINT('Ctrl Pts',(3.75768258797375,-2.50866321799992,378.793729376779));
#28403=CARTESIAN_POINT('Ctrl Pts',(4.1732855524065,-1.88613883459371,378.820105335266));
#28404=CARTESIAN_POINT('Ctrl Pts',(4.43086821971381,-1.15811865748618,378.846481293753));
#28405=CARTESIAN_POINT('Ctrl Pts',(4.49924592843132,-0.412741624749648,
378.872857252239));
#28406=CARTESIAN_POINT('Ctrl Pts',(4.56762363714884,0.332635407986881,378.899233210726));
#28407=CARTESIAN_POINT('Ctrl Pts',(4.44679638727653,1.09536929635249,378.925609169213));
#28408=CARTESIAN_POINT('Ctrl Pts',(4.15139232488624,1.78311843077862,378.951985127699));
#28409=CARTESIAN_POINT('Ctrl Pts',(3.85598826249595,2.47086756520474,378.978361086186));
#28410=CARTESIAN_POINT('Ctrl Pts',(3.38600738758769,3.08363194569147,379.004737044672));
#28411=CARTESIAN_POINT('Ctrl Pts',(2.79834869352904,3.54722626325572,379.031113003159));
#28412=CARTESIAN_POINT('Ctrl Pts',(2.2106899994704,4.01082058081996,379.057488961645));
#28413=CARTESIAN_POINT('Ctrl Pts',(1.5053534862614,4.32524483546169,379.083864920132));
#28414=CARTESIAN_POINT('Ctrl Pts',(0.767731857583539,4.4524327471797,379.110240878618));
#28415=CARTESIAN_POINT('Ctrl Pts',(0.030110228905678,4.5796206588977,379.136616837105));
#28416=CARTESIAN_POINT('Ctrl Pts',(-0.739796515241018,4.51957222769198,
379.162992795591));
#28417=CARTESIAN_POINT('Ctrl Pts',(-1.44877837192307,4.27955731382987,379.189368754078));
#28418=CARTESIAN_POINT('Ctrl Pts',(-2.15776022860516,4.03954239996775,379.215744712565));
#28419=CARTESIAN_POINT('Ctrl Pts',(-2.80581719782259,3.61956100344924,379.242120671052));
#28420=CARTESIAN_POINT('Ctrl Pts',(-3.31449121636045,3.0704588500705,379.268496629538));
#28421=CARTESIAN_POINT('Ctrl Pts',(-3.82316523489829,2.52135669669179,379.294872588025));
#28422=CARTESIAN_POINT('Ctrl Pts',(-4.19245630275656,1.84313378645288,379.321248546511));
#28423=CARTESIAN_POINT('Ctrl Pts',(-4.37765560061389,1.11790027091894,379.347624504998));
#28424=CARTESIAN_POINT('Ctrl Pts',(-4.4707894813135,0.753191481541508,379.360888569168));
#28425=CARTESIAN_POINT('Ctrl Pts',(-4.51736785070585,0.376594041376692,
379.374152633338));
#28426=CARTESIAN_POINT('Ctrl Pts',(-4.51737365644452,-1.98811769755447E-6,
379.387416697508));
#28427=CARTESIAN_POINT('Origin',(0.,0.,387.));
#28428=CARTESIAN_POINT('',(-4.51796103056296,9.30366574888874E-5,380.387416697508));
#28429=CARTESIAN_POINT('',(-4.51744861143269,-7.15418913582019E-5,380.112583302492));
#28430=CARTESIAN_POINT('',(-4.51775,5.53264807684796E-16,387.));
#28431=CARTESIAN_POINT('Ctrl Pts',(-4.51744861143269,-7.15418913582019E-5,
380.112583302492));
#28432=CARTESIAN_POINT('Ctrl Pts',(-4.51718913038702,0.45796072853139,380.09645021147));
#28433=CARTESIAN_POINT('Ctrl Pts',(-4.44792028854276,0.916069730534027,
380.080317120448));
#28434=CARTESIAN_POINT('Ctrl Pts',(-4.31082918580142,1.35289366117352,380.064184029426));
#28435=CARTESIAN_POINT('Ctrl Pts',(-4.08669921406521,2.0670562382494,380.037808070939));
#28436=CARTESIAN_POINT('Ctrl Pts',(-3.68128769636301,2.72432612859277,380.011432112453));
#28437=CARTESIAN_POINT('Ctrl Pts',(-3.14367643259018,3.24512989181911,379.985056153966));
#28438=CARTESIAN_POINT('Ctrl Pts',(-2.60606516881736,3.76593365504543,379.958680195479));
#28439=CARTESIAN_POINT('Ctrl Pts',(-1.93625415897387,4.15027129115475,379.932304236993));
#28440=CARTESIAN_POINT('Ctrl Pts',(-1.21533515432327,4.35161234374879,379.905928278506));
#28441=CARTESIAN_POINT('Ctrl Pts',(-0.494416149672638,4.55295339634284,
379.87955232002));
#28442=CARTESIAN_POINT('Ctrl Pts',(0.27761084978516,4.57129786542164,379.853176361533));
#28443=CARTESIAN_POINT('Ctrl Pts',(1.0072791489844,4.40442484822049,379.826800403046));
#28444=CARTESIAN_POINT('Ctrl Pts',(1.73694744818368,4.23755183101932,379.80042444456));
#28445=CARTESIAN_POINT('Ctrl Pts',(2.4242570471244,3.88546132753817,379.774048486073));
#28446=CARTESIAN_POINT('Ctrl Pts',(2.98599769960395,3.39077974300318,379.747672527587));
#28447=CARTESIAN_POINT('Ctrl Pts',(3.5477383520835,2.89609815846819,379.7212965691));
#28448=CARTESIAN_POINT('Ctrl Pts',(3.98391005810188,2.25882549287937,379.694920610614));
#28449=CARTESIAN_POINT('Ctrl Pts',(4.24170698590533,1.55611419032241,379.668544652127));
#28450=CARTESIAN_POINT('Ctrl Pts',(4.49950391370875,0.853402887765529,379.64216869364));
#28451=CARTESIAN_POINT('Ctrl Pts',(4.57892606329728,0.0852529482405344,
379.615792735154));
#28452=CARTESIAN_POINT('Ctrl Pts',(4.47035806391024,-0.655338315706838,
379.589416776667));
#28453=CARTESIAN_POINT('Ctrl Pts',(4.36179006452319,-1.39592957965429,379.56304081818));
#28454=CARTESIAN_POINT('Ctrl Pts',(4.06523191616051,-2.10896216802411,379.536664859694));
#28455=CARTESIAN_POINT('Ctrl Pts',(3.61658690982335,-2.70811163937072,379.510288901207));
#28456=CARTESIAN_POINT('Ctrl Pts',(3.16794190348622,-3.30726111071731,379.483912942721));
#28457=CARTESIAN_POINT('Ctrl Pts',(2.56721003917463,-3.79252746504069,379.457536984234));
#28458=CARTESIAN_POINT('Ctrl Pts',(1.88711988987541,-4.10516114773068,379.431161025748));
#28459=CARTESIAN_POINT('Ctrl Pts',(1.20702974057619,-4.41779483042066,379.404785067261));
#28460=CARTESIAN_POINT('Ctrl Pts',(0.447581306289357,-4.55779584147724,
379.378409108774));
#28461=CARTESIAN_POINT('Ctrl Pts',(-0.299281562218895,-4.50821473247633,
379.352033150288));
#28462=CARTESIAN_POINT('Ctrl Pts',(-1.04614443072715,-4.45863362347542,
379.325657191801));
#28463=CARTESIAN_POINT('Ctrl Pts',(-1.7804217334568,-4.21947039441701,379.299281233315));
#28464=CARTESIAN_POINT('Ctrl Pts',(-2.41321700332044,-3.81967972773712,
379.272905274828));
#28465=CARTESIAN_POINT('Ctrl Pts',(-3.04601227318407,-3.41988906105724,
379.246529316342));
#28466=CARTESIAN_POINT('Ctrl Pts',(-3.57732551018167,-2.85947095675588,
379.220153357855));
#28467=CARTESIAN_POINT('Ctrl Pts',(-3.94283241951303,-2.20627333738088,
379.193777399368));
#28468=CARTESIAN_POINT('Ctrl Pts',(-4.30833932884442,-1.55307571800585,
379.167401440882));
#28469=CARTESIAN_POINT('Ctrl Pts',(-4.50803991050956,-0.807098583557167,
379.141025482395));
#28470=CARTESIAN_POINT('Ctrl Pts',(-4.51775709118839,-0.0586548601377958,
379.114649523908));
#28471=CARTESIAN_POINT('Ctrl Pts',(-4.51801083042644,-0.0391111728918336,
379.113960783436));
#28472=CARTESIAN_POINT('Ctrl Pts',(-4.51813502773401,-0.0195658037794806,
379.113272042964));
#28473=CARTESIAN_POINT('Ctrl Pts',(-4.51813007169143,-2.03714566067892E-5,
379.112583302492));
#28474=CARTESIAN_POINT('Ctrl Pts',(-4.51737365644452,-1.98811769755447E-6,
379.387416697508));
#28475=CARTESIAN_POINT('Ctrl Pts',(-4.51737939557777,-0.372277579931259,
379.400528591825));
#28476=CARTESIAN_POINT('Ctrl Pts',(-4.47187503399554,-0.744551793256104,
379.413640486141));
#28477=CARTESIAN_POINT('Ctrl Pts',(-4.38084409953505,-1.10533911035289,
379.426752380458));
#28478=CARTESIAN_POINT('Ctrl Pts',(-4.19772577274251,-1.83110085526187,
379.453128338944));
#28479=CARTESIAN_POINT('Ctrl Pts',(-3.83038159130104,-2.51038022425081,
379.479504297431));
#28480=CARTESIAN_POINT('Ctrl Pts',(-3.32328467158491,-3.06093916387039,
379.505880255917));
#28481=CARTESIAN_POINT('Ctrl Pts',(-2.81618775186881,-3.61149810348995,
379.532256214404));
#28482=CARTESIAN_POINT('Ctrl Pts',(-2.16933809387807,-4.03333661374015,
379.558632172891));
#28483=CARTESIAN_POINT('Ctrl Pts',(-1.46104759574481,-4.27538413435274,
379.585008131377));
#28484=CARTESIAN_POINT('Ctrl Pts',(-0.752757097611556,-4.51743165496533,
379.611384089864));
#28485=CARTESIAN_POINT('Ctrl Pts',(0.0169742406642152,-4.57968818594031,
379.63776004835));
#28486=CARTESIAN_POINT('Ctrl Pts',(0.75495765194394,-4.45461653984696,379.664136006837));
#28487=CARTESIAN_POINT('Ctrl Pts',(1.49294106322366,-4.32954489375361,379.690511965324));
#28488=CARTESIAN_POINT('Ctrl Pts',(2.19917654750734,-4.01714507059193,379.71688792381));
#28489=CARTESIAN_POINT('Ctrl Pts',(2.78816256572898,-3.55523825929773,379.743263882297));
#28490=CARTESIAN_POINT('Ctrl Pts',(3.37714858395063,-3.09333144800353,379.769639840783));
#28491=CARTESIAN_POINT('Ctrl Pts',(3.84888513611024,-2.48191764857682,379.79601579927));
#28492=CARTESIAN_POINT('Ctrl Pts',(4.14626067493935,-1.79501865972427,379.822391757756));
#28493=CARTESIAN_POINT('Ctrl Pts',(4.44363621376846,-1.10811967087172,379.848767716243));
#28494=CARTESIAN_POINT('Ctrl Pts',(4.56665073926708,-0.34573549259334,379.87514367473));
#28495=CARTESIAN_POINT('Ctrl Pts',(4.50041129930853,0.399834603758797,379.901519633216));
#28496=CARTESIAN_POINT('Ctrl Pts',(4.43417185934997,1.14540470011094,379.927895591703));
#28497=CARTESIAN_POINT('Ctrl Pts',(4.17867845393423,1.87416071453683,379.954271550189));
#28498=CARTESIAN_POINT('Ctrl Pts',(3.76486280466181,2.49787462363122,379.980647508676));
#28499=CARTESIAN_POINT('Ctrl Pts',(3.35104715538937,3.12158853272565,380.007023467163));
#28500=CARTESIAN_POINT('Ctrl Pts',(2.77890926226022,3.64026033648856,380.033399425649));
#28501=CARTESIAN_POINT('Ctrl Pts',(2.11771592297733,3.99109619564288,380.059775384136));
#28502=CARTESIAN_POINT('Ctrl Pts',(1.45652258369447,4.34193205479719,380.086151342622));
#28503=CARTESIAN_POINT('Ctrl Pts',(0.706273798257865,4.52493196934294,380.112527301109));
#28504=CARTESIAN_POINT('Ctrl Pts',(-0.0422003529064303,4.5179407591868,
380.138903259596));
#28505=CARTESIAN_POINT('Ctrl Pts',(-0.790674504070726,4.51094954903066,
380.165279218082));
#28506=CARTESIAN_POINT('Ctrl Pts',(-1.53737402096271,4.31396721417262,380.191655176569));
#28507=CARTESIAN_POINT('Ctrl Pts',(-2.19189852108271,3.95084173899465,380.218031135055));
#28508=CARTESIAN_POINT('Ctrl Pts',(-2.84642302120274,3.58771626381665,380.244407093542));
#28509=CARTESIAN_POINT('Ctrl Pts',(-3.40877250455077,3.05844764831869,380.270783052029));
#28510=CARTESIAN_POINT('Ctrl Pts',(-3.81086522305661,2.42711265189824,380.297159010515));
#28511=CARTESIAN_POINT('Ctrl Pts',(-4.21295794156245,1.7957776554778,380.323534969002));
#28512=CARTESIAN_POINT('Ctrl Pts',(-4.4547938952261,1.06237627813486,380.349910927489));
#28513=CARTESIAN_POINT('Ctrl Pts',(-4.50709482389231,0.315698941635839,
380.376286885975));
#28514=CARTESIAN_POINT('Ctrl Pts',(-4.51445126403015,0.210674283980221,
380.379996823153));
#28515=CARTESIAN_POINT('Ctrl Pts',(-4.51805792159162,0.105386973232761,
380.38370676033));
#28516=CARTESIAN_POINT('Ctrl Pts',(-4.51796103056296,9.30366574888874E-5,
380.387416697508));
#28517=CARTESIAN_POINT('Origin',(0.,0.,387.));
#28518=CARTESIAN_POINT('',(-4.51777632728029,-0.000114640610663838,381.387416697508));
#28519=CARTESIAN_POINT('',(-4.51771140424386,0.000115276608145368,381.112583302492));
#28520=CARTESIAN_POINT('',(-4.51775,5.53264807684796E-16,387.));
#28521=CARTESIAN_POINT('Ctrl Pts',(-4.51771140424386,0.000115276608145367,
381.112583302492));
#28522=CARTESIAN_POINT('Ctrl Pts',(-4.51789787410811,0.186866521003934,
381.106004338462));
#28523=CARTESIAN_POINT('Ctrl Pts',(-4.50653449305084,0.373595224723727,
381.099425374433));
#28524=CARTESIAN_POINT('Ctrl Pts',(-4.48344098370869,0.558861765736475,
381.092846410403));
#28525=CARTESIAN_POINT('Ctrl Pts',(-4.3908559747359,1.30162043908853,381.066470451916));
#28526=CARTESIAN_POINT('Ctrl Pts',(-4.10973064608376,2.02087752596908,381.04009449343));
#28527=CARTESIAN_POINT('Ctrl Pts',(-3.6740998895201,2.62955500597139,381.013718534943));
#28528=CARTESIAN_POINT('Ctrl Pts',(-3.23846913295646,3.23823248597366,380.987342576457));
#28529=CARTESIAN_POINT('Ctrl Pts',(-2.6483329484813,3.73633035909772,380.96096661797));
#28530=CARTESIAN_POINT('Ctrl Pts',(-1.9751371259962,4.06354560219426,380.934590659483));
#28531=CARTESIAN_POINT('Ctrl Pts',(-1.30194130351109,4.3907608452908,380.908214700997));
#28532=CARTESIAN_POINT('Ctrl Pts',(-0.545685843016022,4.54709345835984,
380.88183874251));
#28533=CARTESIAN_POINT('Ctrl Pts',(0.202071967249689,4.51361678121356,380.855462784024));
#28534=CARTESIAN_POINT('Ctrl Pts',(0.949829777515443,4.48014010406728,380.829086825537));
#28535=CARTESIAN_POINT('Ctrl Pts',(1.68908993755185,4.25685413670566,380.802710867051));
#28536=CARTESIAN_POINT('Ctrl Pts',(2.33035272260718,3.87079135524483,380.776334908564));
#28537=CARTESIAN_POINT('Ctrl Pts',(2.97161550766248,3.48472857378402,380.749958950077));
#28538=CARTESIAN_POINT('Ctrl Pts',(3.51488091773671,2.93588897822401,380.723582991591));
#28539=CARTESIAN_POINT('Ctrl Pts',(3.89437764890032,2.29071872025929,380.697207033104));
#28540=CARTESIAN_POINT('Ctrl Pts',(4.27387438006393,1.64554846229457,380.670831074617));
#28541=CARTESIAN_POINT('Ctrl Pts',(4.48960243231693,0.904047541925131,380.644455116131));
#28542=CARTESIAN_POINT('Ctrl Pts',(4.51544434073745,0.155986965169938,380.618079157644));
#28543=CARTESIAN_POINT('Ctrl Pts',(4.54128624915798,-0.592073611585275,
380.591703199158));
#28544=CARTESIAN_POINT('Ctrl Pts',(4.37724201374605,-1.34669384472619,380.565327240671));
#28545=CARTESIAN_POINT('Ctrl Pts',(4.04317191469819,-2.01651441745319,380.538951282185));
#28546=CARTESIAN_POINT('Ctrl Pts',(3.70910181565035,-2.68633499018016,380.512575323698));
#28547=CARTESIAN_POINT('Ctrl Pts',(3.20500585296659,-3.27135590249316,380.486199365211));
#28548=CARTESIAN_POINT('Ctrl Pts',(2.59191321819219,-3.70075065317313,380.459823406725));
#28549=CARTESIAN_POINT('Ctrl Pts',(1.9788205834178,-4.13014540385311,380.433447448238));
#28550=CARTESIAN_POINT('Ctrl Pts',(1.25673127655275,-4.40391399290007,380.407071489751));
#28551=CARTESIAN_POINT('Ctrl Pts',(0.513066205288616,-4.48891218410335,
380.380695531265));
#28552=CARTESIAN_POINT('Ctrl Pts',(-0.230598865975566,-4.57391037530665,
380.354319572778));
#28553=CARTESIAN_POINT('Ctrl Pts',(-0.995839701638859,-4.47013816866624,
380.327943614292));
#28554=CARTESIAN_POINT('Ctrl Pts',(-1.69001118451102,-4.19015891391108,
380.301567655805));
#28555=CARTESIAN_POINT('Ctrl Pts',(-2.38418266738314,-3.91017965915592,
380.275191697319));
#28556=CARTESIAN_POINT('Ctrl Pts',(-3.00728479746414,-3.45399335628602,
380.248815738832));
#28557=CARTESIAN_POINT('Ctrl Pts',(-3.48388070942679,-2.87682893653492,
380.222439780345));
#28558=CARTESIAN_POINT('Ctrl Pts',(-3.96047662138947,-2.2996645167838,380.196063821859));
#28559=CARTESIAN_POINT('Ctrl Pts',(-4.29056631523378,-1.60152198015145,
380.169687863372));
#28560=CARTESIAN_POINT('Ctrl Pts',(-4.43418694927082,-0.866923079931074,
380.143311904886));
#28561=CARTESIAN_POINT('Ctrl Pts',(-4.48996073737275,-0.581648170267025,
380.133069037421));
#28562=CARTESIAN_POINT('Ctrl Pts',(-4.5176133554335,-0.290875321156064,
380.122826169956));
#28563=CARTESIAN_POINT('Ctrl Pts',(-4.51744861143269,-7.15418913582019E-5,
380.112583302492));
#28564=CARTESIAN_POINT('Ctrl Pts',(-4.51796103056296,9.30366574888874E-5,
380.387416697508));
#28565=CARTESIAN_POINT('Ctrl Pts',(-4.5173690706415,-0.643204813367623,
380.410082718817));
#28566=CARTESIAN_POINT('Ctrl Pts',(-4.37853653898567,-1.28674998247137,
380.432748740126));
#28567=CARTESIAN_POINT('Ctrl Pts',(-4.11200700232459,-1.87215597270644,
380.455414761435));
#28568=CARTESIAN_POINT('Ctrl Pts',(-3.80185234842186,-2.55338025489479,
380.481790719921));
#28569=CARTESIAN_POINT('Ctrl Pts',(-3.3187771369476,-3.15587552361643,380.508166678408));
#28570=CARTESIAN_POINT('Ctrl Pts',(-2.72126564826557,-3.60669971648272,
380.534542636895));
#28571=CARTESIAN_POINT('Ctrl Pts',(-2.12375415958355,-4.05752390934902,
380.560918595381));
#28572=CARTESIAN_POINT('Ctrl Pts',(-1.41180639369374,-4.35667702635998,
380.587294553868));
#28573=CARTESIAN_POINT('Ctrl Pts',(-0.671615456256834,-4.46794161244568,
380.613670512354));
#28574=CARTESIAN_POINT('Ctrl Pts',(0.0685754811800957,-4.57920619853139,
380.640046470841));
#28575=CARTESIAN_POINT('Ctrl Pts',(0.837009590164088,-4.50258225369185,
380.666422429328));
#28576=CARTESIAN_POINT('Ctrl Pts',(1.54065515471516,-4.24734637951232,380.692798387814));
#28577=CARTESIAN_POINT('Ctrl Pts',(2.24430071926626,-3.99211050533279,380.719174346301));
#28578=CARTESIAN_POINT('Ctrl Pts',(2.88315773938438,-3.55826270181326,380.745550304787));
#28579=CARTESIAN_POINT('Ctrl Pts',(3.37988195854491,-2.99832745369971,380.771926263274));
#28580=CARTESIAN_POINT('Ctrl Pts',(3.87660617770542,-2.4383922055862,380.79830222176));
#28581=CARTESIAN_POINT('Ctrl Pts',(4.23119759590837,-1.75236951287867,380.824678180247));
#28582=CARTESIAN_POINT('Ctrl Pts',(4.40072703064927,-1.02331382039902,380.851054138734));
#28583=CARTESIAN_POINT('Ctrl Pts',(4.57025646539019,-0.294258127919331,
380.87743009722));
#28584=CARTESIAN_POINT('Ctrl Pts',(4.55472391666906,0.477830564332509,380.903806055707));
#28585=CARTESIAN_POINT('Ctrl Pts',(4.35600985757286,1.19947809235303,380.930182014193));
#28586=CARTESIAN_POINT('Ctrl Pts',(4.15729579847668,1.92112562037352,380.95655797268));
#28587=CARTESIAN_POINT('Ctrl Pts',(3.77540022900545,2.59233198416271,380.982933931167));
#28588=CARTESIAN_POINT('Ctrl Pts',(3.25655795281734,3.131836501679,381.009309889653));
#28589=CARTESIAN_POINT('Ctrl Pts',(2.73771567662922,3.6713410191953,381.03568584814));
#28590=CARTESIAN_POINT('Ctrl Pts',(2.08192669372421,4.07914369043871,381.062061806626));
#28591=CARTESIAN_POINT('Ctrl Pts',(1.36858515603701,4.30587322665008,381.088437765113));
#28592=CARTESIAN_POINT('Ctrl Pts',(0.655243618349795,4.53260276286145,381.1148137236));
#28593=CARTESIAN_POINT('Ctrl Pts',(-0.11565047411956,4.57825916404077,381.141189682086));
#28594=CARTESIAN_POINT('Ctrl Pts',(-0.850767583518968,4.43731496427064,
381.167565640573));
#28595=CARTESIAN_POINT('Ctrl Pts',(-1.58588469291835,4.2963707645005,381.193941599059));
#28596=CARTESIAN_POINT('Ctrl Pts',(-2.28522481924775,3.96882596378091,381.220317557546));
#28597=CARTESIAN_POINT('Ctrl Pts',(-2.8641212210839,3.49433530220608,381.246693516033));
#28598=CARTESIAN_POINT('Ctrl Pts',(-3.44301762292008,3.01984464063123,381.273069474519));
#28599=CARTESIAN_POINT('Ctrl Pts',(-3.90147030026302,2.39840811820112,381.299445433006));
#28600=CARTESIAN_POINT('Ctrl Pts',(-4.18397593959467,1.70526095076376,381.325821391492));
#28601=CARTESIAN_POINT('Ctrl Pts',(-4.40388606866954,1.16569620642928,381.346353160164));
#28602=CARTESIAN_POINT('Ctrl Pts',(-4.51718122901344,0.58267845338523,381.366884928836));
#28603=CARTESIAN_POINT('Ctrl Pts',(-4.51777632728029,-0.000114640610663838,
381.387416697508));
#28604=CARTESIAN_POINT('Origin',(0.,0.,387.));
#28605=CARTESIAN_POINT('',(-4.51741634198117,5.54534861180178E-5,382.387416697508));
#28606=CARTESIAN_POINT('',(-4.51801683772092,-7.91791388051273E-5,382.112583302492));
#28607=CARTESIAN_POINT('',(-4.51775,5.53264807684796E-16,387.));
#28608=CARTESIAN_POINT('Ctrl Pts',(-4.51801683772092,-7.91791388051273E-5,
382.112583302492));
#28609=CARTESIAN_POINT('Ctrl Pts',(-4.51747244268795,0.664048991360067,
382.089182506968));
#28610=CARTESIAN_POINT('Ctrl Pts',(-4.36919765227329,1.32841221793627,382.065781711444));
#28611=CARTESIAN_POINT('Ctrl Pts',(-4.08568376167234,1.92892657382487,382.04238091592));
#28612=CARTESIAN_POINT('Ctrl Pts',(-3.76612408682134,2.60578996102738,382.016004957434));
#28613=CARTESIAN_POINT('Ctrl Pts',(-3.27475081492882,3.20153698377045,381.989628998947));
#28614=CARTESIAN_POINT('Ctrl Pts',(-2.67105284443962,3.64404256695937,381.963253040461));
#28615=CARTESIAN_POINT('Ctrl Pts',(-2.06735487395043,4.08654815014828,381.936877081974));
#28616=CARTESIAN_POINT('Ctrl Pts',(-1.35133220486457,4.37581229378304,381.910501123487));
#28617=CARTESIAN_POINT('Ctrl Pts',(-0.609671277576736,4.47681476732048,
381.884125165001));
#28618=CARTESIAN_POINT('Ctrl Pts',(0.131989649711098,4.57781724085793,381.857749206514));
#28619=CARTESIAN_POINT('Ctrl Pts',(0.899288835200903,4.49055804429805,381.831373248027));
#28620=CARTESIAN_POINT('Ctrl Pts',(1.59933196425767,4.22560135314543,381.804997289541));
#28621=CARTESIAN_POINT('Ctrl Pts',(2.29937509331447,3.9606446619928,381.778621331054));
#28622=CARTESIAN_POINT('Ctrl Pts',(2.93216216593823,3.5179904762474,381.752245372568));
#28623=CARTESIAN_POINT('Ctrl Pts',(3.42108379359719,2.95122943953659,381.725869414081));
#28624=CARTESIAN_POINT('Ctrl Pts',(3.91000542125612,2.38446840282581,381.699493455595));
#28625=CARTESIAN_POINT('Ctrl Pts',(4.25506160395026,1.69360051514964,381.673117497108));
#28626=CARTESIAN_POINT('Ctrl Pts',(4.41447755785592,0.962266812681007,381.646741538621));
#28627=CARTESIAN_POINT('Ctrl Pts',(4.57389351176158,0.23093311021233,381.620365580135));
#28628=CARTESIAN_POINT('Ctrl Pts',(4.54766923687872,-0.540866407048814,
381.593989621648));
#28629=CARTESIAN_POINT('Ctrl Pts',(4.33897961738306,-1.25969258453608,381.567613663161));
#28630=CARTESIAN_POINT('Ctrl Pts',(4.1302899978874,-1.9785187620233,381.541237704675));
#28631=CARTESIAN_POINT('Ctrl Pts',(3.73913503377896,-2.64437159973664,381.514861746188));
#28632=CARTESIAN_POINT('Ctrl Pts',(3.21287053227619,-3.17663854891175,381.488485787702));
#28633=CARTESIAN_POINT('Ctrl Pts',(2.68660603077342,-3.70890549808685,381.462109829215));
#28634=CARTESIAN_POINT('Ctrl Pts',(2.02523199187631,-4.1075865587237,381.435733870728));
#28635=CARTESIAN_POINT('Ctrl Pts',(1.3088187313399,-4.32441476457735,381.409357912242));
#28636=CARTESIAN_POINT('Ctrl Pts',(0.592405470803483,-4.54124297043101,
381.382981953755));
#28637=CARTESIAN_POINT('Ctrl Pts',(-0.179047011372244,-4.57621832150146,
381.356605995269));
#28638=CARTESIAN_POINT('Ctrl Pts',(-0.912141574983824,-4.42510647044643,
381.330230036782));
#28639=CARTESIAN_POINT('Ctrl Pts',(-1.64523613859541,-4.2739946193914,381.303854078296));
#28640=CARTESIAN_POINT('Ctrl Pts',(-2.33997278364284,-3.93679556621089,
381.277478119809));
#28641=CARTESIAN_POINT('Ctrl Pts',(-2.91224209659624,-3.45433285865933,
381.251102161322));
#28642=CARTESIAN_POINT('Ctrl Pts',(-3.48451140954963,-2.97187015110778,
381.224726202836));
#28643=CARTESIAN_POINT('Ctrl Pts',(-3.93431339040899,-2.34414378918517,
381.198350244349));
#28644=CARTESIAN_POINT('Ctrl Pts',(-4.20719203619195,-1.64715047831211,
381.171974285863));
#28645=CARTESIAN_POINT('Ctrl Pts',(-4.4120064713043,-1.1240084389856,381.152177291406));
#28646=CARTESIAN_POINT('Ctrl Pts',(-4.51715029114881,-0.561844529442614,
381.132380296949));
#28647=CARTESIAN_POINT('Ctrl Pts',(-4.51771140424386,0.000115276608145367,
381.112583302492));
#28648=CARTESIAN_POINT('Ctrl Pts',(-4.51777632728029,-0.000114640610663838,
381.387416697508));
#28649=CARTESIAN_POINT('Ctrl Pts',(-4.51794571683875,-0.166001638386794,
381.393260887323));
#28650=CARTESIAN_POINT('Ctrl Pts',(-4.50898407036945,-0.331870434133353,
381.399105077137));
#28651=CARTESIAN_POINT('Ctrl Pts',(-4.49075105445655,-0.496713740704063,
381.404949266952));
#28652=CARTESIAN_POINT('Ctrl Pts',(-4.40846192866641,-1.24068345228999,
381.431325225439));
#28653=CARTESIAN_POINT('Ctrl Pts',(-4.13732507576575,-1.96376506301729,
381.457701183925));
#28654=CARTESIAN_POINT('Ctrl Pts',(-3.71016611657994,-2.57841753032532,
381.484077142412));
#28655=CARTESIAN_POINT('Ctrl Pts',(-3.28300715739413,-3.19306999763336,
381.510453100898));
#28656=CARTESIAN_POINT('Ctrl Pts',(-2.69982609192317,-3.69929332152213,
381.536829059385));
#28657=CARTESIAN_POINT('Ctrl Pts',(-2.03122667735788,-4.03580075802764,
381.563205017872));
#28658=CARTESIAN_POINT('Ctrl Pts',(-1.36262726279259,-4.37230819453315,
381.589580976358));
#28659=CARTESIAN_POINT('Ctrl Pts',(-0.608609499132967,-4.5390997436554,
381.615956934845));
#28660=CARTESIAN_POINT('Ctrl Pts',(0.139540235761641,-4.51598251722816,
381.642332893331));
#28661=CARTESIAN_POINT('Ctrl Pts',(0.887689970656269,-4.49286529080092,
381.668708851818));
#28662=CARTESIAN_POINT('Ctrl Pts',(1.62997167678589,-4.2798392888242,381.695084810305));
#28663=CARTESIAN_POINT('Ctrl Pts',(2.27651982104296,-3.90269484814088,381.721460768791));
#28664=CARTESIAN_POINT('Ctrl Pts',(2.92306796530002,-3.52555040745756,381.747836727278));
#28665=CARTESIAN_POINT('Ctrl Pts',(3.47388254768454,-2.98428752806765,381.774212685764));
#28666=CARTESIAN_POINT('Ctrl Pts',(3.86227831153366,-2.3444350742905,381.800588644251));
#28667=CARTESIAN_POINT('Ctrl Pts',(4.25067407538277,-1.70458262051336,381.826964602737));
#28668=CARTESIAN_POINT('Ctrl Pts',(4.47665102069649,-0.966140592348972,
381.853340561224));
#28669=CARTESIAN_POINT('Ctrl Pts',(4.51285088376856,-0.21850966609316,381.879716519711));
#28670=CARTESIAN_POINT('Ctrl Pts',(4.54905074684063,0.529121260162651,381.906092478197));
#28671=CARTESIAN_POINT('Ctrl Pts',(4.39547352767104,1.28594108450989,381.932468436684));
#28672=CARTESIAN_POINT('Ctrl Pts',(4.07071230023681,1.96032419308837,381.95884439517));
#28673=CARTESIAN_POINT('Ctrl Pts',(3.74595107280257,2.63470730166687,381.985220353657));
#28674=CARTESIAN_POINT('Ctrl Pts',(3.25000583710367,3.2266536944766,382.011596312144));
#28675=CARTESIAN_POINT('Ctrl Pts',(2.64291900376427,3.66449842582154,382.03797227063));
#28676=CARTESIAN_POINT('Ctrl Pts',(2.03583217042486,4.10234315716648,382.064348229117));
#28677=CARTESIAN_POINT('Ctrl Pts',(1.31760373944494,4.38608622704663,382.090724187603));
#28678=CARTESIAN_POINT('Ctrl Pts',(0.575187195343948,4.48137582262626,382.11710014609));
#28679=CARTESIAN_POINT('Ctrl Pts',(-0.167229348757025,4.57666541820589,
382.143476104577));
#28680=CARTESIAN_POINT('Ctrl Pts',(-0.933834005979071,4.48350153948501,
382.169852063063));
#28681=CARTESIAN_POINT('Ctrl Pts',(-1.63181654587318,4.21316322184666,382.19622802155));
#28682=CARTESIAN_POINT('Ctrl Pts',(-2.32979908576728,3.94282490420832,382.222603980037));
#28683=CARTESIAN_POINT('Ctrl Pts',(-2.95915950833345,3.4953121476525,382.248979938523));
#28684=CARTESIAN_POINT('Ctrl Pts',(-3.44370327796121,2.9248038065255,382.27535589701));
#28685=CARTESIAN_POINT('Ctrl Pts',(-3.92824704758899,2.35429546539847,382.301731855496));
#28686=CARTESIAN_POINT('Ctrl Pts',(-4.26797416427836,1.66079153970024,382.328107813983));
#28687=CARTESIAN_POINT('Ctrl Pts',(-4.42175501618481,0.928252201802573,
382.354483772469));
#28688=CARTESIAN_POINT('Ctrl Pts',(-4.48575841876287,0.623370224843185,
382.365461414149));
#28689=CARTESIAN_POINT('Ctrl Pts',(-4.5175519448549,0.311726478256462,382.376439055828));
#28690=CARTESIAN_POINT('Ctrl Pts',(-4.51741634198117,5.54534861180178E-5,
382.387416697508));
#28691=CARTESIAN_POINT('Origin',(0.,0.,387.));
#28692=CARTESIAN_POINT('',(-4.51810647145572,4.12515443024009E-5,383.387416697508));
#28693=CARTESIAN_POINT('',(-4.51737744603353,-1.71510238390164E-5,383.112583302492));
#28694=CARTESIAN_POINT('',(-4.51775,5.53264807684796E-16,387.));
#28695=CARTESIAN_POINT('Ctrl Pts',(-4.51737744603353,-1.71510238390164E-5,
383.112583302492));
#28696=CARTESIAN_POINT('Ctrl Pts',(-4.51732510787532,0.393119355640695,
383.09873663396));
#28697=CARTESIAN_POINT('Ctrl Pts',(-4.46651507043149,0.786269138328428,
383.084889965429));
#28698=CARTESIAN_POINT('Ctrl Pts',(-4.36511527641182,1.16590657912072,383.071043296898));
#28699=CARTESIAN_POINT('Ctrl Pts',(-4.17196291261205,1.8890625754899,383.044667338411));
#28700=CARTESIAN_POINT('Ctrl Pts',(-3.79524613196318,2.56318917681575,383.018291379924));
#28701=CARTESIAN_POINT('Ctrl Pts',(-3.28057275969385,3.10667215778483,382.991915421438));
#28702=CARTESIAN_POINT('Ctrl Pts',(-2.76589938742451,3.65015513875392,382.965539462951));
#28703=CARTESIAN_POINT('Ctrl Pts',(-2.11326942353471,4.06299449936623,382.939163504465));
#28704=CARTESIAN_POINT('Ctrl Pts',(-1.40169456822207,4.29520917593283,382.912787545978));
#28705=CARTESIAN_POINT('Ctrl Pts',(-0.690119712909428,4.52742385249943,
382.886411587491));
#28706=CARTESIAN_POINT('Ctrl Pts',(0.0804000338260355,4.57901384502031,
382.860035629005));
#28707=CARTESIAN_POINT('Ctrl Pts',(0.816580454902776,4.44373332776299,382.833659670518));
#28708=CARTESIAN_POINT('Ctrl Pts',(1.55276087597956,4.30845281050567,382.807283712031));
#28709=CARTESIAN_POINT('Ctrl Pts',(2.2546019713976,3.98630178347012,382.780907753545));
#28710=CARTESIAN_POINT('Ctrl Pts',(2.83713421587333,3.51628198083169,382.754531795058));
#28711=CARTESIAN_POINT('Ctrl Pts',(3.41966646034902,3.04626217819329,382.728155836572));
#28712=CARTESIAN_POINT('Ctrl Pts',(3.88288985388241,2.42837359995203,382.701779878085));
#28713=CARTESIAN_POINT('Ctrl Pts',(4.17072350849794,1.7374219243648,382.675403919598));
#28714=CARTESIAN_POINT('Ctrl Pts',(4.45855716311345,1.04647024877758,382.649027961112));
#28715=CARTESIAN_POINT('Ctrl Pts',(4.57100107881112,0.282455475844346,382.622652002625));
#28716=CARTESIAN_POINT('Ctrl Pts',(4.4944420514052,-0.462125712508384,382.596276044139));
#28717=CARTESIAN_POINT('Ctrl Pts',(4.41788302399928,-1.20670690086118,382.569900085652));
#28718=CARTESIAN_POINT('Ctrl Pts',(4.15232105348975,-1.93185450463351,382.543524127166));
#28719=CARTESIAN_POINT('Ctrl Pts',(3.72990682856509,-2.54977735848138,382.517148168679));
#28720=CARTESIAN_POINT('Ctrl Pts',(3.30749260364046,-3.16770021232922,382.490772210192));
#28721=CARTESIAN_POINT('Ctrl Pts',(2.72822612430073,-3.6783983162526,382.464396251706));
#28722=CARTESIAN_POINT('Ctrl Pts',(2.06223722204694,-4.02004317981846,382.438020293219));
#28723=CARTESIAN_POINT('Ctrl Pts',(1.39624831979316,-4.36168804338432,382.411644334732));
#28724=CARTESIAN_POINT('Ctrl Pts',(0.643536994625335,-4.53427966659265,
382.385268376246));
#28725=CARTESIAN_POINT('Ctrl Pts',(-0.104768541682353,-4.51692296594424,
382.358892417759));
#28726=CARTESIAN_POINT('Ctrl Pts',(-0.853074077990042,-4.49956626529584,
382.332516459273));
#28727=CARTESIAN_POINT('Ctrl Pts',(-1.59697382543758,-4.29226124079071,
382.306140500786));
#28728=CARTESIAN_POINT('Ctrl Pts',(-2.2464063601331,-3.92010560989808,382.2797645423));
#28729=CARTESIAN_POINT('Ctrl Pts',(-2.89583889482865,-3.54794997900543,
382.253388583813));
#28730=CARTESIAN_POINT('Ctrl Pts',(-3.45080421677215,-3.01094374172526,
382.227012625326));
#28731=CARTESIAN_POINT('Ctrl Pts',(-3.84411455331502,-2.37410042512789,
382.20063666684));
#28732=CARTESIAN_POINT('Ctrl Pts',(-4.23742488985787,-1.73725710853056,
382.174260708353));
#28733=CARTESIAN_POINT('Ctrl Pts',(-4.46908024100009,-1.00057671261605,
382.147884749867));
#28734=CARTESIAN_POINT('Ctrl Pts',(-4.51103487766645,-0.253246638827817,
382.12150879138));
#28735=CARTESIAN_POINT('Ctrl Pts',(-4.51576728885779,-0.168949085903131,
382.118533628417));
#28736=CARTESIAN_POINT('Ctrl Pts',(-4.51808605177553,-0.0845160322941951,
382.115558465455));
#28737=CARTESIAN_POINT('Ctrl Pts',(-4.51801683772092,-7.91791388051273E-5,
382.112583302492));
#28738=CARTESIAN_POINT('Ctrl Pts',(-4.51741634198117,5.54534861180178E-5,
382.387416697508));
#28739=CARTESIAN_POINT('Ctrl Pts',(-4.51722613209177,-0.43712489171991,
382.402815014315));
#28740=CARTESIAN_POINT('Ctrl Pts',(-4.45421338524669,-0.874358908440133,
382.418213331122));
#28741=CARTESIAN_POINT('Ctrl Pts',(-4.32915293519383,-1.29306010572185,
382.433611647929));
#28742=CARTESIAN_POINT('Ctrl Pts',(-4.11493541517289,-2.01025832525158,
382.459987606416));
#28743=CARTESIAN_POINT('Ctrl Pts',(-3.71866578800746,-2.67308001421398,
382.486363564902));
#28744=CARTESIAN_POINT('Ctrl Pts',(-3.1883190758562,-3.2012795947618,382.512739523389));
#28745=CARTESIAN_POINT('Ctrl Pts',(-2.65797236370492,-3.72947917530964,
382.539115481875));
#28746=CARTESIAN_POINT('Ctrl Pts',(-1.99354856656775,-4.1230566474429,382.565491440362));
#28747=CARTESIAN_POINT('Ctrl Pts',(-1.27548722410474,-4.33436291909808,
382.591867398849));
#28748=CARTESIAN_POINT('Ctrl Pts',(-0.557425881641732,-4.54566919075325,
382.618243357335));
#28749=CARTESIAN_POINT('Ctrl Pts',(0.214273006147169,-4.57470426193039,
382.644619315822));
#28750=CARTESIAN_POINT('Ctrl Pts',(0.94618246756513,-4.4179529548626,382.670995274309));
#28751=CARTESIAN_POINT('Ctrl Pts',(1.67809192898305,-4.26120164779482,382.697371232795));
#28752=CARTESIAN_POINT('Ctrl Pts',(2.37021196402998,-3.91866396248217,382.723747191282));
#28753=CARTESIAN_POINT('Ctrl Pts',(2.93874994329017,-3.4318097767969,382.750123149768));
#28754=CARTESIAN_POINT('Ctrl Pts',(3.50728792255042,-2.94495559111159,382.776499108255));
#28755=CARTESIAN_POINT('Ctrl Pts',(3.95224384602383,-2.31378490505366,382.802875066742));
#28756=CARTESIAN_POINT('Ctrl Pts',(4.21974840648906,-1.61471141670574,382.829251025228));
#28757=CARTESIAN_POINT('Ctrl Pts',(4.48725296695428,-0.91563792835784,382.855626983715));
#28758=CARTESIAN_POINT('Ctrl Pts',(4.57730616441131,-0.148661637719957,
382.882002942201));
#28759=CARTESIAN_POINT('Ctrl Pts',(4.47900556312629,0.593362232359432,382.908378900688));
#28760=CARTESIAN_POINT('Ctrl Pts',(4.38070496184126,1.33538610243882,382.934754859174));
#28761=CARTESIAN_POINT('Ctrl Pts',(4.09405056181417,2.05245755195971,382.961130817661));
#28762=CARTESIAN_POINT('Ctrl Pts',(3.6537466407651,2.65776316823087,382.987506776148));
#28763=CARTESIAN_POINT('Ctrl Pts',(3.21344271971605,3.26306878450199,383.013882734634));
#28764=CARTESIAN_POINT('Ctrl Pts',(2.61948927764498,3.75660856752342,383.040258693121));
#28765=CARTESIAN_POINT('Ctrl Pts',(1.94379424690704,4.07863132668275,383.066634651607));
#28766=CARTESIAN_POINT('Ctrl Pts',(1.26809921616909,4.4006540858421,383.093010610094));
#28767=CARTESIAN_POINT('Ctrl Pts',(0.510662596764224,4.55115982113938,383.119386568581));
#28768=CARTESIAN_POINT('Ctrl Pts',(-0.236815324157952,4.51192731275126,
383.145762527067));
#28769=CARTESIAN_POINT('Ctrl Pts',(-0.984293245080149,4.47269480436314,
383.172138485554));
#28770=CARTESIAN_POINT('Ctrl Pts',(-1.72181246751965,4.24372405228961,383.19851444404));
#28771=CARTESIAN_POINT('Ctrl Pts',(-2.36008403614551,3.85273577028557,383.224890402527));
#28772=CARTESIAN_POINT('Ctrl Pts',(-2.99835560477138,3.46174748828153,383.251266361013));
#28773=CARTESIAN_POINT('Ctrl Pts',(-3.53737951958361,2.90874167634699,383.2776423195));
#28774=CARTESIAN_POINT('Ctrl Pts',(-3.91189798012409,2.26066887588782,383.304018277987));
#28775=CARTESIAN_POINT('Ctrl Pts',(-4.28641644066456,1.61259607542868,383.330394236473));
#28776=CARTESIAN_POINT('Ctrl Pts',(-4.49642944693329,0.869456286444925,
383.35677019496));
#28777=CARTESIAN_POINT('Ctrl Pts',(-4.51651143527701,0.121218927230134,
383.383146153446));
#28778=CARTESIAN_POINT('Ctrl Pts',(-4.5175952633915,0.0808364375906089,
383.384569668134));
#28779=CARTESIAN_POINT('Ctrl Pts',(-4.51812586459283,0.0404390998600549,
383.385993182821));
#28780=CARTESIAN_POINT('Ctrl Pts',(-4.51810647145572,4.12515443024009E-5,
383.387416697508));
#28781=CARTESIAN_POINT('Origin',(0.,0.,387.));
#28782=CARTESIAN_POINT('',(-4.51758348284472,-0.000105543616906456,384.387416697508));
#28783=CARTESIAN_POINT('',(-4.51791286673421,0.000101789655423226,384.112583302492));
#28784=CARTESIAN_POINT('',(-4.51775,5.53264807684796E-16,387.));
#28785=CARTESIAN_POINT('Ctrl Pts',(-4.51791286673421,0.000101789655423226,
384.112583302492));
#28786=CARTESIAN_POINT('Ctrl Pts',(-4.51803160945122,0.121934720290465,
384.108290760953));
#28787=CARTESIAN_POINT('Ctrl Pts',(-4.51320179205148,0.243758262585871,
384.103998219414));
#28788=CARTESIAN_POINT('Ctrl Pts',(-4.50335615873677,0.365175074681226,
384.099705677874));
#28789=CARTESIAN_POINT('Ctrl Pts',(-4.4428586625063,1.11123303735971,384.073329719388));
#28790=CARTESIAN_POINT('Ctrl Pts',(-4.19298336184317,1.84193444118764,384.046953760901));
#28791=CARTESIAN_POINT('Ctrl Pts',(-3.78398181342604,2.46881574105112,384.020577802415));
#28792=CARTESIAN_POINT('Ctrl Pts',(-3.37498026500888,3.09569704091462,383.994201843928));
#28793=CARTESIAN_POINT('Ctrl Pts',(-2.80685246883769,3.61875823681367,383.967825885442));
#28794=CARTESIAN_POINT('Ctrl Pts',(-2.14837973375322,3.97467408062589,383.941449926955));
#28795=CARTESIAN_POINT('Ctrl Pts',(-1.48990699866878,4.33058992443809,383.915073968468));
#28796=CARTESIAN_POINT('Ctrl Pts',(-0.741089324671071,4.5193604161635,383.888698009982));
#28797=CARTESIAN_POINT('Ctrl Pts',(0.00741646763062709,4.51813175146638,
383.862322051495));
#28798=CARTESIAN_POINT('Ctrl Pts',(0.755922259932325,4.51690308676927,383.835946093009));
#28799=CARTESIAN_POINT('Ctrl Pts',(1.50411617053801,4.32567526564963,383.809570134522));
#28800=CARTESIAN_POINT('Ctrl Pts',(2.16141689576047,3.96759959299347,383.783194176035));
#28801=CARTESIAN_POINT('Ctrl Pts',(2.81871762098293,3.60952392033731,383.756818217549));
#28802=CARTESIAN_POINT('Ctrl Pts',(3.38512516082216,3.08460039614464,383.730442259062));
#28803=CARTESIAN_POINT('Ctrl Pts',(3.79206647204748,2.45637973431923,383.704066300576));
#28804=CARTESIAN_POINT('Ctrl Pts',(4.19900778327279,1.82815907249382,383.677690342089));
#28805=CARTESIAN_POINT('Ctrl Pts',(4.44648286588418,1.09664127303568,383.651314383602));
#28806=CARTESIAN_POINT('Ctrl Pts',(4.50453074947641,0.35038871931369,383.624938425116));
#28807=CARTESIAN_POINT('Ctrl Pts',(4.56257863306864,-0.395863834408303,
383.598562466629));
#28808=CARTESIAN_POINT('Ctrl Pts',(4.4311993176417,-1.15685114239415,383.572186508143));
#28809=CARTESIAN_POINT('Ctrl Pts',(4.12629845211925,-1.84044304764888,383.545810549656));
#28810=CARTESIAN_POINT('Ctrl Pts',(3.8213975865968,-2.52403495290361,383.519434591169));
#28811=CARTESIAN_POINT('Ctrl Pts',(3.34297517097883,-3.13023145542722,383.493058632683));
#28812=CARTESIAN_POINT('Ctrl Pts',(2.74895218738718,-3.58564239698551,383.466682674196));
#28813=CARTESIAN_POINT('Ctrl Pts',(2.15492920379552,-4.04105333854382,383.44030671571));
#28814=CARTESIAN_POINT('Ctrl Pts',(1.44530565223012,-4.34567871913682,383.413930757223));
#28815=CARTESIAN_POINT('Ctrl Pts',(0.705993253592304,-4.46263857526945,
383.387554798737));
#28816=CARTESIAN_POINT('Ctrl Pts',(-0.0333191450455116,-4.57959843140208,
383.36117884025));
#28817=CARTESIAN_POINT('Ctrl Pts',(-0.802320390755788,-4.50889276307437,
383.334802881763));
#28818=CARTESIAN_POINT('Ctrl Pts',(-1.50791010623509,-4.25908166617111,
383.308426923277));
#28819=CARTESIAN_POINT('Ctrl Pts',(-2.21349982171436,-4.00927056926786,
383.28205096479));
#28820=CARTESIAN_POINT('Ctrl Pts',(-2.8556780069626,-3.58035404378911,383.255675006304));
#28821=CARTESIAN_POINT('Ctrl Pts',(-3.35669832323709,-3.02425956134359,
383.229299047817));
#28822=CARTESIAN_POINT('Ctrl Pts',(-3.85771863951158,-2.46816507889806,
383.20292308933));
#28823=CARTESIAN_POINT('Ctrl Pts',(-4.21758108681228,-1.78489263948572,
383.176547130844));
#28824=CARTESIAN_POINT('Ctrl Pts',(-4.39271833698727,-1.05716372407332,
383.150171172357));
#28825=CARTESIAN_POINT('Ctrl Pts',(-4.4759132430793,-0.711472908911519,
383.137641882402));
#28826=CARTESIAN_POINT('Ctrl Pts',(-4.51742480471468,-0.355750464977554,
383.125112592447));
#28827=CARTESIAN_POINT('Ctrl Pts',(-4.51737744603353,-1.71510238390164E-5,
383.112583302492));
#28828=CARTESIAN_POINT('Ctrl Pts',(-4.51810647145572,4.12515443024009E-5,
383.387416697508));
#28829=CARTESIAN_POINT('Ctrl Pts',(-4.51776653385746,-0.70808283654263,
383.412369141307));
#28830=CARTESIAN_POINT('Ctrl Pts',(-4.34843679840707,-1.41636380567975,
383.437321585107));
#28831=CARTESIAN_POINT('Ctrl Pts',(-4.0275273935072,-2.04758215167448,383.462274028906));
#28832=CARTESIAN_POINT('Ctrl Pts',(-3.68831039297495,-2.71481094191849,
383.488649987393));
#28833=CARTESIAN_POINT('Ctrl Pts',(-3.17972542149173,-3.29593359296068,
383.515025945879));
#28834=CARTESIAN_POINT('Ctrl Pts',(-2.56334513970026,-3.72059555287616,
383.541401904366));
#28835=CARTESIAN_POINT('Ctrl Pts',(-1.94696485790879,-4.14525751279165,
383.567777862853));
#28836=CARTESIAN_POINT('Ctrl Pts',(-1.22278926580908,-4.41345878158044,
383.594153821339));
#28837=CARTESIAN_POINT('Ctrl Pts',(-0.478491850582746,-4.49272913964694,
383.620529779826));
#28838=CARTESIAN_POINT('Ctrl Pts',(0.265805564643564,-4.57199949771343,
383.646905738312));
#28839=CARTESIAN_POINT('Ctrl Pts',(1.0302248029965,-4.46233894505765,383.673281696799));
#28840=CARTESIAN_POINT('Ctrl Pts',(1.72222021529061,-4.17702371352512,383.699657655286));
#28841=CARTESIAN_POINT('Ctrl Pts',(2.41421562758474,-3.89170848199258,383.726033613772));
#28842=CARTESIAN_POINT('Ctrl Pts',(3.03378721382,-3.43073857158334,383.752409572259));
#28843=CARTESIAN_POINT('Ctrl Pts',(3.50592553965972,-2.84992204870037,383.778785530746));
#28844=CARTESIAN_POINT('Ctrl Pts',(3.97806386549944,-2.2691055258174,383.805161489232));
#28845=CARTESIAN_POINT('Ctrl Pts',(4.30276893094358,-1.56844239046068,383.831537447719));
#28846=CARTESIAN_POINT('Ctrl Pts',(4.44072979303352,-0.832759556277373,
383.857913406205));
#28847=CARTESIAN_POINT('Ctrl Pts',(4.57869065512346,-0.0970767220940631,
383.884289364692));
#28848=CARTESIAN_POINT('Ctrl Pts',(4.52990731385923,0.673625810915847,383.910665323178));
#28849=CARTESIAN_POINT('Ctrl Pts',(4.30028580320783,1.38604169635549,383.937041281665));
#28850=CARTESIAN_POINT('Ctrl Pts',(4.07066429255644,2.0984575817951,383.963417240152));
#28851=CARTESIAN_POINT('Ctrl Pts',(3.66020461251785,2.75258681966445,383.989793198638));
#28852=CARTESIAN_POINT('Ctrl Pts',(3.11859972691059,3.26923619774099,384.016169157125));
#28853=CARTESIAN_POINT('Ctrl Pts',(2.57699484130331,3.78588557581757,384.042545115611));
#28854=CARTESIAN_POINT('Ctrl Pts',(1.90424475012738,4.16505509410136,384.068921074098));
#28855=CARTESIAN_POINT('Ctrl Pts',(1.18179702927259,4.36083998272228,384.095297032584));
#28856=CARTESIAN_POINT('Ctrl Pts',(0.459349308417798,4.55662487134321,384.121672991071));
#28857=CARTESIAN_POINT('Ctrl Pts',(-0.312796042115809,4.56902513030122,
384.148048949558));
#28858=CARTESIAN_POINT('Ctrl Pts',(-1.04115799889843,4.39653950222634,384.174424908044));
#28859=CARTESIAN_POINT('Ctrl Pts',(-1.76951995568104,4.22405387415146,384.200800866531));
#28860=CARTESIAN_POINT('Ctrl Pts',(-2.45409851871268,3.86668235904368,384.227176825017));
#28861=CARTESIAN_POINT('Ctrl Pts',(-3.0120140790621,3.36769071632751,384.253552783504));
#28862=CARTESIAN_POINT('Ctrl Pts',(-3.56992963941149,2.86869907361137,384.279928741991));
#28863=CARTESIAN_POINT('Ctrl Pts',(-4.00118219707867,2.22808730328684,384.306304700477));
#28864=CARTESIAN_POINT('Ctrl Pts',(-4.25356146494663,1.52341210354517,384.332680658964));
#28865=CARTESIAN_POINT('Ctrl Pts',(-4.42814268873775,1.0359589946372,384.350926005145));
#28866=CARTESIAN_POINT('Ctrl Pts',(-4.51713190568983,0.51785112729682,384.369171351326));
#28867=CARTESIAN_POINT('Ctrl Pts',(-4.51758348284472,-0.000105543616906456,
384.387416697508));
#28868=CARTESIAN_POINT('Origin',(0.,0.,387.));
#28869=CARTESIAN_POINT('',(-4.51754236316255,9.86160820556914E-5,385.387416697508));
#28870=CARTESIAN_POINT('',(-4.51782825948384,-0.000111641905798056,385.112583302492));
#28871=CARTESIAN_POINT('',(-4.51775,5.53264807684796E-16,387.));
#28872=CARTESIAN_POINT('Ctrl Pts',(-4.51782825948384,-0.000111641905798056,
385.112583302492));
#28873=CARTESIAN_POINT('Ctrl Pts',(-4.51721726779753,0.599198793910267,
385.091468929459));
#28874=CARTESIAN_POINT('Ctrl Pts',(-4.39722715972494,1.19874658011254,385.070354556425));
#28875=CARTESIAN_POINT('Ctrl Pts',(-4.16499712691276,1.75110492558535,385.049240183392));
#28876=CARTESIAN_POINT('Ctrl Pts',(-3.87489664914265,2.44110792813221,385.022864224905));
#28877=CARTESIAN_POINT('Ctrl Pts',(-3.40964724164981,3.05747242764947,384.996488266419));
#28878=CARTESIAN_POINT('Ctrl Pts',(-2.82557507506063,3.52557726093145,384.970112307932));
#28879=CARTESIAN_POINT('Ctrl Pts',(-2.24150290847142,3.99368209421345,384.943736349446));
#28880=CARTESIAN_POINT('Ctrl Pts',(-1.53860798278584,4.31352726126017,384.917360390959));
#28881=CARTESIAN_POINT('Ctrl Pts',(-0.801987406950171,4.44639019055842,
384.890984432472));
#28882=CARTESIAN_POINT('Ctrl Pts',(-0.065366831114539,4.57925311985666,
384.864608473986));
#28883=CARTESIAN_POINT('Ctrl Pts',(0.7049793948712,4.52513381140646,384.838232515499));
#28884=CARTESIAN_POINT('Ctrl Pts',(1.41578806149518,4.29058430665667,384.811856557012));
#28885=CARTESIAN_POINT('Ctrl Pts',(2.12659672811916,4.05603480190689,384.785480598526));
#28886=CARTESIAN_POINT('Ctrl Pts',(2.77786783538139,3.64105510085751,384.759104640039));
#28887=CARTESIAN_POINT('Ctrl Pts',(3.29075419525559,3.09588539096791,384.732728681553));
#28888=CARTESIAN_POINT('Ctrl Pts',(3.8036405551298,2.55071568107831,384.706352723066));
#28889=CARTESIAN_POINT('Ctrl Pts',(4.178142167616,1.87535596234848,384.67997676458));
#28890=CARTESIAN_POINT('Ctrl Pts',(4.36891939039539,1.15156974944116,384.653600806093));
#28891=CARTESIAN_POINT('Ctrl Pts',(4.55969661317478,0.427783536533828,384.627224847606));
#28892=CARTESIAN_POINT('Ctrl Pts',(4.56674944624736,-0.344429170550942,
384.60084888912));
#28893=CARTESIAN_POINT('Ctrl Pts',(4.38922402699095,-1.07157919375385,384.574472930633));
#28894=CARTESIAN_POINT('Ctrl Pts',(4.21169860773453,-1.79872921695679,384.548096972147));
#28895=CARTESIAN_POINT('Ctrl Pts',(3.84959493614911,-2.48081655627781,384.52172101366));
#28896=CARTESIAN_POINT('Ctrl Pts',(3.34675167782285,-3.03526320680608,384.495345055174));
#28897=CARTESIAN_POINT('Ctrl Pts',(2.84390841949662,-3.58970985733432,384.468969096687));
#28898=CARTESIAN_POINT('Ctrl Pts',(2.20032557442955,-4.01651581906983,384.4425931382));
#28899=CARTESIAN_POINT('Ctrl Pts',(1.49391953877316,-4.26400913921072,384.416217179714));
#28900=CARTESIAN_POINT('Ctrl Pts',(0.787513503116781,-4.51150245935161,
384.389841221227));
#28901=CARTESIAN_POINT('Ctrl Pts',(0.0182842768710745,-4.57968313789789,
384.363465262741));
#28902=CARTESIAN_POINT('Ctrl Pts',(-0.720640161828923,-4.46029677092904,
384.337089304254));
#28903=CARTESIAN_POINT('Ctrl Pts',(-1.45956460052894,-4.34091040396018,
384.310713345767));
#28904=CARTESIAN_POINT('Ctrl Pts',(-2.16818425168326,-4.03395699147619,
384.284337387281));
#28905=CARTESIAN_POINT('Ctrl Pts',(-2.76070893321464,-3.57659834391139,
384.257961428794));
#28906=CARTESIAN_POINT('Ctrl Pts',(-3.35323361474601,-3.11923969634659,
384.231585470308));
#28907=CARTESIAN_POINT('Ctrl Pts',(-3.82966332665445,-2.51147581370097,
384.205209511821));
#28908=CARTESIAN_POINT('Ctrl Pts',(-4.13231833670975,-1.82688661161363,
384.178833553334));
#28909=CARTESIAN_POINT('Ctrl Pts',(-4.38571791578798,-1.25371052039765,
384.156750136387));
#28910=CARTESIAN_POINT('Ctrl Pts',(-4.51730198273802,-0.626680125117799,
384.134666719439));
#28911=CARTESIAN_POINT('Ctrl Pts',(-4.51791286673421,0.000101789655423226,
384.112583302492));
#28912=CARTESIAN_POINT('Ctrl Pts',(-4.51758348284472,-0.000105543616906456,
384.387416697508));
#28913=CARTESIAN_POINT('Ctrl Pts',(-4.51778471765472,-0.230920834279876,
384.395547309813));
#28914=CARTESIAN_POINT('Ctrl Pts',(-4.50040387332536,-0.461706099887457,
384.403677922118));
#28915=CARTESIAN_POINT('Ctrl Pts',(-4.46518027924831,-0.689735200724739,
384.411808534423));
#28916=CARTESIAN_POINT('Ctrl Pts',(-4.35091384761331,-1.42946867609407,
384.43818449291));
#28917=CARTESIAN_POINT('Ctrl Pts',(-4.04887500627456,-2.14019699767394,
384.464560451397));
#28918=CARTESIAN_POINT('Ctrl Pts',(-3.59563057517656,-2.73587469379764,
384.490936409884));
#28919=CARTESIAN_POINT('Ctrl Pts',(-3.14238614407856,-3.33155238992132,
384.51731236837));
#28920=CARTESIAN_POINT('Ctrl Pts',(-2.53793612322135,-3.81217946058886,
384.543688326857));
#28921=CARTESIAN_POINT('Ctrl Pts',(-1.85545923021652,-4.11956801355568,
384.570064285343));
#28922=CARTESIAN_POINT('Ctrl Pts',(-1.17298233721168,-4.42695656652252,
384.59644024383));
#28923=CARTESIAN_POINT('Ctrl Pts',(-0.412478572059261,-4.56110660178858,
384.622816202316));
#28924=CARTESIAN_POINT('Ctrl Pts',(0.333980449139521,-4.50577702875979,
384.649192160803));
#28925=CARTESIAN_POINT('Ctrl Pts',(1.08043947033828,-4.450447455731,384.67556811929));
#28926=CARTESIAN_POINT('Ctrl Pts',(1.81285374758341,-4.20563827440736,384.701944077776));
#28927=CARTESIAN_POINT('Ctrl Pts',(2.44255236397545,-3.80098770355085,384.728320036263));
#28928=CARTESIAN_POINT('Ctrl Pts',(3.0722509803675,-3.39633713269433,384.754695994749));
#28929=CARTESIAN_POINT('Ctrl Pts',(3.59923393590646,-2.83184517230493,384.781071953236));
#28930=CARTESIAN_POINT('Ctrl Pts',(3.95970118830781,-2.17585295289468,384.807447911723));
#28931=CARTESIAN_POINT('Ctrl Pts',(4.32016844070917,-1.51986073348444,384.833823870209));
#28932=CARTESIAN_POINT('Ctrl Pts',(4.51411998997293,-0.772368255053362,
384.860199828696));
#28933=CARTESIAN_POINT('Ctrl Pts',(4.51807477866807,-0.023871901270034,
384.886575787182));
#28934=CARTESIAN_POINT('Ctrl Pts',(4.52202956736322,0.724624452513337,384.912951745669));
#28935=CARTESIAN_POINT('Ctrl Pts',(4.33598759548973,1.47412468164896,384.939327704155));
#28936=CARTESIAN_POINT('Ctrl Pts',(3.98247233472248,2.13388933088782,384.965703662642));
#28937=CARTESIAN_POINT('Ctrl Pts',(3.62895707395525,2.79365398012665,384.992079621129));
#28938=CARTESIAN_POINT('Ctrl Pts',(3.10796852429429,3.36368304946875,385.018455579615));
#28939=CARTESIAN_POINT('Ctrl Pts',(2.48258100559898,3.77496504936747,385.044831538102));
#28940=CARTESIAN_POINT('Ctrl Pts',(1.8571934869037,4.18624704926618,385.071207496588));
#28941=CARTESIAN_POINT('Ctrl Pts',(1.12740699917409,4.43878197972154,385.097583455075));
#28942=CARTESIAN_POINT('Ctrl Pts',(0.38157432172954,4.50199629168033,385.123959413562));
#28943=CARTESIAN_POINT('Ctrl Pts',(-0.364258355715052,4.56521060363914,
385.150335372048));
#28944=CARTESIAN_POINT('Ctrl Pts',(-1.12613722287458,4.43910429710136,385.176711330535));
#28945=CARTESIAN_POINT('Ctrl Pts',(-1.81182418470336,4.13894463565663,385.203087289021));
#28946=CARTESIAN_POINT('Ctrl Pts',(-2.49751114653216,3.8387849742119,385.229463247508));
#28947=CARTESIAN_POINT('Ctrl Pts',(-3.1070062030302,3.36457195786021,385.255839205995));
#28948=CARTESIAN_POINT('Ctrl Pts',(-3.56651985120111,2.7737169510055,385.282215164481));
#28949=CARTESIAN_POINT('Ctrl Pts',(-4.02603349937199,2.18286194415082,385.308591122968));
#28950=CARTESIAN_POINT('Ctrl Pts',(-4.33556573921576,1.47536494679312,385.334967081454));
#28951=CARTESIAN_POINT('Ctrl Pts',(-4.45764255040047,0.736880225115328,
385.361343039941));
#28952=CARTESIAN_POINT('Ctrl Pts',(-4.49786843733614,0.493539965571841,
385.37003425913));
#28953=CARTESIAN_POINT('Ctrl Pts',(-4.51774064501623,0.246835097138747,
385.378725478319));
#28954=CARTESIAN_POINT('Ctrl Pts',(-4.51754236316255,9.86160820556914E-5,
385.387416697508));
#28955=CARTESIAN_POINT('Origin',(0.,0.,387.));
#28956=CARTESIAN_POINT('',(-4.51812581071634,-2.54303748789628E-5,386.387416697508));
#28957=CARTESIAN_POINT('',(-4.51739693228094,4.16105383547416E-5,386.112583302492));
#28958=CARTESIAN_POINT('',(-4.51775,5.53264807684796E-16,387.));
#28959=CARTESIAN_POINT('Ctrl Pts',(-4.51739693228094,4.16105383547416E-5,
386.112583302492));
#28960=CARTESIAN_POINT('Ctrl Pts',(-4.51750350848484,0.328257645647765,
386.101023056451));
#28961=CARTESIAN_POINT('Ctrl Pts',(-4.48221658085224,0.656451107309221,
386.08946281041));
#28962=CARTESIAN_POINT('Ctrl Pts',(-4.41129467440341,0.976754228647579,
386.077902564369));
#28963=CARTESIAN_POINT('Ctrl Pts',(-4.24947863228365,1.70756063203963,386.051526605882));
#28964=CARTESIAN_POINT('Ctrl Pts',(-3.90215620987833,2.39729198722953,386.025150647396));
#28965=CARTESIAN_POINT('Ctrl Pts',(-3.41137655698045,2.96244485418463,385.998774688909));
#28966=CARTESIAN_POINT('Ctrl Pts',(-2.92059690408257,3.52759772113973,385.972398730423));
#28967=CARTESIAN_POINT('Ctrl Pts',(-2.28636002069214,3.96817209986003,385.946022771936));
#28968=CARTESIAN_POINT('Ctrl Pts',(-1.58545081902196,4.23082914191337,385.91964681345));
#28969=CARTESIAN_POINT('Ctrl Pts',(-0.884541617351764,4.49348618396671,
385.893270854963));
#28970=CARTESIAN_POINT('Ctrl Pts',(-0.116960097401826,4.57822588935307,
385.866894896476));
#28971=CARTESIAN_POINT('Ctrl Pts',(0.624365244915622,4.47478910883432,385.84051893799));
#28972=CARTESIAN_POINT('Ctrl Pts',(1.36569058723307,4.37135232831557,385.814142979503));
#28973=CARTESIAN_POINT('Ctrl Pts',(2.08075975191802,4.07973906189171,385.787767021017));
#28974=CARTESIAN_POINT('Ctrl Pts',(2.68300173612543,3.63525394044883,385.76139106253));
#28975=CARTESIAN_POINT('Ctrl Pts',(3.28524372033282,3.19076881900596,385.735015104043));
#28976=CARTESIAN_POINT('Ctrl Pts',(3.77465852406267,2.5934118425441,385.708639145557));
#28977=CARTESIAN_POINT('Ctrl Pts',(4.09199435398004,1.91550299780405,385.68226318707));
#28978=CARTESIAN_POINT('Ctrl Pts',(4.4093301838974,1.23759415306402,385.655887228584));
#28979=CARTESIAN_POINT('Ctrl Pts',(4.55458704000229,0.479133440045757,385.629511270097));
#28980=CARTESIAN_POINT('Ctrl Pts',(4.51017916650468,-0.268054870554405,
385.60313531161));
#28981=CARTESIAN_POINT('Ctrl Pts',(4.46577129300707,-1.01524318115463,385.576759353124));
#28982=CARTESIAN_POINT('Ctrl Pts',(4.23169868990694,-1.7511590893368,385.550383394637));
#28983=CARTESIAN_POINT('Ctrl Pts',(3.83629973479027,-2.38670774759897,385.524007436151));
#28984=CARTESIAN_POINT('Ctrl Pts',(3.44090077967361,-3.0222564058611,385.497631477664));
#28985=CARTESIAN_POINT('Ctrl Pts',(2.88417547254044,-3.55743781420323,385.471255519177));
#28986=CARTESIAN_POINT('Ctrl Pts',(2.23352466148768,-3.92745937141648,385.444879560691));
#28987=CARTESIAN_POINT('Ctrl Pts',(1.58287385043492,-4.29748092862973,385.418503602204));
#28988=CARTESIAN_POINT('Ctrl Pts',(0.838297535462584,-4.5023426347141,385.392127643717));
#28989=CARTESIAN_POINT('Ctrl Pts',(0.0899390502021953,-4.5172425764895,
385.365751685231));
#28990=CARTESIAN_POINT('Ctrl Pts',(-0.658419435058194,-4.53214251826491,
385.339375726744));
#28991=CARTESIAN_POINT('Ctrl Pts',(-1.41056009060662,-4.35708069573135,
385.312999768258));
#28992=CARTESIAN_POINT('Ctrl Pts',(-2.07542379370768,-4.01325125105728,
385.286623809771));
#28993=CARTESIAN_POINT('Ctrl Pts',(-2.74028749680876,-3.6694218063832,385.260247851285));
#28994=CARTESIAN_POINT('Ctrl Pts',(-3.31787424746246,-3.15682473956861,
385.233871892798));
#28995=CARTESIAN_POINT('Ctrl Pts',(-3.73825757323288,-2.53751844205472,
385.207495934311));
#28996=CARTESIAN_POINT('Ctrl Pts',(-4.15864089900331,-1.91821214454083,
385.181119975825));
#28997=CARTESIAN_POINT('Ctrl Pts',(-4.42182079989046,-1.19219661632765,
385.154744017338));
#28998=CARTESIAN_POINT('Ctrl Pts',(-4.49593497631034,-0.44736809943281,
385.128368058852));
#28999=CARTESIAN_POINT('Ctrl Pts',(-4.51071957921785,-0.298786621658729,
385.123106473398));
#29000=CARTESIAN_POINT('Ctrl Pts',(-4.51798051524647,-0.149456501261902,
385.117844887945));
#29001=CARTESIAN_POINT('Ctrl Pts',(-4.51782825948384,-0.000111641905798056,
385.112583302492));
#29002=CARTESIAN_POINT('Ctrl Pts',(-4.51754236316255,9.86160820556914E-5,
385.387416697508));
#29003=CARTESIAN_POINT('Ctrl Pts',(-4.51713890274882,-0.501956417601758,
385.405101436806));
#29004=CARTESIAN_POINT('Ctrl Pts',(-4.43363680853372,-1.00414233826904,
385.422786176103));
#29005=CARTESIAN_POINT('Ctrl Pts',(-4.26942186585053,-1.47837968895145,
385.440470915401));
#29006=CARTESIAN_POINT('Ctrl Pts',(-4.02450298759024,-2.18568243534247,
385.466846873887));
#29007=CARTESIAN_POINT('Ctrl Pts',(-3.60004384854402,-2.83081548212662,
385.493222832374));
#29008=CARTESIAN_POINT('Ctrl Pts',(-3.04743227963612,-3.33567475547881,
385.519598790861));
#29009=CARTESIAN_POINT('Ctrl Pts',(-2.49482071072822,-3.84053402883101,
385.545974749347));
#29010=CARTESIAN_POINT('Ctrl Pts',(-1.81405671195863,-4.20511952875126,
385.572350707834));
#29011=CARTESIAN_POINT('Ctrl Pts',(-1.0875580758779,-4.38529212309734,385.59872666632));
#29012=CARTESIAN_POINT('Ctrl Pts',(-0.361059439797152,-4.56546471744342,
385.625102624807));
#29013=CARTESIAN_POINT('Ctrl Pts',(0.411173833594756,-4.56122440621533,
385.651478583294));
#29014=CARTESIAN_POINT('Ctrl Pts',(1.13565007634523,-4.37308454953753,385.67785454178));
#29015=CARTESIAN_POINT('Ctrl Pts',(1.86012631909569,-4.18494469285974,385.704230500267));
#29016=CARTESIAN_POINT('Ctrl Pts',(2.53684553120472,-3.81290529073225,385.730606458753));
#29017=CARTESIAN_POINT('Ctrl Pts',(3.08387960874885,-3.30200789400175,385.75698241724));
#29018=CARTESIAN_POINT('Ctrl Pts',(3.63091368629297,-2.79111049727125,385.783358375726));
#29019=CARTESIAN_POINT('Ctrl Pts',(4.04826262927219,-2.14135510593772,385.809734334213));
#29020=CARTESIAN_POINT('Ctrl Pts',(4.28539941412795,-1.43140540543153,385.8361102927));
#29021=CARTESIAN_POINT('Ctrl Pts',(4.52253619898372,-0.721455704925321,
385.862486251186));
#29022=CARTESIAN_POINT('Ctrl Pts',(4.57946082571602,0.048688304753508,385.888862209673));
#29023=CARTESIAN_POINT('Ctrl Pts',(4.44928162248921,0.785787895736858,385.915238168159));
#29024=CARTESIAN_POINT('Ctrl Pts',(4.31910241926241,1.52288748672023,385.941614126646));
#29025=CARTESIAN_POINT('Ctrl Pts',(4.00181938607647,2.22694265900807,385.967990085133));
#29026=CARTESIAN_POINT('Ctrl Pts',(3.53584490557238,2.81271583652609,385.994366043619));
#29027=CARTESIAN_POINT('Ctrl Pts',(3.06987042506831,3.39848901404408,386.020742002106));
#29028=CARTESIAN_POINT('Ctrl Pts',(2.45520449724608,3.86598019679227,386.047117960592));
#29029=CARTESIAN_POINT('Ctrl Pts',(1.76626264498691,4.1585918100038,386.073493919079));
#29030=CARTESIAN_POINT('Ctrl Pts',(1.07732079272774,4.45120342321533,386.099869877566));
#29031=CARTESIAN_POINT('Ctrl Pts',(0.3141030160316,4.56893546689021,386.126245836052));
#29032=CARTESIAN_POINT('Ctrl Pts',(-0.43099049281119,4.49753452109188,386.152621794539));
#29033=CARTESIAN_POINT('Ctrl Pts',(-1.17608400165398,4.42613357529356,386.178997753025));
#29034=CARTESIAN_POINT('Ctrl Pts',(-1.90305324264344,4.16559964002203,386.205373711512));
#29035=CARTESIAN_POINT('Ctrl Pts',(-2.52388651098497,3.74747467676233,386.231749669998));
#29036=CARTESIAN_POINT('Ctrl Pts',(-3.14471977932654,3.3293497135026,386.258125628485));
#29037=CARTESIAN_POINT('Ctrl Pts',(-3.65941707502018,2.75363372225468,386.284501586972));
#29038=CARTESIAN_POINT('Ctrl Pts',(-4.00566573902476,2.09002668894682,386.310877545458));
#29039=CARTESIAN_POINT('Ctrl Pts',(-4.34058663747219,1.44813002069409,386.336390596142));
#29040=CARTESIAN_POINT('Ctrl Pts',(-4.51790043884109,0.723999072118772,
386.361903646825));
#29041=CARTESIAN_POINT('Ctrl Pts',(-4.51812581071634,-2.54303748789628E-5,
386.387416697508));
#29042=CARTESIAN_POINT('Origin',(0.,0.,387.));
#29043=CARTESIAN_POINT('',(-4.51744020728156,-6.7888199640348E-5,387.387416697508));
#29044=CARTESIAN_POINT('',(-4.51807831563064,5.66723631286815E-5,387.112583302492));
#29045=CARTESIAN_POINT('',(-4.51775,5.53264807684796E-16,387.));
#29046=CARTESIAN_POINT('Ctrl Pts',(-4.51807831563064,5.66723631286815E-5,
387.112583302492));
#29047=CARTESIAN_POINT('Ctrl Pts',(-4.51811411951228,0.0569892498064094,
387.110577183443));
#29048=CARTESIAN_POINT('Ctrl Pts',(-4.51706018525489,0.113920500037806,
387.108571064395));
#29049=CARTESIAN_POINT('Ctrl Pts',(-4.51490790649659,0.170810197164546,
387.106564945346));
#29050=CARTESIAN_POINT('Ctrl Pts',(-4.4866102761939,0.918781904413813,387.08018898686));
#29051=CARTESIAN_POINT('Ctrl Pts',(-4.26844906050963,1.65957059993282,387.053813028373));
#29052=CARTESIAN_POINT('Ctrl Pts',(-3.88683629922459,2.30349150435396,387.027437069886));
#29053=CARTESIAN_POINT('Ctrl Pts',(-3.50522353793953,2.94741240877514,387.0010611114));
#29054=CARTESIAN_POINT('Ctrl Pts',(-2.96015923105368,3.49446552209844,386.974685152913));
#29055=CARTESIAN_POINT('Ctrl Pts',(-2.31763246884327,3.87842097598549,386.948309194426));
#29056=CARTESIAN_POINT('Ctrl Pts',(-1.67510570663291,4.26237642987252,386.92193323594));
#29057=CARTESIAN_POINT('Ctrl Pts',(-0.935116489098005,4.48323422432332,
386.895557277453));
#29058=CARTESIAN_POINT('Ctrl Pts',(-0.187252805513337,4.51425585389532,
386.869181318967));
#29059=CARTESIAN_POINT('Ctrl Pts',(0.560610878071331,4.54527748346732,386.84280536048));
#29060=CARTESIAN_POINT('Ctrl Pts',(1.31634902770576,4.38646294816051,386.816429401993));
#29061=CARTESIAN_POINT('Ctrl Pts',(1.98846698422516,4.05703938608529,386.790053443507));
#29062=CARTESIAN_POINT('Ctrl Pts',(2.66058494074455,3.72761582401007,386.76367748502));
#29063=CARTESIAN_POINT('Ctrl Pts',(3.2490827041489,3.22758323516643,386.737301526534));
#29064=CARTESIAN_POINT('Ctrl Pts',(3.68271284262869,2.6174788721857,386.710925568047));
#29065=CARTESIAN_POINT('Ctrl Pts',(4.1163429811085,2.00737450920494,386.684549609561));
#29066=CARTESIAN_POINT('Ctrl Pts',(4.39510549466373,1.28719837208709,386.658173651074));
#29067=CARTESIAN_POINT('Ctrl Pts',(4.48525154955086,0.544139747539571,386.631797692587));
#29068=CARTESIAN_POINT('Ctrl Pts',(4.57539760443799,-0.198918877007948,
386.605421734101));
#29069=CARTESIAN_POINT('Ctrl Pts',(4.47692720065701,-0.96485998898513,386.579045775614));
#29070=CARTESIAN_POINT('Ctrl Pts',(4.20176181661432,-1.66095369111926,386.552669817128));
#29071=CARTESIAN_POINT('Ctrl Pts',(3.92659643257165,-2.35704739325338,386.526293858641));
#29072=CARTESIAN_POINT('Ctrl Pts',(3.47473606826728,-2.98329368554445,386.499917900154));
#29073=CARTESIAN_POINT('Ctrl Pts',(2.90088592819845,-3.46387504959129,386.473541941668));
#29074=CARTESIAN_POINT('Ctrl Pts',(2.32703578812962,-3.94445641363812,386.447165983181));
#29075=CARTESIAN_POINT('Ctrl Pts',(1.63119587229633,-4.27937284944072,386.420790024695));
#29076=CARTESIAN_POINT('Ctrl Pts',(0.897609163487301,-4.4280771580026,386.394414066208));
#29077=CARTESIAN_POINT('Ctrl Pts',(0.164022454678273,-4.57678146656449,
386.368038107722));
#29078=CARTESIAN_POINT('Ctrl Pts',(-0.607311047106494,-4.53927364788568,
386.341662149235));
#29079=CARTESIAN_POINT('Ctrl Pts',(-1.32300860621665,-4.3200946465879,386.315286190748));
#29080=CARTESIAN_POINT('Ctrl Pts',(-2.03870616532682,-4.10091564529013,
386.288910232262));
#29081=CARTESIAN_POINT('Ctrl Pts',(-2.69876778176237,-3.7000654613734,386.262534273775));
#29082=CARTESIAN_POINT('Ctrl Pts',(-3.22328203031241,-3.16607366949443,
386.236158315289));
#29083=CARTESIAN_POINT('Ctrl Pts',(-3.74779627886247,-2.63208187761544,
386.209782356802));
#29084=CARTESIAN_POINT('Ctrl Pts',(-4.136763159527,-1.9649484777742,386.183406398315));
#29085=CARTESIAN_POINT('Ctrl Pts',(-4.34309176894218,-1.24544105205646,
386.157030439829));
#29086=CARTESIAN_POINT('Ctrl Pts',(-4.45898918165419,-0.84128454994014,
386.142214727383));
#29087=CARTESIAN_POINT('Ctrl Pts',(-4.51726034328579,-0.420602931019958,
386.127399014937));
#29088=CARTESIAN_POINT('Ctrl Pts',(-4.51739693228094,4.16105383547416E-5,
386.112583302492));
#29089=CARTESIAN_POINT('Ctrl Pts',(-4.51812581071634,-2.54303748789628E-5,
386.387416697508));
#29090=CARTESIAN_POINT('Ctrl Pts',(-4.51813343329163,-0.024513540432781,
386.388279605311));
#29091=CARTESIAN_POINT('Ctrl Pts',(-4.51793847697299,-0.049001528722538,
386.389142513115));
#29092=CARTESIAN_POINT('Ctrl Pts',(-4.51754018801501,-0.0734862094280138,
386.390005420918));
#29093=CARTESIAN_POINT('Ctrl Pts',(-4.50536594068517,-0.821893999127264,
386.416381379405));
#29094=CARTESIAN_POINT('Ctrl Pts',(-4.30321741370996,-1.56721150315799,
386.442757337891));
#29095=CARTESIAN_POINT('Ctrl Pts',(-3.9355680448604,-2.21920565463873,386.469133296378));
#29096=CARTESIAN_POINT('Ctrl Pts',(-3.56791867601083,-2.87119980611948,
386.495509254864));
#29097=CARTESIAN_POINT('Ctrl Pts',(-3.03476846528691,-3.42987060505022,
386.521885213351));
#29098=CARTESIAN_POINT('Ctrl Pts',(-2.40066410367865,-3.8275816692287,386.548261171838));
#29099=CARTESIAN_POINT('Ctrl Pts',(-1.76655974207041,-4.22529273340718,
386.574637130324));
#29100=CARTESIAN_POINT('Ctrl Pts',(-1.0315012295778,-4.46204406283341,386.601013088811));
#29101=CARTESIAN_POINT('Ctrl Pts',(-0.28447961170951,-4.50917297559413,
386.627389047297));
#29102=CARTESIAN_POINT('Ctrl Pts',(0.4625420061588,-4.55630188835485,386.653765005784));
#29103=CARTESIAN_POINT('Ctrl Pts',(1.22152672940277,-4.4138083844501,386.68014096427));
#29104=CARTESIAN_POINT('Ctrl Pts',(1.90058684718235,-4.09894366997453,386.706516922757));
#29105=CARTESIAN_POINT('Ctrl Pts',(2.57964696496189,-3.78407895549898,386.732892881244));
#29106=CARTESIAN_POINT('Ctrl Pts',(3.17878247727702,-3.29684303045261,386.75926883973));
#29107=CARTESIAN_POINT('Ctrl Pts',(3.62545807607245,-2.69622389870498,386.785644798217));
#29108=CARTESIAN_POINT('Ctrl Pts',(4.07213367486792,-2.0956047669573,386.812020756704));
#29109=CARTESIAN_POINT('Ctrl Pts',(4.3663493601437,-1.38160242850832,386.83839671519));
#29110=CARTESIAN_POINT('Ctrl Pts',(4.47248543497401,-0.64065872916252,386.864772673677));
#29111=CARTESIAN_POINT('Ctrl Pts',(4.57862150980431,0.10028497018324,386.891148632163));
#29112=CARTESIAN_POINT('Ctrl Pts',(4.49667797418915,0.868170030425805,386.91752459065));
#29113=CARTESIAN_POINT('Ctrl Pts',(4.23657545455911,1.57003120705739,386.943900549137));
#29114=CARTESIAN_POINT('Ctrl Pts',(3.97647293492907,2.27189238368897,386.970276507623));
#29115=CARTESIAN_POINT('Ctrl Pts',(3.53821143128416,2.90772967670955,386.99665246611));
#29116=CARTESIAN_POINT('Ctrl Pts',(2.97484978010159,3.40056441773073,387.023028424596));
#29117=CARTESIAN_POINT('Ctrl Pts',(2.41148812891902,3.8933991587519,387.049404383083));
#29118=CARTESIAN_POINT('Ctrl Pts',(1.72302633019879,4.24323134777366,387.07578034157));
#29119=CARTESIAN_POINT('Ctrl Pts',(0.992814123069943,4.40770798605575,387.102156300056));
#29120=CARTESIAN_POINT('Ctrl Pts',(0.262601915941074,4.57218462433785,387.128532258543));
#29121=CARTESIAN_POINT('Ctrl Pts',(-0.509360699596469,4.55130571188027,
387.154908217029));
#29122=CARTESIAN_POINT('Ctrl Pts',(-1.2296148232201,4.34759898792704,387.181284175516));
#29123=CARTESIAN_POINT('Ctrl Pts',(-1.94986894684372,4.14389226397381,387.207660134002));
#29124=CARTESIAN_POINT('Ctrl Pts',(-2.61841457855343,3.75735772852497,387.234036092489));
#29125=CARTESIAN_POINT('Ctrl Pts',(-3.15431316213248,3.23479180914392,387.260412050976));
#29126=CARTESIAN_POINT('Ctrl Pts',(-3.69021174571151,2.71222588976291,387.286788009462));
#29127=CARTESIAN_POINT('Ctrl Pts',(-4.09346328115986,2.05362858644968,387.313163967949));
#29128=CARTESIAN_POINT('Ctrl Pts',(-4.3152474703208,1.33873404498307,387.339539926435));
#29129=CARTESIAN_POINT('Ctrl Pts',(-4.4494392553304,0.906183036834296,387.355498850126));
#29130=CARTESIAN_POINT('Ctrl Pts',(-4.51719722678179,0.453022038514597,
387.371457773817));
#29131=CARTESIAN_POINT('Ctrl Pts',(-4.51744020728156,-6.7888199640348E-5,
387.387416697508));
#29132=CARTESIAN_POINT('Origin',(0.,0.,387.));
#29133=CARTESIAN_POINT('',(-4.51772665650122,0.000115440622527052,388.387416697508));
#29134=CARTESIAN_POINT('',(-4.51762944300479,-0.000110891096316518,388.112583302492));
#29135=CARTESIAN_POINT('',(-4.51775,5.53264807684796E-16,387.));
#29136=CARTESIAN_POINT('Ctrl Pts',(-4.51762944300479,-0.000110891096316518,
388.112583302492));
#29137=CARTESIAN_POINT('Ctrl Pts',(-4.51713192095981,0.534369387836516,
388.093755351949));
#29138=CARTESIAN_POINT('Ctrl Pts',(-4.42224443214638,1.0690216395804,388.074927401406));
#29139=CARTESIAN_POINT('Ctrl Pts',(-4.23657544981682,1.57003120529822,388.056099450863));
#29140=CARTESIAN_POINT('Ctrl Pts',(-3.97647293047822,2.27189238114416,388.029723492377));
#29141=CARTESIAN_POINT('Ctrl Pts',(-3.53821142732417,2.90772967345308,388.00334753389));
#29142=CARTESIAN_POINT('Ctrl Pts',(-2.97484977677246,3.40056441392273,387.976971575404));
#29143=CARTESIAN_POINT('Ctrl Pts',(-2.41148812622074,3.89339915439239,387.950595616917));
#29144=CARTESIAN_POINT('Ctrl Pts',(-1.72302632827134,4.24323134302276,387.924219658431));
#29145=CARTESIAN_POINT('Ctrl Pts',(-0.992814121960003,4.40770798112098,
387.897843699944));
#29146=CARTESIAN_POINT('Ctrl Pts',(-0.262601915648666,4.5721846192192,387.871467741457));
#29147=CARTESIAN_POINT('Ctrl Pts',(0.509360699024613,4.55130570678527,387.845091782971));
#29148=CARTESIAN_POINT('Ctrl Pts',(1.22961482184198,4.34759898306034,387.818715824484));
#29149=CARTESIAN_POINT('Ctrl Pts',(1.94986894465933,4.14389225933542,387.792339865998));
#29150=CARTESIAN_POINT('Ctrl Pts',(2.61841457562078,3.75735772431952,387.765963907511));
#29151=CARTESIAN_POINT('Ctrl Pts',(3.15431315860007,3.2347918055237,387.739587949024));
#29152=CARTESIAN_POINT('Ctrl Pts',(3.69021174157935,2.71222588672787,387.713211990538));
#29153=CARTESIAN_POINT('Ctrl Pts',(4.09346327657648,2.05362858415213,387.686836032051));
#29154=CARTESIAN_POINT('Ctrl Pts',(4.3152474654894,1.3387340434859,387.660460073565));
#29155=CARTESIAN_POINT('Ctrl Pts',(4.53703165440232,0.62383950281966,387.634084115078));
#29156=CARTESIAN_POINT('Ctrl Pts',(4.57734849723102,-0.147352275937061,
387.607708156591));
#29157=CARTESIAN_POINT('Ctrl Pts',(4.4313169703101,-0.881475715061101,387.581332198105));
#29158=CARTESIAN_POINT('Ctrl Pts',(4.28528544338918,-1.61559915418514,387.554956239618));
#29159=CARTESIAN_POINT('Ctrl Pts',(3.95290554671864,-2.3126542536765,387.528580281132));
#29160=CARTESIAN_POINT('Ctrl Pts',(3.47441738908987,-2.88825091257507,387.502204322645));
#29161=CARTESIAN_POINT('Ctrl Pts',(2.99592923146112,-3.46384757147362,387.475828364158));
#29162=CARTESIAN_POINT('Ctrl Pts',(2.37133281287417,-3.91798578977939,387.449452405672));
#29163=CARTESIAN_POINT('Ctrl Pts',(1.67624590710662,-4.19568459092305,387.423076447185));
#29164=CARTESIAN_POINT('Ctrl Pts',(0.981159001339069,-4.47338339206671,
387.396700488698));
#29165=CARTESIAN_POINT('Ctrl Pts',(0.215581608390928,-4.57464277604826,
387.370324530212));
#29166=CARTESIAN_POINT('Ctrl Pts',(-0.527800408696545,-4.48720361207072,
387.343948571725));
#29167=CARTESIAN_POINT('Ctrl Pts',(-1.27118242578404,-4.39976444809319,
387.317572613239));
#29168=CARTESIAN_POINT('Ctrl Pts',(-1.99236906701087,-4.12362673615656,
387.291196654752));
#29169=CARTESIAN_POINT('Ctrl Pts',(-2.60404870735825,-3.69222153415889,
387.264820696266));
#29170=CARTESIAN_POINT('Ctrl Pts',(-3.21572834770564,-3.26081633216121,
387.238444737779));
#29171=CARTESIAN_POINT('Ctrl Pts',(-3.71790098717359,-2.67414364010249,
387.212068779293));
#29172=CARTESIAN_POINT('Ctrl Pts',(-4.049770284447,-2.00322993458336,387.185692820806));
#29173=CARTESIAN_POINT('Ctrl Pts',(-4.35639806038402,-1.38334500078815,
387.161322981368));
#29174=CARTESIAN_POINT('Ctrl Pts',(-4.51764337890668,-0.691546237269266,
387.13695314193));
#29175=CARTESIAN_POINT('Ctrl Pts',(-4.51807831563064,5.66723631286815E-5,
387.112583302492));
#29176=CARTESIAN_POINT('Ctrl Pts',(-4.51744020728156,-6.7888199640348E-5,
387.387416697508));
#29177=CARTESIAN_POINT('Ctrl Pts',(-4.51759881047873,-0.295818004161051,
387.397833732304));
#29178=CARTESIAN_POINT('Ctrl Pts',(-4.48899129636465,-0.591537838638136,
387.408250767099));
#29179=CARTESIAN_POINT('Ctrl Pts',(-4.43131697527066,-0.881475716049439,
387.418667801895));
#29180=CARTESIAN_POINT('Ctrl Pts',(-4.28528544818601,-1.61559915599528,
387.445043760382));
#29181=CARTESIAN_POINT('Ctrl Pts',(-3.95290555114312,-2.31265425626688,
387.471419718868));
#29182=CARTESIAN_POINT('Ctrl Pts',(-3.47441739297849,-2.88825091580966,
387.497795677355));
#29183=CARTESIAN_POINT('Ctrl Pts',(-2.99592923481386,-3.46384757535244,
387.524171635842));
#29184=CARTESIAN_POINT('Ctrl Pts',(-2.37133281552749,-3.91798579416642,
387.550547594328));
#29185=CARTESIAN_POINT('Ctrl Pts',(-1.67624590898167,-4.19568459562072,
387.576923552815));
#29186=CARTESIAN_POINT('Ctrl Pts',(-0.981159002435877,-4.47338339707502,
387.603299511301));
#29187=CARTESIAN_POINT('Ctrl Pts',(-0.215581608630632,-4.57464278116965,
387.629675469788));
#29188=CARTESIAN_POINT('Ctrl Pts',(0.527800409289026,-4.48720361709396,
387.656051428274));
#29189=CARTESIAN_POINT('Ctrl Pts',(1.27118242720868,-4.39976445301828,387.682427386761));
#29190=CARTESIAN_POINT('Ctrl Pts',(1.99236906924277,-4.12362674077227,387.708803345248));
#29191=CARTESIAN_POINT('Ctrl Pts',(2.60404871027476,-3.69222153829144,387.735179303734));
#29192=CARTESIAN_POINT('Ctrl Pts',(3.21572835130679,-3.26081633581058,387.761555262221));
#29193=CARTESIAN_POINT('Ctrl Pts',(3.71790099133673,-2.67414364309488,387.787931220707));
#29194=CARTESIAN_POINT('Ctrl Pts',(4.04977028898144,-2.00322993682453,387.814307179194));
#29195=CARTESIAN_POINT('Ctrl Pts',(4.38163958662613,-1.33231623055421,387.840683137681));
#29196=CARTESIAN_POINT('Ctrl Pts',(4.54320554188561,-0.577161510729227,
387.867059096167));
#29197=CARTESIAN_POINT('Ctrl Pts',(4.51490791155097,0.170810197357385,387.893435054654));
#29198=CARTESIAN_POINT('Ctrl Pts',(4.48661028121633,0.918781905443997,387.919811013141));
#29199=CARTESIAN_POINT('Ctrl Pts',(4.26844906528759,1.65957060179219,387.946186971627));
#29200=CARTESIAN_POINT('Ctrl Pts',(3.88683630357511,2.30349150693406,387.972562930114));
#29201=CARTESIAN_POINT('Ctrl Pts',(3.50522354186264,2.94741241207594,387.9989388886));
#29202=CARTESIAN_POINT('Ctrl Pts',(2.96015923436644,3.49446552601145,388.025314847087));
#29203=CARTESIAN_POINT('Ctrl Pts',(2.31763247143664,3.87842098032811,388.051690805573));
#29204=CARTESIAN_POINT('Ctrl Pts',(1.67510570850681,4.2623764346448,388.07806676406));
#29205=CARTESIAN_POINT('Ctrl Pts',(0.935116490143367,4.48323422934263,388.104442722547));
#29206=CARTESIAN_POINT('Ctrl Pts',(0.187252805721414,4.5142558589491,388.130818681033));
#29207=CARTESIAN_POINT('Ctrl Pts',(-0.560610878700497,4.54527748855557,
388.15719463952));
#29208=CARTESIAN_POINT('Ctrl Pts',(-1.31634902918093,4.38646295307071,388.183570598006));
#29209=CARTESIAN_POINT('Ctrl Pts',(-1.98846698645264,4.05703939062647,388.209946556493));
#29210=CARTESIAN_POINT('Ctrl Pts',(-2.66058494372436,3.72761582818222,388.23632251498));
#29211=CARTESIAN_POINT('Ctrl Pts',(-3.24908270778736,3.22758323877859,388.262698473466));
#29212=CARTESIAN_POINT('Ctrl Pts',(-3.68271284675239,2.6174788751147,388.289074431953));
#29213=CARTESIAN_POINT('Ctrl Pts',(-4.11634298571743,2.00737451145079,388.315450390439));
#29214=CARTESIAN_POINT('Ctrl Pts',(-4.3951054995845,1.28719837352659,388.341826348926));
#29215=CARTESIAN_POINT('Ctrl Pts',(-4.48525155457229,0.544139748147192,
388.368202307413));
#29216=CARTESIAN_POINT('Ctrl Pts',(-4.50714145691119,0.363704999850856,
388.374607104111));
#29217=CARTESIAN_POINT('Ctrl Pts',(-4.51790959247399,0.181920986011914,
388.381011900809));
#29218=CARTESIAN_POINT('Ctrl Pts',(-4.51772665650122,0.000115440622527052,
388.387416697508));
#29219=CARTESIAN_POINT('Origin',(0.,0.,387.));
#29220=CARTESIAN_POINT('',(-4.51800421755028,-8.27334347235434E-5,389.387416697508));
#29221=CARTESIAN_POINT('',(-4.51750342669873,8.9713446903977E-5,389.112583302492));
#29222=CARTESIAN_POINT('',(-4.51775,5.53264807684796E-16,387.));
#29223=CARTESIAN_POINT('Ctrl Pts',(-4.51750342669873,8.9713446903977E-5,
389.112583302492));
#29224=CARTESIAN_POINT('Ctrl Pts',(-4.51769355714261,0.263372352578081,
389.103309478941));
#29225=CARTESIAN_POINT('Ctrl Pts',(-4.49505280568826,0.526622657629559,
389.094035655391));
#29226=CARTESIAN_POINT('Ctrl Pts',(-4.4492816175085,0.7857878948557,389.084761831841));
#29227=CARTESIAN_POINT('Ctrl Pts',(-4.31910241442768,1.52288748501391,389.058385873354));
#29228=CARTESIAN_POINT('Ctrl Pts',(-4.00181938159719,2.22694265651365,389.032009914867));
#29229=CARTESIAN_POINT('Ctrl Pts',(-3.53584490161497,2.81271583337604,389.005633956381));
#29230=CARTESIAN_POINT('Ctrl Pts',(-3.06987042163275,3.39848901023841,388.979257997894));
#29231=CARTESIAN_POINT('Ctrl Pts',(-2.45520449449881,3.86598019246346,388.952882039408));
#29232=CARTESIAN_POINT('Ctrl Pts',(-1.76626264301101,4.15859180534764,388.926506080921));
#29233=CARTESIAN_POINT('Ctrl Pts',(-1.07732079152318,4.45120341823184,388.900130122435));
#29234=CARTESIAN_POINT('Ctrl Pts',(-0.314103015681492,4.56893546177518,
388.873754163948));
#29235=CARTESIAN_POINT('Ctrl Pts',(0.430990492327212,4.49753451605703,388.847378205461));
#29236=CARTESIAN_POINT('Ctrl Pts',(1.1760840003359,4.42613357033888,388.821002246975));
#29237=CARTESIAN_POINT('Ctrl Pts',(1.90305324051159,4.16559963535927,388.794626288488));
#29238=CARTESIAN_POINT('Ctrl Pts',(2.52388650815824,3.74747467256786,388.768250330001));
#29239=CARTESIAN_POINT('Ctrl Pts',(3.14471977580489,3.32934970977646,388.741874371515));
#29240=CARTESIAN_POINT('Ctrl Pts',(3.65941707092249,2.75363371917326,388.715498413028));
#29241=CARTESIAN_POINT('Ctrl Pts',(4.00566573453967,2.09002668660847,388.689122454542));
#29242=CARTESIAN_POINT('Ctrl Pts',(4.35191439815685,1.42641965404367,388.662746496055));
#29243=CARTESIAN_POINT('Ctrl Pts',(4.52971443027359,0.67492157951728,388.636370537568));
#29244=CARTESIAN_POINT('Ctrl Pts',(4.51754018295765,-0.0734862093441271,
388.609994579082));
#29245=CARTESIAN_POINT('Ctrl Pts',(4.50536593564171,-0.821893998205556,
388.583618620595));
#29246=CARTESIAN_POINT('Ctrl Pts',(4.30321740889306,-1.567211501402,388.557242662109));
#29247=CARTESIAN_POINT('Ctrl Pts',(3.93556804045529,-2.21920565215297,388.530866703622));
#29248=CARTESIAN_POINT('Ctrl Pts',(3.56791867201753,-2.87119980290394,388.504490745136));
#29249=CARTESIAN_POINT('Ctrl Pts',(3.03476846189066,-3.42987060120944,388.478114786649));
#29250=CARTESIAN_POINT('Ctrl Pts',(2.40066410099242,-3.8275816649429,388.451738828162));
#29251=CARTESIAN_POINT('Ctrl Pts',(1.7665597400942,-4.22529272867635,388.425362869676));
#29252=CARTESIAN_POINT('Ctrl Pts',(1.03150122842463,-4.46204405783778,388.398986911189));
#29253=CARTESIAN_POINT('Ctrl Pts',(0.284479611392651,-4.509172970546,388.372610952703));
#29254=CARTESIAN_POINT('Ctrl Pts',(-0.462542005639328,-4.55630188325423,
388.346234994216));
#29255=CARTESIAN_POINT('Ctrl Pts',(-1.22152672803371,-4.41380837950926,
388.319859035729));
#29256=CARTESIAN_POINT('Ctrl Pts',(-1.90058684505317,-4.09894366538644,
388.293483077243));
#29257=CARTESIAN_POINT('Ctrl Pts',(-2.57964696207265,-3.78407895126361,
388.267107118756));
#29258=CARTESIAN_POINT('Ctrl Pts',(-3.17878247371721,-3.29684302676292,
388.24073116027));
#29259=CARTESIAN_POINT('Ctrl Pts',(-3.62545807201282,-2.6962238956878,388.214355201783));
#29260=CARTESIAN_POINT('Ctrl Pts',(-4.07213367030842,-2.09560476461269,
388.187979243296));
#29261=CARTESIAN_POINT('Ctrl Pts',(-4.36634935525508,-1.38160242696316,
388.16160328481));
#29262=CARTESIAN_POINT('Ctrl Pts',(-4.47248542996683,-0.640658728446904,
388.135227326323));
#29263=CARTESIAN_POINT('Ctrl Pts',(-4.50285839007941,-0.428622872948985,
388.127679318379));
#29264=CARTESIAN_POINT('Ctrl Pts',(-4.51782889648961,-0.2143807013974,388.120131310436));
#29265=CARTESIAN_POINT('Ctrl Pts',(-4.51762944300479,-0.000110891096316518,
388.112583302492));
#29266=CARTESIAN_POINT('Ctrl Pts',(-4.51772665650122,0.000115440622527052,
388.387416697508));
#29267=CARTESIAN_POINT('Ctrl Pts',(-4.51715623341347,-0.566782797039444,
388.407387859296));
#29268=CARTESIAN_POINT('Ctrl Pts',(-4.41010960182223,-1.13389038388221,
388.427359021084));
#29269=CARTESIAN_POINT('Ctrl Pts',(-4.20176182131765,-1.66095369298009,
388.447330182872));
#29270=CARTESIAN_POINT('Ctrl Pts',(-3.9265964369667,-2.35704739589339,388.473706141359));
#29271=CARTESIAN_POINT('Ctrl Pts',(-3.47473607215626,-2.9832936888854,388.500082099846));
#29272=CARTESIAN_POINT('Ctrl Pts',(-2.90088593144485,-3.46387505347005,
388.526458058332));
#29273=CARTESIAN_POINT('Ctrl Pts',(-2.32703579073342,-3.94445641805472,
388.552834016819));
#29274=CARTESIAN_POINT('Ctrl Pts',(-1.631195874121,-4.27937285423203,388.579209975305));
#29275=CARTESIAN_POINT('Ctrl Pts',(-0.897609164490652,-4.42807716296015,
388.605585933792));
#29276=CARTESIAN_POINT('Ctrl Pts',(-0.164022454860301,-4.57678147168827,
388.631961892278));
#29277=CARTESIAN_POINT('Ctrl Pts',(0.607311047787985,-4.53927365296719,
388.658337850765));
#29278=CARTESIAN_POINT('Ctrl Pts',(1.32300860769931,-4.32009465142378,388.684713809252));
#29279=CARTESIAN_POINT('Ctrl Pts',(2.03870616761062,-4.10091564988038,388.711089767738));
#29280=CARTESIAN_POINT('Ctrl Pts',(2.69876778478497,-3.70006546551466,388.737465726225));
#29281=CARTESIAN_POINT('Ctrl Pts',(3.22328203392201,-3.16607367303769,388.763841684711));
#29282=CARTESIAN_POINT('Ctrl Pts',(3.74779628305905,-2.63208188056073,388.790217643198));
#29283=CARTESIAN_POINT('Ctrl Pts',(4.13676316415879,-1.96494847997252,388.816593601685));
#29284=CARTESIAN_POINT('Ctrl Pts',(4.3430917738047,-1.24544105344924,388.842969560171));
#29285=CARTESIAN_POINT('Ctrl Pts',(4.54942038345061,-0.525933626925946,
388.869345518658));
#29286=CARTESIAN_POINT('Ctrl Pts',(4.57311072164268,0.245947825532416,388.895721477144));
#29287=CARTESIAN_POINT('Ctrl Pts',(4.41129467934152,0.976754229742574,388.922097435631));
#29288=CARTESIAN_POINT('Ctrl Pts',(4.24947863704035,1.70756063395273,388.948473394118));
#29289=CARTESIAN_POINT('Ctrl Pts',(3.90215621424595,2.39729198991468,388.974849352604));
#29290=CARTESIAN_POINT('Ctrl Pts',(3.41137656079843,2.96244485750231,389.001225311091));
#29291=CARTESIAN_POINT('Ctrl Pts',(2.92059690735092,3.52759772508993,389.027601269577));
#29292=CARTESIAN_POINT('Ctrl Pts',(2.2863600232503,3.96817210430322,389.053977228064));
#29293=CARTESIAN_POINT('Ctrl Pts',(1.58545082079536,4.23082914665035,389.08035318655));
#29294=CARTESIAN_POINT('Ctrl Pts',(0.88454161834042,4.49348618899748,389.106729145037));
#29295=CARTESIAN_POINT('Ctrl Pts',(0.116960097531164,4.57822589447844,389.133105103524));
#29296=CARTESIAN_POINT('Ctrl Pts',(-0.624365245616139,4.47478911384364,
389.15948106201));
#29297=CARTESIAN_POINT('Ctrl Pts',(-1.36569058876346,4.37135233320883,389.185857020497));
#29298=CARTESIAN_POINT('Ctrl Pts',(-2.08075975424883,4.07973906645826,389.212232978983));
#29299=CARTESIAN_POINT('Ctrl Pts',(-2.6830017391303,3.63525394451758,389.23860893747));
#29300=CARTESIAN_POINT('Ctrl Pts',(-3.28524372401176,3.19076882257689,389.264984895957));
#29301=CARTESIAN_POINT('Ctrl Pts',(-3.77465852828932,2.59341184544609,389.291360854443));
#29302=CARTESIAN_POINT('Ctrl Pts',(-4.09199435856171,1.91550299994699,389.31773681293));
#29303=CARTESIAN_POINT('Ctrl Pts',(-4.37143979921575,1.3185375205331,389.340963441123));
#29304=CARTESIAN_POINT('Ctrl Pts',(-4.51744597443699,0.659107802205375,
389.364190069315));
#29305=CARTESIAN_POINT('Ctrl Pts',(-4.51800421755028,-8.27334347235434E-5,
389.387416697508));
#29306=CARTESIAN_POINT('Origin',(0.,0.,387.));
#29307=CARTESIAN_POINT('',(-4.51737568732049,-1.26367906908009E-5,390.387416697508));
#29308=CARTESIAN_POINT('',(-4.51813713037119,-8.34916185418341E-6,390.112583302492));
#29309=CARTESIAN_POINT('',(-4.51775,5.53264807684796E-16,387.));
#29310=CARTESIAN_POINT('Ctrl Pts',(-4.5181365124173,-8.33583456870006E-6,
390.112583302492));
#29311=CARTESIAN_POINT('Ctrl Pts',(-4.51805642563476,0.740544543431,390.086487647447));
#29312=CARTESIAN_POINT('Ctrl Pts',(-4.33223070178982,1.48113615227849,390.060391992403));
#29313=CARTESIAN_POINT('Ctrl Pts',(-3.98247233026486,2.13388932849751,390.034296337358));
#29314=CARTESIAN_POINT('Ctrl Pts',(-3.62895706989363,2.79365397699786,390.007920378871));
#29315=CARTESIAN_POINT('Ctrl Pts',(-3.10796852081612,3.36368304570199,389.981544420385));
#29316=CARTESIAN_POINT('Ctrl Pts',(-2.48258100282108,3.7749650451405,389.955168461898));
#29317=CARTESIAN_POINT('Ctrl Pts',(-1.85719348482602,4.18624704457905,389.928792503412));
#29318=CARTESIAN_POINT('Ctrl Pts',(-1.12740699791342,4.43878197475195,389.902416544925));
#29319=CARTESIAN_POINT('Ctrl Pts',(-0.381574321303787,4.50199628664022,
389.876040586438));
#29320=CARTESIAN_POINT('Ctrl Pts',(0.364258355305801,4.56521059852849,389.849664627952));
#29321=CARTESIAN_POINT('Ctrl Pts',(1.12613722161242,4.43910429213214,389.823288669465));
#29322=CARTESIAN_POINT('Ctrl Pts',(1.81182418267365,4.13894463102368,389.796912710979));
#29323=CARTESIAN_POINT('Ctrl Pts',(2.49751114373488,3.83878496991522,389.770536752492));
#29324=CARTESIAN_POINT('Ctrl Pts',(3.10700619955072,3.36457195409465,389.744160794005));
#29325=CARTESIAN_POINT('Ctrl Pts',(3.56651984720739,2.7737169479016,389.717784835519));
#29326=CARTESIAN_POINT('Ctrl Pts',(4.02603349486408,2.18286194170853,389.691408877032));
#29327=CARTESIAN_POINT('Ctrl Pts',(4.33556573436158,1.47536494514296,389.665032918546));
#29328=CARTESIAN_POINT('Ctrl Pts',(4.45764254540988,0.736880224291923,389.638656960059));
#29329=CARTESIAN_POINT('Ctrl Pts',(4.57971935645818,-0.0016044965591186,
389.612281001572));
#29330=CARTESIAN_POINT('Ctrl Pts',(4.51434073905728,-0.77107694169564,389.585905043086));
#29331=CARTESIAN_POINT('Ctrl Pts',(4.26942186107142,-1.47837968729494,389.559529084599));
#29332=CARTESIAN_POINT('Ctrl Pts',(4.02450298308556,-2.18568243289422,389.533153126113));
#29333=CARTESIAN_POINT('Ctrl Pts',(3.60004384451474,-2.83081547895628,389.506777167626));
#29334=CARTESIAN_POINT('Ctrl Pts',(3.04743227622566,-3.33567475174347,389.480401209139));
#29335=CARTESIAN_POINT('Ctrl Pts',(2.49482070793658,-3.84053402453067,389.454025250653));
#29336=CARTESIAN_POINT('Ctrl Pts',(1.81405670992924,-4.205119524043,389.427649292166));
#29337=CARTESIAN_POINT('Ctrl Pts',(1.08755807466189,-4.38529211818763,389.40127333368));
#29338=CARTESIAN_POINT('Ctrl Pts',(0.361059439394515,-4.56546471233226,
389.374897375193));
#29339=CARTESIAN_POINT('Ctrl Pts',(-0.411173833132874,-4.56122440110918,
389.348521416706));
#29340=CARTESIAN_POINT('Ctrl Pts',(-1.13565007507237,-4.37308454464225,
389.32214545822));
#29341=CARTESIAN_POINT('Ctrl Pts',(-1.86012631701186,-4.18494468817533,
389.295769499733));
#29342=CARTESIAN_POINT('Ctrl Pts',(-2.53684552836345,-3.81290528646455,
389.269393541247));
#29343=CARTESIAN_POINT('Ctrl Pts',(-3.08387960529535,-3.30200789030617,
389.24301758276));
#29344=CARTESIAN_POINT('Ctrl Pts',(-3.63091368222724,-2.79111049414779,
389.216641624274));
#29345=CARTESIAN_POINT('Ctrl Pts',(-4.04826262473945,-2.14135510354181,
389.190265665787));
#29346=CARTESIAN_POINT('Ctrl Pts',(-4.28539940932997,-1.43140540383048,
389.1638897073));
#29347=CARTESIAN_POINT('Ctrl Pts',(-4.43915857188131,-0.971075002245244,
389.146787572364));
#29348=CARTESIAN_POINT('Ctrl Pts',(-4.51715280146967,-0.485437663288439,
389.129685437428));
#29349=CARTESIAN_POINT('Ctrl Pts',(-4.51750342669873,8.9713446903977E-5,
389.112583302492));
#29350=CARTESIAN_POINT('Ctrl Pts',(-4.51800421755028,-8.27334347235434E-5,
389.387416697508));
#29351=CARTESIAN_POINT('Ctrl Pts',(-4.51807991049777,-0.089463280026118,
389.390566027802));
#29352=CARTESIAN_POINT('Ctrl Pts',(-4.5154815404334,-0.178839429239229,
389.393715358096));
#29353=CARTESIAN_POINT('Ctrl Pts',(-4.51017917155373,-0.268054870856108,
389.39686468839));
#29354=CARTESIAN_POINT('Ctrl Pts',(-4.46577129800614,-1.01524318229275,
389.423240646876));
#29355=CARTESIAN_POINT('Ctrl Pts',(-4.23169869464373,-1.75115909129866,
389.449616605363));
#29356=CARTESIAN_POINT('Ctrl Pts',(-3.83629973908422,-2.38670775027215,
389.475992563849));
#29357=CARTESIAN_POINT('Ctrl Pts',(-3.4409007835247,-3.02225640924567,389.502368522336));
#29358=CARTESIAN_POINT('Ctrl Pts',(-2.88417547576807,-3.55743781818676,
389.528744480823));
#29359=CARTESIAN_POINT('Ctrl Pts',(-2.23352466398677,-3.92745937581404,
389.555120439309));
#29360=CARTESIAN_POINT('Ctrl Pts',(-1.58287385220546,-4.29748093344132,
389.581496397796));
#29361=CARTESIAN_POINT('Ctrl Pts',(-0.838297536399466,-4.50234263975477,
389.607872356282));
#29362=CARTESIAN_POINT('Ctrl Pts',(-0.0899390503012636,-4.51724258154659,
389.634248314769));
#29363=CARTESIAN_POINT('Ctrl Pts',(0.658419435796918,-4.53214252333841,
389.660624273256));
#29364=CARTESIAN_POINT('Ctrl Pts',(1.4105600921873,-4.3570807006086,389.687000231742));
#29365=CARTESIAN_POINT('Ctrl Pts',(2.07542379603256,-4.01325125554937,389.713376190229));
#29366=CARTESIAN_POINT('Ctrl Pts',(2.74028749987779,-3.66942181049016,389.739752148715));
#29367=CARTESIAN_POINT('Ctrl Pts',(3.31787425117789,-3.15682474310154,389.766128107202));
#29368=CARTESIAN_POINT('Ctrl Pts',(3.7382575774187,-2.53751844489424,389.792504065688));
#29369=CARTESIAN_POINT('Ctrl Pts',(4.15864090365956,-1.91821214668688,389.818880024175));
#29370=CARTESIAN_POINT('Ctrl Pts',(4.4218208048411,-1.19219661766082,389.845255982662));
#29371=CARTESIAN_POINT('Ctrl Pts',(4.4959349813437,-0.447368099932093,389.871631941148));
#29372=CARTESIAN_POINT('Ctrl Pts',(4.5700491578463,0.297460417796599,389.898007899635));
#29373=CARTESIAN_POINT('Ctrl Pts',(4.45509760966997,1.06110192422797,389.924383858122));
#29374=CARTESIAN_POINT('Ctrl Pts',(4.16499713157485,1.7511049275472,389.950759816608));
#29375=CARTESIAN_POINT('Ctrl Pts',(3.87489665347973,2.44110793086643,389.977135775095));
#29376=CARTESIAN_POINT('Ctrl Pts',(3.40964724546582,3.05747243107353,390.003511733581));
#29377=CARTESIAN_POINT('Ctrl Pts',(2.8255750782226,3.52557726487935,390.029887692068));
#29378=CARTESIAN_POINT('Ctrl Pts',(2.24150291097938,3.99368209868516,390.056263650554));
#29379=CARTESIAN_POINT('Ctrl Pts',(1.53860798450686,4.31352726608968,390.082639609041));
#29380=CARTESIAN_POINT('Ctrl Pts',(0.80198740784653,4.44639019553642,390.109015567528));
#29381=CARTESIAN_POINT('Ctrl Pts',(0.0653668311861832,4.57925312498317,
390.135391526014));
#29382=CARTESIAN_POINT('Ctrl Pts',(-0.704979395661959,4.52513381647212,
390.161767484501));
#29383=CARTESIAN_POINT('Ctrl Pts',(-1.41578806308163,4.2905843114595,390.188143442987));
#29384=CARTESIAN_POINT('Ctrl Pts',(-2.1265967305013,4.05603480644688,390.214519401474));
#29385=CARTESIAN_POINT('Ctrl Pts',(-2.7778678384925,3.64105510493269,390.240895359961));
#29386=CARTESIAN_POINT('Ctrl Pts',(-3.2907541989407,3.09588539443257,390.267271318447));
#29387=CARTESIAN_POINT('Ctrl Pts',(-3.8036405593889,2.55071568393247,390.293647276934));
#29388=CARTESIAN_POINT('Ctrl Pts',(-4.17814217229411,1.87535596444644,390.320023235421));
#29389=CARTESIAN_POINT('Ctrl Pts',(-4.36891939528681,1.15156975072878,390.346399193907));
#29390=CARTESIAN_POINT('Ctrl Pts',(-4.46781255254173,0.776380811874881,
390.360071695107));
#29391=CARTESIAN_POINT('Ctrl Pts',(-4.51733762799004,0.388179321285348,
390.373744196308));
#29392=CARTESIAN_POINT('Ctrl Pts',(-4.51737568732049,-1.26367906908009E-5,
390.387416697508));
#29393=CARTESIAN_POINT('Origin',(0.,0.,387.));
#29394=CARTESIAN_POINT('',(-4.51792755410097,9.93894350090341E-5,391.387416697508));
#29395=CARTESIAN_POINT('',(-4.51747010126728,-7.96701847477171E-5,391.112583302492));
#29396=CARTESIAN_POINT('',(-4.51775,5.53264807684796E-16,387.));
#29397=CARTESIAN_POINT('Ctrl Pts',(-4.51747010126728,-7.96701847477171E-5,
391.112583302492));
#29398=CARTESIAN_POINT('Ctrl Pts',(-4.51717195077355,0.469542077919004,
391.09604177444));
#29399=CARTESIAN_POINT('Ctrl Pts',(-4.44429158523714,0.939254240738123,
391.079500246387));
#29400=CARTESIAN_POINT('Ctrl Pts',(-4.30028579839415,1.38604169480228,391.062958718335));
#29401=CARTESIAN_POINT('Ctrl Pts',(-4.07066428800006,2.09845757944446,391.036582759848));
#29402=CARTESIAN_POINT('Ctrl Pts',(-3.66020460842122,2.75258681658163,391.010206801362));
#29403=CARTESIAN_POINT('Ctrl Pts',(-3.11859972342044,3.26923619408001,390.983830842875));
#29404=CARTESIAN_POINT('Ctrl Pts',(-2.57699483841966,3.78588557157838,390.957454884389));
#29405=CARTESIAN_POINT('Ctrl Pts',(-1.90424474799695,4.16505508943795,390.931078925902));
#29406=CARTESIAN_POINT('Ctrl Pts',(-1.181797027951,4.36083997783993,390.904702967415));
#29407=CARTESIAN_POINT('Ctrl Pts',(-0.459349307905077,4.55662486624191,
390.878327008929));
#29408=CARTESIAN_POINT('Ctrl Pts',(0.312796041764081,4.5690251251863,390.851951050442));
#29409=CARTESIAN_POINT('Ctrl Pts',(1.04115799773134,4.39653949730477,390.825575091955));
#29410=CARTESIAN_POINT('Ctrl Pts',(1.76951995369859,4.22405386942324,390.799199133469));
#29411=CARTESIAN_POINT('Ctrl Pts',(2.45409851596394,3.86668235471579,390.772823174982));
#29412=CARTESIAN_POINT('Ctrl Pts',(3.01201407568894,3.36769071255846,390.746447216496));
#29413=CARTESIAN_POINT('Ctrl Pts',(3.56992963541394,2.86869907040112,390.720071258009));
#29414=CARTESIAN_POINT('Ctrl Pts',(4.00118219259857,2.22808730079389,390.693695299523));
#29415=CARTESIAN_POINT('Ctrl Pts',(4.25356146018424,1.52341210184117,390.667319341036));
#29416=CARTESIAN_POINT('Ctrl Pts',(4.5059407277699,0.818736902888453,390.640943382549));
#29417=CARTESIAN_POINT('Ctrl Pts',(4.5794467057566,0.0499982745902433,390.614567424063));
#29418=CARTESIAN_POINT('Ctrl Pts',(4.46518027424979,-0.68973519995098,390.588191465576));
#29419=CARTESIAN_POINT('Ctrl Pts',(4.35091384274297,-1.42946867449225,390.56181550709));
#29420=CARTESIAN_POINT('Ctrl Pts',(4.04887500174263,-2.14019699527652,390.535439548603));
#29421=CARTESIAN_POINT('Ctrl Pts',(3.59563057115222,-2.73587469073354,390.509063590117));
#29422=CARTESIAN_POINT('Ctrl Pts',(3.14238614056185,-3.33155238619052,390.48268763163));
#29423=CARTESIAN_POINT('Ctrl Pts',(2.53793612038144,-3.81217945632025,390.456311673143));
#29424=CARTESIAN_POINT('Ctrl Pts',(1.85545922814075,-4.11956800894318,390.429935714657));
#29425=CARTESIAN_POINT('Ctrl Pts',(1.17298233590006,-4.42695656156612,390.40355975617));
#29426=CARTESIAN_POINT('Ctrl Pts',(0.412478571599103,-4.56110659668227,
390.377183797684));
#29427=CARTESIAN_POINT('Ctrl Pts',(-0.333980448764015,-4.50577702371569,
390.350807839197));
#29428=CARTESIAN_POINT('Ctrl Pts',(-1.08043946912713,-4.45044745074911,
390.32443188071));
#29429=CARTESIAN_POINT('Ctrl Pts',(-1.81285374555241,-4.2056382696998,390.298055922224));
#29430=CARTESIAN_POINT('Ctrl Pts',(-2.44255236123965,-3.80098769929651,
390.271679963737));
#29431=CARTESIAN_POINT('Ctrl Pts',(-3.07225097692695,-3.39633712889319,
390.245304005251));
#29432=CARTESIAN_POINT('Ctrl Pts',(-3.59923393187618,-2.83184516913586,
390.218928046764));
#29433=CARTESIAN_POINT('Ctrl Pts',(-3.95970118387424,-2.17585295046006,
390.192552088277));
#29434=CARTESIAN_POINT('Ctrl Pts',(-4.32016843587225,-1.51986073178434,
390.166176129791));
#29435=CARTESIAN_POINT('Ctrl Pts',(-4.51411998491911,-0.772368254190162,
390.139800171304));
#29436=CARTESIAN_POINT('Ctrl Pts',(-4.51807477361008,-0.0238719012447998,
390.113424212818));
#29437=CARTESIAN_POINT('Ctrl Pts',(-4.51811680206878,-0.0159174565147239,
390.113143909376));
#29438=CARTESIAN_POINT('Ctrl Pts',(-4.51813737266016,-0.00796289840890401,
390.112863605934));
#29439=CARTESIAN_POINT('Ctrl Pts',(-4.5181365124173,-8.33583456870006E-6,
390.112583302492));
#29440=CARTESIAN_POINT('Ctrl Pts',(-4.51737568732049,-1.26367906908009E-5,
390.387416697508));
#29441=CARTESIAN_POINT('Ctrl Pts',(-4.51741104918088,-0.360691336761726,
390.400120154794));
#29442=CARTESIAN_POINT('Ctrl Pts',(-4.47472562929359,-0.721361807575693,
390.412823612081));
#29443=CARTESIAN_POINT('Ctrl Pts',(-4.38922403190431,-1.07157919495506,
390.425527069367));
#29444=CARTESIAN_POINT('Ctrl Pts',(-4.2116986124489,-1.79872921897196,390.451903027853));
#29445=CARTESIAN_POINT('Ctrl Pts',(-3.84959494045787,-2.48081655905642,
390.47827898634));
#29446=CARTESIAN_POINT('Ctrl Pts',(-3.3467516815685,-3.03526321020521,390.504654944827));
#29447=CARTESIAN_POINT('Ctrl Pts',(-2.84390842267912,-3.589709861354,390.531030903313));
#29448=CARTESIAN_POINT('Ctrl Pts',(-2.2003255768914,-4.01651582356711,390.5574068618));
#29449=CARTESIAN_POINT('Ctrl Pts',(-1.49391954044408,-4.26400914398482,
390.583782820286));
#29450=CARTESIAN_POINT('Ctrl Pts',(-0.787513503996787,-4.51150246440253,
390.610158778773));
#29451=CARTESIAN_POINT('Ctrl Pts',(-0.018284276889904,-4.57968314302485,
390.636534737259));
#29452=CARTESIAN_POINT('Ctrl Pts',(0.720640162637278,-4.46029677592208,
390.662910695746));
#29453=CARTESIAN_POINT('Ctrl Pts',(1.45956460216448,-4.34091040881931,390.689286654233));
#29454=CARTESIAN_POINT('Ctrl Pts',(2.16818425411199,-4.03395699599143,390.715662612719));
#29455=CARTESIAN_POINT('Ctrl Pts',(2.76070893630653,-3.57659834791441,390.742038571206));
#29456=CARTESIAN_POINT('Ctrl Pts',(3.35323361850104,-3.11923969983741,390.768414529692));
#29457=CARTESIAN_POINT('Ctrl Pts',(3.8296633309426,-2.51147581651127,390.794790488179));
#29458=CARTESIAN_POINT('Ctrl Pts',(4.13231834133649,-1.82688661365747,390.821166446666));
#29459=CARTESIAN_POINT('Ctrl Pts',(4.43497335173039,-1.14229741080364,390.847542405152));
#29460=CARTESIAN_POINT('Ctrl Pts',(4.5638536600766,-0.380882888422163,390.873918363639));
#29461=CARTESIAN_POINT('Ctrl Pts',(4.50335616377816,0.365175075091525,390.900294322126));
#29462=CARTESIAN_POINT('Ctrl Pts',(4.44285866747971,1.11123303860522,390.926670280612));
#29463=CARTESIAN_POINT('Ctrl Pts',(4.1929833665366,1.84193444325112,390.953046239099));
#29464=CARTESIAN_POINT('Ctrl Pts',(3.78398181766136,2.46881574381626,390.979422197585));
#29465=CARTESIAN_POINT('Ctrl Pts',(3.37498026878612,3.0956970443814,391.005798156072));
#29466=CARTESIAN_POINT('Ctrl Pts',(2.80685247197875,3.61875824086581,391.032174114558));
#29467=CARTESIAN_POINT('Ctrl Pts',(2.14837973615702,3.97467408507625,391.058550073045));
#29468=CARTESIAN_POINT('Ctrl Pts',(1.48990700033531,4.33058992928668,391.084926031532));
#29469=CARTESIAN_POINT('Ctrl Pts',(0.74108932549923,4.51936042122317,391.111301990018));
#29470=CARTESIAN_POINT('Ctrl Pts',(-0.00741646764041988,4.51813175652443,
391.137677948505));
#29471=CARTESIAN_POINT('Ctrl Pts',(-0.75592226078007,4.51690309182569,391.164053906991));
#29472=CARTESIAN_POINT('Ctrl Pts',(-1.5041161722233,4.32567527049173,391.190429865478));
#29473=CARTESIAN_POINT('Ctrl Pts',(-2.16141689818149,3.96759959743449,391.216805823964));
#29474=CARTESIAN_POINT('Ctrl Pts',(-2.81871762413969,3.60952392437724,391.243181782451));
#29475=CARTESIAN_POINT('Ctrl Pts',(-3.38512516461286,3.0846003995967,391.269557740938));
#29476=CARTESIAN_POINT('Ctrl Pts',(-3.79206647629354,2.45637973706784,391.295933699424));
#29477=CARTESIAN_POINT('Ctrl Pts',(-4.19900778797422,1.82815907453898,391.322309657911));
#29478=CARTESIAN_POINT('Ctrl Pts',(-4.44648287086241,1.0966412742618,391.348685616397));
#29479=CARTESIAN_POINT('Ctrl Pts',(-4.50453075451936,0.350388719704337,
391.375061574884));
#29480=CARTESIAN_POINT('Ctrl Pts',(-4.51359442160846,0.233867939052437,
391.379179949092));
#29481=CARTESIAN_POINT('Ctrl Pts',(-4.51803983860459,0.116987923926286,
391.3832983233));
#29482=CARTESIAN_POINT('Ctrl Pts',(-4.51792755410097,9.93894350090341E-5,
391.387416697508));
#29483=CARTESIAN_POINT('Origin',(0.,0.,387.));
#29484=CARTESIAN_POINT('',(-4.51781275651133,-0.000112770352403077,392.387416697508));
#29485=CARTESIAN_POINT('',(-4.51767617872592,0.000114137193723671,392.112583302492));
#29486=CARTESIAN_POINT('',(-4.51775,5.53264807684796E-16,387.));
#29487=CARTESIAN_POINT('Ctrl Pts',(-4.51767617872592,0.000114137193723671,
392.112583302492));
#29488=CARTESIAN_POINT('Ctrl Pts',(-4.5178695555558,0.198463769522385,392.105595901432));
#29489=CARTESIAN_POINT('Ctrl Pts',(-4.5050469141142,0.396788584023774,392.098608500372));
#29490=CARTESIAN_POINT('Ctrl Pts',(-4.47900555811224,0.593362231693622,
392.091621099312));
#29491=CARTESIAN_POINT('Ctrl Pts',(-4.38070495693752,1.33538610094233,392.065245140825));
#29492=CARTESIAN_POINT('Ctrl Pts',(-4.0940505572316,2.05245754966054,392.038869182339));
#29493=CARTESIAN_POINT('Ctrl Pts',(-3.65374663667568,2.65776316525419,392.012493223852));
#29494=CARTESIAN_POINT('Ctrl Pts',(-3.21344271611974,3.26306878084786,391.986117265366));
#29495=CARTESIAN_POINT('Ctrl Pts',(-2.61948927471379,3.75660856331697,391.959741306879));
#29496=CARTESIAN_POINT('Ctrl Pts',(-1.94379424473237,4.07863132211605,391.933365348393));
#29497=CARTESIAN_POINT('Ctrl Pts',(-1.26809921475095,4.40065408091513,391.906989389906));
#29498=CARTESIAN_POINT('Ctrl Pts',(-0.510662596194056,4.55115981604418,
391.88061343142));
#29499=CARTESIAN_POINT('Ctrl Pts',(0.236815323891349,4.51192730770023,391.854237472933));
#29500=CARTESIAN_POINT('Ctrl Pts',(0.984293243976733,4.47269479935628,391.827861514446));
#29501=CARTESIAN_POINT('Ctrl Pts',(1.72181246559064,4.24372404753933,391.80148555596));
#29502=CARTESIAN_POINT('Ctrl Pts',(2.36008403350207,3.85273576597324,391.775109597473));
#29503=CARTESIAN_POINT('Ctrl Pts',(2.99835560141351,3.46174748440714,391.748733638986));
#29504=CARTESIAN_POINT('Ctrl Pts',(3.53737951562248,2.90874167309189,391.7223576805));
#29505=CARTESIAN_POINT('Ctrl Pts',(3.9118979757439,2.2606688733584,391.695981722013));
#29506=CARTESIAN_POINT('Ctrl Pts',(4.28641643586534,1.6125960736249,391.669605763527));
#29507=CARTESIAN_POINT('Ctrl Pts',(4.49642944189922,0.869456285473188,391.64322980504));
#29508=CARTESIAN_POINT('Ctrl Pts',(4.51651143022073,0.121218927096046,391.616853846553));
#29509=CARTESIAN_POINT('Ctrl Pts',(4.53659341854224,-0.627018431281127,
391.590477888067));
#29510=CARTESIAN_POINT('Ctrl Pts',(4.36674438915135,-1.3803533598837,391.56410192958));
#29511=CARTESIAN_POINT('Ctrl Pts',(4.02752738899906,-2.04758214938088,391.537725971094));
#29512=CARTESIAN_POINT('Ctrl Pts',(3.68831038884679,-2.71481093887802,391.511350012607));
#29513=CARTESIAN_POINT('Ctrl Pts',(3.17972541793314,-3.29593358926979,391.48497405412));
#29514=CARTESIAN_POINT('Ctrl Pts',(2.56334513683187,-3.72059554871007,391.458598095634));
#29515=CARTESIAN_POINT('Ctrl Pts',(1.94696485573061,-4.14525750815035,391.432222137147));
#29516=CARTESIAN_POINT('Ctrl Pts',(1.22278926444172,-4.41345877663913,391.405846178661));
#29517=CARTESIAN_POINT('Ctrl Pts',(0.478491850048684,-4.49272913461715,
391.379470220174));
#29518=CARTESIAN_POINT('Ctrl Pts',(-0.265805564344378,-4.57199949259517,
391.353094261688));
#29519=CARTESIAN_POINT('Ctrl Pts',(-1.03022480184161,-4.46233894006242,
391.326718303201));
#29520=CARTESIAN_POINT('Ctrl Pts',(-1.72222021336115,-4.17702370884953,
391.300342344714));
#29521=CARTESIAN_POINT('Ctrl Pts',(-2.41421562488067,-3.89170847763665,
391.273966386228));
#29522=CARTESIAN_POINT('Ctrl Pts',(-3.03378721042251,-3.43073856774365,
391.247590427741));
#29523=CARTESIAN_POINT('Ctrl Pts',(-3.50592553573386,-2.84992204551108,
391.221214469255));
#29524=CARTESIAN_POINT('Ctrl Pts',(-3.97806386104521,-2.26910552327851,
391.194838510768));
#29525=CARTESIAN_POINT('Ctrl Pts',(-4.30276892612607,-1.56844238870636,
391.168462552281));
#29526=CARTESIAN_POINT('Ctrl Pts',(-4.44072978806182,-0.83275955534669,
391.142086593795));
#29527=CARTESIAN_POINT('Ctrl Pts',(-4.4921693025746,-0.558455906816085,
391.13225216336));
#29528=CARTESIAN_POINT('Ctrl Pts',(-4.51764736060392,-0.279283767746957,
391.122417732926));
#29529=CARTESIAN_POINT('Ctrl Pts',(-4.51747010126728,-7.96701847477171E-5,
391.112583302492));
#29530=CARTESIAN_POINT('Ctrl Pts',(-4.51792755410097,9.93894350090341E-5,
391.387416697508));
#29531=CARTESIAN_POINT('Ctrl Pts',(-4.51732071711229,-0.631619894993005,
391.409674281787));
#29532=CARTESIAN_POINT('Ctrl Pts',(-4.38359173091614,-1.26358801454013,
391.431931866065));
#29533=CARTESIAN_POINT('Ctrl Pts',(-4.12629845673798,-1.84044304971073,
391.454189450344));
#29534=CARTESIAN_POINT('Ctrl Pts',(-3.82139759087395,-2.52403495573063,
391.48056540883));
#29535=CARTESIAN_POINT('Ctrl Pts',(-3.34297517472017,-3.13023145893271,
391.506941367317));
#29536=CARTESIAN_POINT('Ctrl Pts',(-2.74895219046335,-3.58564240100063,
391.533317325804));
#29537=CARTESIAN_POINT('Ctrl Pts',(-2.15492920620652,-4.04105334306855,
391.55969328429));
#29538=CARTESIAN_POINT('Ctrl Pts',(-1.44530565384664,-4.34567872400231,
391.586069242777));
#29539=CARTESIAN_POINT('Ctrl Pts',(-0.705993254381129,-4.46263858026562,
391.612445201263));
#29540=CARTESIAN_POINT('Ctrl Pts',(0.0333191450843864,-4.57959843652893,
391.63882115975));
#29541=CARTESIAN_POINT('Ctrl Pts',(0.802320391655539,-4.5088927681218,391.665197118237));
#29542=CARTESIAN_POINT('Ctrl Pts',(1.50791010792466,-4.25908167093864,391.691573076723));
#29543=CARTESIAN_POINT('Ctrl Pts',(2.21349982419377,-4.00927057375548,391.71794903521));
#29544=CARTESIAN_POINT('Ctrl Pts',(2.85567801016084,-3.58035404779628,391.744324993696));
#29545=CARTESIAN_POINT('Ctrl Pts',(3.35669832699602,-3.02425956472802,391.770700952183));
#29546=CARTESIAN_POINT('Ctrl Pts',(3.85771864383119,-2.46816508165977,391.79707691067));
#29547=CARTESIAN_POINT('Ctrl Pts',(4.21758109153447,-1.78489264148247,391.823452869156));
#29548=CARTESIAN_POINT('Ctrl Pts',(4.39271834190528,-1.05716372525534,391.849828827643));
#29549=CARTESIAN_POINT('Ctrl Pts',(4.56785559227609,-0.329434809028198,
391.876204786129));
#29550=CARTESIAN_POINT('Ctrl Pts',(4.55826764531442,0.442750583248765,391.902580744616));
#29551=CARTESIAN_POINT('Ctrl Pts',(4.36511528129817,1.16590658042746,391.928956703102));
#29552=CARTESIAN_POINT('Ctrl Pts',(4.17196291728192,1.88906257760614,391.955332661589));
#29553=CARTESIAN_POINT('Ctrl Pts',(3.79524613621108,2.56318917968655,391.981708620076));
#29554=CARTESIAN_POINT('Ctrl Pts',(3.28057276336538,3.10667216126389,392.008084578562));
#29555=CARTESIAN_POINT('Ctrl Pts',(2.76589939051967,3.65015514284124,392.034460537049));
#29556=CARTESIAN_POINT('Ctrl Pts',(2.11326942589908,4.0629945039155,392.060836495535));
#29557=CARTESIAN_POINT('Ctrl Pts',(1.40169456978973,4.29520918074182,392.087212454022));
#29558=CARTESIAN_POINT('Ctrl Pts',(0.690119713680387,4.52742385756813,392.113588412509));
#29559=CARTESIAN_POINT('Ctrl Pts',(-0.0804000339177079,4.57901385014649,
392.139964370995));
#29560=CARTESIAN_POINT('Ctrl Pts',(-0.816580455818562,4.44373333273746,
392.166340329482));
#29561=CARTESIAN_POINT('Ctrl Pts',(-1.55276087771942,4.30845281532842,392.192716287968));
#29562=CARTESIAN_POINT('Ctrl Pts',(-2.25460197392303,3.98630178793199,392.219092246455));
#29563=CARTESIAN_POINT('Ctrl Pts',(-2.83713421905071,3.51628198476719,392.245468204942));
#29564=CARTESIAN_POINT('Ctrl Pts',(-3.4196664641784,3.0462621816024,392.271844163428));
#29565=CARTESIAN_POINT('Ctrl Pts',(-3.88288985823016,2.42837360266924,392.298220121915));
#29566=CARTESIAN_POINT('Ctrl Pts',(-4.17072351316767,1.73742192630838,392.324596080401));
#29567=CARTESIAN_POINT('Ctrl Pts',(-4.3992382776818,1.18886668648237,392.345536286104));
#29568=CARTESIAN_POINT('Ctrl Pts',(-4.51720537865769,0.59425998006379,392.366476491806));
#29569=CARTESIAN_POINT('Ctrl Pts',(-4.51781275651133,-0.000112770352403077,
392.387416697508));
#29570=CARTESIAN_POINT('Origin',(0.,0.,387.));
#29571=CARTESIAN_POINT('',(-4.51740214664894,4.58334405226135E-5,393.387416697508));
#29572=CARTESIAN_POINT('',(-4.51804470017939,-7.02313581118758E-5,393.112583302492));
#29573=CARTESIAN_POINT('',(-4.51775,5.53264807684796E-16,387.));
#29574=CARTESIAN_POINT('Ctrl Pts',(-4.51804470017939,-7.02313581118758E-5,
393.112583302492));
#29575=CARTESIAN_POINT('Ctrl Pts',(-4.51753951069973,0.675637543377085,
393.088774069938));
#29576=CARTESIAN_POINT('Ctrl Pts',(-4.36387000533556,1.351567384844,393.064964837384));
#29577=CARTESIAN_POINT('Ctrl Pts',(-4.07071229568028,1.96032419089247,393.04115560483));
#29578=CARTESIAN_POINT('Ctrl Pts',(-3.74595106860983,2.63470729871608,393.014779646343));
#29579=CARTESIAN_POINT('Ctrl Pts',(-3.25000583346633,3.2266536908633,392.988403687856));
#29580=CARTESIAN_POINT('Ctrl Pts',(-2.64291900080672,3.66449842171826,392.96202772937));
#29581=CARTESIAN_POINT('Ctrl Pts',(-2.03583216814709,4.10234315257323,392.935651770883));
#29582=CARTESIAN_POINT('Ctrl Pts',(-1.31760373797134,4.38608622213596,392.909275812397));
#29583=CARTESIAN_POINT('Ctrl Pts',(-0.575187194701503,4.48137581760917,
392.88289985391));
#29584=CARTESIAN_POINT('Ctrl Pts',(0.167229348568301,4.57666541308236,392.856523895423));
#29585=CARTESIAN_POINT('Ctrl Pts',(0.933834004932164,4.48350153446603,392.830147936937));
#29586=CARTESIAN_POINT('Ctrl Pts',(1.63181654404497,4.21316321713056,392.80377197845));
#29587=CARTESIAN_POINT('Ctrl Pts',(2.32979908315777,3.94282489979509,392.777396019963));
#29588=CARTESIAN_POINT('Ctrl Pts',(2.95915950501951,3.49531214374047,392.751020061477));
#29589=CARTESIAN_POINT('Ctrl Pts',(3.44370327410501,2.92480380325231,392.72464410299));
#29590=CARTESIAN_POINT('Ctrl Pts',(3.92824704319053,2.35429546276414,392.698268144504));
#29591=CARTESIAN_POINT('Ctrl Pts',(4.26797415949979,1.66079153784243,392.671892186017));
#29592=CARTESIAN_POINT('Ctrl Pts',(4.42175501123433,0.928252200764915,392.64551622753));
#29593=CARTESIAN_POINT('Ctrl Pts',(4.57553586296886,0.195712863687411,392.619140269044));
#29594=CARTESIAN_POINT('Ctrl Pts',(4.54337045012868,-0.575861885545891,
392.592764310557));
#29595=CARTESIAN_POINT('Ctrl Pts',(4.32915293034778,-1.29306010427281,392.566388352071));
#29596=CARTESIAN_POINT('Ctrl Pts',(4.11493541056688,-2.01025832299973,392.540012393584));
#29597=CARTESIAN_POINT('Ctrl Pts',(3.71866578384527,-2.67308001122027,392.513636435098));
#29598=CARTESIAN_POINT('Ctrl Pts',(3.18831907228789,-3.20127959117695,392.487260476611));
#29599=CARTESIAN_POINT('Ctrl Pts',(2.65797236073051,-3.72947917113363,392.460884518124));
#29600=CARTESIAN_POINT('Ctrl Pts',(1.99354856433737,-4.12305664282645,392.434508559638));
#29601=CARTESIAN_POINT('Ctrl Pts',(1.27548722267832,-4.33436291424531,392.408132601151));
#29602=CARTESIAN_POINT('Ctrl Pts',(0.557425881019256,-4.54566918566418,
392.381756642665));
#29603=CARTESIAN_POINT('Ctrl Pts',(-0.214273005905716,-4.57470425680908,
392.355380684178));
#29604=CARTESIAN_POINT('Ctrl Pts',(-0.946182466504358,-4.41795294991702,
392.329004725691));
#29605=CARTESIAN_POINT('Ctrl Pts',(-1.678091927103,-4.26120164302497,392.302628767205));
#29606=CARTESIAN_POINT('Ctrl Pts',(-2.37021196137532,-3.91866395809597,
392.276252808718));
#29607=CARTESIAN_POINT('Ctrl Pts',(-2.93874993999921,-3.43180977295588,
392.249876850232));
#29608=CARTESIAN_POINT('Ctrl Pts',(-3.50728791862308,-2.9449555878158,392.223500891745));
#29609=CARTESIAN_POINT('Ctrl Pts',(-3.95224384159854,-2.31378490246464,
392.197124933258));
#29610=CARTESIAN_POINT('Ctrl Pts',(-4.21974840176451,-1.61471141489946,
392.170748974772));
#29611=CARTESIAN_POINT('Ctrl Pts',(-4.41638684920909,-1.1008333518145,392.151360417345));
#29612=CARTESIAN_POINT('Ctrl Pts',(-4.51713959899635,-0.550264065511563,
392.131971859919));
#29613=CARTESIAN_POINT('Ctrl Pts',(-4.51767617872592,0.000114137193723671,
392.112583302492));
#29614=CARTESIAN_POINT('Ctrl Pts',(-4.51781275651133,-0.000112770352403077,
392.387416697508));
#29615=CARTESIAN_POINT('Ctrl Pts',(-4.51797042238654,-0.154402722371687,
392.392852450292));
#29616=CARTESIAN_POINT('Ctrl Pts',(-4.51021990758361,-0.308676909473601,
392.398288203077));
#29617=CARTESIAN_POINT('Ctrl Pts',(-4.49444205643657,-0.462125713027313,
392.403723955861));
#29618=CARTESIAN_POINT('Ctrl Pts',(-4.41788302894468,-1.20670690221361,
392.430099914348));
#29619=CARTESIAN_POINT('Ctrl Pts',(-4.15232105813761,-1.93185450679764,
392.456475872834));
#29620=CARTESIAN_POINT('Ctrl Pts',(-3.72990683273987,-2.54977736133712,
392.482851831321));
#29621=CARTESIAN_POINT('Ctrl Pts',(-3.30749260734213,-3.16770021587658,
392.509227789807));
#29622=CARTESIAN_POINT('Ctrl Pts',(-2.72822612735372,-3.67839832037151,
392.535603748294));
#29623=CARTESIAN_POINT('Ctrl Pts',(-2.06223722435424,-4.02004318431961,
392.561979706781));
#29624=CARTESIAN_POINT('Ctrl Pts',(-1.39624832135474,-4.36168804826772,
392.588355665267));
#29625=CARTESIAN_POINT('Ctrl Pts',(-0.643536995344169,-4.53427967166901,
392.614731623754));
#29626=CARTESIAN_POINT('Ctrl Pts',(0.10476854180126,-4.5169229710009,392.64110758224));
#29627=CARTESIAN_POINT('Ctrl Pts',(0.853074078946657,-4.4995662703328,392.667483540727));
#29628=CARTESIAN_POINT('Ctrl Pts',(1.59697382722691,-4.29226124559533,392.693859499214));
#29629=CARTESIAN_POINT('Ctrl Pts',(2.24640636264933,-3.92010561428585,392.7202354577));
#29630=CARTESIAN_POINT('Ctrl Pts',(2.89583889807178,-3.54794998297635,392.746611416187));
#29631=CARTESIAN_POINT('Ctrl Pts',(3.45080422063637,-3.01094374509482,392.772987374673));
#29632=CARTESIAN_POINT('Ctrl Pts',(3.84411455761933,-2.37410042778438,392.79936333316));
#29633=CARTESIAN_POINT('Ctrl Pts',(4.23742489460227,-1.73725711047397,392.825739291647));
#29634=CARTESIAN_POINT('Ctrl Pts',(4.46908024600357,-1.00057671373466,392.852115250133));
#29635=CARTESIAN_POINT('Ctrl Pts',(4.51103488271665,-0.253246639109774,
392.87849120862));
#29636=CARTESIAN_POINT('Ctrl Pts',(4.55298951942973,0.494083435515108,392.904867167106));
#29637=CARTESIAN_POINT('Ctrl Pts',(4.40524344145459,1.25206318802556,392.931243125593));
#29638=CARTESIAN_POINT('Ctrl Pts',(4.0856837662456,1.92892657598571,392.95761908408));
#29639=CARTESIAN_POINT('Ctrl Pts',(3.76612409103661,2.60578996394588,392.983995042566));
#29640=CARTESIAN_POINT('Ctrl Pts',(3.27475081859377,3.20153698735573,393.010371001053));
#29641=CARTESIAN_POINT('Ctrl Pts',(2.67105284742856,3.64404257103983,393.03674695954));
#29642=CARTESIAN_POINT('Ctrl Pts',(2.06735487626337,4.08654815472391,393.063122918026));
#29643=CARTESIAN_POINT('Ctrl Pts',(1.35133220637582,4.37581229868225,393.089498876512));
#29644=CARTESIAN_POINT('Ctrl Pts',(0.60967127825766,4.4768147723325,393.115874834999));
#29645=CARTESIAN_POINT('Ctrl Pts',(-0.131989649860521,4.57781724598275,
393.142250793486));
#29646=CARTESIAN_POINT('Ctrl Pts',(-0.89928883620931,4.49055804932491,393.168626751973));
#29647=CARTESIAN_POINT('Ctrl Pts',(-1.5993319660497,4.2256013578754,393.195002710459));
#29648=CARTESIAN_POINT('Ctrl Pts',(-2.29937509589006,3.9606446664259,393.221378668946));
#29649=CARTESIAN_POINT('Ctrl Pts',(-2.93216216922203,3.51799048018475,393.247754627432));
#29650=CARTESIAN_POINT('Ctrl Pts',(-3.42108379742811,2.95122944283932,393.274130585919));
#29651=CARTESIAN_POINT('Ctrl Pts',(-3.91000542563421,2.38446840549387,393.300506544405));
#29652=CARTESIAN_POINT('Ctrl Pts',(-4.25506160871441,1.69360051704413,393.326882502892));
#29653=CARTESIAN_POINT('Ctrl Pts',(-4.41447756279827,0.962266813756684,
393.353258461379));
#29654=CARTESIAN_POINT('Ctrl Pts',(-4.4832948761755,0.646561770734553,393.364644540088));
#29655=CARTESIAN_POINT('Ctrl Pts',(-4.51751793652066,0.323315880315216,
393.376030618798));
#29656=CARTESIAN_POINT('Ctrl Pts',(-4.51740214664894,4.58334405226135E-5,
393.387416697508));
#29657=CARTESIAN_POINT('Origin',(0.,0.,387.));
#29658=CARTESIAN_POINT('',(-4.51808751818987,5.21912322906659E-5,394.387416697508));
#29659=CARTESIAN_POINT('',(-4.5173836733729,-2.76243915998559E-5,394.112583302492));
#29660=CARTESIAN_POINT('',(-4.51775,5.53264807684796E-16,387.));
#29661=CARTESIAN_POINT('Ctrl Pts',(-4.5173836733729,-2.76243915998559E-5,
394.112583302492));
#29662=CARTESIAN_POINT('Ctrl Pts',(-4.51729674156455,0.40470368583773,394.09832819693));
#29663=CARTESIAN_POINT('Ctrl Pts',(-4.46340651421681,0.809457698610517,
394.084073091368));
#29664=CARTESIAN_POINT('Ctrl Pts',(-4.35600985269673,1.19947809100869,394.069817985807));
#29665=CARTESIAN_POINT('Ctrl Pts',(-4.15729579382325,1.92112561822137,394.04344202732));
#29666=CARTESIAN_POINT('Ctrl Pts',(-3.77540022477979,2.59233198125928,394.017066068833));
#29667=CARTESIAN_POINT('Ctrl Pts',(-3.2565579491727,3.13183649817179,393.990690110347));
#29668=CARTESIAN_POINT('Ctrl Pts',(-2.7377156735656,3.6713410150843,393.96431415186));
#29669=CARTESIAN_POINT('Ctrl Pts',(-2.08192669139488,4.0791436858714,393.937938193374));
#29670=CARTESIAN_POINT('Ctrl Pts',(-1.36858515450633,4.30587322182919,393.911562234887));
#29671=CARTESIAN_POINT('Ctrl Pts',(-0.655243617617784,4.53260275778698,
393.885186276401));
#29672=CARTESIAN_POINT('Ctrl Pts',(0.115650473988585,4.57825915891545,393.858810317914));
#29673=CARTESIAN_POINT('Ctrl Pts',(0.850767582565068,4.43731495930334,393.832434359427));
#29674=CARTESIAN_POINT('Ctrl Pts',(1.58588469114154,4.29637075969123,393.806058400941));
#29675=CARTESIAN_POINT('Ctrl Pts',(2.28522481668813,3.96882595933856,393.779682442454));
#29676=CARTESIAN_POINT('Ctrl Pts',(2.86412121787636,3.49433529829511,393.753306483967));
#29677=CARTESIAN_POINT('Ctrl Pts',(3.44301761906461,3.01984463725166,393.726930525481));
#29678=CARTESIAN_POINT('Ctrl Pts',(3.9014702958945,2.39840811551743,393.700554566994));
#29679=CARTESIAN_POINT('Ctrl Pts',(4.18397593491012,1.70526094885616,393.674178608508));
#29680=CARTESIAN_POINT('Ctrl Pts',(4.46648157392573,1.0121137821949,393.647802650021));
#29681=CARTESIAN_POINT('Ctrl Pts',(4.57304017512708,0.247255970606617,393.621426691535));
#29682=CARTESIAN_POINT('Ctrl Pts',(4.49075104942932,-0.496713740146479,
393.595050733048));
#29683=CARTESIAN_POINT('Ctrl Pts',(4.40846192373155,-1.24068345089957,393.568674774561));
#29684=CARTESIAN_POINT('Ctrl Pts',(4.13732507113467,-1.96376506081748,393.542298816075));
#29685=CARTESIAN_POINT('Ctrl Pts',(3.71016611242726,-2.57841752743756,393.515922857588));
#29686=CARTESIAN_POINT('Ctrl Pts',(3.28300715371985,-3.19306999405764,393.489546899101));
#29687=CARTESIAN_POINT('Ctrl Pts',(2.69982608890194,-3.69929331737988,393.463170940615));
#29688=CARTESIAN_POINT('Ctrl Pts',(2.03122667508525,-4.03580075350889,393.436794982129));
#29689=CARTESIAN_POINT('Ctrl Pts',(1.36262726126856,-4.37230818963791,393.410419023642));
#29690=CARTESIAN_POINT('Ctrl Pts',(0.60860949845307,-4.53909973857368,393.384043065155));
#29691=CARTESIAN_POINT('Ctrl Pts',(-0.139540235604001,-4.51598251217256,
393.357667106668));
#29692=CARTESIAN_POINT('Ctrl Pts',(-0.887689969661061,-4.49286528577144,
393.331291148182));
#29693=CARTESIAN_POINT('Ctrl Pts',(-1.62997167495974,-4.27983928403344,
393.304915189695));
#29694=CARTESIAN_POINT('Ctrl Pts',(-2.2765198184931,-3.90269484377256,393.278539231209));
#29695=CARTESIAN_POINT('Ctrl Pts',(-2.92306796202647,-3.52555040351167,
393.252163272722));
#29696=CARTESIAN_POINT('Ctrl Pts',(-3.47388254379453,-2.9842875247279,393.225787314236));
#29697=CARTESIAN_POINT('Ctrl Pts',(-3.86227830720905,-2.3444350716672,393.199411355749));
#29698=CARTESIAN_POINT('Ctrl Pts',(-4.25067407062357,-1.7045826186065,393.173035397262));
#29699=CARTESIAN_POINT('Ctrl Pts',(-4.47665101568456,-0.966140591268864,
393.146659438776));
#29700=CARTESIAN_POINT('Ctrl Pts',(-4.51285087871635,-0.218509665850027,
393.120283480289));
#29701=CARTESIAN_POINT('Ctrl Pts',(-4.51637359912257,-0.145755392857762,
393.117716754357));
#29702=CARTESIAN_POINT('Ctrl Pts',(-4.51809916152901,-0.0729141025000744,
393.115150028424));
#29703=CARTESIAN_POINT('Ctrl Pts',(-4.51804470017939,-7.02313581118758E-5,
393.112583302492));
#29704=CARTESIAN_POINT('Ctrl Pts',(-4.51740214664894,4.58334405226135E-5,
393.387416697508));
#29705=CARTESIAN_POINT('Ctrl Pts',(-4.51724970819312,-0.425542225591553,
393.402406577285));
#29706=CARTESIAN_POINT('Ctrl Pts',(-4.4575812765459,-0.851172152520294,
393.417396457061));
#29707=CARTESIAN_POINT('Ctrl Pts',(-4.33897962224013,-1.25969258594773,
393.432386336838));
#29708=CARTESIAN_POINT('Ctrl Pts',(-4.13029000251061,-1.97851876423963,
393.458762295325));
#29709=CARTESIAN_POINT('Ctrl Pts',(-3.73913503796403,-2.64437160269829,
393.485138253812));
#29710=CARTESIAN_POINT('Ctrl Pts',(-3.21287053587191,-3.1766385524691,393.511514212298));
#29711=CARTESIAN_POINT('Ctrl Pts',(-2.68660603377979,-3.7089055022399,393.537890170785));
#29712=CARTESIAN_POINT('Ctrl Pts',(-2.02523199414213,-4.10758656332286,
393.564266129271));
#29713=CARTESIAN_POINT('Ctrl Pts',(-1.3088187328036,-4.324414769419,393.590642087758));
#29714=CARTESIAN_POINT('Ctrl Pts',(-0.592405471465078,-4.54124297551514,
393.617018046244));
#29715=CARTESIAN_POINT('Ctrl Pts',(0.179047011574318,-4.57621832662447,
393.643394004731));
#29716=CARTESIAN_POINT('Ctrl Pts',(0.912141576006553,-4.42510647540001,
393.669769963218));
#29717=CARTESIAN_POINT('Ctrl Pts',(1.6452361404388,-4.27399462417554,393.696145921704));
#29718=CARTESIAN_POINT('Ctrl Pts',(2.33997278626389,-3.93679557061728,393.722521880191));
#29719=CARTESIAN_POINT('Ctrl Pts',(2.91224209985778,-3.45433286252538,393.748897838677));
#29720=CARTESIAN_POINT('Ctrl Pts',(3.48451141345166,-2.97187015443348,393.775273797164));
#29721=CARTESIAN_POINT('Ctrl Pts',(3.93431339481433,-2.34414379180799,393.801649755651));
#29722=CARTESIAN_POINT('Ctrl Pts',(4.20719204090252,-1.64715048015453,393.828025714137));
#29723=CARTESIAN_POINT('Ctrl Pts',(4.48007068699071,-0.950157168501087,
393.854401672624));
#29724=CARTESIAN_POINT('Ctrl Pts',(4.5760259978044,-0.183896907819673,393.88077763111));
#29725=CARTESIAN_POINT('Ctrl Pts',(4.48344098872769,0.558861766363823,393.907153589597));
#29726=CARTESIAN_POINT('Ctrl Pts',(4.39085597965098,1.30162044054734,393.933529548083));
#29727=CARTESIAN_POINT('Ctrl Pts',(4.10973065068387,2.02087752823294,393.95990550657));
#29728=CARTESIAN_POINT('Ctrl Pts',(3.67409989363231,2.62955500891649,393.986281465057));
#29729=CARTESIAN_POINT('Ctrl Pts',(3.23846913658077,3.23823248960003,394.012657423543));
#29730=CARTESIAN_POINT('Ctrl Pts',(2.64833295144478,3.73633036328149,394.03903338203));
#29731=CARTESIAN_POINT('Ctrl Pts',(1.97513712820591,4.06354560674411,394.065409340517));
#29732=CARTESIAN_POINT('Ctrl Pts',(1.30194130496704,4.39076085020672,394.091785299003));
#29733=CARTESIAN_POINT('Ctrl Pts',(0.54568584362529,4.54709346345051,394.11816125749));
#29734=CARTESIAN_POINT('Ctrl Pts',(-0.202071967477526,4.51361678626648,
394.144537215976));
#29735=CARTESIAN_POINT('Ctrl Pts',(-0.949829778580352,4.48014010908246,
394.170913174463));
#29736=CARTESIAN_POINT('Ctrl Pts',(-1.68908993944425,4.25685414147062,394.19728913295));
#29737=CARTESIAN_POINT('Ctrl Pts',(-2.33035272521732,3.8707913595774,394.223665091436));
#29738=CARTESIAN_POINT('Ctrl Pts',(-2.97161551099039,3.48472857768417,394.250041049923));
#29739=CARTESIAN_POINT('Ctrl Pts',(-3.51488092167263,2.93588898150954,394.276417008409));
#29740=CARTESIAN_POINT('Ctrl Pts',(-3.89437765326087,2.29071872282242,394.302792966896));
#29741=CARTESIAN_POINT('Ctrl Pts',(-4.27387438484911,1.64554846413529,394.329168925382));
#29742=CARTESIAN_POINT('Ctrl Pts',(-4.48960243734335,0.904047542935649,
394.355544883869));
#29743=CARTESIAN_POINT('Ctrl Pts',(-4.51544434579255,0.15598696534298,394.381920842355));
#29744=CARTESIAN_POINT('Ctrl Pts',(-4.51723920487186,0.104030147904069,
394.383752794073));
#29745=CARTESIAN_POINT('Ctrl Pts',(-4.51811804423603,0.0520416863733224,
394.38558474579));
#29746=CARTESIAN_POINT('Ctrl Pts',(-4.51808751818987,5.21912322906659E-5,
394.387416697508));
#29747=CARTESIAN_POINT('Origin',(0.,0.,387.));
#29748=CARTESIAN_POINT('',(-4.51761539860092,-0.000109498206778275,395.387416697508));
#29749=CARTESIAN_POINT('',(-4.51787769339044,0.000106674156513836,395.112583302492));
#29750=CARTESIAN_POINT('',(-4.51775,5.53264807684796E-16,387.));
#29751=CARTESIAN_POINT('Ctrl Pts',(-4.51787769339044,0.000106674156513836,
395.112583302492));
#29752=CARTESIAN_POINT('Ctrl Pts',(-4.51801115526906,0.13353505519604,395.107882323922));
#29753=CARTESIAN_POINT('Ctrl Pts',(-4.51221712826522,0.266951885784635,
395.103181345353));
#29754=CARTESIAN_POINT('Ctrl Pts',(-4.50041129427044,0.39983460330973,395.098480366784));
#29755=CARTESIAN_POINT('Ctrl Pts',(-4.43417185438628,1.14540469882723,395.072104408297));
#29756=CARTESIAN_POINT('Ctrl Pts',(-4.17867844925679,1.87416071243738,395.04572844981));
#29757=CARTESIAN_POINT('Ctrl Pts',(-3.76486280044783,2.49787462083366,395.019352491324));
#29758=CARTESIAN_POINT('Ctrl Pts',(-3.35104715163886,3.12158852922995,394.992976532837));
#29759=CARTESIAN_POINT('Ctrl Pts',(-2.77890925915041,3.64026033241238,394.966600574351));
#29760=CARTESIAN_POINT('Ctrl Pts',(-2.11771592060786,3.99109619117415,394.940224615864));
#29761=CARTESIAN_POINT('Ctrl Pts',(-1.45652258206532,4.34193204993591,394.913848657377));
#29762=CARTESIAN_POINT('Ctrl Pts',(-0.706273797468684,4.52493196427704,
394.887472698891));
#29763=CARTESIAN_POINT('Ctrl Pts',(0.0422003528576968,4.51794075412897,
394.861096740404));
#29764=CARTESIAN_POINT('Ctrl Pts',(0.790674503184078,4.51094954398091,394.834720781918));
#29765=CARTESIAN_POINT('Ctrl Pts',(1.5373740192402,4.31396720934364,394.808344823431));
#29766=CARTESIAN_POINT('Ctrl Pts',(2.19189851862757,3.9508417345724,394.781968864945));
#29767=CARTESIAN_POINT('Ctrl Pts',(2.84642301801496,3.58771625980115,394.755592906458));
#29768=CARTESIAN_POINT('Ctrl Pts',(3.4087725007336,3.05844764489591,394.729216947971));
#29769=CARTESIAN_POINT('Ctrl Pts',(3.81086521878951,2.4271126491824,394.702840989485));
#29770=CARTESIAN_POINT('Ctrl Pts',(4.2129579368454,1.79577765346891,394.676465030998));
#29771=CARTESIAN_POINT('Ctrl Pts',(4.45479389023857,1.06237627694715,394.650089072511));
#29772=CARTESIAN_POINT('Ctrl Pts',(4.50709481884649,0.315698941284091,394.623713114025));
#29773=CARTESIAN_POINT('Ctrl Pts',(4.55939574745442,-0.430978394378985,
394.597337155538));
#29774=CARTESIAN_POINT('Ctrl Pts',(4.4221616512771,-1.19093168918336,394.570961197052));
#29775=CARTESIAN_POINT('Ctrl Pts',(4.11200699772181,-1.8721559706092,394.544585238565));
#29776=CARTESIAN_POINT('Ctrl Pts',(3.80185234416652,-2.55338025203503,394.518209280079));
#29777=CARTESIAN_POINT('Ctrl Pts',(3.31877713323327,-3.15587552008233,394.491833321592));
#29778=CARTESIAN_POINT('Ctrl Pts',(2.72126564522031,-3.60669971244412,394.465457363105));
#29779=CARTESIAN_POINT('Ctrl Pts',(2.12375415720733,-4.05752390480593,394.439081404619));
#29780=CARTESIAN_POINT('Ctrl Pts',(1.41180639211463,-4.35667702148223,394.412705446132));
#29781=CARTESIAN_POINT('Ctrl Pts',(0.67161545550637,-4.46794160744361,394.386329487646));
#29782=CARTESIAN_POINT('Ctrl Pts',(-0.0685754811018632,-4.57920619340499,
394.359953529159));
#29783=CARTESIAN_POINT('Ctrl Pts',(-0.837009589225651,-4.50258224865146,
394.333577570673));
#29784=CARTESIAN_POINT('Ctrl Pts',(-1.54065515298906,-4.2473463747579,394.307201612186));
#29785=CARTESIAN_POINT('Ctrl Pts',(-2.24430071675247,-3.99211050086433,
394.280825653699));
#29786=CARTESIAN_POINT('Ctrl Pts',(-2.88315773615551,-3.55826269783073,
394.254449695213));
#29787=CARTESIAN_POINT('Ctrl Pts',(-3.37988195476012,-2.99832745034422,
394.228073736726));
#29788=CARTESIAN_POINT('Ctrl Pts',(-3.87660617336475,-2.43839220285771,
394.20169777824));
#29789=CARTESIAN_POINT('Ctrl Pts',(-4.23119759117096,-1.75236951091828,
394.175321819753));
#29790=CARTESIAN_POINT('Ctrl Pts',(-4.40072702572232,-1.02331381925484,
394.148945861266));
#29791=CARTESIAN_POINT('Ctrl Pts',(-4.47863287106505,-0.688282323920289,
394.136825008341));
#29792=CARTESIAN_POINT('Ctrl Pts',(-4.51745758988365,-0.34416318088334,
394.124704155417));
#29793=CARTESIAN_POINT('Ctrl Pts',(-4.5173836733729,-2.76243915998559E-5,
394.112583302492));
#29794=CARTESIAN_POINT('Ctrl Pts',(-4.51808751818987,5.21912322906659E-5,
394.387416697508));
#29795=CARTESIAN_POINT('Ctrl Pts',(-4.51767853826069,-0.696489376170657,
394.411960704277));
#29796=CARTESIAN_POINT('Ctrl Pts',(-4.35403905930357,-1.39321647594668,
394.436504711046));
#29797=CARTESIAN_POINT('Ctrl Pts',(-4.0431719192238,-2.01651441971212,394.461048717815));
#29798=CARTESIAN_POINT('Ctrl Pts',(-3.70910181980172,-2.68633499318885,
394.487424676302));
#29799=CARTESIAN_POINT('Ctrl Pts',(-3.20500585655341,-3.27135590615661,
394.513800634789));
#29800=CARTESIAN_POINT('Ctrl Pts',(-2.59191322109249,-3.70075065731708,
394.540176593275));
#29801=CARTESIAN_POINT('Ctrl Pts',(-1.97882058563158,-4.13014540847754,
394.566552551762));
#29802=CARTESIAN_POINT('Ctrl Pts',(-1.25673127795806,-4.40391399783071,
394.592928510249));
#29803=CARTESIAN_POINT('Ctrl Pts',(-0.513066205861354,-4.48891218912888,
394.619304468735));
#29804=CARTESIAN_POINT('Ctrl Pts',(0.230598866235364,-4.57391038042705,
394.645680427222));
#29805=CARTESIAN_POINT('Ctrl Pts',(0.995839702755266,-4.47013817367021,
394.672056385708));
#29806=CARTESIAN_POINT('Ctrl Pts',(1.69001118640443,-4.19015891860138,394.698432344195));
#29807=CARTESIAN_POINT('Ctrl Pts',(2.3841826700536,-3.91017966353254,394.724808302681));
#29808=CARTESIAN_POINT('Ctrl Pts',(3.00728480083202,-3.45399336015171,394.751184261168));
#29809=CARTESIAN_POINT('Ctrl Pts',(3.48388071332803,-2.87682893975429,394.777560219655));
#29810=CARTESIAN_POINT('Ctrl Pts',(3.96047662582402,-2.29966451935688,394.803936178141));
#29811=CARTESIAN_POINT('Ctrl Pts',(4.29056632003761,-1.6015219819429,394.830312136628));
#29812=CARTESIAN_POINT('Ctrl Pts',(4.43418695423518,-0.866923080900132,
394.856688095114));
#29813=CARTESIAN_POINT('Ctrl Pts',(4.57780758843275,-0.132324179857343,
394.883064053601));
#29814=CARTESIAN_POINT('Ctrl Pts',(4.5349591626143,0.638731084814249,394.909440012088));
#29815=CARTESIAN_POINT('Ctrl Pts',(4.31082919062693,1.35289366268957,394.935815970574));
#29816=CARTESIAN_POINT('Ctrl Pts',(4.08669921863955,2.06705624056489,394.962191929061));
#29817=CARTESIAN_POINT('Ctrl Pts',(3.68128770048325,2.72432613164396,394.988567887547));
#29818=CARTESIAN_POINT('Ctrl Pts',(3.14367643610836,3.24512989545316,395.014943846034));
#29819=CARTESIAN_POINT('Ctrl Pts',(2.60606517173349,3.76593365926234,395.04131980452));
#29820=CARTESIAN_POINT('Ctrl Pts',(1.93625416114004,4.15027129580166,395.067695763007));
#29821=CARTESIAN_POINT('Ctrl Pts',(1.21533515568228,4.35161234862086,395.094071721494));
#29822=CARTESIAN_POINT('Ctrl Pts',(0.494416150224501,4.55295340144005,395.12044767998));
#29823=CARTESIAN_POINT('Ctrl Pts',(-0.277610850097608,4.57129787053912,
395.146823638467));
#29824=CARTESIAN_POINT('Ctrl Pts',(-1.00727915011366,4.40442485315088,395.173199596953));
#29825=CARTESIAN_POINT('Ctrl Pts',(-1.73694745012971,4.23755183576263,395.19957555544));
#29826=CARTESIAN_POINT('Ctrl Pts',(-2.42425704983972,3.88546133188709,395.225951513927));
#29827=CARTESIAN_POINT('Ctrl Pts',(-2.98599770294795,3.39077974679813,395.252327472413));
#29828=CARTESIAN_POINT('Ctrl Pts',(-3.54773835605617,2.89609816170917,395.2787034309));
#29829=CARTESIAN_POINT('Ctrl Pts',(-3.9839100625626,2.25882549540681,395.305079389386));
#29830=CARTESIAN_POINT('Ctrl Pts',(-4.24170699065442,1.55611419206311,395.331455347873));
#29831=CARTESIAN_POINT('Ctrl Pts',(-4.42402787244154,1.05913796579184,395.350109131085));
#29832=CARTESIAN_POINT('Ctrl Pts',(-4.5171311009058,0.529431318295306,395.368762914296));
#29833=CARTESIAN_POINT('Ctrl Pts',(-4.51761539860092,-0.000109498206778275,
395.387416697508));
#29834=CARTESIAN_POINT('Origin',(0.,0.,387.));
#29835=CARTESIAN_POINT('',(-4.51751463264715,9.2546932777271E-5,396.387416697508));
#29836=CARTESIAN_POINT('',(-4.51786437784292,-0.000108222965875699,396.112583302492));
#29837=CARTESIAN_POINT('',(-4.51775,5.53264807684796E-16,387.));
#29838=CARTESIAN_POINT('Ctrl Pts',(-4.51786437784292,-0.000108222965875699,
396.112583302492));
#29839=CARTESIAN_POINT('Ctrl Pts',(-4.5172490555957,0.610781207776803,396.091060492428));
#29840=CARTESIAN_POINT('Ctrl Pts',(-4.39244234778488,1.22191440722307,396.069537682365));
#29841=CARTESIAN_POINT('Ctrl Pts',(-4.15139232023937,1.78311842878099,396.048014872301));
#29842=CARTESIAN_POINT('Ctrl Pts',(-3.85598825818002,2.47086756243728,396.021638913814));
#29843=CARTESIAN_POINT('Ctrl Pts',(-3.38600738379809,3.0836319422382,395.995262955328));
#29844=CARTESIAN_POINT('Ctrl Pts',(-2.79834869039748,3.54722625928365,395.968886996841));
#29845=CARTESIAN_POINT('Ctrl Pts',(-2.21068999699688,4.0108205763291,395.942511038355));
#29846=CARTESIAN_POINT('Ctrl Pts',(-1.50535348457759,4.32524483061908,395.916135079868));
#29847=CARTESIAN_POINT('Ctrl Pts',(-0.767731856725531,4.45243274219494,
395.889759121381));
#29848=CARTESIAN_POINT('Ctrl Pts',(-0.0301102288734742,4.5796206537708,
395.863383162895));
#29849=CARTESIAN_POINT('Ctrl Pts',(0.739796514411352,4.51957222263255,395.837007204408));
#29850=CARTESIAN_POINT('Ctrl Pts',(1.44877837029978,4.27955730903937,395.810631245922));
#29851=CARTESIAN_POINT('Ctrl Pts',(2.15776022618821,4.03954239544619,395.784255287435));
#29852=CARTESIAN_POINT('Ctrl Pts',(2.80581719468025,3.61956099939807,395.757879328948));
#29853=CARTESIAN_POINT('Ctrl Pts',(3.31449121264882,3.07045884663426,395.731503370462));
#29854=CARTESIAN_POINT('Ctrl Pts',(3.82316523061738,2.52135669387044,395.705127411975));
#29855=CARTESIAN_POINT('Ctrl Pts',(4.19245629806247,1.84313378439093,395.678751453489));
#29856=CARTESIAN_POINT('Ctrl Pts',(4.37765559571272,1.11790026966896,395.652375495002));
#29857=CARTESIAN_POINT('Ctrl Pts',(4.56285489336297,0.392666754946975,395.625999536516));
#29858=CARTESIAN_POINT('Ctrl Pts',(4.56396242121836,-0.379577365017472,
395.599623578029));
#29859=CARTESIAN_POINT('Ctrl Pts',(4.38084409463107,-1.10533910911399,395.573247619542));
#29860=CARTESIAN_POINT('Ctrl Pts',(4.19772576804378,-1.8311008532105,395.546871661056));
#29861=CARTESIAN_POINT('Ctrl Pts',(3.8303815870138,-2.51038022143909,395.520495702569));
#29862=CARTESIAN_POINT('Ctrl Pts',(3.32328466786559,-3.06093916044248,395.494119744083));
#29863=CARTESIAN_POINT('Ctrl Pts',(2.81618774871737,-3.61149809944587,395.467743785596));
#29864=CARTESIAN_POINT('Ctrl Pts',(2.16933809145092,-4.03333660922406,395.441367827109));
#29865=CARTESIAN_POINT('Ctrl Pts',(1.46104759411067,-4.27538412956593,395.414991868623));
#29866=CARTESIAN_POINT('Ctrl Pts',(0.75275709677042,-4.5174316499078,395.388615910136));
#29867=CARTESIAN_POINT('Ctrl Pts',(-0.0169742406436262,-4.57968818081335,
395.36223995165));
#29868=CARTESIAN_POINT('Ctrl Pts',(-0.754957651097232,-4.45461653486027,
395.335863993163));
#29869=CARTESIAN_POINT('Ctrl Pts',(-1.49294106155083,-4.3295448889072,395.309488034676));
#29870=CARTESIAN_POINT('Ctrl Pts',(-2.19917654504398,-4.01714506609549,
395.28311207619));
#29871=CARTESIAN_POINT('Ctrl Pts',(-2.78816256260641,-3.5552382553186,395.256736117703));
#29872=CARTESIAN_POINT('Ctrl Pts',(-3.37714858016886,-3.0933314445417,395.230360159217));
#29873=CARTESIAN_POINT('Ctrl Pts',(-3.84888513180058,-2.4819176457996,395.20398420073));
#29874=CARTESIAN_POINT('Ctrl Pts',(-4.14626067029702,-1.79501865771611,
395.177608242243));
#29875=CARTESIAN_POINT('Ctrl Pts',(-4.39063506253172,-1.23054545461321,
395.155933262326));
#29876=CARTESIAN_POINT('Ctrl Pts',(-4.51726233565243,-0.615096615266284,
395.134258282409));
#29877=CARTESIAN_POINT('Ctrl Pts',(-4.51787769339044,0.000106674156513836,
395.112583302492));
#29878=CARTESIAN_POINT('Ctrl Pts',(-4.51761539860092,-0.000109498206778275,
395.387416697508));
#29879=CARTESIAN_POINT('Ctrl Pts',(-4.51781588509979,-0.219325458522322,
395.395138872783));
#29880=CARTESIAN_POINT('Ctrl Pts',(-4.5021438757463,-0.438512999682626,
395.402861048058));
#29881=CARTESIAN_POINT('Ctrl Pts',(-4.47035806891458,-0.655338316442091,
395.410583223333));
#29882=CARTESIAN_POINT('Ctrl Pts',(-4.36179006940572,-1.39592958121857,
395.436959181819));
#29883=CARTESIAN_POINT('Ctrl Pts',(-4.06523192071081,-2.10896217038649,
395.463335140306));
#29884=CARTESIAN_POINT('Ctrl Pts',(-3.61658691387121,-2.70811164240368,
395.489711098793));
#29885=CARTESIAN_POINT('Ctrl Pts',(-3.16794190703161,-3.30726111442086,
395.516087057279));
#29886=CARTESIAN_POINT('Ctrl Pts',(-2.56721004204732,-3.79252746928731,
395.542463015766));
#29887=CARTESIAN_POINT('Ctrl Pts',(-1.88711989198663,-4.10516115232706,
395.568838974252));
#29888=CARTESIAN_POINT('Ctrl Pts',(-1.20702974192593,-4.4177948353668,395.595214932739));
#29889=CARTESIAN_POINT('Ctrl Pts',(-0.447581306788832,-4.55779584657986,
395.621590891225));
#29890=CARTESIAN_POINT('Ctrl Pts',(0.299281562555524,-4.50821473752317,
395.647966849712));
#29891=CARTESIAN_POINT('Ctrl Pts',(1.04614443189988,-4.45863362846649,395.674342808199));
#29892=CARTESIAN_POINT('Ctrl Pts',(1.78042173545149,-4.21947039914007,395.700718766685));
#29893=CARTESIAN_POINT('Ctrl Pts',(2.4132170060234,-3.81967973201239,395.727094725172));
#29894=CARTESIAN_POINT('Ctrl Pts',(3.04601227659532,-3.41988906488471,395.753470683659));
#29895=CARTESIAN_POINT('Ctrl Pts',(3.57732551418753,-2.85947095995576,395.779846642145));
#29896=CARTESIAN_POINT('Ctrl Pts',(3.94283242392784,-2.20627333984937,395.806222600631));
#29897=CARTESIAN_POINT('Ctrl Pts',(4.30833933366816,-1.55307571974297,395.832598559118));
#29898=CARTESIAN_POINT('Ctrl Pts',(4.50803991555659,-0.807098584459129,
395.858974517605));
#29899=CARTESIAN_POINT('Ctrl Pts',(4.51775709624605,-0.0586548602019053,
395.885350476092));
#29900=CARTESIAN_POINT('Ctrl Pts',(4.5274742769355,0.689788864055318,395.911726434578));
#29901=CARTESIAN_POINT('Ctrl Pts',(4.34720805642599,1.44069917728592,395.938102393065));
#29902=CARTESIAN_POINT('Ctrl Pts',(3.99878265572902,2.10316591013349,395.964478351551));
#29903=CARTESIAN_POINT('Ctrl Pts',(3.65035725503204,2.76563264298105,395.990854310038));
#29904=CARTESIAN_POINT('Ctrl Pts',(3.13377267414759,3.33965579544558,396.017230268524));
#29905=CARTESIAN_POINT('Ctrl Pts',(2.5115700593453,3.75574032785908,396.043606227011));
#29906=CARTESIAN_POINT('Ctrl Pts',(1.88936744454301,4.17182486027259,396.069982185498));
#29907=CARTESIAN_POINT('Ctrl Pts',(1.16154679582287,4.42997077263507,396.096358143984));
#29908=CARTESIAN_POINT('Ctrl Pts',(0.416222895030907,4.49892521331027,396.122734102471));
#29909=CARTESIAN_POINT('Ctrl Pts',(-0.329101005761055,4.56787965398547,
396.149110060957));
#29910=CARTESIAN_POINT('Ctrl Pts',(-1.09192815862484,4.44764262297338,396.175486019444));
#29911=CARTESIAN_POINT('Ctrl Pts',(-1.77990566277504,4.15277081054664,396.201861977931));
#29912=CARTESIAN_POINT('Ctrl Pts',(-2.46788316692524,3.85789899811989,396.228237936417));
#29913=CARTESIAN_POINT('Ctrl Pts',(-3.08101102236186,3.38839240427848,396.254613894904));
#29914=CARTESIAN_POINT('Ctrl Pts',(-3.54505991542016,2.80109260278699,396.28098985339));
#29915=CARTESIAN_POINT('Ctrl Pts',(-4.00910880847846,2.2137928012955,396.307365811877));
#29916=CARTESIAN_POINT('Ctrl Pts',(-4.32407873915844,1.50869979215393,396.333741770364));
#29917=CARTESIAN_POINT('Ctrl Pts',(-4.45183736430835,0.771176798830757,
396.36011772885));
#29918=CARTESIAN_POINT('Ctrl Pts',(-4.4959138504198,0.516732749092945,396.369217385069));
#29919=CARTESIAN_POINT('Ctrl Pts',(-4.51770775311255,0.258428762447222,
396.378317041289));
#29920=CARTESIAN_POINT('Ctrl Pts',(-4.51751463264715,9.2546932777271E-5,
396.387416697508));
#29921=CARTESIAN_POINT('Origin',(0.,0.,387.));
#29922=CARTESIAN_POINT('',(-4.51813440218219,-1.34914224690988E-5,397.387416697508));
#29923=CARTESIAN_POINT('',(-4.51738673749921,3.14726202902737E-5,397.112583302492));
#29924=CARTESIAN_POINT('',(-4.51775,5.53264807684796E-16,387.));
#29925=CARTESIAN_POINT('Ctrl Pts',(-4.51738673749921,3.14726202902737E-5,
397.112583302492));
#29926=CARTESIAN_POINT('Ctrl Pts',(-4.51746996308395,0.339845959287686,
397.100614619421));
#29927=CARTESIAN_POINT('Ctrl Pts',(-4.47962267703118,0.67964219695818,397.088645936349));
#29928=CARTESIAN_POINT('Ctrl Pts',(-4.40364412455734,1.01068687131693,397.076677253278));
#29929=CARTESIAN_POINT('Ctrl Pts',(-4.236206559874,1.7402258302897,397.050301294792));
#29930=CARTESIAN_POINT('Ctrl Pts',(-3.88358434036526,2.42726278544303,397.023925336305));
#29931=CARTESIAN_POINT('Ctrl Pts',(-3.38846824431658,2.9886204986346,396.997549377818));
#29932=CARTESIAN_POINT('Ctrl Pts',(-2.89335214826789,3.54997821182617,396.971173419332));
#29933=CARTESIAN_POINT('Ctrl Pts',(-2.25574217567927,3.98565668305597,396.944797460845));
#29934=CARTESIAN_POINT('Ctrl Pts',(-1.55283160725287,4.24290979483623,396.918421502359));
#29935=CARTESIAN_POINT('Ctrl Pts',(-0.849921038826476,4.5001629066165,396.892045543872));
#29936=CARTESIAN_POINT('Ctrl Pts',(-0.0817098745623172,4.57899065894722,
396.865669585385));
#29937=CARTESIAN_POINT('Ctrl Pts',(0.658797160721962,4.46984964273134,396.839293626899));
#29938=CARTESIAN_POINT('Ctrl Pts',(1.39930419600623,4.36070862651545,396.812917668412));
#29939=CARTESIAN_POINT('Ctrl Pts',(2.11210710231061,4.06359884175296,396.786541709925));
#29940=CARTESIAN_POINT('Ctrl Pts',(2.71090924501961,3.61449036419631,396.760165751439));
#29941=CARTESIAN_POINT('Ctrl Pts',(3.30971138772862,3.16538188663966,396.733789792952));
#29942=CARTESIAN_POINT('Ctrl Pts',(3.79451276684224,2.56427471628884,396.707413834466));
#29943=CARTESIAN_POINT('Ctrl Pts',(4.10662012072468,1.88394286316225,396.681037875979));
#29944=CARTESIAN_POINT('Ctrl Pts',(4.41872747460713,1.20361101003566,396.654661917493));
#29945=CARTESIAN_POINT('Ctrl Pts',(4.5581408032584,0.444054474133294,396.628285959006));
#29946=CARTESIAN_POINT('Ctrl Pts',(4.50798180697358,-0.302769806282027,
396.601910000519));
#29947=CARTESIAN_POINT('Ctrl Pts',(4.45782281068875,-1.04959408669733,396.575534042033));
#29948=CARTESIAN_POINT('Ctrl Pts',(4.21809148946783,-1.78368611162558,396.549158083546));
#29949=CARTESIAN_POINT('Ctrl Pts',(3.81781130274164,-2.41617184493549,396.52278212506));
#29950=CARTESIAN_POINT('Ctrl Pts',(3.41753111601545,-3.0486575782454,396.496406166573));
#29951=CARTESIAN_POINT('Ctrl Pts',(2.85670206378398,-3.57953701993697,396.470030208087));
#29952=CARTESIAN_POINT('Ctrl Pts',(2.20322182066968,-3.94453839333905,396.4436542496));
#29953=CARTESIAN_POINT('Ctrl Pts',(1.54974157755536,-4.30953976674113,396.417278291113));
#29954=CARTESIAN_POINT('Ctrl Pts',(0.803610143558188,-4.50866307185371,
396.390902332627));
#29955=CARTESIAN_POINT('Ctrl Pts',(0.0551591253050773,-4.51780112427455,
396.36452637414));
#29956=CARTESIAN_POINT('Ctrl Pts',(-0.693291892948023,-4.52693917669538,
396.338150415653));
#29957=CARTESIAN_POINT('Ctrl Pts',(-1.44406249545706,-4.34609197642448,
396.311774457167));
#29958=CARTESIAN_POINT('Ctrl Pts',(-2.10625942716968,-3.9971540817261,396.28539849868));
#29959=CARTESIAN_POINT('Ctrl Pts',(-2.7684563588823,-3.64821618702772,396.259022540194));
#29960=CARTESIAN_POINT('Ctrl Pts',(-3.3420796197985,-3.13118759790186,396.232646581707));
#29961=CARTESIAN_POINT('Ctrl Pts',(-3.7576825837662,-2.5086632151927,396.206270623221));
#29962=CARTESIAN_POINT('Ctrl Pts',(-4.17328554773389,-1.88613883248355,
396.179894664734));
#29963=CARTESIAN_POINT('Ctrl Pts',(-4.43086821475307,-1.15811865619109,
396.153518706247));
#29964=CARTESIAN_POINT('Ctrl Pts',(-4.49924592339428,-0.412741624289035,
396.127142747761));
#29965=CARTESIAN_POINT('Ctrl Pts',(-4.51182734935556,-0.275593039955457,
396.122289599338));
#29966=CARTESIAN_POINT('Ctrl Pts',(-4.51800312599824,-0.137856828684076,
396.117436450915));
#29967=CARTESIAN_POINT('Ctrl Pts',(-4.51786437784292,-0.000108222965875699,
396.112583302492));
#29968=CARTESIAN_POINT('Ctrl Pts',(-4.51751463264715,9.2546932777271E-5,
396.387416697508));
#29969=CARTESIAN_POINT('Ctrl Pts',(-4.51714798060515,-0.490375932126388,
396.404692999775));
#29970=CARTESIAN_POINT('Ctrl Pts',(-4.43752790145426,-0.98096058190497,
396.421969302042));
#29971=CARTESIAN_POINT('Ctrl Pts',(-4.28067705789975,-1.44546653343395,
396.43924560431));
#29972=CARTESIAN_POINT('Ctrl Pts',(-4.04121080672139,-2.1546338948707,396.465621562796));
#29973=CARTESIAN_POINT('Ctrl Pts',(-3.62173098474482,-2.80301564023941,
396.491997521283));
#29974=CARTESIAN_POINT('Ctrl Pts',(-3.07302259383454,-3.3121143867761,396.51837347977));
#29975=CARTESIAN_POINT('Ctrl Pts',(-2.52431420292427,-3.8212131333128,396.544749438256));
#29976=CARTESIAN_POINT('Ctrl Pts',(-1.84637724308029,-4.19102888101748,
396.571125396743));
#29977=CARTESIAN_POINT('Ctrl Pts',(-1.12128724682158,-4.37678928935608,
396.597501355229));
#29978=CARTESIAN_POINT('Ctrl Pts',(-0.396197250562878,-4.56254969769468,
396.623877313716));
#29979=CARTESIAN_POINT('Ctrl Pts',(0.376045782110559,-4.5642547666672,396.650253272203));
#29980=CARTESIAN_POINT('Ctrl Pts',(1.10194900172297,-4.38169806934578,396.676629230689));
#29981=CARTESIAN_POINT('Ctrl Pts',(1.82785222133539,-4.19914137202436,396.703005189176));
#29982=CARTESIAN_POINT('Ctrl Pts',(2.50741562788679,-3.83232290840901,396.729381147662));
#29983=CARTESIAN_POINT('Ctrl Pts',(3.05836678046179,-3.32565214799663,396.755757106149));
#29984=CARTESIAN_POINT('Ctrl Pts',(3.60931793303678,-2.81898138758426,396.782133064635));
#29985=CARTESIAN_POINT('Ctrl Pts',(4.03165683163537,-2.17245833037488,396.808509023122));
#29986=CARTESIAN_POINT('Ctrl Pts',(4.27425233566608,-1.46435533404973,396.834884981609));
#29987=CARTESIAN_POINT('Ctrl Pts',(4.51684783969678,-0.756252337724576,
396.861260940095));
#29988=CARTESIAN_POINT('Ctrl Pts',(4.57969994915959,0.0134305977163408,
396.887636898582));
#29989=CARTESIAN_POINT('Ctrl Pts',(4.45519937195264,0.751510565101793,396.914012857069));
#29990=CARTESIAN_POINT('Ctrl Pts',(4.33069879474569,1.48959053248724,396.940388815555));
#29991=CARTESIAN_POINT('Ctrl Pts',(4.01884553086897,2.19606753181724,396.966764774042));
#29992=CARTESIAN_POINT('Ctrl Pts',(3.5573945991761,2.78541078461679,396.993140732528));
#29993=CARTESIAN_POINT('Ctrl Pts',(3.09594366748323,3.37475403741634,397.019516691015));
#29994=CARTESIAN_POINT('Ctrl Pts',(2.4848950679742,3.84696354368545,397.045892649502));
#29995=CARTESIAN_POINT('Ctrl Pts',(1.79822638583807,4.14487049720285,397.072268607988));
#29996=CARTESIAN_POINT('Ctrl Pts',(1.11155770370195,4.44277745072024,397.098644566475));
#29997=CARTESIAN_POINT('Ctrl Pts',(0.349268938938723,4.56638185148592,397.125020524961));
#29998=CARTESIAN_POINT('Ctrl Pts',(-0.396352188490757,4.50071933317169,
397.151396483448));
#29999=CARTESIAN_POINT('Ctrl Pts',(-1.14197331592023,4.43505681485745,397.177772441934));
#30000=CARTESIAN_POINT('Ctrl Pts',(-1.87092680601596,4.18012737746331,397.204148400421));
#30001=CARTESIAN_POINT('Ctrl Pts',(-2.49496072766192,3.76679446489074,397.230524358908));
#30002=CARTESIAN_POINT('Ctrl Pts',(-3.1189946493079,3.35346155231816,397.256900317394));
#30003=CARTESIAN_POINT('Ctrl Pts',(-3.63810900250409,2.78172516456714,397.283276275881));
#30004=CARTESIAN_POINT('Ctrl Pts',(-3.98945637001185,2.12080349044383,397.309652234368));
#30005=CARTESIAN_POINT('Ctrl Pts',(-4.33474984909618,1.47126982272609,397.335573722081));
#30006=CARTESIAN_POINT('Ctrl Pts',(-4.51800794997827,0.735597803364803,
397.361495209794));
#30007=CARTESIAN_POINT('Ctrl Pts',(-4.51813440218219,-1.34914224690988E-5,
397.387416697508));
#30008=CARTESIAN_POINT('Origin',(0.,0.,387.));
#30009=CARTESIAN_POINT('',(-4.51746064445937,-7.62825515632226E-5,398.387416697508));
#30010=CARTESIAN_POINT('',(-4.51805439081064,6.66898104614677E-5,398.112583302492));
#30011=CARTESIAN_POINT('',(-4.51775,5.53264807684796E-16,387.));
#30012=CARTESIAN_POINT('Ctrl Pts',(-4.51805439081064,6.66898104614677E-5,
398.112583302492));
#30013=CARTESIAN_POINT('Ctrl Pts',(-4.51810357212516,0.0685915430668216,
398.110168746413));
#30014=CARTESIAN_POINT('Ctrl Pts',(-4.51657662108523,0.137114203419027,
398.107754190334));
#30015=CARTESIAN_POINT('Ctrl Pts',(-4.51345907222813,0.205564420371811,
398.105339634255));
#30016=CARTESIAN_POINT('Ctrl Pts',(-4.47940381049539,0.953296103447074,
398.078963675769));
#30017=CARTESIAN_POINT('Ctrl Pts',(-4.255545890619,1.6923832695825,398.052587717282));
#30018=CARTESIAN_POINT('Ctrl Pts',(-3.86898703306984,2.33334713781254,398.026211758796));
#30019=CARTESIAN_POINT('Ctrl Pts',(-3.48242817552068,2.97431100604258,397.999835800309));
#30020=CARTESIAN_POINT('Ctrl Pts',(-2.93316838029875,3.51715157636723,397.973459841822));
#30021=CARTESIAN_POINT('Ctrl Pts',(-2.28770467124889,3.89614897876697,397.947083883336));
#30022=CARTESIAN_POINT('Ctrl Pts',(-1.64224096219904,4.27514638116671,397.920707924849));
#30023=CARTESIAN_POINT('Ctrl Pts',(-0.900573339321256,4.49030061564153,
397.894331966363));
#30024=CARTESIAN_POINT('Ctrl Pts',(-0.15249299074285,4.51556368744535,397.867956007876));
#30025=CARTESIAN_POINT('Ctrl Pts',(0.595587357835559,4.54082675924917,397.841580049389));
#30026=CARTESIAN_POINT('Ctrl Pts',(1.35008043211458,4.37619866838198,397.815204090903));
#30027=CARTESIAN_POINT('Ctrl Pts',(2.01964230998743,4.0416103804436,397.788828132416));
#30028=CARTESIAN_POINT('Ctrl Pts',(2.68920418786027,3.70702209250522,397.76245217393));
#30029=CARTESIAN_POINT('Ctrl Pts',(3.27383486932692,3.20247360749564,397.736076215443));
#30030=CARTESIAN_POINT('Ctrl Pts',(3.70275509709574,2.58904890230608,397.709700256956));
#30031=CARTESIAN_POINT('Ctrl Pts',(4.13167532486456,1.97562419711653,397.68332429847));
#30032=CARTESIAN_POINT('Ctrl Pts',(4.40488509893554,1.25332327174699,397.656948339983));
#30033=CARTESIAN_POINT('Ctrl Pts',(4.48930783693528,0.509592653824902,397.630572381497));
#30034=CARTESIAN_POINT('Ctrl Pts',(4.57373057493501,-0.234137964097188,
397.60419642301));
#30035=CARTESIAN_POINT('Ctrl Pts',(4.4693662768635,-0.999298274571833,397.577820464523));
#30036=CARTESIAN_POINT('Ctrl Pts',(4.18884997495465,-1.69325290932077,397.551444506037));
#30037=CARTESIAN_POINT('Ctrl Pts',(3.9083336730458,-2.3872075440697,397.52506854755));
#30038=CARTESIAN_POINT('Ctrl Pts',(3.4516653672996,-3.00995650309293,397.498692589064));
#30039=CARTESIAN_POINT('Ctrl Pts',(2.87413234340601,-3.48610567828749,397.472316630577));
#30040=CARTESIAN_POINT('Ctrl Pts',(2.29659931951241,-3.96225485348206,397.44594067209));
#30041=CARTESIAN_POINT('Ctrl Pts',(1.5982015774714,-4.29180424484795,397.419564713604));
#30042=CARTESIAN_POINT('Ctrl Pts',(0.863491767430947,-4.43485642328811,
397.393188755117));
#30043=CARTESIAN_POINT('Ctrl Pts',(0.128781957390508,-4.57790860172826,
397.366812796631));
#30044=CARTESIAN_POINT('Ctrl Pts',(-0.642239920649369,-4.53446356724268,
397.340436838144));
#30045=CARTESIAN_POINT('Ctrl Pts',(-1.35622885827011,-4.30978106306993,
397.314060879658));
#30046=CARTESIAN_POINT('Ctrl Pts',(-2.07021779589086,-4.08509855889717,
397.287684921171));
#30047=CARTESIAN_POINT('Ctrl Pts',(-2.72717379309247,-3.67917858503723,
397.261308962684));
#30048=CARTESIAN_POINT('Ctrl Pts',(-3.24756141147036,-3.14116449845108,
397.234933004198));
#30049=CARTESIAN_POINT('Ctrl Pts',(-3.76794902984825,-2.60315041186493,
397.208557045711));
#30050=CARTESIAN_POINT('Ctrl Pts',(-4.15176826940243,-1.93304221255256,
397.182181087224));
#30051=CARTESIAN_POINT('Ctrl Pts',(-4.35255143425054,-1.21196763150028,
397.155805128738));
#30052=CARTESIAN_POINT('Ctrl Pts',(-4.46222473223498,-0.818096823374597,
397.141397853322));
#30053=CARTESIAN_POINT('Ctrl Pts',(-4.51728655488816,-0.409019453899831,
397.126990577907));
#30054=CARTESIAN_POINT('Ctrl Pts',(-4.51738673749921,3.14726202902737E-5,
397.112583302492));
#30055=CARTESIAN_POINT('Ctrl Pts',(-4.51813440218219,-1.34914224690988E-5,
397.387416697508));
#30056=CARTESIAN_POINT('Ctrl Pts',(-4.51813661921663,-0.0129106614282636,
397.387871168281));
#30057=CARTESIAN_POINT('Ctrl Pts',(-4.51808254311073,-0.0258078127678308,
397.388325639054));
#30058=CARTESIAN_POINT('Ctrl Pts',(-4.51797206016886,-0.0387044808823415,
397.388780109827));
#30059=CARTESIAN_POINT('Ctrl Pts',(-4.51156000099881,-0.787183817589628,
397.415156068314));
#30060=CARTESIAN_POINT('Ctrl Pts',(-4.31515550083941,-1.5340355305086,397.4415320268));
#30061=CARTESIAN_POINT('Ctrl Pts',(-3.95253658758193,-2.18884081128186,
397.467907985287));
#30062=CARTESIAN_POINT('Ctrl Pts',(-3.58991767432445,-2.84364609205511,
397.494283943774));
#30063=CARTESIAN_POINT('Ctrl Pts',(-3.06108434796891,-3.40640494068263,
397.52065990226));
#30064=CARTESIAN_POINT('Ctrl Pts',(-2.43006066892999,-3.80898604862584,
397.547035860747));
#30065=CARTESIAN_POINT('Ctrl Pts',(-1.79903698989108,-4.21156715656904,
397.573411819233));
#30066=CARTESIAN_POINT('Ctrl Pts',(-1.0658229581688,-4.45397052382792,397.59978777772));
#30067=CARTESIAN_POINT('Ctrl Pts',(-0.319186314229528,-4.5068491954042,
397.626163736207));
#30068=CARTESIAN_POINT('Ctrl Pts',(0.427450329709741,-4.55972786698048,
397.652539694693));
#30069=CARTESIAN_POINT('Ctrl Pts',(1.18750958586602,-4.42308184287416,397.67891565318));
#30070=CARTESIAN_POINT('Ctrl Pts',(1.86897365333732,-4.11345439459799,397.705291611666));
#30071=CARTESIAN_POINT('Ctrl Pts',(2.55043772080863,-3.80382694632181,397.731667570153));
#30072=CARTESIAN_POINT('Ctrl Pts',(3.15330659959498,-3.32121807387579,397.75804352864));
#30073=CARTESIAN_POINT('Ctrl Pts',(3.60459299560209,-2.72405559953603,397.784419487126));
#30074=CARTESIAN_POINT('Ctrl Pts',(4.0558793916092,-2.12689312519627,397.810795445613));
#30075=CARTESIAN_POINT('Ctrl Pts',(4.35558330483707,-1.41517704896277,397.837171404099));
#30076=CARTESIAN_POINT('Ctrl Pts',(4.46742059718259,-0.675072426614591,
397.863547362586));
#30077=CARTESIAN_POINT('Ctrl Pts',(4.57925788952811,0.065032195733587,397.889923321072));
#30078=CARTESIAN_POINT('Ctrl Pts',(4.50322856099129,0.833525364196443,397.916299279559));
#30079=CARTESIAN_POINT('Ctrl Pts',(4.24853722497469,1.53736821266419,397.942675238046));
#30080=CARTESIAN_POINT('Ctrl Pts',(3.9938458889581,2.24121106113193,397.969051196532));
#30081=CARTESIAN_POINT('Ctrl Pts',(3.56049254546173,2.88040358960456,397.995427155019));
#30082=CARTESIAN_POINT('Ctrl Pts',(3.00094181663071,3.37756092269383,398.021803113505));
#30083=CARTESIAN_POINT('Ctrl Pts',(2.44139108779969,3.87471825578309,398.048179071992));
#30084=CARTESIAN_POINT('Ctrl Pts',(1.75564297363402,4.22984039348899,398.074555030479));
#30085=CARTESIAN_POINT('Ctrl Pts',(1.02671867666087,4.39993390090012,398.100930988965));
#30086=CARTESIAN_POINT('Ctrl Pts',(0.297794379687701,4.57002740831124,398.127306947452));
#30087=CARTESIAN_POINT('Ctrl Pts',(-0.474306100092957,4.55509228542758,
398.153682905938));
#30088=CARTESIAN_POINT('Ctrl Pts',(-1.19610717160092,4.35693667699891,398.180058864425));
#30089=CARTESIAN_POINT('Ctrl Pts',(-1.91790824310887,4.15878106857024,398.206434822912));
#30090=CARTESIAN_POINT('Ctrl Pts',(-2.58940990634414,3.77740497459655,398.232810781398));
#30091=CARTESIAN_POINT('Ctrl Pts',(-3.12931572836207,3.25898030762527,398.259186739885));
#30092=CARTESIAN_POINT('Ctrl Pts',(-3.66922155038001,2.74055564065398,398.285562698372));
#30093=CARTESIAN_POINT('Ctrl Pts',(-4.07753153118063,2.08508240068509,398.311938656858));
#30094=CARTESIAN_POINT('Ctrl Pts',(-4.30481296375181,1.37191651366358,398.338314615345));
#30095=CARTESIAN_POINT('Ctrl Pts',(-4.44585038591782,0.929367920299095,
398.354681976066));
#30096=CARTESIAN_POINT('Ctrl Pts',(-4.51717896496231,0.464603561951737,
398.371049336787));
#30097=CARTESIAN_POINT('Ctrl Pts',(-4.51746064445937,-7.62825515632226E-5,
398.387416697508));
#30098=CARTESIAN_POINT('Origin',(0.,0.,387.));
#30099=CARTESIAN_POINT('',(-4.51769110620511,0.00011483889287206,399.387416697508));
#30100=CARTESIAN_POINT('',(-4.51766328535307,-0.00011344722995056,399.112583302492));
#30101=CARTESIAN_POINT('',(-4.51775,5.53264807684796E-16,387.));
#30102=CARTESIAN_POINT('',(3.43378788736219,2.93584158412962,400.));
#30103=CARTESIAN_POINT('Ctrl Pts',(-4.51769110620511,0.00011483889287206,
399.387416697508));
#30104=CARTESIAN_POINT('Ctrl Pts',(-4.51714363756808,-0.555201766580607,
399.406979422266));
#30105=CARTESIAN_POINT('Ctrl Pts',(-4.41453063358526,-1.11071503909854,
399.426542147024));
#30106=CARTESIAN_POINT('Ctrl Pts',(-4.21442463507641,-1.62855553809715,
399.446104871782));
#30107=CARTESIAN_POINT('Ctrl Pts',(-3.94462645640127,-2.32674761887018,
399.472480830268));
#30108=CARTESIAN_POINT('Ctrl Pts',(-3.49760073249453,-2.95645628495937,
399.498856788754));
#30109=CARTESIAN_POINT('Ctrl Pts',(-2.92746753734289,-3.44144015063649,
399.525232747241));
#30110=CARTESIAN_POINT('Ctrl Pts',(-2.35733434219124,-3.92642401631361,
399.551608705728));
#30111=CARTESIAN_POINT('Ctrl Pts',(-1.66409367579469,-4.26668308157866,
399.577984664215));
#30112=CARTESIAN_POINT('Ctrl Pts',(-0.931673462414912,-4.42103326728196,
399.604360622701));
#30113=CARTESIAN_POINT('Ctrl Pts',(-0.199253249035141,-4.57538345298525,
399.630736581188));
#30114=CARTESIAN_POINT('Ctrl Pts',(0.572346511327848,-4.5438247591268,399.657112539674));
#30115=CARTESIAN_POINT('Ctrl Pts',(1.28970997251907,-4.33015694611576,399.683488498161));
#30116=CARTESIAN_POINT('Ctrl Pts',(2.00707343371029,-4.11648913310473,399.709864456647));
#30117=CARTESIAN_POINT('Ctrl Pts',(2.67020059572975,-3.72071220094113,399.736240415134));
#30118=CARTESIAN_POINT('Ctrl Pts',(3.19881015567137,-3.19078644074148,399.762616373621));
#30119=CARTESIAN_POINT('Ctrl Pts',(3.72741971561299,-2.66086068054184,399.788992332107));
#30120=CARTESIAN_POINT('Ctrl Pts',(4.12151167347679,-1.99678609230616,399.815368290594));
#30121=CARTESIAN_POINT('Ctrl Pts',(4.33336809368492,-1.27886829832022,399.84174424908));
#30122=CARTESIAN_POINT('Ctrl Pts',(4.54522451389304,-0.560950504334284,
399.868120207567));
#30123=CARTESIAN_POINT('Ctrl Pts',(4.57484539644551,0.210810495401909,399.894496166054));
#30124=CARTESIAN_POINT('Ctrl Pts',(4.41862185200597,0.942742363213577,399.92087212454));
#30125=CARTESIAN_POINT('Ctrl Pts',(4.26239830756643,1.67467423102524,399.947248083027));
#30126=CARTESIAN_POINT('Ctrl Pts',(3.92033033613488,2.36677696691239,399.973624041513));
#30127=CARTESIAN_POINT('Ctrl Pts',(3.43378788736214,2.93584158412968,400.));
#30128=CARTESIAN_POINT('',(-3.43408816619742,2.93604416807593,400.));
#30129=CARTESIAN_POINT('Origin',(0.,0.,400.));
#30130=CARTESIAN_POINT('Ctrl Pts',(-3.43408816619742,2.93604416807593,400.));
#30131=CARTESIAN_POINT('Ctrl Pts',(-2.97450238708434,3.47304931101404,399.975093589943));
#30132=CARTESIAN_POINT('Ctrl Pts',(-2.38685943846713,3.90077490879642,399.950187179887));
#30133=CARTESIAN_POINT('Ctrl Pts',(-1.73419289785415,4.17206489997238,399.92528076983));
#30134=CARTESIAN_POINT('Ctrl Pts',(-1.04301719081029,4.45936176567177,399.898904811344));
#30135=CARTESIAN_POINT('Ctrl Pts',(-0.278918372417421,4.57121813647734,
399.872528852857));
#30136=CARTESIAN_POINT('Ctrl Pts',(0.465602633104777,4.49408395991645,399.84615289437));
#30137=CARTESIAN_POINT('Ctrl Pts',(1.21012363862699,4.41694978335555,399.819776935884));
#30138=CARTESIAN_POINT('Ctrl Pts',(1.93506683127852,4.15082505942817,399.793400977397));
#30139=CARTESIAN_POINT('Ctrl Pts',(2.55266298782158,3.72793237180886,399.767025018911));
#30140=CARTESIAN_POINT('Ctrl Pts',(3.17025914436463,3.30503968418955,399.740649060424));
#30141=CARTESIAN_POINT('Ctrl Pts',(3.68050826479921,2.72537903287831,399.714273101937));
#30142=CARTESIAN_POINT('Ctrl Pts',(4.02163754117277,2.05912619043133,399.687897143451));
#30143=CARTESIAN_POINT('Ctrl Pts',(4.36276681754633,1.39287334798434,399.661521184964));
#30144=CARTESIAN_POINT('Ctrl Pts',(4.53477624985888,0.640028314401621,399.635145226478));
#30145=CARTESIAN_POINT('Ctrl Pts',(4.51684061200005,-0.108263669819661,
399.608769267991));
#30146=CARTESIAN_POINT('Ctrl Pts',(4.49890497414122,-0.856555654040941,
399.582393309504));
#30147=CARTESIAN_POINT('Ctrl Pts',(4.29102426611101,-1.60029458890078,399.556017351018));
#30148=CARTESIAN_POINT('Ctrl Pts',(3.91836619751067,-2.24943891706491,399.529641392531));
#30149=CARTESIAN_POINT('Ctrl Pts',(3.54570812891033,-2.89858324522903,399.503265434045));
#30150=CARTESIAN_POINT('Ctrl Pts',(3.00827269973986,-3.45313296669745,399.476889475558));
#30151=CARTESIAN_POINT('Ctrl Pts',(2.37112525795217,-3.84595043629749,399.450513517072));
#30152=CARTESIAN_POINT('Ctrl Pts',(1.73397781616448,-4.23876790589754,399.424137558585));
#30153=CARTESIAN_POINT('Ctrl Pts',(0.99711836175957,-4.4698531236292,399.397761600098));
#30154=CARTESIAN_POINT('Ctrl Pts',(0.249756040315393,-4.51122947332523,
399.371385641612));
#30155=CARTESIAN_POINT('Ctrl Pts',(-0.497606281128785,-4.55260582302126,
399.345009683125));
#30156=CARTESIAN_POINT('Ctrl Pts',(-1.25547146961223,-4.40427330468165,
399.318633724638));
#30157=CARTESIAN_POINT('Ctrl Pts',(-1.93208738383067,-4.08418999214993,
399.292257766152));
#30158=CARTESIAN_POINT('Ctrl Pts',(-2.60870329804912,-3.7641066796182,399.265881807665));
#30159=CARTESIAN_POINT('Ctrl Pts',(-3.20406993800257,-3.27227257289437,
399.239505849179));
#30160=CARTESIAN_POINT('Ctrl Pts',(-3.64610826548277,-2.6682323819666,399.213129890692));
#30161=CARTESIAN_POINT('Ctrl Pts',(-4.08814659296297,-2.06419219103883,
399.186753932205));
#30162=CARTESIAN_POINT('Ctrl Pts',(-4.37685660796992,-1.34794591590712,
399.160377973719));
#30163=CARTESIAN_POINT('Ctrl Pts',(-4.47728517341772,-0.606207058821207,
399.134002015232));
#30164=CARTESIAN_POINT('Ctrl Pts',(-4.50446965905899,-0.405429628414596,
399.126862444319));
#30165=CARTESIAN_POINT('Ctrl Pts',(-4.51785871427772,-0.20278434994614,
399.119722873405));
#30166=CARTESIAN_POINT('Ctrl Pts',(-4.51766328535307,-0.00011344722995056,
399.112583302492));
#30167=CARTESIAN_POINT('Origin',(0.,0.,402.208336844637));
#30168=CARTESIAN_POINT('',(-5.07399177313997,5.16404304284901E-5,375.791663155363));
#30169=CARTESIAN_POINT('',(-5.07400718786956,-4.16755268873004E-5,375.708336844637));
#30170=CARTESIAN_POINT('',(-5.0736,-1.59740085886799E-13,402.208336844637));
#30171=CARTESIAN_POINT('',(1.3130361863572,-4.90075024188303,375.));
#30172=CARTESIAN_POINT('Ctrl Pts',(-5.07400718786956,-4.16755268873182E-5,
375.708336844637));
#30173=CARTESIAN_POINT('Ctrl Pts',(-5.07365763063996,0.800054575924722,
375.683232230984));
#30174=CARTESIAN_POINT('Ctrl Pts',(-4.67875473787853,2.4410987772414,375.631751658845));
#30175=CARTESIAN_POINT('Ctrl Pts',(-2.98728944096456,4.36266186682328,375.553895128218));
#30176=CARTESIAN_POINT('Ctrl Pts',(-0.544875549618088,5.2592655277028,375.474767252759));
#30177=CARTESIAN_POINT('Ctrl Pts',(2.02945798133318,4.88240903418803,375.395639377299));
#30178=CARTESIAN_POINT('Ctrl Pts',(4.1124194375256,3.3233956145555,375.316511501839));
#30179=CARTESIAN_POINT('Ctrl Pts',(5.19956989745793,0.959601216722932,375.237383626379));
#30180=CARTESIAN_POINT('Ctrl Pts',(5.02785240284651,-1.63637626402564,375.15825575092));
#30181=CARTESIAN_POINT('Ctrl Pts',(3.63845954881624,-3.83644847785649,375.07912787546));
#30182=CARTESIAN_POINT('Ctrl Pts',(2.1252131908655,-4.68314727417153,375.026375958487));
#30183=CARTESIAN_POINT('Ctrl Pts',(1.3130361863572,-4.90075024188303,375.));
#30184=CARTESIAN_POINT('',(-1.31318542874413,-4.90112866933894,375.));
#30185=CARTESIAN_POINT('Origin',(0.,0.,375.));
#30186=CARTESIAN_POINT('Ctrl Pts',(-5.07399177313997,5.16404304287937E-5,
375.791663155363));
#30187=CARTESIAN_POINT('Ctrl Pts',(-5.07401862443284,0.0509709830336597,
375.790065473344));
#30188=CARTESIAN_POINT('Ctrl Pts',(-5.06087568855098,0.942498320863251,
375.762091832839));
#30189=CARTESIAN_POINT('Ctrl Pts',(-4.56924148341307,2.66059337382158,375.707742233848));
#30190=CARTESIAN_POINT('Ctrl Pts',(-2.74710339271414,4.51775908713646,375.628614358388));
#30191=CARTESIAN_POINT('Ctrl Pts',(-0.25980027835232,5.28102544478076,375.549486482929));
#30192=CARTESIAN_POINT('Ctrl Pts',(2.29040909674433,4.76557955369675,375.470358607468));
#30193=CARTESIAN_POINT('Ctrl Pts',(4.28603436317887,3.09622956904483,375.391230732009));
#30194=CARTESIAN_POINT('Ctrl Pts',(5.24386820297344,0.677177255244125,375.312102856549));
#30195=CARTESIAN_POINT('Ctrl Pts',(4.93198748823577,-1.90583737857549,375.232974981089));
#30196=CARTESIAN_POINT('Ctrl Pts',(3.42590832840442,-4.02739560248487,375.153847105629));
#30197=CARTESIAN_POINT('Ctrl Pts',(1.13368018117025,-5.15247588128094,375.0761887786));
#30198=CARTESIAN_POINT('Ctrl Pts',(-0.546344062323364,-5.10618409554666,
375.024906410057));
#30199=CARTESIAN_POINT('Ctrl Pts',(-1.31318542874413,-4.90112866933894,
375.));
#30200=CARTESIAN_POINT('Origin',(0.,0.,402.208336844637));
#30201=CARTESIAN_POINT('',(-5.07342806457247,-0.000120553681964564,376.791663155363));
#30202=CARTESIAN_POINT('',(-5.0732320111606,-6.61733612274322E-5,376.708336844637));
#30203=CARTESIAN_POINT('',(-5.0736,-1.59740085886799E-13,402.208336844637));
#30204=CARTESIAN_POINT('Ctrl Pts',(-5.0732320111606,-6.61733612272383E-5,
376.708336844637));
#30205=CARTESIAN_POINT('Ctrl Pts',(-5.07300240190748,0.495753489740335,
376.692786357976));
#30206=CARTESIAN_POINT('Ctrl Pts',(-4.87836138639172,1.83273410665417,376.650859912829));
#30207=CARTESIAN_POINT('Ctrl Pts',(-3.72041242686768,3.75702756739127,376.582557509196));
#30208=CARTESIAN_POINT('Ctrl Pts',(-1.47810086816716,5.0766073897426,376.503429633736));
#30209=CARTESIAN_POINT('Ctrl Pts',(1.12210802704861,5.16697187426544,376.424301758276));
#30210=CARTESIAN_POINT('Ctrl Pts',(3.45061728097363,4.00624077340234,376.345173882816));
#30211=CARTESIAN_POINT('Ctrl Pts',(4.94361743453053,1.87546566308182,376.266046007357));
#30212=CARTESIAN_POINT('Ctrl Pts',(5.23960352937691,-0.709422013391795,
376.186918131896));
#30213=CARTESIAN_POINT('Ctrl Pts',(4.2669075188957,-3.12253502690154,376.107790256437));
#30214=CARTESIAN_POINT('Ctrl Pts',(2.26105138176727,-4.77957859502704,376.028662380977));
#30215=CARTESIAN_POINT('Ctrl Pts',(-0.292280359441297,-5.27932727476591,
375.949534505517));
#30216=CARTESIAN_POINT('Ctrl Pts',(-2.77484145645776,-4.50077558721857,
375.870406630058));
#30217=CARTESIAN_POINT('Ctrl Pts',(-4.58552092957851,-2.63243616845826,
375.791278754598));
#30218=CARTESIAN_POINT('Ctrl Pts',(-5.06368921675185,-0.921683996926001,
375.737255492791));
#30219=CARTESIAN_POINT('Ctrl Pts',(-5.07402489010486,-0.0405600539318397,
375.709608189471));
#30220=CARTESIAN_POINT('Ctrl Pts',(-5.07400718786956,-4.16755268873182E-5,
375.708336844637));
#30221=CARTESIAN_POINT('Ctrl Pts',(-5.07342806457247,-0.000120553681964737,
376.791663155363));
#30222=CARTESIAN_POINT('Ctrl Pts',(-5.07290494961689,0.587111569129446,
376.77324364185));
#30223=CARTESIAN_POINT('Ctrl Pts',(-4.82510106239333,2.01566514286781,376.728448169851));
#30224=CARTESIAN_POINT('Ctrl Pts',(-3.51189274247934,3.95263634434836,376.657276739365));
#30225=CARTESIAN_POINT('Ctrl Pts',(-1.20153141562281,5.1490821475793,376.578148863906));
#30226=CARTESIAN_POINT('Ctrl Pts',(1.39976059245402,5.09876406487689,376.499020988446));
#30227=CARTESIAN_POINT('Ctrl Pts',(3.66212404867255,3.81386577598244,376.419893112986));
#30228=CARTESIAN_POINT('Ctrl Pts',(5.03776558457334,1.60550385251465,376.340765237526));
#30229=CARTESIAN_POINT('Ctrl Pts',(5.19359667332446,-0.99160390296118,376.261637362067));
#30230=CARTESIAN_POINT('Ctrl Pts',(4.09188543028651,-3.34861140308599,376.182509486607));
#30231=CARTESIAN_POINT('Ctrl Pts',(1.99939275591558,-4.89480881330613,376.103381611147));
#30232=CARTESIAN_POINT('Ctrl Pts',(-0.577219342064538,-5.2558103583336,
376.024253735687));
#30233=CARTESIAN_POINT('Ctrl Pts',(-3.01406745721832,-4.34420557675964,
375.945125860227));
#30234=CARTESIAN_POINT('Ctrl Pts',(-4.68664255775979,-2.42036918652462,
375.867595666786));
#30235=CARTESIAN_POINT('Ctrl Pts',(-5.0735753393625,-0.789650899948463,
375.816441431831));
#30236=CARTESIAN_POINT('Ctrl Pts',(-5.07399177313997,5.16404304287937E-5,
375.791663155363));
#30237=CARTESIAN_POINT('Origin',(0.,0.,402.208336844637));
#30238=CARTESIAN_POINT('',(-5.07335325700037,0.000107956674043064,377.791663155363));
#30239=CARTESIAN_POINT('',(-5.07361435362778,0.000129215856731547,377.708336844637));
#30240=CARTESIAN_POINT('',(-5.0736,-1.59740085886799E-13,402.208336844637));
#30241=CARTESIAN_POINT('Ctrl Pts',(-5.07361435362778,0.000129215856731774,
377.708336844637));
#30242=CARTESIAN_POINT('Ctrl Pts',(-5.07380906160703,0.191278857423315,
377.702340484969));
#30243=CARTESIAN_POINT('Ctrl Pts',(-5.01660264728387,1.22311525648581,377.669968166814));
#30244=CARTESIAN_POINT('Ctrl Pts',(-4.33319923422642,3.02986949626759,377.611219890172));
#30245=CARTESIAN_POINT('Ctrl Pts',(-2.36351373006459,4.72974921277116,377.532092014713));
#30246=CARTESIAN_POINT('Ctrl Pts',(0.178456984968689,5.28439948077629,377.452964139253));
#30247=CARTESIAN_POINT('Ctrl Pts',(2.67721733402229,4.55952104001336,377.373836263793));
#30248=CARTESIAN_POINT('Ctrl Pts',(4.52773440567874,2.73063104786141,377.294708388334));
#30249=CARTESIAN_POINT('Ctrl Pts',(5.28193652635228,0.240564543316707,377.215580512874));
#30250=CARTESIAN_POINT('Ctrl Pts',(4.75720630136386,-2.3077506308472,377.136452637414));
#30251=CARTESIAN_POINT('Ctrl Pts',(3.08059835436342,-4.29728269340077,377.057324761954));
#30252=CARTESIAN_POINT('Ctrl Pts',(0.658075181053442,-5.24629982216222,
376.978196886494));
#30253=CARTESIAN_POINT('Ctrl Pts',(-1.923789860657,-4.92501343550216,376.899069011035));
#30254=CARTESIAN_POINT('Ctrl Pts',(-4.03984145181191,-3.4112176436405,376.819941135575));
#30255=CARTESIAN_POINT('Ctrl Pts',(-4.95409465736432,-1.5312714924381,376.756363746775));
#30256=CARTESIAN_POINT('Ctrl Pts',(-5.07339185365009,-0.345231048960516,
376.719162316463));
#30257=CARTESIAN_POINT('Ctrl Pts',(-5.0732320111606,-6.61733612272383E-5,
376.708336844637));
#30258=CARTESIAN_POINT('Ctrl Pts',(-5.07335325700037,0.00010795667404348,
377.791663155363));
#30259=CARTESIAN_POINT('Ctrl Pts',(-5.07357381709386,0.28275711441475,377.782797768842));
#30260=CARTESIAN_POINT('Ctrl Pts',(-4.98125011308217,1.40619065190393,377.747556423836));
#30261=CARTESIAN_POINT('Ctrl Pts',(-4.16308913613231,3.25966463764834,377.685939120343));
#30262=CARTESIAN_POINT('Ctrl Pts',(-2.1043987453421,4.85059075019948,377.606811244883));
#30263=CARTESIAN_POINT('Ctrl Pts',(0.463836508427624,5.26702766261653,377.527683369423));
#30264=CARTESIAN_POINT('Ctrl Pts',(2.91976153075723,4.40814216068722,377.448555493963));
#30265=CARTESIAN_POINT('Ctrl Pts',(4.66871526619766,2.48189896419878,377.369427618503));
#30266=CARTESIAN_POINT('Ctrl Pts',(5.28721789969248,-0.0452944421492617,
377.290299743044));
#30267=CARTESIAN_POINT('Ctrl Pts',(4.62550939154664,-2.56152055897115,377.211171867584));
#30268=CARTESIAN_POINT('Ctrl Pts',(2.84381135938942,-4.45751743210561,377.132043992124));
#30269=CARTESIAN_POINT('Ctrl Pts',(0.373532100567371,-5.27420121678766,
377.052916116664));
#30270=CARTESIAN_POINT('Ctrl Pts',(-2.18719169184094,-4.81382563128935,
376.973788241204));
#30271=CARTESIAN_POINT('Ctrl Pts',(-4.21832369780876,-3.18786290260816,
376.894660365745));
#30272=CARTESIAN_POINT('Ctrl Pts',(-4.99301148124094,-1.34818805955531,
376.833952003797));
#30273=CARTESIAN_POINT('Ctrl Pts',(-5.07365402794313,-0.253779808523861,
376.799619600337));
#30274=CARTESIAN_POINT('Ctrl Pts',(-5.07342806457247,-0.000120553681964737,
376.791663155363));
#30275=CARTESIAN_POINT('Origin',(0.,0.,402.208336844637));
#30276=CARTESIAN_POINT('',(-5.07402683453791,-2.287789782323E-5,378.791663155363));
#30277=CARTESIAN_POINT('',(-5.07385055213498,-0.000101541417780425,378.708336844637));
#30278=CARTESIAN_POINT('',(-5.0736,-1.59740085886799E-13,402.208336844637));
#30279=CARTESIAN_POINT('Ctrl Pts',(-5.07385055213498,-0.000101541417780338,
378.708336844637));
#30280=CARTESIAN_POINT('Ctrl Pts',(-5.07319426513103,0.727190265934581,
378.685518653475));
#30281=CARTESIAN_POINT('Ctrl Pts',(-4.73238867060224,2.2957670138656,378.636324503826));
#30282=CARTESIAN_POINT('Ctrl Pts',(-3.17247821056078,4.22990623671853,378.56075439569));
#30283=CARTESIAN_POINT('Ctrl Pts',(-0.770966287939471,5.23090200164121,
378.48162652023));
#30284=CARTESIAN_POINT('Ctrl Pts',(1.81722219130848,4.96532257515351,378.40249864477));
#30285=CARTESIAN_POINT('Ctrl Pts',(3.96540079385267,3.49747356130477,378.323370769311));
#30286=CARTESIAN_POINT('Ctrl Pts',(5.15342409853101,1.18276998126983,378.244242893851));
#30287=CARTESIAN_POINT('Ctrl Pts',(5.09363218664291,-1.41832151330666,378.165115018391));
#30288=CARTESIAN_POINT('Ctrl Pts',(3.80050266687247,-3.67599024033094,378.085987142931));
#30289=CARTESIAN_POINT('Ctrl Pts',(1.58714516515185,-5.04357958127442,378.006859267472));
#30290=CARTESIAN_POINT('Ctrl Pts',(-1.01051292004705,-5.18995071328536,
377.927731392012));
#30291=CARTESIAN_POINT('Ctrl Pts',(-3.36349224912901,-4.07966232156074,
377.848603516552));
#30292=CARTESIAN_POINT('Ctrl Pts',(-4.78546484347183,-2.14054821676427,
377.77547200076));
#30293=CARTESIAN_POINT('Ctrl Pts',(-5.07295260704762,-0.649523777787379,
377.728716443455));
#30294=CARTESIAN_POINT('Ctrl Pts',(-5.07361435362778,0.000129215856731774,
377.708336844637));
#30295=CARTESIAN_POINT('Ctrl Pts',(-5.07402683453791,-2.28778978229567E-5,
378.791663155363));
#30296=CARTESIAN_POINT('Ctrl Pts',(-5.07381925213896,0.818631858438491,
378.765975937348));
#30297=CARTESIAN_POINT('Ctrl Pts',(-4.66448051806342,2.47809170659261,378.713912760847));
#30298=CARTESIAN_POINT('Ctrl Pts',(-2.9391988257698,4.39520590733944,378.63547362586));
#30299=CARTESIAN_POINT('Ctrl Pts',(-0.487090471470337,5.2649280695866,378.5563457504));
#30300=CARTESIAN_POINT('Ctrl Pts',(2.08295867142411,4.85983619872698,378.47721787494));
#30301=CARTESIAN_POINT('Ctrl Pts',(4.1486543056634,3.27801649742928,378.398089999481));
#30302=CARTESIAN_POINT('Ctrl Pts',(5.20982287752563,0.902480077413658,378.318962124021));
#30303=CARTESIAN_POINT('Ctrl Pts',(5.00952021436078,-1.69157675771122,378.239834248561));
#30304=CARTESIAN_POINT('Ctrl Pts',(3.59624624674644,-3.8760466506584,378.160706373101));
#30305=CARTESIAN_POINT('Ctrl Pts',(1.31220156369858,-5.12199685294173,378.081578497641));
#30306=CARTESIAN_POINT('Ctrl Pts',(-1.28957072085835,-5.12774141910675,
378.002450622182));
#30307=CARTESIAN_POINT('Ctrl Pts',(-3.57909508295452,-3.89188939879962,
377.923322746722));
#30308=CARTESIAN_POINT('Ctrl Pts',(-4.84258096039032,-1.9577252596909,377.853060257782));
#30309=CARTESIAN_POINT('Ctrl Pts',(-5.07291761514975,-0.558169836019873,
377.809173727329));
#30310=CARTESIAN_POINT('Ctrl Pts',(-5.07335325700037,0.00010795667404348,
377.791663155363));
#30311=CARTESIAN_POINT('Origin',(0.,0.,402.208336844637));
#30312=CARTESIAN_POINT('',(-5.07326152951467,-8.03441847486985E-5,379.791663155363));
#30313=CARTESIAN_POINT('',(-5.07317735229637,-2.23272941127382E-6,379.708336844637));
#30314=CARTESIAN_POINT('',(-5.0736,-1.59740085886799E-13,402.208336844637));
#30315=CARTESIAN_POINT('Ctrl Pts',(-5.07317735229636,-2.23272941118208E-6,
379.708336844637));
#30316=CARTESIAN_POINT('Ctrl Pts',(-5.07317083223754,0.422929008539474,
379.695072780467));
#30317=CARTESIAN_POINT('Ctrl Pts',(-4.91684325738401,1.68687545589345,379.65543275781));
#30318=CARTESIAN_POINT('Ctrl Pts',(-3.87882817196482,3.59324599495851,379.589416776668));
#30319=CARTESIAN_POINT('Ctrl Pts',(-1.69545248338881,5.00820982432685,379.510288901207));
#30320=CARTESIAN_POINT('Ctrl Pts',(0.898448589337301,5.21051963821565,379.431161025747));
#30321=CARTESIAN_POINT('Ctrl Pts',(3.27480540417913,4.15118950816177,379.352033150288));
#30322=CARTESIAN_POINT('Ctrl Pts',(4.85822301267979,2.08671845896413,379.272905274828));
#30323=CARTESIAN_POINT('Ctrl Pts',(5.26530339668872,-0.483016468385486,
379.193777399368));
#30324=CARTESIAN_POINT('Ctrl Pts',(4.39747886842774,-2.93579705866137,379.114649523908));
#30325=CARTESIAN_POINT('Ctrl Pts',(2.4648785829925,-4.67772362790043,379.035521648449));
#30326=CARTESIAN_POINT('Ctrl Pts',(-0.0645507124447473,-5.28701787148826,
378.956393772989));
#30327=CARTESIAN_POINT('Ctrl Pts',(-2.57835013545374,-4.61614940691036,
378.877265897529));
#30328=CARTESIAN_POINT('Ctrl Pts',(-4.46784531508162,-2.82755778162292,
378.798138022069));
#30329=CARTESIAN_POINT('Ctrl Pts',(-5.04261473172305,-1.0675305862618,378.741828337772));
#30330=CARTESIAN_POINT('Ctrl Pts',(-5.07395287910916,-0.113499444385656,
378.711894611961));
#30331=CARTESIAN_POINT('Ctrl Pts',(-5.07385055213498,-0.000101541417780338,
378.708336844637));
#30332=CARTESIAN_POINT('Ctrl Pts',(-5.07326152951467,-8.03441847485598E-5,
379.791663155363));
#30333=CARTESIAN_POINT('Ctrl Pts',(-5.07297012272296,0.514306801455685,
379.775530064341));
#30334=CARTESIAN_POINT('Ctrl Pts',(-4.86799754311315,1.86989152588461,379.733021014832));
#30335=CARTESIAN_POINT('Ctrl Pts',(-3.67892986111526,3.7976571438602,379.664136006837));
#30336=CARTESIAN_POINT('Ctrl Pts',(-1.42226240084736,5.09253319757995,379.585008131377));
#30337=CARTESIAN_POINT('Ctrl Pts',(1.17878204679748,5.15433774518764,379.505880255918));
#30338=CARTESIAN_POINT('Ctrl Pts',(3.49440419135096,3.9681058520139,379.426752380457));
#30339=CARTESIAN_POINT('Ctrl Pts',(4.96391496617568,1.82106367650753,379.347624504998));
#30340=CARTESIAN_POINT('Ctrl Pts',(5.2314969825461,-0.766918526917405,379.268496629538));
#30341=CARTESIAN_POINT('Ctrl Pts',(4.23235974285854,-3.16920427116154,379.189368754078));
#30342=CARTESIAN_POINT('Ctrl Pts',(2.20842757301423,-4.80412035237133,379.110240878619));
#30343=CARTESIAN_POINT('Ctrl Pts',(-0.350238295746339,-5.27579926091873,
379.031113003158));
#30344=CARTESIAN_POINT('Ctrl Pts',(-2.82409983509395,-4.47003185970082,
378.951985127699));
#30345=CARTESIAN_POINT('Ctrl Pts',(-4.61415296279982,-2.58192121126957,
378.872857252239));
#30346=CARTESIAN_POINT('Ctrl Pts',(-5.06855147600533,-0.884525550463806,
378.819416594794));
#30347=CARTESIAN_POINT('Ctrl Pts',(-5.07403240035665,-0.0219731198176094,
378.792351895835));
#30348=CARTESIAN_POINT('Ctrl Pts',(-5.07402683453791,-2.28778978229567E-5,
378.791663155363));
#30349=CARTESIAN_POINT('Origin',(0.,0.,402.208336844637));
#30350=CARTESIAN_POINT('',(-5.07355665554129,0.000129459885802874,380.791663155363));
#30351=CARTESIAN_POINT('',(-5.07383699511133,0.000104483598321417,380.708336844637));
#30352=CARTESIAN_POINT('',(-5.0736,-1.59740085886799E-13,402.208336844637));
#30353=CARTESIAN_POINT('Ctrl Pts',(-5.07383699511133,0.000104483598321794,
380.708336844637));
#30354=CARTESIAN_POINT('Ctrl Pts',(-5.07394580731281,0.118353460768718,
380.704626907459));
#30355=CARTESIAN_POINT('Ctrl Pts',(-5.04109883614377,1.0772383012794,380.674541011795));
#30356=CARTESIAN_POINT('Ctrl Pts',(-4.45971656638884,2.84036140577044,380.618079157644));
#30357=CARTESIAN_POINT('Ctrl Pts',(-2.56509888808806,4.6235259772432,380.538951282184));
#30358=CARTESIAN_POINT('Ctrl Pts',(-0.0493855337170155,5.28718127521391,
380.459823406725));
#30359=CARTESIAN_POINT('Ctrl Pts',(2.47828569939099,4.67063429954727,380.380695531265));
#30360=CARTESIAN_POINT('Ctrl Pts',(4.40588161411396,2.92317156019379,380.301567655805));
#30361=CARTESIAN_POINT('Ctrl Pts',(5.26666718771851,0.467911852513223,380.222439780345));
#30362=CARTESIAN_POINT('Ctrl Pts',(4.8522176299277,-2.10064486282949,380.143311904886));
#30363=CARTESIAN_POINT('Ctrl Pts',(3.26288495036134,-4.1605656548862,380.064184029426));
#30364=CARTESIAN_POINT('Ctrl Pts',(0.883499402425967,-5.21307525111868,
379.985056153966));
#30365=CARTESIAN_POINT('Ctrl Pts',(-1.70981070849824,-5.0033261046046,379.905928278506));
#30366=CARTESIAN_POINT('Ctrl Pts',(-3.88911883186622,-3.58210545343612,
379.826800403046));
#30367=CARTESIAN_POINT('Ctrl Pts',(-4.91928148884334,-1.67716650260946,
379.760936591757));
#30368=CARTESIAN_POINT('Ctrl Pts',(-5.07318379755486,-0.418081463015616,
379.721448738954));
#30369=CARTESIAN_POINT('Ctrl Pts',(-5.07317735229636,-2.23272941118208E-6,
379.708336844637));
#30370=CARTESIAN_POINT('Ctrl Pts',(-5.07355665554129,0.000129459885803325,
380.791663155363));
#30371=CARTESIAN_POINT('Ctrl Pts',(-5.07376606808144,0.209858000324401,
380.785084191333));
#30372=CARTESIAN_POINT('Ctrl Pts',(-5.00984200321542,1.26028988400143,380.752129268817));
#30373=CARTESIAN_POINT('Ctrl Pts',(-4.29966508516876,3.07727230850615,380.692798387814));
#30374=CARTESIAN_POINT('Ctrl Pts',(-2.31143093395199,4.75541919738815,380.613670512354));
#30375=CARTESIAN_POINT('Ctrl Pts',(0.236477452546483,5.28212108151216,380.534542636895));
#30376=CARTESIAN_POINT('Ctrl Pts',(2.7271267899117,4.52984593303835,380.455414761435));
#30377=CARTESIAN_POINT('Ctrl Pts',(4.55744811217567,2.68074456264382,380.376286885975));
#30378=CARTESIAN_POINT('Ctrl Pts',(5.28425980776137,0.182545855597361,380.297159010515));
#30379=CARTESIAN_POINT('Ctrl Pts',(4.73157661405697,-2.35985326887651,380.218031135055));
#30380=CARTESIAN_POINT('Ctrl Pts',(3.03322149728047,-4.33085350176541,380.138903259596));
#30381=CARTESIAN_POINT('Ctrl Pts',(0.600422665576261,-5.25321019263273,
380.059775384136));
#30382=CARTESIAN_POINT('Ctrl Pts',(-1.97775844481349,-4.90359013777528,
379.980647508676));
#30383=CARTESIAN_POINT('Ctrl Pts',(-4.07705851709219,-3.36664796994342,
379.901519633216));
#30384=CARTESIAN_POINT('Ctrl Pts',(-4.96242349460837,-1.49409344074893,
379.838524848778));
#30385=CARTESIAN_POINT('Ctrl Pts',(-5.07344654310827,-0.326663721856642,
379.801906022827));
#30386=CARTESIAN_POINT('Ctrl Pts',(-5.07326152951467,-8.03441847485598E-5,
379.791663155363));
#30387=CARTESIAN_POINT('Origin',(0.,0.,402.208336844637));
#30388=CARTESIAN_POINT('',(-5.07389966860957,-8.89210953775033E-5,381.791663155363));
#30389=CARTESIAN_POINT('',(-5.0736295665075,-0.000128745637012367,381.708336844637));
#30390=CARTESIAN_POINT('',(-5.0736,-1.59740085886799E-13,402.208336844637));
#30391=CARTESIAN_POINT('Ctrl Pts',(-5.0736295665075,-0.000128745637012449,
381.708336844637));
#30392=CARTESIAN_POINT('Ctrl Pts',(-5.07296124918876,0.654369409793758,
381.687805075965));
#30393=CARTESIAN_POINT('Ctrl Pts',(-4.78227571732073,2.15023935796871,381.640897348807));
#30394=CARTESIAN_POINT('Ctrl Pts',(-3.35177659407457,4.08929314568265,381.567613663161));
#30395=CARTESIAN_POINT('Ctrl Pts',(-0.995622270609436,5.1928278483096,381.488485787702));
#30396=CARTESIAN_POINT('Ctrl Pts',(1.60160528794473,5.03900637720777,381.409357912242));
#30397=CARTESIAN_POINT('Ctrl Pts',(3.81103098679937,3.66507402184023,381.330230036782));
#30398=CARTESIAN_POINT('Ctrl Pts',(5.09767944760569,1.40370545962173,381.251102161322));
#30399=CARTESIAN_POINT('Ctrl Pts',(5.15001032416474,-1.1975468378773,381.171974285863));
#30400=CARTESIAN_POINT('Ctrl Pts',(3.95535257236717,-3.50883325283227,381.092846410403));
#30401=CARTESIAN_POINT('Ctrl Pts',(1.8029725310162,-4.97051454281288,381.013718534943));
#30402=CARTESIAN_POINT('Ctrl Pts',(-0.785967070782117,-5.22866909753901,
380.934590659483));
#30403=CARTESIAN_POINT('Ctrl Pts',(-3.18459792796892,-4.22078912113472,
380.855462784024));
#30404=CARTESIAN_POINT('Ctrl Pts',(-4.73582433047741,-2.28608714092918,
380.780044845741));
#30405=CARTESIAN_POINT('Ctrl Pts',(-5.07317220227002,-0.722342746081139,
380.731002865946));
#30406=CARTESIAN_POINT('Ctrl Pts',(-5.07383699511133,0.000104483598321794,
380.708336844637));
#30407=CARTESIAN_POINT('Ctrl Pts',(-5.07389966860957,-8.89210953773471E-5,
381.791663155363));
#30408=CARTESIAN_POINT('Ctrl Pts',(-5.07328829289394,0.745751527323211,
381.768262359839));
#30409=CARTESIAN_POINT('Ctrl Pts',(-4.71908116243226,2.33281964194823,381.718485605828));
#30410=CARTESIAN_POINT('Ctrl Pts',(-3.12583571520092,4.26449009693918,381.642332893332));
#30411=CARTESIAN_POINT('Ctrl Pts',(-0.713476057932961,5.23905302703404,
381.563205017871));
#30412=CARTESIAN_POINT('Ctrl Pts',(1.87163986094335,4.94506713162178,381.484077142412));
#30413=CARTESIAN_POINT('Ctrl Pts',(4.00356957706116,3.45371616479241,381.404949266952));
#30414=CARTESIAN_POINT('Ctrl Pts',(5.16610206459392,1.12610575148009,381.325821391492));
#30415=CARTESIAN_POINT('Ctrl Pts',(5.07774957870228,-1.47417228345499,381.246693516033));
#30416=CARTESIAN_POINT('Ctrl Pts',(3.75990519207135,-3.71750422352859,381.167565640573));
#30417=CARTESIAN_POINT('Ctrl Pts',(1.53166282114666,-5.06070486272762,381.088437765113));
#30418=CARTESIAN_POINT('Ctrl Pts',(-1.0674460141586,-5.17854069330105,381.009309889653));
#30419=CARTESIAN_POINT('Ctrl Pts',(-3.40809069944175,-4.04247974511891,
380.930182014193));
#30420=CARTESIAN_POINT('Ctrl Pts',(-4.79752508832052,-2.10343849769112,
380.857633102763));
#30421=CARTESIAN_POINT('Ctrl Pts',(-5.07292650482488,-0.630972144226672,
380.81146014982));
#30422=CARTESIAN_POINT('Ctrl Pts',(-5.07355665554129,0.000129459885803325,
380.791663155363));
#30423=CARTESIAN_POINT('Origin',(0.,0.,402.208336844637));
#30424=CARTESIAN_POINT('',(-5.0731816081447,-1.92612327425123E-5,382.791663155363));
#30425=CARTESIAN_POINT('',(-5.07322528972955,6.22763117692481E-5,382.708336844637));
#30426=CARTESIAN_POINT('',(-5.0736,-1.59740085886799E-13,402.208336844637));
#30427=CARTESIAN_POINT('Ctrl Pts',(-5.07322528972955,6.22763117691383E-5,
382.708336844637));
#30428=CARTESIAN_POINT('Ctrl Pts',(-5.07337757676184,0.350080340895845,
382.697359202958));
#30429=CARTESIAN_POINT('Ctrl Pts',(-4.95188321010373,1.54098189440445,382.660005602791));
#30430=CARTESIAN_POINT('Ctrl Pts',(-4.03004033454984,3.42279121037416,382.596276044139));
#30431=CARTESIAN_POINT('Ctrl Pts',(-1.90965538190854,4.93051124025298,382.517148168679));
#30432=CARTESIAN_POINT('Ctrl Pts',(0.673120594328623,5.24439066369047,382.438020293219));
#30433=CARTESIAN_POINT('Ctrl Pts',(3.09291170766135,4.28842884242289,382.35889241776));
#30434=CARTESIAN_POINT('Ctrl Pts',(4.76380612269667,2.29409589888282,382.2797645423));
#30435=CARTESIAN_POINT('Ctrl Pts',(5.28122477966896,-0.255713891925586,
382.20063666684));
#30436=CARTESIAN_POINT('Ctrl Pts',(4.51988342850276,-2.74360685242242,382.12150879138));
#30437=CARTESIAN_POINT('Ctrl Pts',(2.66412810880644,-4.56718142707082,382.04238091592));
#30438=CARTESIAN_POINT('Ctrl Pts',(0.16329884807764,-5.28488961607806,381.96325304046));
#30439=CARTESIAN_POINT('Ctrl Pts',(-2.37707049000228,-4.72295041827389,
381.884125165001));
#30440=CARTESIAN_POINT('Ctrl Pts',(-4.3418720751543,-3.0174279860352,381.804997289541));
#30441=CARTESIAN_POINT('Ctrl Pts',(-5.01833358746616,-1.21340586700331,
381.746401182753));
#30442=CARTESIAN_POINT('Ctrl Pts',(-5.07381979723383,-0.186425967023143,
381.714181034452));
#30443=CARTESIAN_POINT('Ctrl Pts',(-5.0736295665075,-0.000128745637012449,
381.708336844637));
#30444=CARTESIAN_POINT('Ctrl Pts',(-5.0731816081447,-1.92612327423736E-5,
382.791663155363));
#30445=CARTESIAN_POINT('Ctrl Pts',(-5.07312283046122,0.441487546406695,
382.777816486831));
#30446=CARTESIAN_POINT('Ctrl Pts',(-4.90736705066614,1.72404611325897,382.737593859813));
#30447=CARTESIAN_POINT('Ctrl Pts',(-3.83913463932894,3.63562510806912,382.670995274309));
#30448=CARTESIAN_POINT('Ctrl Pts',(-1.64035202533435,5.0265266276326,382.591867398849));
#30449=CARTESIAN_POINT('Ctrl Pts',(0.955614320991023,5.2003390249901,382.512739523389));
#30450=CARTESIAN_POINT('Ctrl Pts',(3.32019468624774,4.11497654315675,382.433611647929));
#30451=CARTESIAN_POINT('Ctrl Pts',(4.8808455917412,2.03324150432223,382.354483772469));
#30452=CARTESIAN_POINT('Ctrl Pts',(5.25968159463003,-0.540808864968189,
382.27535589701));
#30453=CARTESIAN_POINT('Ctrl Pts',(4.36497391033337,-2.98391143759783,382.19622802155));
#30454=CARTESIAN_POINT('Ctrl Pts',(2.41336099931917,-4.70450989926509,382.11710014609));
#30455=CARTESIAN_POINT('Ctrl Pts',(-0.122606802820077,-5.28599018890692,
382.03797227063));
#30456=CARTESIAN_POINT('Ctrl Pts',(-2.6288874239146,-4.58755660648474,381.958844395171));
#30457=CARTESIAN_POINT('Ctrl Pts',(-4.49862704479611,-2.77832313044165,
381.879716519711));
#30458=CARTESIAN_POINT('Ctrl Pts',(-5.04828738596174,-1.03036438158544,
381.823989439775));
#30459=CARTESIAN_POINT('Ctrl Pts',(-5.07397739854758,-0.0949146237502798,
381.794638318325));
#30460=CARTESIAN_POINT('Ctrl Pts',(-5.07389966860957,-8.89210953773471E-5,
381.791663155363));
#30461=CARTESIAN_POINT('Origin',(0.,0.,402.208336844637));
#30462=CARTESIAN_POINT('',(-5.07378290535392,0.000114313540020838,383.791663155363));
#30463=CARTESIAN_POINT('',(-5.07400033060213,4.63270069165547E-5,383.708336844637));
#30464=CARTESIAN_POINT('',(-5.0736,-1.59740085886799E-13,402.208336844637));
#30465=CARTESIAN_POINT('Ctrl Pts',(-5.07400033060213,4.63270069167923E-5,
383.708336844637));
#30466=CARTESIAN_POINT('Ctrl Pts',(-5.0740221098109,0.0454146017487004,
383.70691332995));
#30467=CARTESIAN_POINT('Ctrl Pts',(-5.06238522132993,0.931389441082911,
383.679113856776));
#30468=CARTESIAN_POINT('Ctrl Pts',(-4.57795151673967,2.64557832586642,383.624938425116));
#30469=CARTESIAN_POINT('Ctrl Pts',(-2.76192026167378,4.50871614055144,383.545810549656));
#30470=CARTESIAN_POINT('Ctrl Pts',(-0.277136335846315,5.28014395819535,
383.466682674197));
#30471=CARTESIAN_POINT('Ctrl Pts',(2.27475150580887,4.77307347049397,383.387554798736));
#30472=CARTESIAN_POINT('Ctrl Pts',(4.27584642055071,3.11028329188466,383.308426923277));
#30473=CARTESIAN_POINT('Ctrl Pts',(5.24161683545466,0.6943901771998,383.229299047817));
#30474=CARTESIAN_POINT('Ctrl Pts',(4.93821764164047,-1.8896378731662,383.150171172357));
#30475=CARTESIAN_POINT('Ctrl Pts',(3.43911186553428,-4.01612180396144,383.071043296897));
#30476=CARTESIAN_POINT('Ctrl Pts',(1.1072828290795,-5.17016919494313,382.991915421438));
#30477=CARTESIAN_POINT('Ctrl Pts',(-1.49265617402097,-5.07234682509687,
382.912787545978));
#30478=CARTESIAN_POINT('Ctrl Pts',(-3.73117351815568,-3.74634074068643,
382.833659670518));
#30479=CARTESIAN_POINT('Ctrl Pts',(-4.88103073617416,-1.82302830121342,
382.765509436738));
#30480=CARTESIAN_POINT('Ctrl Pts',(-5.07301167700312,-0.490907387666408,
382.723735161444));
#30481=CARTESIAN_POINT('Ctrl Pts',(-5.07322528972955,6.22763117691383E-5,
382.708336844637));
#30482=CARTESIAN_POINT('Ctrl Pts',(-5.07378290535392,0.000114313540020942,
383.791663155363));
#30483=CARTESIAN_POINT('Ctrl Pts',(-5.07391625780791,0.136937191492554,
383.787370613824));
#30484=CARTESIAN_POINT('Ctrl Pts',(-5.03516348602304,1.11440684342152,383.756702113798));
#30485=CARTESIAN_POINT('Ctrl Pts',(-4.42825589269063,2.88916500985471,383.699657655286));
#30486=CARTESIAN_POINT('Ctrl Pts',(-2.51417043865664,4.65141609735177,383.620529779826));
#30487=CARTESIAN_POINT('Ctrl Pts',(0.00867922154690349,5.28740478651213,
383.541401904366));
#30488=CARTESIAN_POINT('Ctrl Pts',(2.52942735381344,4.6431370825228,383.462274028906));
#30489=CARTESIAN_POINT('Ctrl Pts',(4.43771707378134,2.87461160478899,383.383146153446));
#30490=CARTESIAN_POINT('Ctrl Pts',(5.27148802998996,0.410047137522666,383.304018277987));
#30491=CARTESIAN_POINT('Ctrl Pts',(4.82885656869832,-2.15380336712922,383.224890402527));
#30492=CARTESIAN_POINT('Ctrl Pts',(3.2169984748157,-4.19614650820864,383.145762527067));
#30493=CARTESIAN_POINT('Ctrl Pts',(0.82619815304806,-5.22246314656389,383.066634651607));
#30494=CARTESIAN_POINT('Ctrl Pts',(-1.76465219517988,-4.98424792073636,
382.987506776148));
#30495=CARTESIAN_POINT('Ctrl Pts',(-3.92822160960685,-3.5391806525149,382.908378900688));
#30496=CARTESIAN_POINT('Ctrl Pts',(-4.9284760402056,-1.63999308805888,382.84309769376));
#30497=CARTESIAN_POINT('Ctrl Pts',(-5.07323479369165,-0.399520902907398,
382.804192445318));
#30498=CARTESIAN_POINT('Ctrl Pts',(-5.0731816081447,-1.92612327423736E-5,
382.791663155363));
#30499=CARTESIAN_POINT('Origin',(0.,0.,402.208336844637));
#30500=CARTESIAN_POINT('',(-5.07368788828891,-0.000125377980982264,384.791663155363));
#30501=CARTESIAN_POINT('',(-5.07341299508847,-0.000118529377325131,384.708336844637));
#30502=CARTESIAN_POINT('',(-5.0736,-1.59740085886799E-13,402.208336844637));
#30503=CARTESIAN_POINT('Ctrl Pts',(-5.07341299508847,-0.000118529377325025,
384.708336844637));
#30504=CARTESIAN_POINT('Ctrl Pts',(-5.07290585727583,0.581565929821983,
384.690091498456));
#30505=CARTESIAN_POINT('Ctrl Pts',(-4.82849439364024,2.00456420438781,384.645470193788));
#30506=CARTESIAN_POINT('Ctrl Pts',(-3.52485021126398,3.94108560628483,384.574472930633));
#30507=CARTESIAN_POINT('Ctrl Pts',(-1.21842922909547,5.14510981239459,384.495345055173));
#30508=CARTESIAN_POINT('Ctrl Pts',(1.38301395642869,5.10333196688562,384.416217179714));
#30509=CARTESIAN_POINT('Ctrl Pts',(3.64958350715001,3.82586787438508,384.337089304254));
#30510=CARTESIAN_POINT('Ctrl Pts',(5.03246761935876,1.62203404033908,384.257961428794));
#30511=CARTESIAN_POINT('Ctrl Pts',(5.19682409785237,-0.974548133184912,
384.178833553334));
#30512=CARTESIAN_POINT('Ctrl Pts',(4.10285677781212,-3.33515982055948,384.099705677875));
#30513=CARTESIAN_POINT('Ctrl Pts',(2.0154514986864,-4.88821849187982,384.020577802414));
#30514=CARTESIAN_POINT('Ctrl Pts',(-0.559961559389509,-5.25767703647906,
383.941449926955));
#30515=CARTESIAN_POINT('Ctrl Pts',(-2.99978931706339,-4.3540772640303,383.862322051495));
#30516=CARTESIAN_POINT('Ctrl Pts',(-4.68244282170845,-2.43143282852321,
383.784617690723));
#30517=CARTESIAN_POINT('Ctrl Pts',(-5.0736185681322,-0.795203160750922,
383.733289288436));
#30518=CARTESIAN_POINT('Ctrl Pts',(-5.07400033060213,4.63270069167923E-5,
383.708336844637));
#30519=CARTESIAN_POINT('Ctrl Pts',(-5.07368788828891,-0.000125377980982003,
384.791663155363));
#30520=CARTESIAN_POINT('Ctrl Pts',(-5.07300172207351,0.67292236196844,384.770548782329));
#30521=CARTESIAN_POINT('Ctrl Pts',(-4.76991529656479,2.18733716132669,384.72305845081));
#30522=CARTESIAN_POINT('Ctrl Pts',(-3.30666744538294,4.12585447040522,384.649192160803));
#30523=CARTESIAN_POINT('Ctrl Pts',(-0.93853660926441,5.20344825460853,384.570064285343));
#30524=CARTESIAN_POINT('Ctrl Pts',(1.65684512644118,5.02111431181428,384.490936409884));
#30525=CARTESIAN_POINT('Ctrl Pts',(3.85104960199139,3.62300174831864,384.411808534424));
#30526=CARTESIAN_POINT('Ctrl Pts',(5.11278700298303,1.34764007340457,384.332680658964));
#30527=CARTESIAN_POINT('Ctrl Pts',(5.13654877856401,-1.25403004379905,384.253552783504));
#30528=CARTESIAN_POINT('Ctrl Pts',(3.91658141328989,-3.55205781743347,384.174424908044));
#30529=CARTESIAN_POINT('Ctrl Pts',(1.74827954439566,-4.99001436270134,384.095297032584));
#30530=CARTESIAN_POINT('Ctrl Pts',(-0.843338895500463,-5.21972261836337,
384.016169157125));
#30531=CARTESIAN_POINT('Ctrl Pts',(-3.23075696562154,-4.18556258278454,
383.937041281665));
#30532=CARTESIAN_POINT('Ctrl Pts',(-4.74882528908407,-2.24901858620394,
383.862205947744));
#30533=CARTESIAN_POINT('Ctrl Pts',(-5.07309686007849,-0.703784911249602,
383.81374657231));
#30534=CARTESIAN_POINT('Ctrl Pts',(-5.07378290535392,0.000114313540020942,
383.791663155363));
#30535=CARTESIAN_POINT('Origin',(0.,0.,402.208336844637));
#30536=CARTESIAN_POINT('',(-5.07320349191978,4.67301704154544E-5,385.791663155363));
#30537=CARTESIAN_POINT('',(-5.07336681616767,0.000110749500208817,385.708336844637));
#30538=CARTESIAN_POINT('',(-5.0736,-1.59740085886799E-13,402.208336844637));
#30539=CARTESIAN_POINT('Ctrl Pts',(-5.07336681616767,0.000110749500209159,
385.708336844637));
#30540=CARTESIAN_POINT('Ctrl Pts',(-5.07358949400792,0.277204924762013,
385.699645625448));
#30541=CARTESIAN_POINT('Ctrl Pts',(-4.98354435800546,1.39507636552693,385.664578447772));
#30542=CARTESIAN_POINT('Ctrl Pts',(-4.1737680903862,3.24597977436508,385.60313531161));
#30543=CARTESIAN_POINT('Ctrl Pts',(-2.12031175571847,4.84365593601313,385.524007436151));
#30544=CARTESIAN_POINT('Ctrl Pts',(0.446542510511727,5.26852204647746,385.44487956069));
#30545=CARTESIAN_POINT('Ctrl Pts',(2.90527399685678,4.41770390260608,385.365751685231));
#30546=CARTESIAN_POINT('Ctrl Pts',(4.66054210967394,2.4972128487314,385.286623809771));
#30547=CARTESIAN_POINT('Ctrl Pts',(5.2873381133244,-0.0279364153108744,
385.207495934311));
#30548=CARTESIAN_POINT('Ctrl Pts',(4.63389386761938,-2.54632134491165,385.128368058852));
#30549=CARTESIAN_POINT('Ctrl Pts',(2.85842993763932,-4.44815726560116,385.049240183392));
#30550=CARTESIAN_POINT('Ctrl Pts',(0.390845137441743,-5.27294650517633,
384.970112307932));
#30551=CARTESIAN_POINT('Ctrl Pts',(-2.1713762578616,-4.82098018194518,384.890984432472));
#30552=CARTESIAN_POINT('Ctrl Pts',(-4.20783530881936,-3.2016943610792,384.811856557012));
#30553=CARTESIAN_POINT('Ctrl Pts',(-4.99079834853979,-1.35930215545066,
384.750974027734));
#30554=CARTESIAN_POINT('Ctrl Pts',(-5.07363898920769,-0.259332620176451,
384.716467456942));
#30555=CARTESIAN_POINT('Ctrl Pts',(-5.07341299508847,-0.000118529377325025,
384.708336844637));
#30556=CARTESIAN_POINT('Ctrl Pts',(-5.07320349191978,4.6730170415385E-5,
385.791663155363));
#30557=CARTESIAN_POINT('Ctrl Pts',(-5.07332318093048,0.368645452041058,
385.780102909322));
#30558=CARTESIAN_POINT('Ctrl Pts',(-4.94327787593756,1.57815905047111,385.742166704794));
#30559=CARTESIAN_POINT('Ctrl Pts',(-3.99220955212729,3.46684115546438,385.67785454178));
#30560=CARTESIAN_POINT('Ctrl Pts',(-1.85539526299902,4.95118502212943,385.59872666632));
#30561=CARTESIAN_POINT('Ctrl Pts',(0.73067187193628,5.23668247279509,385.51959879086));
#30562=CARTESIAN_POINT('Ctrl Pts',(3.13981906729605,4.25420508790564,385.440470915401));
#30563=CARTESIAN_POINT('Ctrl Pts',(4.78871173391359,2.24164328892807,385.361343039941));
#30564=CARTESIAN_POINT('Ctrl Pts',(5.27809816640793,-0.313694837508304,
385.282215164481));
#30565=CARTESIAN_POINT('Ctrl Pts',(4.48948164772799,-2.79307702006795,385.203087289022));
#30566=CARTESIAN_POINT('Ctrl Pts',(2.61381244185943,-4.59616244535579,385.123959413562));
#30567=CARTESIAN_POINT('Ctrl Pts',(0.105252389857621,-5.28636421747,385.044831538102));
#30568=CARTESIAN_POINT('Ctrl Pts',(-2.42879276314368,-4.69656155277656,
384.965703662642));
#30569=CARTESIAN_POINT('Ctrl Pts',(-4.3747464822184,-2.96956527485689,384.886575787182));
#30570=CARTESIAN_POINT('Ctrl Pts',(-5.02482764874857,-1.17623295765146,
384.828562284756));
#30571=CARTESIAN_POINT('Ctrl Pts',(-5.0738588771301,-0.167845167351579,
384.796924740816));
#30572=CARTESIAN_POINT('Ctrl Pts',(-5.07368788828891,-0.000125377980982003,
384.791663155363));
#30573=CARTESIAN_POINT('Origin',(0.,0.,402.208336844637));
#30574=CARTESIAN_POINT('',(-5.07396871057133,6.36451556410011E-5,386.791663155363));
#30575=CARTESIAN_POINT('',(-5.07402204930561,-2.85592496231871E-5,386.708336844637));
#30576=CARTESIAN_POINT('',(-5.0736,-1.59740085886799E-13,402.208336844637));
#30577=CARTESIAN_POINT('Ctrl Pts',(-5.07402204930561,-2.85592496232024E-5,
386.708336844637));
#30578=CARTESIAN_POINT('Ctrl Pts',(-5.07376894837123,0.813077680770696,
386.682823793954));
#30579=CARTESIAN_POINT('Ctrl Pts',(-4.66877404608003,2.46703434122352,386.630934784784));
#30580=CARTESIAN_POINT('Ctrl Pts',(-2.95361232316089,4.38553292227813,386.552669817127));
#30581=CARTESIAN_POINT('Ctrl Pts',(-0.504372453036948,5.26330059910421,
386.473541941668));
#30582=CARTESIAN_POINT('Ctrl Pts',(2.06699274767947,4.86664830750627,386.394414066208));
#30583=CARTESIAN_POINT('Ctrl Pts',(4.1378703204085,3.29161874757629,386.315286190749));
#30584=CARTESIAN_POINT('Ctrl Pts',(5.20683199193,0.919578912180737,386.236158315288));
#30585=CARTESIAN_POINT('Ctrl Pts',(5.01504662121074,-1.67512153439562,386.157030439829));
#30586=CARTESIAN_POINT('Ctrl Pts',(3.60895181930755,-3.86421939514695,386.077902564369));
#30587=CARTESIAN_POINT('Ctrl Pts',(1.32900986066236,-5.11766133679979,385.998774688909));
#30588=CARTESIAN_POINT('Ctrl Pts',(-1.2727295467071,-5.13194741485647,385.91964681345));
#30589=CARTESIAN_POINT('Ctrl Pts',(-3.5662988394905,-3.90361849510962,385.84051893799));
#30590=CARTESIAN_POINT('Ctrl Pts',(-4.83927537814081,-1.96882864770619,
385.770082281719));
#30591=CARTESIAN_POINT('Ctrl Pts',(-5.07291371523136,-0.563715584161085,
385.726021583935));
#30592=CARTESIAN_POINT('Ctrl Pts',(-5.07336681616767,0.000110749500209159,
385.708336844637));
#30593=CARTESIAN_POINT('Ctrl Pts',(-5.07396871057133,6.36451556408537E-5,
386.791663155363));
#30594=CARTESIAN_POINT('Ctrl Pts',(-5.07400891965194,0.0640010310039327,
386.789657036314));
#30595=CARTESIAN_POINT('Ctrl Pts',(-5.05726353871135,0.968550309919132,
386.761274958779));
#30596=CARTESIAN_POINT('Ctrl Pts',(-4.54862274572651,2.695692085973,386.706516922757));
#30597=CARTESIAN_POINT('Ctrl Pts',(-2.71224074091265,4.53877459989496,386.627389047297));
#30598=CARTESIAN_POINT('Ctrl Pts',(-0.219135128106394,5.28286896496098,
386.548261171838));
#30599=CARTESIAN_POINT('Ctrl Pts',(2.32703038082081,4.74780520999492,386.469133296378));
#30600=CARTESIAN_POINT('Ctrl Pts',(4.30974451002784,3.06314004962277,386.390005420918));
#30601=CARTESIAN_POINT('Ctrl Pts',(5.24892628554031,0.636786898642001,386.310877545458));
#30602=CARTESIAN_POINT('Ctrl Pts',(4.91716859158436,-1.94375352019086,386.231749669999));
#30603=CARTESIAN_POINT('Ctrl Pts',(3.39480098979053,-4.05364662310803,386.152621794539));
#30604=CARTESIAN_POINT('Ctrl Pts',(1.05043926306477,-5.18201718059,386.073493919079));
#30605=CARTESIAN_POINT('Ctrl Pts',(-1.54826871412865,-5.0556491862241,385.994366043619));
#30606=CARTESIAN_POINT('Ctrl Pts',(-3.772089388456,-3.70514053050835,385.91523816816));
#30607=CARTESIAN_POINT('Ctrl Pts',(-4.89110742269369,-1.78586579845603,
385.84767053874));
#30608=CARTESIAN_POINT('Ctrl Pts',(-5.07305009743672,-0.472352615975399,
385.806478867808));
#30609=CARTESIAN_POINT('Ctrl Pts',(-5.07320349191978,4.6730170415385E-5,
385.791663155363));
#30610=CARTESIAN_POINT('Origin',(0.,0.,402.208336844637));
#30611=CARTESIAN_POINT('',(-5.07346461004462,-0.000124534794222197,387.791663155363));
#30612=CARTESIAN_POINT('',(-5.07325209134275,-7.62409538748165E-5,387.708336844637));
#30613=CARTESIAN_POINT('',(-5.0736,-1.59740085886799E-13,402.208336844637));
#30614=CARTESIAN_POINT('Ctrl Pts',(-5.07325209134275,-7.62409538748038E-5,
387.708336844637));
#30615=CARTESIAN_POINT('Ctrl Pts',(-5.0729792152731,0.508760470280088,387.692377920946));
#30616=CARTESIAN_POINT('Ctrl Pts',(-4.87111972002504,1.85878392032608,387.650043038769));
#30617=CARTESIAN_POINT('Ctrl Pts',(-3.69137763771595,3.78555886279474,387.581332198105));
#30618=CARTESIAN_POINT('Ctrl Pts',(-1.43897337649567,5.08783651365194,387.502204322645));
#30619=CARTESIAN_POINT('Ctrl Pts',(1.16185415459233,5.15817988164137,387.423076447186));
#30620=CARTESIAN_POINT('Ctrl Pts',(3.48135818778607,3.97955649994419,387.343948571725));
#30621=CARTESIAN_POINT('Ctrl Pts',(4.95790972221771,1.83735025355874,387.264820696266));
#30622=CARTESIAN_POINT('Ctrl Pts',(5.23398656730458,-0.749739542233496,
387.185692820806));
#30623=CARTESIAN_POINT('Ctrl Pts',(4.24274134513742,-3.15529248187465,387.106564945346));
#30624=CARTESIAN_POINT('Ctrl Pts',(2.22418746193322,-4.79684426494046,387.027437069886));
#30625=CARTESIAN_POINT('Ctrl Pts',(-0.332916112977428,-5.27692065788687,
386.948309194427));
#30626=CARTESIAN_POINT('Ctrl Pts',(-2.80940963451955,-4.47927921359921,
386.869181318967));
#30627=CARTESIAN_POINT('Ctrl Pts',(-4.6056517301173,-2.59705543044056,386.790053443507));
#30628=CARTESIAN_POINT('Ctrl Pts',(-5.06711936969965,-0.895633636916161,
386.73643861873));
#30629=CARTESIAN_POINT('Ctrl Pts',(-5.07403060973901,-0.0275296106999626,
386.70919975244));
#30630=CARTESIAN_POINT('Ctrl Pts',(-5.07402204930561,-2.85592496232024E-5,
386.708336844637));
#30631=CARTESIAN_POINT('Ctrl Pts',(-5.07346461004462,-0.000124534794222232,
387.791663155363));
#30632=CARTESIAN_POINT('Ctrl Pts',(-5.07290587442459,0.600116546096426,
387.77283520482));
#30633=CARTESIAN_POINT('Ctrl Pts',(-4.81706146775411,2.04169530250574,387.727631295791));
#30634=CARTESIAN_POINT('Ctrl Pts',(-3.48135818389009,3.97955649548785,387.656051428275));
#30635=CARTESIAN_POINT('Ctrl Pts',(-1.16185415329344,5.15817987586638,387.576923552815));
#30636=CARTESIAN_POINT('Ctrl Pts',(1.43897337488296,5.0878365079566,387.497795677355));
#30637=CARTESIAN_POINT('Ctrl Pts',(3.69137763358211,3.7855588585581,387.418667801895));
#30638=CARTESIAN_POINT('Ctrl Pts',(5.04997670698908,1.56667161976776,387.339539926436));
#30639=CARTESIAN_POINT('Ctrl Pts',(5.1858086147589,-1.03155887685117,387.260412050976));
#30640=CARTESIAN_POINT('Ctrl Pts',(4.06598393848355,-3.38001469187811,387.181284175516));
#30641=CARTESIAN_POINT('Ctrl Pts',(1.96164944276588,-4.91005663602919,387.102156300056));
#30642=CARTESIAN_POINT('Ctrl Pts',(-0.617665566383616,-5.25121071310437,
387.023028424596));
#30643=CARTESIAN_POINT('Ctrl Pts',(-3.04742321760052,-4.32087218488899,
386.943900549136));
#30644=CARTESIAN_POINT('Ctrl Pts',(-4.69640454618417,-2.39441853297418,
386.866778792725));
#30645=CARTESIAN_POINT('Ctrl Pts',(-5.07348026057684,-0.776631949401611,
386.816032994801));
#30646=CARTESIAN_POINT('Ctrl Pts',(-5.07396871057133,6.36451556408537E-5,
386.791663155363));
#30647=CARTESIAN_POINT('Origin',(0.,0.,402.208336844637));
#30648=CARTESIAN_POINT('',(-5.07332308908166,0.000100751512192854,388.791663155363));
#30649=CARTESIAN_POINT('',(-5.07357378438926,0.00012964408007953,388.708336844637));
#30650=CARTESIAN_POINT('',(-5.0736,-1.59740085886799E-13,402.208336844637));
#30651=CARTESIAN_POINT('Ctrl Pts',(-5.07357378438926,0.000129644080079632,
388.708336844637));
#30652=CARTESIAN_POINT('Ctrl Pts',(-5.07377922823885,0.204303981988881,
388.701932047939));
#30653=CARTESIAN_POINT('Ctrl Pts',(-5.01188528533374,1.24917654214382,388.669151292754));
#30654=CARTESIAN_POINT('Ctrl Pts',(-4.30974451485365,3.06314005305047,388.609994579082));
#30655=CARTESIAN_POINT('Ctrl Pts',(-2.32703038342756,4.74780521530929,388.530866703622));
#30656=CARTESIAN_POINT('Ctrl Pts',(0.2191351283499,5.28286897087523,388.451738828163));
#30657=CARTESIAN_POINT('Ctrl Pts',(2.71224074394742,4.53877460497707,388.372610952702));
#30658=CARTESIAN_POINT('Ctrl Pts',(4.54862275081774,2.69569208899244,388.293483077243));
#30659=CARTESIAN_POINT('Ctrl Pts',(5.28363204425109,0.199892943537846,388.214355201783));
#30660=CARTESIAN_POINT('Ctrl Pts',(4.73929845080001,-2.34430692575821,388.135227326323));
#30661=CARTESIAN_POINT('Ctrl Pts',(3.04742322101362,-4.32087218972514,388.056099450863));
#30662=CARTESIAN_POINT('Ctrl Pts',(0.617665567076949,-5.25121071898288,
387.976971575404));
#30663=CARTESIAN_POINT('Ctrl Pts',(-1.96164944496022,-4.9100566415267,387.897843699944));
#30664=CARTESIAN_POINT('Ctrl Pts',(-4.06598394303424,-3.38001469566346,
387.818715824484));
#30665=CARTESIAN_POINT('Ctrl Pts',(-4.95995652391698,-1.50520772763894,
387.755546872715));
#30666=CARTESIAN_POINT('Ctrl Pts',(-5.07343020858722,-0.332214537305361,
387.718753879433));
#30667=CARTESIAN_POINT('Ctrl Pts',(-5.07325209134275,-7.62409538748038E-5,
387.708336844637));
#30668=CARTESIAN_POINT('Ctrl Pts',(-5.07332308908166,0.000100751512193097,
388.791663155363));
#30669=CARTESIAN_POINT('Ctrl Pts',(-5.07353661258784,0.295776873009828,
388.782389331812));
#30670=CARTESIAN_POINT('Ctrl Pts',(-4.97579423080698,1.43225469143156,388.746739549775));
#30671=CARTESIAN_POINT('Ctrl Pts',(-4.13787031577727,3.29161874388992,388.684713809251));
#30672=CARTESIAN_POINT('Ctrl Pts',(-2.0669927453671,4.86664830205737,388.605585933792));
#30673=CARTESIAN_POINT('Ctrl Pts',(0.504372452470541,5.2633005932121,388.526458058332));
#30674=CARTESIAN_POINT('Ctrl Pts',(2.95361231985281,4.38553291736953,388.447330182872));
#30675=CARTESIAN_POINT('Ctrl Pts',(4.68768449948338,2.44588199605403,388.368202307412));
#30676=CARTESIAN_POINT('Ctrl Pts',(5.28671249546426,-0.0859982303311033,
388.289074431953));
#30677=CARTESIAN_POINT('Ctrl Pts',(4.60565172496217,-2.59705542753155,388.209946556493));
#30678=CARTESIAN_POINT('Ctrl Pts',(2.80940963137597,-4.47927920858367,388.130818681033));
#30679=CARTESIAN_POINT('Ctrl Pts',(0.332916112606594,-5.27692065197923,
388.051690805573));
#30680=CARTESIAN_POINT('Ctrl Pts',(-2.22418745944155,-4.79684425957118,
387.972562930114));
#30681=CARTESIAN_POINT('Ctrl Pts',(-4.24274134038657,-3.15529247834378,
387.893435054654));
#30682=CARTESIAN_POINT('Ctrl Pts',(-4.99812636818859,-1.3221248286521,387.833135129737));
#30683=CARTESIAN_POINT('Ctrl Pts',(-5.07368860366989,-0.240757440453781,
387.799211163307));
#30684=CARTESIAN_POINT('Ctrl Pts',(-5.07346461004462,-0.000124534794222232,
387.791663155363));
#30685=CARTESIAN_POINT('Origin',(0.,0.,402.208336844637));
#30686=CARTESIAN_POINT('',(-5.07403406771079,-9.36144982375056E-6,389.791663155363));
#30687=CARTESIAN_POINT('',(-5.07388549569213,-9.2912700738374E-5,389.708336844637));
#30688=CARTESIAN_POINT('',(-5.0736,-1.59740085886799E-13,402.208336844637));
#30689=CARTESIAN_POINT('Ctrl Pts',(-5.07388549569213,-9.2912700738277E-5,
389.708336844637));
#30690=CARTESIAN_POINT('Ctrl Pts',(-5.07325856807114,0.740202389523463,
389.685110216444));
#30691=CARTESIAN_POINT('Ctrl Pts',(-4.72308495981242,2.32174429013103,389.635507629765));
#30692=CARTESIAN_POINT('Ctrl Pts',(-3.13981907081257,4.25420509266713,389.559529084599));
#30693=CARTESIAN_POINT('Ctrl Pts',(-0.730671872756092,5.23668247865729,
389.48040120914));
#30694=CARTESIAN_POINT('Ctrl Pts',(1.85539526507438,4.95118502767294,389.401273333679));
#30695=CARTESIAN_POINT('Ctrl Pts',(3.99220955659535,3.46684115934693,389.32214545822));
#30696=CARTESIAN_POINT('Ctrl Pts',(5.16237725796638,1.14305984722794,389.24301758276));
#30697=CARTESIAN_POINT('Ctrl Pts',(5.08256188536855,-1.45749423645932,389.1638897073));
#30698=CARTESIAN_POINT('Ctrl Pts',(3.77208939268016,-3.70514053465492,389.08476183184));
#30699=CARTESIAN_POINT('Ctrl Pts',(1.54826871586373,-5.05564919188336,389.005633956381));
#30700=CARTESIAN_POINT('Ctrl Pts',(-1.05043926423896,-5.18201718639165,
388.926506080921));
#30701=CARTESIAN_POINT('Ctrl Pts',(-3.39480099358967,-4.05364662764723,
388.847378205461));
#30702=CARTESIAN_POINT('Ctrl Pts',(-4.79394457591898,-2.1145332421108,388.7746551267));
#30703=CARTESIAN_POINT('Ctrl Pts',(-5.07293317820744,-0.636518001009154,
388.728308006425));
#30704=CARTESIAN_POINT('Ctrl Pts',(-5.07357378438926,0.000129644080079632,
388.708336844637));
#30705=CARTESIAN_POINT('Ctrl Pts',(-5.07403406771079,-9.36144982382212E-6,
389.791663155363));
#30706=CARTESIAN_POINT('Ctrl Pts',(-5.07394412729799,0.831658855747162,
389.765567500318));
#30707=CARTESIAN_POINT('Ctrl Pts',(-4.65432422371577,2.50401601420859,389.713095886787));
#30708=CARTESIAN_POINT('Ctrl Pts',(-2.90527399360582,4.41770389765948,389.634248314769));
#30709=CARTESIAN_POINT('Ctrl Pts',(-0.446542510013585,5.2685220405792,389.55512043931));
#30710=CARTESIAN_POINT('Ctrl Pts',(2.12031175334316,4.84365593059135,389.475992563849));
#30711=CARTESIAN_POINT('Ctrl Pts',(4.17376808571255,3.24597977073262,389.39686468839));
#30712=CARTESIAN_POINT('Ctrl Pts',(5.21661647505316,0.862344048232485,389.31773681293));
#30713=CARTESIAN_POINT('Ctrl Pts',(4.99634867366186,-1.73009382303836,389.23860893747));
#30714=CARTESIAN_POINT('Ctrl Pts',(3.56629883549932,-3.90361849073832,389.15948106201));
#30715=CARTESIAN_POINT('Ctrl Pts',(1.27272954528402,-5.13194740911081,389.08035318655));
#30716=CARTESIAN_POINT('Ctrl Pts',(-1.3290098591728,-5.11766133107102,389.001225311091));
#30717=CARTESIAN_POINT('Ctrl Pts',(-3.60895181526604,-3.86421939082217,
388.922097435631));
#30718=CARTESIAN_POINT('Ctrl Pts',(-4.85025165556801,-1.93168481258741,
388.852243383721));
#30719=CARTESIAN_POINT('Ctrl Pts',(-5.07292932400786,-0.545164413360684,
388.808765290299));
#30720=CARTESIAN_POINT('Ctrl Pts',(-5.07332308908166,0.000100751512193097,
388.791663155363));
#30721=CARTESIAN_POINT('Origin',(0.,0.,402.208336844637));
#30722=CARTESIAN_POINT('',(-5.0732856633921,-8.9472558095216E-5,390.791663155363));
#30723=CARTESIAN_POINT('',(-5.07317963304504,-1.41915822972106E-5,390.708336844637));
#30724=CARTESIAN_POINT('',(-5.0736,-1.59740085886799E-13,402.208336844637));
#30725=CARTESIAN_POINT('Ctrl Pts',(-5.07317963304504,-1.41915822972002E-5,
390.708336844637));
#30726=CARTESIAN_POINT('Ctrl Pts',(-5.07313689101218,0.435939705489138,
390.694664343437));
#30727=CARTESIAN_POINT('Ctrl Pts',(-4.9102234101679,1.71293434968472,390.65461588375));
#30728=CARTESIAN_POINT('Ctrl Pts',(-3.85104960630393,3.62300175237324,390.588191465576));
#30729=CARTESIAN_POINT('Ctrl Pts',(-1.65684512829777,5.02111431743484,390.509063590116));
#30730=CARTESIAN_POINT('Ctrl Pts',(0.938536610313288,5.20344826043412,390.429935714657));
#30731=CARTESIAN_POINT('Ctrl Pts',(3.30666744908329,4.12585447502528,390.350807839197));
#30732=CARTESIAN_POINT('Ctrl Pts',(4.874144221702,2.04925422384882,390.271679963737));
#30733=CARTESIAN_POINT('Ctrl Pts',(5.26142871608132,-0.523538569265068,
390.192552088277));
#30734=CARTESIAN_POINT('Ctrl Pts',(4.37474648711696,-2.96956527817979,390.113424212818));
#30735=CARTESIAN_POINT('Ctrl Pts',(2.42879276586438,-4.69656155803349,390.034296337358));
#30736=CARTESIAN_POINT('Ctrl Pts',(-0.105252389973582,-5.28636422338813,
389.955168461898));
#30737=CARTESIAN_POINT('Ctrl Pts',(-2.61381244478399,-4.59616245050211,
389.876040586438));
#30738=CARTESIAN_POINT('Ctrl Pts',(-4.48948165275299,-2.79307702319636,
389.796912710979));
#30739=CARTESIAN_POINT('Ctrl Pts',(-5.04661334373894,-1.04147487532298,
389.741011463711));
#30740=CARTESIAN_POINT('Ctrl Pts',(-5.07397050166598,-0.10047056555588,
389.711486174931));
#30741=CARTESIAN_POINT('Ctrl Pts',(-5.07388549569213,-9.2912700738277E-5,
389.708336844637));
#30742=CARTESIAN_POINT('Ctrl Pts',(-5.0732856633921,-8.94725580950079E-5,
390.791663155363));
#30743=CARTESIAN_POINT('Ctrl Pts',(-5.07295082938292,0.527313084285289,
390.77512162731));
#30744=CARTESIAN_POINT('Ctrl Pts',(-4.86059546998445,1.89593815106623,390.732204140772));
#30745=CARTESIAN_POINT('Ctrl Pts',(-3.64958350306562,3.82586787010077,390.662910695746));
#30746=CARTESIAN_POINT('Ctrl Pts',(-1.38301395488213,5.10333196117197,390.583782820286));
#30747=CARTESIAN_POINT('Ctrl Pts',(1.21842922772966,5.14510980663504,390.504654944826));
#30748=CARTESIAN_POINT('Ctrl Pts',(3.52485020731651,3.94108560187402,390.425527069367));
#30749=CARTESIAN_POINT('Ctrl Pts',(4.97778782502355,1.78279361519087,390.346399193907));
#30750=CARTESIAN_POINT('Ctrl Pts',(5.2254376041702,-0.807171945896316,390.267271318447));
#30751=CARTESIAN_POINT('Ctrl Pts',(4.2078353041098,-3.20169435749343,390.188143442988));
#30752=CARTESIAN_POINT('Ctrl Pts',(2.17137625543244,-4.82098017654731,390.109015567527));
#30753=CARTESIAN_POINT('Ctrl Pts',(-0.390845137002325,-5.27294649927341,
390.029887692068));
#30754=CARTESIAN_POINT('Ctrl Pts',(-2.85842993443779,-4.44815726062243,
389.950759816608));
#30755=CARTESIAN_POINT('Ctrl Pts',(-4.63389386243089,-2.54632134206259,
389.871631941148));
#30756=CARTESIAN_POINT('Ctrl Pts',(-5.07183812704173,-0.858476903537314,
389.818599720733));
#30757=CARTESIAN_POINT('Ctrl Pts',(-5.07403503379527,-0.00894262882346251,
389.791943458805));
#30758=CARTESIAN_POINT('Ctrl Pts',(-5.07403406771079,-9.36144982382212E-6,
389.791663155363));
#30759=CARTESIAN_POINT('Origin',(0.,0.,402.208336844637));
#30760=CARTESIAN_POINT('',(-5.07351709598447,0.000128180283586465,391.791663155363));
#30761=CARTESIAN_POINT('',(-5.07379939980891,0.000111618004047815,391.708336844637));
#30762=CARTESIAN_POINT('',(-5.0736,-1.59740085886799E-13,402.208336844637));
#30763=CARTESIAN_POINT('Ctrl Pts',(-5.07379939980891,0.000111618004048301,
391.708336844637));
#30764=CARTESIAN_POINT('Ctrl Pts',(-5.07392549945089,0.131381756589591,
391.704218470429));
#30765=CARTESIAN_POINT('Ctrl Pts',(-5.03695972030326,1.10329526429473,391.673724137734));
#30766=CARTESIAN_POINT('Ctrl Pts',(-4.43771707875037,2.8746116080056,391.616853846554));
#30767=CARTESIAN_POINT('Ctrl Pts',(-2.52942735664669,4.64313708771996,391.537725971094));
#30768=CARTESIAN_POINT('Ctrl Pts',(-0.00867922155838994,5.28740479243137,
391.458598095634));
#30769=CARTESIAN_POINT('Ctrl Pts',(2.51417044146968,4.65141610255989,391.379470220174));
#30770=CARTESIAN_POINT('Ctrl Pts',(4.42825589764708,2.88916501309064,391.300342344714));
#30771=CARTESIAN_POINT('Ctrl Pts',(5.27011345519119,0.427351070346123,391.221214469255));
#30772=CARTESIAN_POINT('Ctrl Pts',(4.8359014254693,-2.1379387669101,391.142086593795));
#30773=CARTESIAN_POINT('Ctrl Pts',(3.23075696923981,-4.18556258746916,391.062958718335));
#30774=CARTESIAN_POINT('Ctrl Pts',(0.843338896446427,-5.21972262420654,
390.983830842875));
#30775=CARTESIAN_POINT('Ctrl Pts',(-1.7482795463511,-4.99001436828829,390.904702967415));
#30776=CARTESIAN_POINT('Ctrl Pts',(-3.91658141767327,-3.55205782141137,
390.825575091956));
#30777=CARTESIAN_POINT('Ctrl Pts',(-4.92575069087544,-1.65110613686035,
390.760119717696));
#30778=CARTESIAN_POINT('Ctrl Pts',(-5.07321934571947,-0.405069684288436,
390.721040301923));
#30779=CARTESIAN_POINT('Ctrl Pts',(-5.07317963304504,-1.41915822972002E-5,
390.708336844637));
#30780=CARTESIAN_POINT('Ctrl Pts',(-5.07351709598447,0.0001281802835865,
391.791663155363));
#30781=CARTESIAN_POINT('Ctrl Pts',(-5.07373426530186,0.222882138466162,
391.784675754303));
#30782=CARTESIAN_POINT('Ctrl Pts',(-5.00497588579108,1.28635201118677,391.751312394756));
#30783=CARTESIAN_POINT('Ctrl Pts',(-4.27584641576499,3.1102832884012,391.691573076723));
#30784=CARTESIAN_POINT('Ctrl Pts',(-2.27475150326393,4.77307346514974,391.612445201264));
#30785=CARTESIAN_POINT('Ctrl Pts',(0.277136335534271,5.28014395228432,391.533317325804));
#30786=CARTESIAN_POINT('Ctrl Pts',(2.76192025858026,4.50871613550486,391.454189450344));
#30787=CARTESIAN_POINT('Ctrl Pts',(4.57795151161372,2.64557832290629,391.375061574885));
#30788=CARTESIAN_POINT('Ctrl Pts',(5.28550858366077,0.141858088829558,391.295933699424));
#30789=CARTESIAN_POINT('Ctrl Pts',(4.71326839627705,-2.39621070233275,391.216805823965));
#30790=CARTESIAN_POINT('Ctrl Pts',(2.99978931370662,-4.35407725915487,391.137677948505));
#30791=CARTESIAN_POINT('Ctrl Pts',(0.559961558764467,-5.2576770305929,391.058550073045));
#30792=CARTESIAN_POINT('Ctrl Pts',(-2.01545149642842,-4.88821848640817,
390.979422197585));
#30793=CARTESIAN_POINT('Ctrl Pts',(-4.10285677321784,-3.33515981682715,
390.900294322126));
#30794=CARTESIAN_POINT('Ctrl Pts',(-4.96813235745424,-1.46802940120253,
390.837707974718));
#30795=CARTESIAN_POINT('Ctrl Pts',(-5.07348473216978,-0.313645979534272,
390.801497585797));
#30796=CARTESIAN_POINT('Ctrl Pts',(-5.0732856633921,-8.94725580950079E-5,
390.791663155363));
#30797=CARTESIAN_POINT('Origin',(0.,0.,402.208336844637));
#30798=CARTESIAN_POINT('',(-5.07393095917883,-7.88724074329838E-5,392.791663155363));
#30799=CARTESIAN_POINT('',(-5.07367047787857,-0.000126645267990005,392.708336844637));
#30800=CARTESIAN_POINT('',(-5.0736,-1.59740085886799E-13,402.208336844637));
#30801=CARTESIAN_POINT('Ctrl Pts',(-5.07367047787857,-0.000126645267989993,
392.708336844637));
#30802=CARTESIAN_POINT('Ctrl Pts',(-5.07298837013062,0.667375891727513,
392.687396638935));
#30803=CARTESIAN_POINT('Ctrl Pts',(-4.77363543308555,2.17624796267435,392.640080474746));
#30804=CARTESIAN_POINT('Ctrl Pts',(-3.32019468996614,4.11497654776232,392.566388352071));
#30805=CARTESIAN_POINT('Ctrl Pts',(-0.955614322062658,5.20033903081154,
392.487260476611));
#30806=CARTESIAN_POINT('Ctrl Pts',(1.64035202716895,5.02652663326038,392.408132601151));
#30807=CARTESIAN_POINT('Ctrl Pts',(3.83913464362559,3.63562511214056,392.329004725691));
#30808=CARTESIAN_POINT('Ctrl Pts',(5.10833519286426,1.36441794376124,392.249876850232));
#30809=CARTESIAN_POINT('Ctrl Pts',(5.14063804785052,-1.23716014683014,392.170748974772));
#30810=CARTESIAN_POINT('Ctrl Pts',(3.92822161400576,-3.53918065647562,392.091621099312));
#30811=CARTESIAN_POINT('Ctrl Pts',(1.76465219715718,-4.98424792631562,392.012493223852));
#30812=CARTESIAN_POINT('Ctrl Pts',(-0.826198153971171,-5.22246315241074,
391.933365348392));
#30813=CARTESIAN_POINT('Ctrl Pts',(-3.21699847841567,-4.19614651290735,
391.854237472933));
#30814=CARTESIAN_POINT('Ctrl Pts',(-4.74496408021847,-2.26010134957161,
391.779227971681));
#30815=CARTESIAN_POINT('Ctrl Pts',(-5.07311789947229,-0.7093324551461,391.730594428916));
#30816=CARTESIAN_POINT('Ctrl Pts',(-5.07379939980891,0.000111618004048301,
391.708336844637));
#30817=CARTESIAN_POINT('Ctrl Pts',(-5.07393095917883,-7.88724074328884E-5,
392.791663155363));
#30818=CARTESIAN_POINT('Ctrl Pts',(-5.07336361274665,0.758765898971362,
392.767853922809));
#30819=CARTESIAN_POINT('Ctrl Pts',(-4.7096061531202,2.35878746105711,392.717668731768));
#30820=CARTESIAN_POINT('Ctrl Pts',(-3.09291170420029,4.28842883762094,392.64110758224));
#30821=CARTESIAN_POINT('Ctrl Pts',(-0.67312059357683,5.24439065781915,392.561979706781));
#30822=CARTESIAN_POINT('Ctrl Pts',(1.90965537976903,4.9305112347339,392.482851831321));
#30823=CARTESIAN_POINT('Ctrl Pts',(4.03004033003705,3.4227912065437,392.403723955861));
#30824=CARTESIAN_POINT('Ctrl Pts',(5.17461860283211,1.0862996918631,392.324596080401));
#30825=CARTESIAN_POINT('Ctrl Pts',(5.06624976530063,-1.51322107469774,392.245468204942));
#30826=CARTESIAN_POINT('Ctrl Pts',(3.73117351397988,-3.74634073649114,392.166340329482));
#30827=CARTESIAN_POINT('Ctrl Pts',(1.49265617235166,-5.07234681941786,392.087212454022));
#30828=CARTESIAN_POINT('Ctrl Pts',(-1.10728282783815,-5.1701691891555,392.008084578562));
#30829=CARTESIAN_POINT('Ctrl Pts',(-3.43911186168285,-4.01612179946654,
391.928956703103));
#30830=CARTESIAN_POINT('Ctrl Pts',(-4.80583883513493,-2.07741741105628,
391.856816228703));
#30831=CARTESIAN_POINT('Ctrl Pts',(-5.07291449714329,-0.617966855796078,
391.811051712789));
#30832=CARTESIAN_POINT('Ctrl Pts',(-5.07351709598447,0.0001281802835865,
391.791663155363));
#30833=CARTESIAN_POINT('Origin',(0.,0.,402.208336844637));
#30834=CARTESIAN_POINT('',(-5.07318860167667,-3.10232113821807E-5,393.791663155363));
#30835=CARTESIAN_POINT('',(-5.07320934784751,5.14726455261062E-5,393.708336844637));
#30836=CARTESIAN_POINT('',(-5.0736,-1.59740085886799E-13,402.208336844637));
#30837=CARTESIAN_POINT('Ctrl Pts',(-5.07320934784751,5.14726455259906E-5,
393.708336844637));
#30838=CARTESIAN_POINT('Ctrl Pts',(-5.07333938414724,0.363095667172288,
393.696950765927));
#30839=CARTESIAN_POINT('Ctrl Pts',(-4.94587345760415,1.56704518273248,393.659188728731));
#30840=CARTESIAN_POINT('Ctrl Pts',(-4.00356958154437,3.45371616865744,393.595050733048));
#30841=CARTESIAN_POINT('Ctrl Pts',(-1.8716398630404,4.94506713715712,393.515922857588));
#30842=CARTESIAN_POINT('Ctrl Pts',(0.713476058729831,5.23905303289941,393.436794982128));
#30843=CARTESIAN_POINT('Ctrl Pts',(3.12583571869877,4.26449010171441,393.357667106669));
#30844=CARTESIAN_POINT('Ctrl Pts',(4.78132668327137,2.25735241283907,393.278539231209));
#30845=CARTESIAN_POINT('Ctrl Pts',(5.2790995798779,-0.296365304389928,393.199411355749));
#30846=CARTESIAN_POINT('Ctrl Pts',(4.49862704983328,-2.77832313355043,393.120283480289));
#30847=CARTESIAN_POINT('Ctrl Pts',(2.62888742685924,-4.58755661161959,393.041155604829));
#30848=CARTESIAN_POINT('Ctrl Pts',(0.122606802959192,-5.28599019482455,
392.96202772937));
#30849=CARTESIAN_POINT('Ctrl Pts',(-2.41336100201929,-4.70450990453263,
392.88289985391));
#30850=CARTESIAN_POINT('Ctrl Pts',(-4.3649739152189,-2.98391144093985,392.80377197845));
#30851=CARTESIAN_POINT('Ctrl Pts',(-5.02290836650147,-1.18734550240995,
392.745584308693));
#30852=CARTESIAN_POINT('Ctrl Pts',(-5.07384754247588,-0.173399956222615,
392.713772597422));
#30853=CARTESIAN_POINT('Ctrl Pts',(-5.07367047787857,-0.000126645267989993,
392.708336844637));
#30854=CARTESIAN_POINT('Ctrl Pts',(-5.07318860167666,-3.10232113822501E-5,
393.791663155363));
#30855=CARTESIAN_POINT('Ctrl Pts',(-5.07309097404724,0.454497176795154,
393.777408049801));
#30856=CARTESIAN_POINT('Ctrl Pts',(-4.90058989979703,1.75010317897161,393.736776985753));
#30857=CARTESIAN_POINT('Ctrl Pts',(-3.81103098253419,3.66507401773587,393.669769963218));
#30858=CARTESIAN_POINT('Ctrl Pts',(-1.60160528615343,5.03900637156607,393.590642087758));
#30859=CARTESIAN_POINT('Ctrl Pts',(0.995622269493122,5.19282784249655,393.511514212298));
#30860=CARTESIAN_POINT('Ctrl Pts',(3.3517765903209,4.08929314110579,393.432386336838));
#30861=CARTESIAN_POINT('Ctrl Pts',(4.89635442297923,1.99560468778007,393.353258461378));
#30862=CARTESIAN_POINT('Ctrl Pts',(5.2553621496497,-0.581285972088894,393.274130585919));
#30863=CARTESIAN_POINT('Ctrl Pts',(4.34187207029457,-3.01742798265574,393.195002710459));
#30864=CARTESIAN_POINT('Ctrl Pts',(2.37707048734272,-4.72295041298575,393.115874834999));
#30865=CARTESIAN_POINT('Ctrl Pts',(-0.163298847893048,-5.28488961016167,
393.03674695954));
#30866=CARTESIAN_POINT('Ctrl Pts',(-2.66412810582239,-4.56718142195876,
392.957619084079));
#30867=CARTESIAN_POINT('Ctrl Pts',(-4.51988342344183,-2.74360684935247,
392.87849120862));
#30868=CARTESIAN_POINT('Ctrl Pts',(-5.05214048257081,-1.00431002992741,
392.823172565714));
#30869=CARTESIAN_POINT('Ctrl Pts',(-5.07399212128462,-0.0818852283646697,
392.794229881295));
#30870=CARTESIAN_POINT('Ctrl Pts',(-5.07393095917883,-7.88724074328884E-5,
392.791663155363));
#30871=CARTESIAN_POINT('Origin',(0.,0.,402.208336844637));
#30872=CARTESIAN_POINT('',(-5.07374340439062,0.000119799015104727,394.791663155363));
#30873=CARTESIAN_POINT('',(-5.07397904538501,5.86126803115486E-5,394.708336844637));
#30874=CARTESIAN_POINT('',(-5.0736,-1.59740085886799E-13,402.208336844637));
#30875=CARTESIAN_POINT('Ctrl Pts',(-5.07397904538501,5.86126803111056E-5,
394.708336844637));
#30876=CARTESIAN_POINT('Ctrl Pts',(-5.07401332726156,0.0584447346541764,
394.706504892919));
#30877=CARTESIAN_POINT('Ctrl Pts',(-5.05881623778616,0.957440994697868,
394.678296982715));
#30878=CARTESIAN_POINT('Ctrl Pts',(-4.55744811727866,2.68074456564335,394.623713114025));
#30879=CARTESIAN_POINT('Ctrl Pts',(-2.72712679296628,4.52984593810856,394.544585238565));
#30880=CARTESIAN_POINT('Ctrl Pts',(-0.236477452813074,5.28212108742541,
394.465457363106));
#30881=CARTESIAN_POINT('Ctrl Pts',(2.31143093653793,4.75541920271268,394.386329487645));
#30882=CARTESIAN_POINT('Ctrl Pts',(4.29966508998112,3.07727231195273,394.307201612186));
#30883=CARTESIAN_POINT('Ctrl Pts',(5.2468074522505,0.654015540275394,394.228073736726));
#30884=CARTESIAN_POINT('Ctrl Pts',(4.92352338499734,-1.92760012588128,394.148945861266));
#30885=CARTESIAN_POINT('Ctrl Pts',(3.40809070325859,-4.04247974964323,394.069817985806));
#30886=CARTESIAN_POINT('Ctrl Pts',(1.06744601535546,-5.17854069909805,393.990690110347));
#30887=CARTESIAN_POINT('Ctrl Pts',(-1.53166282285958,-5.06070486839363,
393.911562234887));
#30888=CARTESIAN_POINT('Ctrl Pts',(-3.75990519627929,-3.71750422769163,
393.832434359427));
#30889=CARTESIAN_POINT('Ctrl Pts',(-4.88811881465991,-1.79697577151505,
393.764692562677));
#30890=CARTESIAN_POINT('Ctrl Pts',(-5.07303815383513,-0.477899626088436,
393.723326724414));
#30891=CARTESIAN_POINT('Ctrl Pts',(-5.07320934784751,5.14726455259906E-5,
393.708336844637));
#30892=CARTESIAN_POINT('Ctrl Pts',(-5.07374340439062,0.000119799015104727,
394.791663155363));
#30893=CARTESIAN_POINT('Ctrl Pts',(-5.07389328700639,0.149964795759533,
394.786962176793));
#30894=CARTESIAN_POINT('Ctrl Pts',(-5.03087783588661,1.1404650386697,394.755885239737));
#30895=CARTESIAN_POINT('Ctrl Pts',(-4.40588160918252,2.92317155691987,394.698432344195));
#30896=CARTESIAN_POINT('Ctrl Pts',(-2.47828569661807,4.67063429431767,394.619304468735));
#30897=CARTESIAN_POINT('Ctrl Pts',(0.0493855336599835,5.28718126929493,
394.540176593275));
#30898=CARTESIAN_POINT('Ctrl Pts',(2.56509888521489,4.623525972068,394.461048717816));
#30899=CARTESIAN_POINT('Ctrl Pts',(4.45971656139522,2.84036140259214,394.381920842355));
#30900=CARTESIAN_POINT('Ctrl Pts',(5.27448866684743,0.369450955630144,394.302792966896));
#30901=CARTESIAN_POINT('Ctrl Pts',(4.81213180090847,-2.19091584411711,394.223665091436));
#30902=CARTESIAN_POINT('Ctrl Pts',(3.18459792440514,-4.2207891164085,394.144537215977));
#30903=CARTESIAN_POINT('Ctrl Pts',(0.785967069903959,-5.22866909168525,
394.065409340517));
#30904=CARTESIAN_POINT('Ctrl Pts',(-1.8029725289961,-4.97051453724898,393.986281465057));
#30905=CARTESIAN_POINT('Ctrl Pts',(-3.95535256793798,-3.50883324890547,
393.907153589597));
#30906=CARTESIAN_POINT('Ctrl Pts',(-4.9347894212868,-1.61393147469998,393.842280819699));
#30907=CARTESIAN_POINT('Ctrl Pts',(-5.0732716126465,-0.386507955183392,
393.803784008288));
#30908=CARTESIAN_POINT('Ctrl Pts',(-5.07318860167666,-3.10232113822501E-5,
393.791663155363));
#30909=CARTESIAN_POINT('Origin',(0.,0.,402.208336844637));
#30910=CARTESIAN_POINT('',(-5.07372845053928,-0.000121538385184292,395.791663155363));
#30911=CARTESIAN_POINT('',(-5.07344883766069,-0.000122970527678777,395.708336844637));
#30912=CARTESIAN_POINT('',(-5.0736,-1.59740085886799E-13,402.208336844637));
#30913=CARTESIAN_POINT('Ctrl Pts',(-5.07344883766069,-0.000122970527678921,
395.708336844637));
#30914=CARTESIAN_POINT('Ctrl Pts',(-5.07290495347366,0.594570911737787,
395.689683061425));
#30915=CARTESIAN_POINT('Ctrl Pts',(-4.82050381961586,2.03059585572183,395.644653319727));
#30916=CARTESIAN_POINT('Ctrl Pts',(-3.49440419526435,3.96810585645496,395.573247619542));
#30917=CARTESIAN_POINT('Ctrl Pts',(-1.17878204811896,5.1543377509575,395.494119744082));
#30918=CARTESIAN_POINT('Ctrl Pts',(1.42226240243777,5.09253320328156,395.414991868623));
#30919=CARTESIAN_POINT('Ctrl Pts',(3.67892986523249,3.79765714811298,395.335863993163));
#30920=CARTESIAN_POINT('Ctrl Pts',(5.0448061610774,1.58324210563915,395.256736117703));
#30921=CARTESIAN_POINT('Ctrl Pts',(5.18916725226161,-1.01452845991075,395.177608242243));
#30922=CARTESIAN_POINT('Ctrl Pts',(4.07705852165763,-3.36664797371096,395.098480366784));
#30923=CARTESIAN_POINT('Ctrl Pts',(1.97775844702931,-4.90359014326416,395.019352491324));
#30924=CARTESIAN_POINT('Ctrl Pts',(-0.60042266624658,-5.25321019851391,
394.940224615864));
#30925=CARTESIAN_POINT('Ctrl Pts',(-3.03322150067462,-4.33085350661488,
394.861096740404));
#30926=CARTESIAN_POINT('Ctrl Pts',(-4.69225666341608,-2.40548544911562,
394.783800816662));
#30927=CARTESIAN_POINT('Ctrl Pts',(-5.07351974582911,-0.782183276838963,
394.732880851406));
#30928=CARTESIAN_POINT('Ctrl Pts',(-5.07397904538501,5.86126803111056E-5,
394.708336844637));
#30929=CARTESIAN_POINT('Ctrl Pts',(-5.07372845053928,-0.000121538385184274,
395.791663155363));
#30930=CARTESIAN_POINT('Ctrl Pts',(-5.07303742094413,0.685929840247112,
395.770140345299));
#30931=CARTESIAN_POINT('Ctrl Pts',(-4.76110728643783,2.2133386185757,395.722241576749));
#30932=CARTESIAN_POINT('Ctrl Pts',(-3.27480540051438,4.15118950351341,395.647966849712));
#30933=CARTESIAN_POINT('Ctrl Pts',(-0.898448588333209,5.21051963238218,
395.568838974252));
#30934=CARTESIAN_POINT('Ctrl Pts',(1.69545248148909,5.00820981872071,395.489711098793));
#30935=CARTESIAN_POINT('Ctrl Pts',(3.87882816762124,3.59324599093717,395.410583223333));
#30936=CARTESIAN_POINT('Ctrl Pts',(5.12301066540628,1.30823790934658,395.331455347873));
#30937=CARTESIAN_POINT('Ctrl Pts',(5.12674204938754,-1.29353804132683,395.252327472413));
#30938=CARTESIAN_POINT('Ctrl Pts',(3.88911882751359,-3.58210544942458,395.173199596953));
#30939=CARTESIAN_POINT('Ctrl Pts',(1.70981070658587,-5.00332609900278,395.094071721494));
#30940=CARTESIAN_POINT('Ctrl Pts',(-0.883499401435098,-5.21307524528295,
395.014943846034));
#30941=CARTESIAN_POINT('Ctrl Pts',(-3.26288494670713,-4.16056565022955,
394.935815970574));
#30942=CARTESIAN_POINT('Ctrl Pts',(-4.7577955410693,-2.22302453301642,394.861389073684));
#30943=CARTESIAN_POINT('Ctrl Pts',(-5.07305233493801,-0.690776202139344,
394.81333813528));
#30944=CARTESIAN_POINT('Ctrl Pts',(-5.07374340439062,0.000119799015104727,
394.791663155363));
#30945=CARTESIAN_POINT('Origin',(0.,0.,402.208336844637));
#30946=CARTESIAN_POINT('',(-5.07319204280361,3.5344916511082E-5,396.791663155363));
#30947=CARTESIAN_POINT('',(-5.07333567377535,0.000103933621521292,396.708336844637));
#30948=CARTESIAN_POINT('',(-5.0736,-1.59740085886799E-13,402.208336844637));
#30949=CARTESIAN_POINT('Ctrl Pts',(-5.07333567377534,0.000103933621520939,
396.708336844637));
#30950=CARTESIAN_POINT('Ctrl Pts',(-5.07355255518605,0.290225038825201,
396.699237188418));
#30951=CARTESIAN_POINT('Ctrl Pts',(-4.9781337482961,1.42114034886055,396.663761573712));
#30952=CARTESIAN_POINT('Ctrl Pts',(-4.14865431030898,3.27801650109757,396.601910000519));
#30953=CARTESIAN_POINT('Ctrl Pts',(-2.08295867375766,4.85983620416686,396.52278212506));
#30954=CARTESIAN_POINT('Ctrl Pts',(0.487090472013812,5.26492807548086,396.4436542496));
#30955=CARTESIAN_POINT('Ctrl Pts',(2.93919882905869,4.3952059122609,396.36452637414));
#30956=CARTESIAN_POINT('Ctrl Pts',(4.67962948341671,2.46125835008237,396.28539849868));
#30957=CARTESIAN_POINT('Ctrl Pts',(5.2869663411736,-0.0686416434144708,
396.206270623221));
#30958=CARTESIAN_POINT('Ctrl Pts',(4.61415296796628,-2.58192121415839,396.127142747761));
#30959=CARTESIAN_POINT('Ctrl Pts',(2.82409983825713,-4.47003186470401,396.048014872301));
#30960=CARTESIAN_POINT('Ctrl Pts',(0.350238296140284,-5.27579926682488,
395.968886996841));
#30961=CARTESIAN_POINT('Ctrl Pts',(-2.20842757548492,-4.80412035775031,
395.889759121382));
#30962=CARTESIAN_POINT('Ctrl Pts',(-4.23235974759556,-3.16920427471092,
395.810631245921));
#30963=CARTESIAN_POINT('Ctrl Pts',(-4.99595812955649,-1.33323876922698,
395.750157153674));
#30964=CARTESIAN_POINT('Ctrl Pts',(-5.07367399139889,-0.246310585215766,
395.716059019912));
#30965=CARTESIAN_POINT('Ctrl Pts',(-5.07344883766069,-0.000122970527678921,
395.708336844637));
#30966=CARTESIAN_POINT('Ctrl Pts',(-5.07319204280361,3.53449165107697E-5,
396.791663155363));
#30967=CARTESIAN_POINT('Ctrl Pts',(-5.07328550820695,0.381659555984483,
396.779694472291));
#30968=CARTESIAN_POINT('Ctrl Pts',(-4.93711373649749,1.60422160810075,396.741349830733));
#30969=CARTESIAN_POINT('Ctrl Pts',(-3.96540078941456,3.49747355738801,396.676629230689));
#30970=CARTESIAN_POINT('Ctrl Pts',(-1.81722218927578,4.96532256959422,396.597501355229));
#30971=CARTESIAN_POINT('Ctrl Pts',(0.770966287074601,5.23090199578547,396.51837347977));
#30972=CARTESIAN_POINT('Ctrl Pts',(3.17247820700774,4.22990623198423,396.43924560431));
#30973=CARTESIAN_POINT('Ctrl Pts',(4.8058277352491,2.20470961453625,396.36011772885));
#30974=CARTESIAN_POINT('Ctrl Pts',(5.275526676699,-0.354320460537079,396.28098985339));
#30975=CARTESIAN_POINT('Ctrl Pts',(4.46784531008081,-2.82755777845599,396.201861977931));
#30976=CARTESIAN_POINT('Ctrl Pts',(2.57835013256881,-4.61614940174172,396.122734102471));
#30977=CARTESIAN_POINT('Ctrl Pts',(0.0645507123742531,-5.2870178655694,
396.043606227011));
#30978=CARTESIAN_POINT('Ctrl Pts',(-2.46487858023149,-4.67772362266456,
395.964478351551));
#30979=CARTESIAN_POINT('Ctrl Pts',(-4.39747886350376,-2.93579705537622,
395.885350476092));
#30980=CARTESIAN_POINT('Ctrl Pts',(-5.02925481295834,-1.15017365368594,
395.827745410695));
#30981=CARTESIAN_POINT('Ctrl Pts',(-5.0738842698389,-0.154818306903111,
395.796516303786));
#30982=CARTESIAN_POINT('Ctrl Pts',(-5.07372845053928,-0.000121538385184274,
395.791663155363));
#30983=CARTESIAN_POINT('Origin',(0.,0.,402.208336844637));
#30984=CARTESIAN_POINT('',(-5.0739418421154,7.48951186854696E-5,397.791663155363));
#30985=CARTESIAN_POINT('',(-5.07403169783887,-1.51513653288439E-5,397.708336844637));
#30986=CARTESIAN_POINT('',(-5.0736,-1.59740085886799E-13,402.208336844637));
#30987=CARTESIAN_POINT('Ctrl Pts',(-5.07403169783887,-1.51513653288493E-5,
397.708336844637));
#30988=CARTESIAN_POINT('Ctrl Pts',(-5.07388968734652,0.82610348406882,397.682415356923));
#30989=CARTESIAN_POINT('Ctrl Pts',(-4.6586701596041,2.49296234041498,397.630117910723));
#30990=CARTESIAN_POINT('Ctrl Pts',(-2.91976153402742,4.40814216562114,397.551444506037));
#30991=CARTESIAN_POINT('Ctrl Pts',(-0.463836508948714,5.26702766851281,
397.472316630577));
#30992=CARTESIAN_POINT('Ctrl Pts',(2.10439874769627,4.85059075563045,397.393188755117));
#30993=CARTESIAN_POINT('Ctrl Pts',(4.16308914079174,3.25966464129901,397.314060879657));
#30994=CARTESIAN_POINT('Ctrl Pts',(5.21375731827273,0.87946540242969,397.234933004198));
#30995=CARTESIAN_POINT('Ctrl Pts',(5.00200160188481,-1.71368163398425,397.155805128738));
#30996=CARTESIAN_POINT('Ctrl Pts',(3.57909508696266,-3.89188940315535,397.076677253278));
#30997=CARTESIAN_POINT('Ctrl Pts',(1.28957072230382,-5.12774142484681,396.997549377819));
#30998=CARTESIAN_POINT('Ctrl Pts',(-1.31220156516579,-5.12199685867627,
396.918421502358));
#30999=CARTESIAN_POINT('Ctrl Pts',(-3.59624625077107,-3.87604665499891,
396.839293626899));
#31000=CARTESIAN_POINT('Ctrl Pts',(-4.84699459687274,-1.94278943218135,
396.769265407658));
#31001=CARTESIAN_POINT('Ctrl Pts',(-5.07292390999909,-0.550710271536964,
396.725613146904));
#31002=CARTESIAN_POINT('Ctrl Pts',(-5.07333567377534,0.000103933621520939,
396.708336844637));
#31003=CARTESIAN_POINT('Ctrl Pts',(-5.0739418421154,7.48951186850533E-5,
397.791663155363));
#31004=CARTESIAN_POINT('Ctrl Pts',(-5.07399707454689,0.0770308345755981,
397.789248599284));
#31005=CARTESIAN_POINT('Ctrl Pts',(-5.05354999565328,0.994603307815543,
397.760458084718));
#31006=CARTESIAN_POINT('Ctrl Pts',(-4.52773440061085,2.73063104480294,397.705291611666));
#31007=CARTESIAN_POINT('Ctrl Pts',(-2.67721733102668,4.55952103490808,397.626163736206));
#31008=CARTESIAN_POINT('Ctrl Pts',(-0.178456984770649,5.28439947486034,
397.547035860747));
#31009=CARTESIAN_POINT('Ctrl Pts',(2.36351372741711,4.72974920747697,397.467907985287));
#31010=CARTESIAN_POINT('Ctrl Pts',(4.33319922937441,3.02986949287705,397.388780109827));
#31011=CARTESIAN_POINT('Ctrl Pts',(5.25367321071018,0.596357694998765,397.309652234368));
#31012=CARTESIAN_POINT('Ctrl Pts',(4.90205833425909,-1.98155211711401,397.230524358907));
#31013=CARTESIAN_POINT('Ctrl Pts',(3.36349224536493,-4.07966231699243,397.151396483448));
#31014=CARTESIAN_POINT('Ctrl Pts',(1.01051291891753,-5.18995070747486,397.072268607988));
#31015=CARTESIAN_POINT('Ctrl Pts',(-1.58714516337332,-5.04357957562867,
396.993140732529));
#31016=CARTESIAN_POINT('Ctrl Pts',(-3.80050266261658,-3.67599023621695,
396.914012857068));
#31017=CARTESIAN_POINT('Ctrl Pts',(-4.89803666817087,-1.7598107945601,396.84685366468));
#31018=CARTESIAN_POINT('Ctrl Pts',(-5.07307953403386,-0.459343943622233,
396.806070430778));
#31019=CARTESIAN_POINT('Ctrl Pts',(-5.07319204280361,3.53449165107697E-5,
396.791663155363));
#31020=CARTESIAN_POINT('Origin',(0.,0.,402.208336844637));
#31021=CARTESIAN_POINT('',(-5.07350261625086,-0.000127405426567639,398.791663155363));
#31022=CARTESIAN_POINT('',(-5.07327504304777,-8.56681209023223E-5,398.708336844637));
#31023=CARTESIAN_POINT('',(-5.0736,-1.59740085886799E-13,402.208336844637));
#31024=CARTESIAN_POINT('Ctrl Pts',(-5.07327504304777,-8.56681209025073E-5,
398.708336844637));
#31025=CARTESIAN_POINT('Ctrl Pts',(-5.07295870657578,0.521766948573649,
398.691969483916));
#31026=CARTESIAN_POINT('Ctrl Pts',(-4.86376568515234,1.88483153888263,398.649226164708));
#31027=CARTESIAN_POINT('Ctrl Pts',(-3.66212405277363,3.81386578025083,398.580106887014));
#31028=CARTESIAN_POINT('Ctrl Pts',(-1.39976059402284,5.09876407058445,398.500979011554));
#31029=CARTESIAN_POINT('Ctrl Pts',(1.2015314169661,5.14908215334412,398.421851136094));
#31030=CARTESIAN_POINT('Ctrl Pts',(3.51189274640949,3.9526363487746,398.342723260634));
#31031=CARTESIAN_POINT('Ctrl Pts',(4.97190814582059,1.79912594262636,398.263595385175));
#31032=CARTESIAN_POINT('Ctrl Pts',(5.22805937238099,-0.790012637095727,
398.184467509715));
#31033=CARTESIAN_POINT('Ctrl Pts',(4.21832370253235,-3.18786290617544,398.105339634255));
#31034=CARTESIAN_POINT('Ctrl Pts',(2.18719169429123,-4.81382563667766,398.026211758795));
#31035=CARTESIAN_POINT('Ctrl Pts',(-0.37353210098369,-5.27420122269227,
397.947083883336));
#31036=CARTESIAN_POINT('Ctrl Pts',(-2.84381136257153,-4.45751743709679,
397.867956007876));
#31037=CARTESIAN_POINT('Ctrl Pts',(-4.62550939672404,-2.56152056184034,
397.788828132416));
#31038=CARTESIAN_POINT('Ctrl Pts',(-5.07044892396789,-0.869584543074369,
397.73562174467));
#31039=CARTESIAN_POINT('Ctrl Pts',(-5.07403418765037,-0.0144991493159696,
397.70879131541));
#31040=CARTESIAN_POINT('Ctrl Pts',(-5.07403169783887,-1.51513653288493E-5,
397.708336844637));
#31041=CARTESIAN_POINT('Ctrl Pts',(-5.07350261625086,-0.000127405426567848,
398.791663155363));
#31042=CARTESIAN_POINT('Ctrl Pts',(-5.07291128030502,0.613121580961722,
398.77242676779));
#31043=CARTESIAN_POINT('Ctrl Pts',(-4.80890661569317,2.06772180201207,398.72681442173));
#31044=CARTESIAN_POINT('Ctrl Pts',(-3.45061727711166,4.00624076891526,398.654826117184));
#31045=CARTESIAN_POINT('Ctrl Pts',(-1.12210802579434,5.16697186848109,398.575698241724));
#31046=CARTESIAN_POINT('Ctrl Pts',(1.47810086651078,5.07660738405961,398.496570366264));
#31047=CARTESIAN_POINT('Ctrl Pts',(3.72041242270134,3.75702756318667,398.417442490805));
#31048=CARTESIAN_POINT('Ctrl Pts',(5.06188850671742,1.52774652711538,398.338314615344));
#31049=CARTESIAN_POINT('Ctrl Pts',(5.17771318239863,-1.0714527081918,398.259186739885));
#31050=CARTESIAN_POINT('Ctrl Pts',(4.03984144729043,-3.41121763982034,398.180058864425));
#31051=CARTESIAN_POINT('Ctrl Pts',(1.92378985850489,-4.92501342998799,398.100930988965));
#31052=CARTESIAN_POINT('Ctrl Pts',(-0.658075180315041,-5.24629981628919,
398.021803113506));
#31053=CARTESIAN_POINT('Ctrl Pts',(-3.08059835091328,-4.29728268859095,
397.942675238046));
#31054=CARTESIAN_POINT('Ctrl Pts',(-4.70604526230202,-2.36846041862021,
397.865961918665));
#31055=CARTESIAN_POINT('Ctrl Pts',(-5.07339373038246,-0.763615063923845,
397.81562455777));
#31056=CARTESIAN_POINT('Ctrl Pts',(-5.0739418421154,7.48951186850533E-5,
397.791663155363));
#31057=CARTESIAN_POINT('Origin',(0.,0.,402.208336844637));
#31058=CARTESIAN_POINT('',(-5.07330191118131,0.000105688062508047,399.791663155363));
#31059=CARTESIAN_POINT('',(-5.07353386009457,0.000128968315485679,399.708336844637));
#31060=CARTESIAN_POINT('',(-5.0736,-1.59740085886799E-13,402.208336844637));
#31061=CARTESIAN_POINT('',(-1.31303618635556,-4.90075024188347,400.));
#31062=CARTESIAN_POINT('Ctrl Pts',(-1.31303618635555,-4.90075024188347,
400.));
#31063=CARTESIAN_POINT('Ctrl Pts',(-2.12521319086393,-4.68314727417224,
399.973624041513));
#31064=CARTESIAN_POINT('Ctrl Pts',(-3.63845957255092,-3.83644859241818,
399.92087212454));
#31065=CARTESIAN_POINT('Ctrl Pts',(-4.85784323874867,-1.90558193017489,
399.851426509661));
#31066=CARTESIAN_POINT('Ctrl Pts',(-5.07295978880057,-0.532132079631421,
399.808356853268));
#31067=CARTESIAN_POINT('Ctrl Pts',(-5.07330191118131,0.000105688062508012,
399.791663155363));
#31068=CARTESIAN_POINT('',(1.31318543090008,-4.90112867346845,400.));
#31069=CARTESIAN_POINT('Origin',(0.,0.,400.));
#31070=CARTESIAN_POINT('Ctrl Pts',(1.31318543090008,-4.90112867346845,400.));
#31071=CARTESIAN_POINT('Ctrl Pts',(0.546344064728336,-5.10618409880194,
399.975093589943));
#31072=CARTESIAN_POINT('Ctrl Pts',(-1.13368018453605,-5.15247589033718,
399.923811221401));
#31073=CARTESIAN_POINT('Ctrl Pts',(-3.42590833126468,-4.02739560525483,
399.84615289437));
#31074=CARTESIAN_POINT('Ctrl Pts',(-4.8023079180703,-2.08851222235156,399.77383825264));
#31075=CARTESIAN_POINT('Ctrl Pts',(-5.07291903260815,-0.623512076348425,
399.727899569395));
#31076=CARTESIAN_POINT('Ctrl Pts',(-5.07353386009457,0.000128968315485402,
399.708336844637));
#31077=CARTESIAN_POINT('Origin',(0.,0.,20.5));
#31078=CARTESIAN_POINT('',(4.51807726312575,-5.77016670283426E-5,39.6125833024919));
#31079=CARTESIAN_POINT('',(4.51743491291879,0.00013078575649096,39.887416697508));
#31080=CARTESIAN_POINT('',(4.51775,5.53264807684796E-16,20.5));
#31081=CARTESIAN_POINT('',(3.43378788736186,2.93584158413001,40.));
#31082=CARTESIAN_POINT('Ctrl Pts',(4.51743491291879,0.00013078575649096,
39.887416697508));
#31083=CARTESIAN_POINT('Ctrl Pts',(4.51757757737092,0.314458352690014,39.8984871683209));
#31084=CARTESIAN_POINT('Ctrl Pts',(4.48524528727997,0.628740973485904,39.9095576391338));
#31085=CARTESIAN_POINT('Ctrl Pts',(4.42014586550123,0.936043740039879,39.9206281099466));
#31086=CARTESIAN_POINT('Ctrl Pts',(4.26456488388791,1.67046602470259,39.9470854066311));
#31087=CARTESIAN_POINT('Ctrl Pts',(3.92183073605335,2.36502208507763,39.9735427033156));
#31088=CARTESIAN_POINT('Ctrl Pts',(3.43378788736169,2.9358415841302,40.));
#31089=CARTESIAN_POINT('',(4.51775,5.53264807684796E-16,40.));
#31090=CARTESIAN_POINT('Origin',(0.,0.,40.));
#31091=CARTESIAN_POINT('',(4.51775,-5.53264807684796E-16,41.));
#31092=CARTESIAN_POINT('',(4.51775,5.53264807684796E-16,20.5));
#31093=CARTESIAN_POINT('Origin',(0.,0.,41.));
#31094=CARTESIAN_POINT('',(-3.4340910891448,2.93606647242268,40.));
#31095=CARTESIAN_POINT('Origin',(0.,0.,40.));
#31096=CARTESIAN_POINT('Ctrl Pts',(-3.4340910891448,2.93606647242268,40.));
#31097=CARTESIAN_POINT('Ctrl Pts',(-2.96705577784696,3.4818800261268,39.974686898954));
#31098=CARTESIAN_POINT('Ctrl Pts',(-2.36757358452893,3.91460873741648,39.949373797908));
#31099=CARTESIAN_POINT('Ctrl Pts',(-1.70215900486053,4.18523117809469,39.9240606968621));
#31100=CARTESIAN_POINT('Ctrl Pts',(-1.00666654344796,4.46808621784234,39.8976034001776));
#31101=CARTESIAN_POINT('Ctrl Pts',(-0.239146468763622,4.57384880856985,
39.8711461034931));
#31102=CARTESIAN_POINT('Ctrl Pts',(0.506923795872781,4.48961228541996,39.8446888068086));
#31103=CARTESIAN_POINT('Ctrl Pts',(1.25299406050918,4.40537576227008,39.8182315101241));
#31104=CARTESIAN_POINT('Ctrl Pts',(1.97761451509765,4.1311401252428,39.7917742134397));
#31105=CARTESIAN_POINT('Ctrl Pts',(2.59252418705981,3.70032015205324,39.7653169167552));
#31106=CARTESIAN_POINT('Ctrl Pts',(3.2074338590219,3.26950017886373,39.7388596200708));
#31107=CARTESIAN_POINT('Ctrl Pts',(3.71263274835769,2.68209586951196,39.7124023233863));
#31108=CARTESIAN_POINT('Ctrl Pts',(4.0465897798431,2.00964543895381,39.6859450267018));
#31109=CARTESIAN_POINT('Ctrl Pts',(4.35525905337691,1.38811402527266,39.6614911186319));
#31110=CARTESIAN_POINT('Ctrl Pts',(4.51763802149368,0.693928511700309,39.6370372105619));
#31111=CARTESIAN_POINT('Ctrl Pts',(4.51807726312575,-5.77016670283426E-5,
39.6125833024919));
#31112=CARTESIAN_POINT('Origin',(0.,0.,20.5));
#31113=CARTESIAN_POINT('',(4.5173663293175,-1.61899228900975E-5,38.6125833024919));
#31114=CARTESIAN_POINT('',(4.51813342681501,1.37750411066654E-5,38.887416697508));
#31115=CARTESIAN_POINT('',(4.51775,5.53264807684796E-16,20.5));
#31116=CARTESIAN_POINT('Ctrl Pts',(4.51813342681501,1.37750411066654E-5,
38.887416697508));
#31117=CARTESIAN_POINT('Ctrl Pts',(4.51813570137199,0.0130379216071904,
38.8878756447561));
#31118=CARTESIAN_POINT('Ctrl Pts',(4.51808056261842,0.0260620488529043,
38.8883345920043));
#31119=CARTESIAN_POINT('Ctrl Pts',(4.51796789313227,0.039085678406741,38.8887935392524));
#31120=CARTESIAN_POINT('Ctrl Pts',(4.5114727457387,0.789869199672342,38.9152508359369));
#31121=CARTESIAN_POINT('Ctrl Pts',(4.31378754306059,1.53899875733816,38.9417081326213));
#31122=CARTESIAN_POINT('Ctrl Pts',(3.94899006576268,2.19523105353971,38.9681654293058));
#31123=CARTESIAN_POINT('Ctrl Pts',(3.58419258846473,2.85146334974134,38.9946227259902));
#31124=CARTESIAN_POINT('Ctrl Pts',(3.05228283654696,3.41479838447868,39.0210800226747));
#31125=CARTESIAN_POINT('Ctrl Pts',(2.4180469390752,3.81662285121831,39.0475373193592));
#31126=CARTESIAN_POINT('Ctrl Pts',(1.78381104160343,4.21844731795794,39.0739946160436));
#31127=CARTESIAN_POINT('Ctrl Pts',(1.04724899857768,4.45876121669985,39.1004519127281));
#31128=CARTESIAN_POINT('Ctrl Pts',(0.298073044029034,4.50829405706009,39.1269092094126));
#31129=CARTESIAN_POINT('Ctrl Pts',(-0.45110291051953,4.55782689742033,39.1533665060971));
#31130=CARTESIAN_POINT('Ctrl Pts',(-1.21289277659099,4.41657867939895,39.1798238027815));
#31131=CARTESIAN_POINT('Ctrl Pts',(-1.89451099954058,4.10175426806426,39.206281099466));
#31132=CARTESIAN_POINT('Ctrl Pts',(-2.57612922249017,3.78692985672956,39.2327383961504));
#31133=CARTESIAN_POINT('Ctrl Pts',(-3.17757580231788,3.29852925208155,39.2591956928349));
#31134=CARTESIAN_POINT('Ctrl Pts',(-3.62559595151898,2.69603724086566,39.2856529895194));
#31135=CARTESIAN_POINT('Ctrl Pts',(-4.07361610072013,2.0935452296497,39.3121102862039));
#31136=CARTESIAN_POINT('Ctrl Pts',(-4.36820981929462,1.37696181186582,39.3385675828883));
#31137=CARTESIAN_POINT('Ctrl Pts',(-4.4734945205513,0.633569578843569,39.3650248795728));
#31138=CARTESIAN_POINT('Ctrl Pts',(-4.57877922180797,-0.109822654178678,
39.3914821762572));
#31139=CARTESIAN_POINT('Ctrl Pts',(-4.49475490574683,-0.880023702439293,
39.4179394729417));
#31140=CARTESIAN_POINT('Ctrl Pts',(-4.23165828048028,-1.5832305850457,39.4443967696262));
#31141=CARTESIAN_POINT('Ctrl Pts',(-3.96856165521376,-2.28643746765202,
39.4708540663107));
#31142=CARTESIAN_POINT('Ctrl Pts',(-3.52639272074186,-2.92265018460415,
39.4973113629951));
#31143=CARTESIAN_POINT('Ctrl Pts',(-2.95900217961984,-3.41436616507676,
39.5237686596796));
#31144=CARTESIAN_POINT('Ctrl Pts',(-2.39161163849769,-3.90608214554949,
39.5502259563641));
#31145=CARTESIAN_POINT('Ctrl Pts',(-1.69899949072535,-4.25330138954263,
39.5766832530485));
#31146=CARTESIAN_POINT('Ctrl Pts',(-0.965534545329121,-4.41375671437606,
39.603140549733));
#31147=CARTESIAN_POINT('Ctrl Pts',(-0.232069599933061,-4.57421203920946,
39.6295978464175));
#31148=CARTESIAN_POINT('Ctrl Pts',(0.542248143086867,-4.54790344488323,
39.6560551431019));
#31149=CARTESIAN_POINT('Ctrl Pts',(1.26312545635919,-4.33799038903366,39.6825124397864));
#31150=CARTESIAN_POINT('Ctrl Pts',(1.98400276963152,-4.12807733318409,39.7089697364709));
#31151=CARTESIAN_POINT('Ctrl Pts',(2.65143965315624,-3.73455981581118,39.7354270331553));
#31152=CARTESIAN_POINT('Ctrl Pts',(3.18410908512153,-3.20545326780569,39.7618843298398));
#31153=CARTESIAN_POINT('Ctrl Pts',(3.71677851708688,-2.67634671980015,39.7883416265243));
#31154=CARTESIAN_POINT('Ctrl Pts',(4.11468049749276,-2.01165114116199,39.8147989232087));
#31155=CARTESIAN_POINT('Ctrl Pts',(4.32941757999969,-1.29215909736769,39.8412562198932));
#31156=CARTESIAN_POINT('Ctrl Pts',(4.45430267828147,-0.873722590951435,
39.8566430457648));
#31157=CARTESIAN_POINT('Ctrl Pts',(4.51723662387398,-0.436752488749845,
39.8720298716364));
#31158=CARTESIAN_POINT('Ctrl Pts',(4.51743491291879,0.00013078575649096,
39.887416697508));
#31159=CARTESIAN_POINT('Ctrl Pts',(4.51807726312575,-5.77016670283426E-5,
39.6125833024919));
#31160=CARTESIAN_POINT('Ctrl Pts',(4.51811324803589,-0.0569125845144851,
39.6105799138774));
#31161=CARTESIAN_POINT('Ctrl Pts',(4.51706233879025,-0.113766129714702,
39.6085765252629));
#31162=CARTESIAN_POINT('Ctrl Pts',(4.51491593042487,-0.170578278221581,
39.6065731366484));
#31163=CARTESIAN_POINT('Ctrl Pts',(4.48656987588623,-0.920855013074376,
39.580115839964));
#31164=CARTESIAN_POINT('Ctrl Pts',(4.26716259317389,-1.66391193101533,39.5536585432795));
#31165=CARTESIAN_POINT('Ctrl Pts',(3.88341809255801,-2.30924747945226,39.527201246595));
#31166=CARTESIAN_POINT('Ctrl Pts',(3.49967359194214,-2.9545830278892,39.5007439499106));
#31167=CARTESIAN_POINT('Ctrl Pts',(2.95159187342274,-3.50219720682209,39.4742866532261));
#31168=CARTESIAN_POINT('Ctrl Pts',(2.305928447501,-3.88539017854137,39.4478293565416));
#31169=CARTESIAN_POINT('Ctrl Pts',(1.66026502157934,-4.2685831502606,39.4213720598571));
#31170=CARTESIAN_POINT('Ctrl Pts',(0.917019888255395,-4.48735491476624,
39.3949147631727));
#31171=CARTESIAN_POINT('Ctrl Pts',(0.16671960730651,-4.51505986234427,39.3684574664882));
#31172=CARTESIAN_POINT('Ctrl Pts',(-0.58358067364246,-4.54276480992229,
39.3420001698038));
#31173=CARTESIAN_POINT('Ctrl Pts',(-1.34093610221634,-4.37940294057267,
39.3155428731193));
#31174=CARTESIAN_POINT('Ctrl Pts',(-2.0131016916631,-4.0448712583889,39.2890855764348));
#31175=CARTESIAN_POINT('Ctrl Pts',(-2.68526728110987,-3.71033957620513,
39.2626282797503));
#31176=CARTESIAN_POINT('Ctrl Pts',(-3.27224303142949,-3.20463808118724,
39.2361709830659));
#31177=CARTESIAN_POINT('Ctrl Pts',(-3.70253591076623,-2.58936080975925,
39.2097136863814));
#31178=CARTESIAN_POINT('Ctrl Pts',(-4.13282879010292,-1.97408353833133,
39.1832563896969));
#31179=CARTESIAN_POINT('Ctrl Pts',(-4.40643879845674,-1.24923049049336,
39.1567990930125));
#31180=CARTESIAN_POINT('Ctrl Pts',(-4.49004055820742,-0.503087883692005,
39.130341796328));
#31181=CARTESIAN_POINT('Ctrl Pts',(-4.5736423179581,0.243054723109393,39.1038844996435));
#31182=CARTESIAN_POINT('Ctrl Pts',(-4.46723582910558,1.01048688887427,39.0774272029591));
#31183=CARTESIAN_POINT('Ctrl Pts',(-4.18378127438633,1.70573618195759,39.0509699062746));
#31184=CARTESIAN_POINT('Ctrl Pts',(-3.90032671966707,2.40098547504095,39.0245126095901));
#31185=CARTESIAN_POINT('Ctrl Pts',(-3.43982409908106,3.02405189544285,38.9980553129056));
#31186=CARTESIAN_POINT('Ctrl Pts',(-2.85836212737563,3.49904666560209,38.9715980162212));
#31187=CARTESIAN_POINT('Ctrl Pts',(-2.27690015567025,3.97404143576128,38.9451407195367));
#31188=CARTESIAN_POINT('Ctrl Pts',(-1.5744788328455,4.30096455567782,38.9186834228523));
#31189=CARTESIAN_POINT('Ctrl Pts',(-0.836652295869176,4.43999713904635,
38.8922261261678));
#31190=CARTESIAN_POINT('Ctrl Pts',(-0.0988257588928058,4.57902972241489,
38.8657688294833));
#31191=CARTESIAN_POINT('Ctrl Pts',(0.67440599223512,4.53017176923538,38.8393115327988));
#31192=CARTESIAN_POINT('Ctrl Pts',(1.38886418452495,4.29937413054893,38.8128542361144));
#31193=CARTESIAN_POINT('Ctrl Pts',(2.10332237681477,4.06857649186248,38.7863969394299));
#31194=CARTESIAN_POINT('Ctrl Pts',(2.75900701026648,3.6558391676691,38.7599396427455));
#31195=CARTESIAN_POINT('Ctrl Pts',(3.27605642296661,3.11143310386805,38.733482346061));
#31196=CARTESIAN_POINT('Ctrl Pts',(3.79310583566678,2.56702704006697,38.7070250493765));
#31197=CARTESIAN_POINT('Ctrl Pts',(4.17152002761535,1.89095223665823,38.680567752692));
#31198=CARTESIAN_POINT('Ctrl Pts',(4.36520856862573,1.1655538582636,38.6541104560076));
#31199=CARTESIAN_POINT('Ctrl Pts',(4.46654587798484,0.786027431472861,38.6402680715023));
#31200=CARTESIAN_POINT('Ctrl Pts',(4.51731724698707,0.392999398715342,38.6264256869971));
#31201=CARTESIAN_POINT('Ctrl Pts',(4.5173663293175,-1.61899228900975E-5,
38.6125833024919));
#31202=CARTESIAN_POINT('Origin',(0.,0.,20.5));
#31203=CARTESIAN_POINT('',(4.51799626797168,8.54686663623316E-5,37.6125833024919));
#31204=CARTESIAN_POINT('',(4.51744515673179,-7.51896715610657E-5,37.887416697508));
#31205=CARTESIAN_POINT('',(4.51775,5.53264807684796E-16,20.5));
#31206=CARTESIAN_POINT('Ctrl Pts',(4.51744515673179,-7.51896715610657E-5,
37.887416697508));
#31207=CARTESIAN_POINT('Ctrl Pts',(4.51717073079397,0.462828384782965,37.9037214178759));
#31208=CARTESIAN_POINT('Ctrl Pts',(4.44640538068968,0.925813963613659,37.9200261382437));
#31209=CARTESIAN_POINT('Ctrl Pts',(4.30642900683072,1.36683241594085,37.9363308586115));
#31210=CARTESIAN_POINT('Ctrl Pts',(4.07929254766704,2.0824629679108,37.962788155296));
#31211=CARTESIAN_POINT('Ctrl Pts',(3.66991785444932,2.74025229569321,37.9892454519805));
#31212=CARTESIAN_POINT('Ctrl Pts',(3.12816631171535,3.26008238708871,38.0157027486649));
#31213=CARTESIAN_POINT('Ctrl Pts',(2.58641476898142,3.77991247848417,38.0421600453494));
#31214=CARTESIAN_POINT('Ctrl Pts',(1.91228637673127,4.16178333349271,38.0686173420339));
#31215=CARTESIAN_POINT('Ctrl Pts',(1.18788922711554,4.35918350473768,38.0950746387183));
#31216=CARTESIAN_POINT('Ctrl Pts',(0.463492077499819,4.55658367598265,38.1215319354028));
#31217=CARTESIAN_POINT('Ctrl Pts',(-0.311173829481454,4.56951316346404,
38.1479892320873));
#31218=CARTESIAN_POINT('Ctrl Pts',(-1.04175504380602,4.39639716966122,38.1744465287717));
#31219=CARTESIAN_POINT('Ctrl Pts',(-1.77233625813064,4.2232811758584,38.2009038254562));
#31220=CARTESIAN_POINT('Ctrl Pts',(-2.45883277979851,3.86411970077134,38.2273611221407));
#31221=CARTESIAN_POINT('Ctrl Pts',(-3.01763009204679,3.36265821505168,38.2538184188251));
#31222=CARTESIAN_POINT('Ctrl Pts',(-3.57642740429506,2.86119672933201,38.2802757155096));
#31223=CARTESIAN_POINT('Ctrl Pts',(-4.00752550712371,2.21743523297976,38.3067330121941));
#31224=CARTESIAN_POINT('Ctrl Pts',(-4.25841712907836,1.50978316287097,38.3331903088785));
#31225=CARTESIAN_POINT('Ctrl Pts',(-4.50930875103297,0.802131092762298,
38.359647605563));
#31226=CARTESIAN_POINT('Ctrl Pts',(-4.57999389211364,0.0305884488970126,
38.3861049022475));
#31227=CARTESIAN_POINT('Ctrl Pts',(-4.46186317968564,-0.710871726876464,
38.412562198932));
#31228=CARTESIAN_POINT('Ctrl Pts',(-4.34373246725763,-1.45233190264998,
38.4390194956164));
#31229=CARTESIAN_POINT('Ctrl Pts',(-4.03678590132095,-2.16370961033178,
38.4654767923008));
#31230=CARTESIAN_POINT('Ctrl Pts',(-3.57840923518433,-2.75835983566992,
38.4919340889853));
#31231=CARTESIAN_POINT('Ctrl Pts',(-3.12003256904766,-3.35301006100813,
38.5183913856698));
#31232=CARTESIAN_POINT('Ctrl Pts',(-2.51022580271103,-3.83093280400264,
38.5448486823543));
#31233=CARTESIAN_POINT('Ctrl Pts',(-1.82326272299569,-4.13391759737145,
38.5713059790388));
#31234=CARTESIAN_POINT('Ctrl Pts',(-1.13629964328034,-4.43690239074026,
38.5977632757232));
#31235=CARTESIAN_POINT('Ctrl Pts',(-0.372180250186292,-4.56494923448336,
38.6242205724077));
#31236=CARTESIAN_POINT('Ctrl Pts',(0.376026555300945,-4.50246217629699,
38.6506778690921));
#31237=CARTESIAN_POINT('Ctrl Pts',(1.12423336078818,-4.4399751181106,38.6771351657766));
#31238=CARTESIAN_POINT('Ctrl Pts',(1.85652757866858,-4.18695415799474,38.7035924624611));
#31239=CARTESIAN_POINT('Ctrl Pts',(2.48371659230794,-3.77421694705527,38.7300497591456));
#31240=CARTESIAN_POINT('Ctrl Pts',(3.1109056059473,-3.3614797361158,38.7565070558301));
#31241=CARTESIAN_POINT('Ctrl Pts',(3.63298941534561,-2.78902627435273,38.7829643525145));
#31242=CARTESIAN_POINT('Ctrl Pts',(3.98637877399025,-2.12658080103845,38.8094216491989));
#31243=CARTESIAN_POINT('Ctrl Pts',(4.33363798730682,-1.47562658212673,38.8354199986353));
#31244=CARTESIAN_POINT('Ctrl Pts',(4.51800457817832,-0.737775404274226,
38.8614183480717));
#31245=CARTESIAN_POINT('Ctrl Pts',(4.51813342681501,1.37750411066654E-5,
38.887416697508));
#31246=CARTESIAN_POINT('Ctrl Pts',(4.5173663293175,-1.61899228900975E-5,
38.6125833024919));
#31247=CARTESIAN_POINT('Ctrl Pts',(4.51741105927625,-0.358181153038861,
38.5999683903127));
#31248=CARTESIAN_POINT('Ctrl Pts',(4.4753302503181,-0.71633578114697,38.5873534781335));
#31249=CARTESIAN_POINT('Ctrl Pts',(4.39100556896819,-1.06425172631817,38.5747385659542));
#31250=CARTESIAN_POINT('Ctrl Pts',(4.21415113822809,-1.79393697912487,38.5482812692697));
#31251=CARTESIAN_POINT('Ctrl Pts',(3.85147938667571,-2.47858553135783,38.5218239725852));
#31252=CARTESIAN_POINT('Ctrl Pts',(3.34716333215496,-3.0348079465722,38.4953666759008));
#31253=CARTESIAN_POINT('Ctrl Pts',(2.84284727763424,-3.59103036178655,38.4689093792163));
#31254=CARTESIAN_POINT('Ctrl Pts',(2.19688692014516,-4.01882663998234,38.4424520825318));
#31255=CARTESIAN_POINT('Ctrl Pts',(1.48795951638629,-4.26609166819816,38.4159947858474));
#31256=CARTESIAN_POINT('Ctrl Pts',(0.779032112627345,-4.513356696414,38.3895374891629));
#31257=CARTESIAN_POINT('Ctrl Pts',(0.00713766259859555,-4.58009047464984,
38.3630801924784));
#31258=CARTESIAN_POINT('Ctrl Pts',(-0.733707943998393,-4.45816490243132,
38.336622895794));
#31259=CARTESIAN_POINT('Ctrl Pts',(-1.4745535505953,-4.33623933021282,38.3101655991095));
#31260=CARTESIAN_POINT('Ctrl Pts',(-2.18435031376045,-4.02565440754,38.283708302425));
#31261=CARTESIAN_POINT('Ctrl Pts',(-2.77664577327751,-3.56423903433536,
38.2572510057406));
#31262=CARTESIAN_POINT('Ctrl Pts',(-3.36894123279463,-3.10282366113066,
38.2307937090561));
#31263=CARTESIAN_POINT('Ctrl Pts',(-3.84373538866364,-2.49057783739411,
38.2043364123716));
#31264=CARTESIAN_POINT('Ctrl Pts',(-4.14319883817823,-1.80207242682554,
38.1778791156872));
#31265=CARTESIAN_POINT('Ctrl Pts',(-4.44266228769283,-1.11356701625697,
38.1514218190027));
#31266=CARTESIAN_POINT('Ctrl Pts',(-4.56679503085301,-0.348802018856373,
38.1249645223182));
#31267=CARTESIAN_POINT('Ctrl Pts',(-4.50047783691868,0.399075035061113,
38.0985072256338));
#31268=CARTESIAN_POINT('Ctrl Pts',(-4.43416064298434,1.14695208897856,38.0720499289493));
#31269=CARTESIAN_POINT('Ctrl Pts',(-4.17739351195555,1.87794119941278,38.0455926322648));
#31270=CARTESIAN_POINT('Ctrl Pts',(-3.76145039622188,2.50300870173274,38.0191353355804));
#31271=CARTESIAN_POINT('Ctrl Pts',(-3.34550728048821,3.1280762040527,37.9926780388959));
#31272=CARTESIAN_POINT('Ctrl Pts',(-2.77038818004956,3.64722209825836,37.9662207422114));
#31273=CARTESIAN_POINT('Ctrl Pts',(-2.10614196483595,3.99721498898437,37.9397634455269));
#31274=CARTESIAN_POINT('Ctrl Pts',(-1.4418957496223,4.34720787971039,37.9133061488425));
#31275=CARTESIAN_POINT('Ctrl Pts',(-0.688522419633467,4.52804776695686,
37.886848852158));
#31276=CARTESIAN_POINT('Ctrl Pts',(0.0622179873187612,4.51770855260138,
37.8603915554735));
#31277=CARTESIAN_POINT('Ctrl Pts',(0.812958394270905,4.5073693382459,37.8339342587891));
#31278=CARTESIAN_POINT('Ctrl Pts',(1.56106587818642,4.30585102228859,37.8074769621046));
#31279=CARTESIAN_POINT('Ctrl Pts',(2.21542177547896,3.93769831258472,37.7810196654202));
#31280=CARTESIAN_POINT('Ctrl Pts',(2.86977767277154,3.56954560288082,37.7545623687357));
#31281=CARTESIAN_POINT('Ctrl Pts',(3.43038198344099,3.03475849943036,37.7281050720512));
#31282=CARTESIAN_POINT('Ctrl Pts',(3.82895372288588,2.3984734795689,37.7016477753667));
#31283=CARTESIAN_POINT('Ctrl Pts',(4.22752546233078,1.76218845970743,37.6751904786822));
#31284=CARTESIAN_POINT('Ctrl Pts',(4.46406463055111,1.02440552343496,37.6487331819978));
#31285=CARTESIAN_POINT('Ctrl Pts',(4.50976101864303,0.274985815861593,37.6222758853133));
#31286=CARTESIAN_POINT('Ctrl Pts',(4.51534128170496,0.18346963073906,37.6190450243729));
#31287=CARTESIAN_POINT('Ctrl Pts',(4.51807563365308,0.0917799142062647,
37.6158141634324));
#31288=CARTESIAN_POINT('Ctrl Pts',(4.51799626797168,8.54686663623316E-5,
37.6125833024919));
#31289=CARTESIAN_POINT('Origin',(0.,0.,20.5));
#31290=CARTESIAN_POINT('',(4.51763788794132,-0.000113968307276224,36.612583302492));
#31291=CARTESIAN_POINT('',(4.51778606435352,0.000115791782295315,36.887416697508));
#31292=CARTESIAN_POINT('',(4.51775,5.53264807684796E-16,20.5));
#31293=CARTESIAN_POINT('Ctrl Pts',(4.51778606435352,0.000115791782295315,
36.887416697508));
#31294=CARTESIAN_POINT('Ctrl Pts',(4.51795287012522,0.16171502012428,36.8931098943111));
#31295=CARTESIAN_POINT('Ctrl Pts',(4.50945045543959,0.323296786803073,36.8988030911142));
#31296=CARTESIAN_POINT('Ctrl Pts',(4.49214571371295,0.483930295567246,36.9044962879172));
#31297=CARTESIAN_POINT('Ctrl Pts',(4.41172750549954,1.23042274011835,36.9309535846017));
#31298=CARTESIAN_POINT('Ctrl Pts',(4.14121195660595,1.9564363604895,36.9574108812862));
#31299=CARTESIAN_POINT('Ctrl Pts',(3.71354756149943,2.57354350122142,36.9838681779707));
#31300=CARTESIAN_POINT('Ctrl Pts',(3.28588316639293,3.1906506419533,37.0103254746552));
#31301=CARTESIAN_POINT('Ctrl Pts',(2.70106992507351,3.69885130304599,37.0367827713396));
#31302=CARTESIAN_POINT('Ctrl Pts',(2.0303374431028,4.03624720641988,37.0632400680241));
#31303=CARTESIAN_POINT('Ctrl Pts',(1.35960496113208,4.37364310979377,37.0896973647085));
#31304=CARTESIAN_POINT('Ctrl Pts',(0.602953238510051,4.54023425544888,37.116154661393));
#31305=CARTESIAN_POINT('Ctrl Pts',(-0.147458382357975,4.51573002621609,
37.1426119580775));
#31306=CARTESIAN_POINT('Ctrl Pts',(-0.897870003226045,4.49122579698331,
37.169069254762));
#31307=CARTESIAN_POINT('Ctrl Pts',(-1.64204152234013,4.27562619286261,37.1955265514464));
#31308=CARTESIAN_POINT('Ctrl Pts',(-2.28933367227002,3.89519100702498,37.2219838481309));
#31309=CARTESIAN_POINT('Ctrl Pts',(-2.93662582219991,3.51475582118734,37.2484411448154));
#31310=CARTESIAN_POINT('Ctrl Pts',(-3.48703860294563,2.96948505363274,37.2748984414998));
#31311=CARTESIAN_POINT('Ctrl Pts',(-3.87353234697123,2.32579208038141,37.3013557381843));
#31312=CARTESIAN_POINT('Ctrl Pts',(-4.26002609099678,1.68209910713015,37.3278130348688));
#31313=CARTESIAN_POINT('Ctrl Pts',(-4.48260079830228,0.939983928182159,
37.3542703315532));
#31314=CARTESIAN_POINT('Ctrl Pts',(-4.51414711586847,0.18983535101083,37.3807276282377));
#31315=CARTESIAN_POINT('Ctrl Pts',(-4.54569343343466,-0.560313226160541,
37.4071849249222));
#31316=CARTESIAN_POINT('Ctrl Pts',(-4.38621136126154,-1.31849520155516,
37.4336422216066));
#31317=CARTESIAN_POINT('Ctrl Pts',(-4.05512563923565,-1.99236484967302,
37.4600995182911));
#31318=CARTESIAN_POINT('Ctrl Pts',(-3.72403991720973,-2.66623449779091,
37.4865568149756));
#31319=CARTESIAN_POINT('Ctrl Pts',(-3.22135054533102,-3.25579181863192,
37.51301411166));
#31320=CARTESIAN_POINT('Ctrl Pts',(-2.60828453275295,-3.68922938300066,
37.5394714083445));
#31321=CARTESIAN_POINT('Ctrl Pts',(-1.99521852017489,-4.1226669473694,37.565928705029));
#31322=CARTESIAN_POINT('Ctrl Pts',(-1.27177586689746,-4.39998475526589,
37.5923860017135));
#31323=CARTESIAN_POINT('Ctrl Pts',(-0.52607108743212,-4.48740580460162,
37.6188432983979));
#31324=CARTESIAN_POINT('Ctrl Pts',(0.219633692033175,-4.57482685393735,
37.6453005950824));
#31325=CARTESIAN_POINT('Ctrl Pts',(0.987600597686399,-4.47235114471234,
37.6717578917668));
#31326=CARTESIAN_POINT('Ctrl Pts',(1.68429211034969,-4.19246010490277,37.6982151884513));
#31327=CARTESIAN_POINT('Ctrl Pts',(2.38098362301298,-3.9125690650932,37.7246724851358));
#31328=CARTESIAN_POINT('Ctrl Pts',(3.00639974268637,-3.45526269469905,37.7511297818202));
#31329=CARTESIAN_POINT('Ctrl Pts',(3.48436547816537,-2.87624040350849,37.7775870785047));
#31330=CARTESIAN_POINT('Ctrl Pts',(3.96233121364435,-2.29721811231796,37.8040443751892));
#31331=CARTESIAN_POINT('Ctrl Pts',(4.29284656492897,-1.596479900331,37.8305016718736));
#31332=CARTESIAN_POINT('Ctrl Pts',(4.43565512801649,-0.859374906258841,
37.8569589685581));
#31333=CARTESIAN_POINT('Ctrl Pts',(4.49045569410255,-0.576522323285484,
37.8671115448747));
#31334=CARTESIAN_POINT('Ctrl Pts',(4.51761603548433,-0.288314654125513,
37.8772641211914));
#31335=CARTESIAN_POINT('Ctrl Pts',(4.51744515673179,-7.51896715610657E-5,
37.887416697508));
#31336=CARTESIAN_POINT('Ctrl Pts',(4.51799626797168,8.54686663623316E-5,
37.6125833024919));
#31337=CARTESIAN_POINT('Ctrl Pts',(4.51742571357972,-0.659099555590392,
37.5893568667479));
#31338=CARTESIAN_POINT('Ctrl Pts',(4.37144018896989,-1.31852897836833,37.5661304310039));
#31339=CARTESIAN_POINT('Ctrl Pts',(4.09200051244546,-1.91548778391919,37.5429039952599));
#31340=CARTESIAN_POINT('Ctrl Pts',(3.77369001019247,-2.59548519725224,37.5164466985755));
#31341=CARTESIAN_POINT('Ctrl Pts',(3.282215397723,-3.19442354504401,37.489989401891));
#31342=CARTESIAN_POINT('Ctrl Pts',(2.67743773890556,-3.63935279939737,37.4635321052065));
#31343=CARTESIAN_POINT('Ctrl Pts',(2.07266008008816,-4.08428205375071,37.4370748085221));
#31344=CARTESIAN_POINT('Ctrl Pts',(1.3545793749228,-4.37520221466565,37.4106175118376));
#31345=CARTESIAN_POINT('Ctrl Pts',(0.610657058576267,-4.47667952851312,
37.3841602151531));
#31346=CARTESIAN_POINT('Ctrl Pts',(-0.133265257770265,-4.57815684236059,
37.3577029184686));
#31347=CARTESIAN_POINT('Ctrl Pts',(-0.903029185297969,-4.49019130914057,
37.3312456217842));
#31348=CARTESIAN_POINT('Ctrl Pts',(-1.60487832955574,-4.22349703344512,
37.3047883250997));
#31349=CARTESIAN_POINT('Ctrl Pts',(-2.30672747381355,-3.95680275774965,
37.2783310284153));
#31350=CARTESIAN_POINT('Ctrl Pts',(-2.94066183480143,-3.51137973957871,
37.2518737317308));
#31351=CARTESIAN_POINT('Ctrl Pts',(-3.42946890894599,-2.94148000958195,
37.2254164350463));
#31352=CARTESIAN_POINT('Ctrl Pts',(-3.91827598309049,-2.37158027958525,
37.1989591383619));
#31353=CARTESIAN_POINT('Ctrl Pts',(-4.26195577039172,-1.67720383776276,
37.1725018416774));
#31354=CARTESIAN_POINT('Ctrl Pts',(-4.41864845311754,-0.942924966240358,
37.1460445449929));
#31355=CARTESIAN_POINT('Ctrl Pts',(-4.57534113584337,-0.208646094717874,
37.1195872483085));
#31356=CARTESIAN_POINT('Ctrl Pts',(-4.54504671399375,0.565535206504528,
37.093129951624));
#31357=CARTESIAN_POINT('Ctrl Pts',(-4.33145501462218,1.28532451174858,37.0666726549395));
#31358=CARTESIAN_POINT('Ctrl Pts',(-4.11786331525061,2.00511381699263,37.040215358255));
#31359=CARTESIAN_POINT('Ctrl Pts',(-3.72097433835709,2.67051112625834,37.0137580615706));
#31360=CARTESIAN_POINT('Ctrl Pts',(-3.18912872207783,3.20047178369309,36.9873007648861));
#31361=CARTESIAN_POINT('Ctrl Pts',(-2.65728310579862,3.73043244112779,36.9608434682017));
#31362=CARTESIAN_POINT('Ctrl Pts',(-1.99048085013371,4.12495644673157,36.9343861715172));
#31363=CARTESIAN_POINT('Ctrl Pts',(-1.26993773185218,4.33599121325395,36.9079288748327));
#31364=CARTESIAN_POINT('Ctrl Pts',(-0.549394613570651,4.54702597977633,
36.8814715781482));
#31365=CARTESIAN_POINT('Ctrl Pts',(0.224889367327489,4.57457150721731,36.8550142814638));
#31366=CARTESIAN_POINT('Ctrl Pts',(0.958607278893124,4.41527278082006,36.8285569847793));
#31367=CARTESIAN_POINT('Ctrl Pts',(1.69232519045884,4.25597405442279,36.8020996880948));
#31368=CARTESIAN_POINT('Ctrl Pts',(2.38547703269204,3.90983107418726,36.7756423914104));
#31369=CARTESIAN_POINT('Ctrl Pts',(2.95363767834151,3.4190036720189,36.7491850947259));
#31370=CARTESIAN_POINT('Ctrl Pts',(3.52179832399097,2.92817626985055,36.7227277980414));
#31371=CARTESIAN_POINT('Ctrl Pts',(3.9649677730567,2.29266444574938,36.6962705013569));
#31372=CARTESIAN_POINT('Ctrl Pts',(4.22916847711195,1.58987283655014,36.6698132046725));
#31373=CARTESIAN_POINT('Ctrl Pts',(4.41966640325359,1.08313556444126,36.6507365706123));
#31374=CARTESIAN_POINT('Ctrl Pts',(4.51712003309545,0.541420116342586,36.6316599365521));
#31375=CARTESIAN_POINT('Ctrl Pts',(4.51763788794132,-0.000113968307276224,
36.612583302492));
#31376=CARTESIAN_POINT('Origin',(0.,0.,20.5));
#31377=CARTESIAN_POINT('',(4.51755220121239,0.000103541448102373,35.6125833024919));
#31378=CARTESIAN_POINT('',(4.51785557016588,-0.00011040733672244,35.887416697508));
#31379=CARTESIAN_POINT('',(4.51775,5.53264807684796E-16,20.5));
#31380=CARTESIAN_POINT('Ctrl Pts',(4.51785557016588,-0.000110407336722441,
35.887416697508));
#31381=CARTESIAN_POINT('Ctrl Pts',(4.51723269271139,0.611237967146432,35.9089556674308));
#31382=CARTESIAN_POINT('Ctrl Pts',(4.39224914626368,1.22283323831731,35.9304946373536));
#31383=CARTESIAN_POINT('Ctrl Pts',(4.1508481772843,1.78438254119822,35.9520336072764));
#31384=CARTESIAN_POINT('Ctrl Pts',(3.85432438440574,2.47415909794758,35.9784909039609));
#31385=CARTESIAN_POINT('Ctrl Pts',(3.38214618261964,3.08842466341222,36.0049482006454));
#31386=CARTESIAN_POINT('Ctrl Pts',(2.79182435432918,3.55236237154543,36.0314054973298));
#31387=CARTESIAN_POINT('Ctrl Pts',(2.20150252603872,4.01630007967864,36.0578627940143));
#31388=CARTESIAN_POINT('Ctrl Pts',(1.4930370712439,4.32990993048042,36.0843200906988));
#31389=CARTESIAN_POINT('Ctrl Pts',(0.752718298257879,4.45499459120493,36.1107773873832));
#31390=CARTESIAN_POINT('Ctrl Pts',(0.0123995252718205,4.58007925192944,
36.1372346840677));
#31391=CARTESIAN_POINT('Ctrl Pts',(-0.759772565905438,4.51663872257667,
36.1636919807522));
#31392=CARTESIAN_POINT('Ctrl Pts',(-1.46974826915546,4.27239998941016,36.1901492774366));
#31393=CARTESIAN_POINT('Ctrl Pts',(-2.17972397240549,4.02816125624364,36.2166065741211));
#31394=CARTESIAN_POINT('Ctrl Pts',(-2.82750328772828,3.60312431926339,36.2430638708056));
#31395=CARTESIAN_POINT('Ctrl Pts',(-3.33418741143512,3.04905820699195,36.26952116749));
#31396=CARTESIAN_POINT('Ctrl Pts',(-3.84087153514189,2.49499209472058,36.2959784641745));
#31397=CARTESIAN_POINT('Ctrl Pts',(-4.20646046723274,1.81189680715804,36.322435760859));
#31398=CARTESIAN_POINT('Ctrl Pts',(-4.3864258803877,1.08297259432656,36.3488930575434));
#31399=CARTESIAN_POINT('Ctrl Pts',(-4.56639129354267,0.354048381494999,
36.3753503542279));
#31400=CARTESIAN_POINT('Ctrl Pts',(-4.56073318776171,-0.420704756605515,
36.4018076509124));
#31401=CARTESIAN_POINT('Ctrl Pts',(-4.37014071406692,-1.14692274519782,
36.4282649475969));
#31402=CARTESIAN_POINT('Ctrl Pts',(-4.17954824037214,-1.87314073379008,
36.4547222442813));
#31403=CARTESIAN_POINT('Ctrl Pts',(-3.80402139876356,-2.55082357287414,
36.4811795409658));
#31404=CARTESIAN_POINT('Ctrl Pts',(-3.28929894294182,-3.09743024266232,
36.5076368376502));
#31405=CARTESIAN_POINT('Ctrl Pts',(-2.77457648712008,-3.64403691245051,
36.5340941343347));
#31406=CARTESIAN_POINT('Ctrl Pts',(-2.12065841708519,-4.05956741294281,
36.5605514310192));
#31407=CARTESIAN_POINT('Ctrl Pts',(-1.40719123005584,-4.29341058905986,
36.5870087277037));
#31408=CARTESIAN_POINT('Ctrl Pts',(-0.693724043026525,-4.52725376517689,
36.6134660243881));
#31409=CARTESIAN_POINT('Ctrl Pts',(0.0792922609972423,-4.57940961691868,
36.6399233210726));
#31410=CARTESIAN_POINT('Ctrl Pts',(0.817705151706661,-4.4435256192656,36.6663806177571));
#31411=CARTESIAN_POINT('Ctrl Pts',(1.55611804241612,-4.30764162161251,36.6928379144415));
#31412=CARTESIAN_POINT('Ctrl Pts',(2.25992751981123,-3.98371777456452,36.719295211126));
#31413=CARTESIAN_POINT('Ctrl Pts',(2.84341036847319,-3.51120764419544,36.7457525078105));
#31414=CARTESIAN_POINT('Ctrl Pts',(3.42689321713519,-3.03869751382634,36.7722098044949));
#31415=CARTESIAN_POINT('Ctrl Pts',(3.89004943706403,-2.41760110013612,36.7986671011794));
#31416=CARTESIAN_POINT('Ctrl Pts',(4.17646711326182,-1.72356725892547,36.8251243978639));
#31417=CARTESIAN_POINT('Ctrl Pts',(4.40125218133937,-1.17887865480133,36.8458884977453));
#31418=CARTESIAN_POINT('Ctrl Pts',(4.51717769407857,-0.589265294821556,
36.8666525976266));
#31419=CARTESIAN_POINT('Ctrl Pts',(4.51778606435352,0.000115791782295315,
36.887416697508));
#31420=CARTESIAN_POINT('Ctrl Pts',(4.51763788794132,-0.000113968307276224,
36.612583302492));
#31421=CARTESIAN_POINT('Ctrl Pts',(4.51783824361694,-0.209631033306269,
36.6052026398677));
#31422=CARTESIAN_POINT('Ctrl Pts',(4.50352846951492,-0.419120950359322,
36.5978219772434));
#31423=CARTESIAN_POINT('Ctrl Pts',(4.47448319596349,-0.626547502778321,
36.5904413146191));
#31424=CARTESIAN_POINT('Ctrl Pts',(4.37036525171502,-1.37010483861031,36.5639840179346));
#31425=CARTESIAN_POINT('Ctrl Pts',(4.07689740417331,-2.08714811597701,36.5375267212501));
#31426=CARTESIAN_POINT('Ctrl Pts',(3.62982371237891,-2.69034225726936,36.5110694245657));
#31427=CARTESIAN_POINT('Ctrl Pts',(3.18275002058453,-3.29353639856167,36.4846121278812));
#31428=CARTESIAN_POINT('Ctrl Pts',(2.58207048453748,-3.78288140377964,36.4581548311967));
#31429=CARTESIAN_POINT('Ctrl Pts',(1.90094720693747,-4.09877559286112,36.4316975345123));
#31430=CARTESIAN_POINT('Ctrl Pts',(1.21982392933739,-4.41466978194264,36.4052402378278));
#31431=CARTESIAN_POINT('Ctrl Pts',(0.458256910184331,-4.55711315488762,
36.3787829411434));
#31432=CARTESIAN_POINT('Ctrl Pts',(-0.290995830438852,-4.50875626651792,
36.3523256444589));
#31433=CARTESIAN_POINT('Ctrl Pts',(-1.04024857106204,-4.46039937814821,
36.3258683477744));
#31434=CARTESIAN_POINT('Ctrl Pts',(-1.77718703315534,-4.2212422284638,36.2994110510899));
#31435=CARTESIAN_POINT('Ctrl Pts',(-2.41205292762861,-3.82041389361357,
36.2729537544055));
#31436=CARTESIAN_POINT('Ctrl Pts',(-3.04691882210185,-3.41958555876337,
36.246496457721));
#31437=CARTESIAN_POINT('Ctrl Pts',(-3.57971214895505,-2.85708603874736,
36.2200391610366));
#31438=CARTESIAN_POINT('Ctrl Pts',(-3.94553927063653,-2.20142715256771,
36.1935818643521));
#31439=CARTESIAN_POINT('Ctrl Pts',(-4.311366392318,-1.54576826638806,36.1671245676676));
#31440=CARTESIAN_POINT('Ctrl Pts',(-4.51022730882774,-0.796950014044777,
36.1406672709831));
#31441=CARTESIAN_POINT('Ctrl Pts',(-4.51790098062044,-0.0461776299327186,
36.1142099742986));
#31442=CARTESIAN_POINT('Ctrl Pts',(-4.52557465241315,0.70459475417934,36.0877526776142));
#31443=CARTESIAN_POINT('Ctrl Pts',(-4.34206107948882,1.45732127006017,36.0612953809297));
#31444=CARTESIAN_POINT('Ctrl Pts',(-3.98971201192945,2.12032066114143,36.0348380842453));
#31445=CARTESIAN_POINT('Ctrl Pts',(-3.63736294437007,2.78332005222269,36.0083807875608));
#31446=CARTESIAN_POINT('Ctrl Pts',(-3.11617838217574,3.3565923185043,35.9819234908763));
#31447=CARTESIAN_POINT('Ctrl Pts',(-2.48963802821032,3.77031353241165,35.9554661941919));
#31448=CARTESIAN_POINT('Ctrl Pts',(-1.86309767424487,4.18403474631902,35.9290088975074));
#31449=CARTESIAN_POINT('Ctrl Pts',(-1.13120152850826,4.43820490785206,35.9025516008229));
#31450=CARTESIAN_POINT('Ctrl Pts',(-0.383093731539153,4.501866372634,35.8760943041385));
#31451=CARTESIAN_POINT('Ctrl Pts',(0.365014065429868,4.56552783741593,35.849637007454));
#31452=CARTESIAN_POINT('Ctrl Pts',(1.12933351363151,4.43868060544686,35.8231797107695));
#31453=CARTESIAN_POINT('Ctrl Pts',(1.81677135017102,4.13677452919484,35.7967224140851));
#31454=CARTESIAN_POINT('Ctrl Pts',(2.50420918671061,3.83486845294278,35.7702651174006));
#31455=CARTESIAN_POINT('Ctrl Pts',(3.11476541158806,3.35790353240771,35.7438078207161));
#31456=CARTESIAN_POINT('Ctrl Pts',(3.57407495233493,2.76397356703885,35.7173505240316));
#31457=CARTESIAN_POINT('Ctrl Pts',(4.03338449308179,2.17004360166999,35.6908932273472));
#31458=CARTESIAN_POINT('Ctrl Pts',(4.34144734969803,1.45914859146745,35.6644359306627));
#31459=CARTESIAN_POINT('Ctrl Pts',(4.46074180719067,0.717874761903989,35.6379786339782));
#31460=CARTESIAN_POINT('Ctrl Pts',(4.49891051264125,0.480701442593838,35.6295135234828));
#31461=CARTESIAN_POINT('Ctrl Pts',(4.51775492478579,0.240418231912197,35.6210484129874));
#31462=CARTESIAN_POINT('Ctrl Pts',(4.51755220121239,0.000103541448102373,
35.6125833024919));
#31463=CARTESIAN_POINT('Origin',(0.,0.,20.5));
#31464=CARTESIAN_POINT('',(4.51806911322653,-6.09724841136444E-5,34.6125833024919));
#31465=CARTESIAN_POINT('',(4.51740954388543,5.82741782004033E-5,34.887416697508));
#31466=CARTESIAN_POINT('',(4.51775,5.53264807684796E-16,20.5));
#31467=CARTESIAN_POINT('Ctrl Pts',(4.51740954388543,5.82741782004033E-5,
34.887416697508));
#31468=CARTESIAN_POINT('Ctrl Pts',(4.51755065915555,0.31030389790581,34.8983441438661));
#31469=CARTESIAN_POINT('Ctrl Pts',(4.48605373157874,0.620521268509011,34.9092715902241));
#31470=CARTESIAN_POINT('Ctrl Pts',(4.42263045256682,0.924067921868281,34.9201990365822));
#31471=CARTESIAN_POINT('Ctrl Pts',(4.26907138171545,1.65900851112936,34.9466563332667));
#31472=CARTESIAN_POINT('Ctrl Pts',(3.92835669717202,2.35484465771423,34.9731136299511));
#31473=CARTESIAN_POINT('Ctrl Pts',(3.44198507043434,2.92682428907246,34.9995709266356));
#31474=CARTESIAN_POINT('Ctrl Pts',(2.95561344369671,3.49880392043062,35.02602822332));
#31475=CARTESIAN_POINT('Ctrl Pts',(2.32358487476487,3.94692703656216,35.0524855200045));
#31476=CARTESIAN_POINT('Ctrl Pts',(1.62287974384894,4.21661273787411,35.078942816689));
#31477=CARTESIAN_POINT('Ctrl Pts',(0.922174612932932,4.48629843918609,35.1054001133734));
#31478=CARTESIAN_POINT('Ctrl Pts',(0.152792920032838,4.57754672567843,35.1318574100579));
#31479=CARTESIAN_POINT('Ctrl Pts',(-0.591555496154874,4.47924365704371,
35.1583147067424));
#31480=CARTESIAN_POINT('Ctrl Pts',(-1.3359039123425,4.380940588409,35.1847720034269));
#31481=CARTESIAN_POINT('Ctrl Pts',(-2.05521905181772,4.09308616464727,35.2112293001113));
#31482=CARTESIAN_POINT('Ctrl Pts',(-2.66188912668102,3.65074073599519,35.2376865967958));
#31483=CARTESIAN_POINT('Ctrl Pts',(-3.26855920154439,3.20839530734307,35.2641438934803));
#31484=CARTESIAN_POINT('Ctrl Pts',(-3.76258421179579,2.61155887380058,35.2906011901647));
#31485=CARTESIAN_POINT('Ctrl Pts',(-4.08379245793952,1.93292545243568,35.3170584868492));
#31486=CARTESIAN_POINT('Ctrl Pts',(-4.40500070408323,1.25429203107082,35.3435157835337));
#31487=CARTESIAN_POINT('Ctrl Pts',(-4.55339218611928,0.493861621883449,
35.3699730802181));
#31488=CARTESIAN_POINT('Ctrl Pts',(-4.51089298576514,-0.255746192879281,
35.3964303769026));
#31489=CARTESIAN_POINT('Ctrl Pts',(-4.468393785411,-1.00535400764205,35.4228876735871));
#31490=CARTESIAN_POINT('Ctrl Pts',(-4.23500390266671,-1.74413922798016,
35.4493449702715));
#31491=CARTESIAN_POINT('Ctrl Pts',(-3.83914996695061,-2.38211863169333,
35.475802266956));
#31492=CARTESIAN_POINT('Ctrl Pts',(-3.44329603123454,-3.02009803540644,
35.5022595636405));
#31493=CARTESIAN_POINT('Ctrl Pts',(-2.88497804254663,-3.55727162249458,
35.5287168603249));
#31494=CARTESIAN_POINT('Ctrl Pts',(-2.23219851400125,-3.92821224455706,
35.5551741570094));
#31495=CARTESIAN_POINT('Ctrl Pts',(-1.57941898545579,-4.29915286661958,
35.5816314536939));
#31496=CARTESIAN_POINT('Ctrl Pts',(-0.83217791705278,-4.50386052365648,
35.6080887503783));
#31497=CARTESIAN_POINT('Ctrl Pts',(-0.081488443928666,-4.51740204959703,
35.6345460470628));
#31498=CARTESIAN_POINT('Ctrl Pts',(0.669201029195319,-4.53094357553758,
35.6610033437473));
#31499=CARTESIAN_POINT('Ctrl Pts',(1.42333890704038,-4.35331897038184,35.6874606404318));
#31500=CARTESIAN_POINT('Ctrl Pts',(2.08907203071298,-4.00616271445508,35.7139179371162));
#31501=CARTESIAN_POINT('Ctrl Pts',(2.75480515438577,-3.65900645852822,35.7403752338007));
#31502=CARTESIAN_POINT('Ctrl Pts',(3.33213352388603,-3.14231855183025,35.7668325304851));
#31503=CARTESIAN_POINT('Ctrl Pts',(3.75073918275594,-2.51903100956234,35.7932898271696));
#31504=CARTESIAN_POINT('Ctrl Pts',(4.16934484162576,-1.89574346729458,35.8197471238541));
#31505=CARTESIAN_POINT('Ctrl Pts',(4.42922778986531,-1.16585628945694,35.8462044205385));
#31506=CARTESIAN_POINT('Ctrl Pts',(4.49873457199958,-0.4182689265211,35.872661717223));
#31507=CARTESIAN_POINT('Ctrl Pts',(4.51165566030144,-0.279294828839705,
35.8775800439847));
#31508=CARTESIAN_POINT('Ctrl Pts',(4.51799780142692,-0.139709054890449,
35.8824983707463));
#31509=CARTESIAN_POINT('Ctrl Pts',(4.51785557016588,-0.000110407336722441,
35.887416697508));
#31510=CARTESIAN_POINT('Ctrl Pts',(4.51755220121239,0.000103541448102373,
35.6125833024919));
#31511=CARTESIAN_POINT('Ctrl Pts',(4.51712132198412,-0.510673802465055,
35.5945911163029));
#31512=CARTESIAN_POINT('Ctrl Pts',(4.43064412559555,-1.02159335775301,35.5765989301139));
#31513=CARTESIAN_POINT('Ctrl Pts',(4.26078183149926,-1.50309674624197,35.5586067439248));
#31514=CARTESIAN_POINT('Ctrl Pts',(4.01100133994626,-2.21114177590013,35.5321494472404));
#31515=CARTESIAN_POINT('Ctrl Pts',(3.58091429847129,-2.85557918629222,35.5056921505559));
#31516=CARTESIAN_POINT('Ctrl Pts',(3.02290483273525,-3.35791721405148,35.4792348538714));
#31517=CARTESIAN_POINT('Ctrl Pts',(2.46489536699924,-3.86025524181071,35.452777557187));
#31518=CARTESIAN_POINT('Ctrl Pts',(1.77896347700217,-4.22049388693713,35.4263202605025));
#31519=CARTESIAN_POINT('Ctrl Pts',(1.04865490780343,-4.39475648114172,35.399862963818));
#31520=CARTESIAN_POINT('Ctrl Pts',(0.318346338604615,-4.56901907534632,
35.3734056671336));
#31521=CARTESIAN_POINT('Ctrl Pts',(-0.456338909795902,-4.55730561862904,
35.3469483704491));
#31522=CARTESIAN_POINT('Ctrl Pts',(-1.18104503151125,-4.36104279705439,
35.3204910737646));
#31523=CARTESIAN_POINT('Ctrl Pts',(-1.9057511532266,-4.16477997547974,35.2940337770802));
#31524=CARTESIAN_POINT('Ctrl Pts',(-2.5804781482568,-3.78396778904771,35.2675764803957));
#31525=CARTESIAN_POINT('Ctrl Pts',(-3.1230450153486,-3.26498874060901,35.2411191837112));
#31526=CARTESIAN_POINT('Ctrl Pts',(-3.66561188244036,-2.74600969217034,
35.2146618870268));
#31527=CARTESIAN_POINT('Ctrl Pts',(-4.07601862159375,-2.08886378172499,
35.1882045903423));
#31528=CARTESIAN_POINT('Ctrl Pts',(-4.30427814618982,-1.37359065388133,
35.1617472936578));
#31529=CARTESIAN_POINT('Ctrl Pts',(-4.53253767078589,-0.658317526037631,
35.1352899969733));
#31530=CARTESIAN_POINT('Ctrl Pts',(-4.57864998082464,0.115082819204295,
35.1088327002889));
#31531=CARTESIAN_POINT('Ctrl Pts',(-4.43699864797729,0.852411075740494,
35.0823754036044));
#31532=CARTESIAN_POINT('Ctrl Pts',(-4.29534731512995,1.58973933227665,35.0559181069199));
#31533=CARTESIAN_POINT('Ctrl Pts',(-3.9659323393965,2.29099550010699,35.0294608102355));
#31534=CARTESIAN_POINT('Ctrl Pts',(-3.48887610024745,2.87076735409185,35.003003513551));
#31535=CARTESIAN_POINT('Ctrl Pts',(-3.0118198610984,3.45053920807671,34.9765462168666));
#31536=CARTESIAN_POINT('Ctrl Pts',(-2.38712235853373,3.90882674821612,34.9500889201821));
#31537=CARTESIAN_POINT('Ctrl Pts',(-1.69087105699361,4.18981105932221,34.9236316234976));
#31538=CARTESIAN_POINT('Ctrl Pts',(-0.994619755453442,4.47079537042831,
34.8971743268131));
#31539=CARTESIAN_POINT('Ctrl Pts',(-0.22681465493779,4.57447645250109,34.8707170301287));
#31540=CARTESIAN_POINT('Ctrl Pts',(0.519026433064394,4.48822606449116,34.8442597334442));
#31541=CARTESIAN_POINT('Ctrl Pts',(1.26486752106653,4.40197567648124,34.8178024367597));
#31542=CARTESIAN_POINT('Ctrl Pts',(1.98874459655524,4.12579381838863,34.7913451400753));
#31543=CARTESIAN_POINT('Ctrl Pts',(2.60249023287332,3.69331913486993,34.7648878433908));
#31544=CARTESIAN_POINT('Ctrl Pts',(3.2162358691914,3.26084445135124,34.7384305467063));
#31545=CARTESIAN_POINT('Ctrl Pts',(3.71985006633887,2.67207694240644,34.7119732500218));
#31546=CARTESIAN_POINT('Ctrl Pts',(4.05199317246873,1.99872783901765,34.6855159533374));
#31547=CARTESIAN_POINT('Ctrl Pts',(4.35719035466755,1.38000583275685,34.6612050697222));
#31548=CARTESIAN_POINT('Ctrl Pts',(4.51760990627478,0.689869322963186,34.6368941861071));
#31549=CARTESIAN_POINT('Ctrl Pts',(4.51806911322653,-6.09724841136444E-5,
34.6125833024919));
#31550=CARTESIAN_POINT('Origin',(0.,0.,20.5));
#31551=CARTESIAN_POINT('',(4.5173649459528,-1.24327273773317E-5,33.6125833024919));
#31552=CARTESIAN_POINT('',(4.51813527504661,9.51052893547258E-6,33.887416697508));
#31553=CARTESIAN_POINT('',(4.51775,5.53264807684796E-16,20.5));
#31554=CARTESIAN_POINT('Ctrl Pts',(4.51813527504661,9.51052893547258E-6,
33.887416697508));
#31555=CARTESIAN_POINT('Ctrl Pts',(4.51813637042829,0.00897485417732503,
33.8877326203013));
#31556=CARTESIAN_POINT('Ctrl Pts',(4.51811024333632,0.0179401914138076,
33.8880485430946));
#31557=CARTESIAN_POINT('Ctrl Pts',(4.51805685504966,0.0269053663078375,
33.8883644658879));
#31558=CARTESIAN_POINT('Ctrl Pts',(4.51358579512714,0.777703653204736,33.9148217625724));
#31559=CARTESIAN_POINT('Ctrl Pts',(4.31792089423795,1.52736336648647,33.9412790592569));
#31560=CARTESIAN_POINT('Ctrl Pts',(3.95489392076193,2.18457678274711,33.9677363559413));
#31561=CARTESIAN_POINT('Ctrl Pts',(3.59186694728593,2.84179019900772,33.9941936526258));
#31562=CARTESIAN_POINT('Ctrl Pts',(3.06147790122311,3.40655731824726,34.0206509493103));
#31563=CARTESIAN_POINT('Ctrl Pts',(2.42832758138582,3.81009013038776,34.0471082459947));
#31564=CARTESIAN_POINT('Ctrl Pts',(1.79517726154854,4.21362294252827,34.0735655426792));
#31565=CARTESIAN_POINT('Ctrl Pts',(1.05926566793676,4.45592144756974,34.1000228393637));
#31566=CARTESIAN_POINT('Ctrl Pts',(0.310226018196078,4.50747395575744,34.1264801360482));
#31567=CARTESIAN_POINT('Ctrl Pts',(-0.438813631544642,4.55902646394514,
34.1529374327326));
#31568=CARTESIAN_POINT('Ctrl Pts',(-1.20098133741429,4.41983297527906,34.1793947294171));
#31569=CARTESIAN_POINT('Ctrl Pts',(-1.8834459163527,4.10684710262894,34.2058520261016));
#31570=CARTESIAN_POINT('Ctrl Pts',(-2.56591049529112,3.79386122997882,34.232309322786));
#31571=CARTESIAN_POINT('Ctrl Pts',(-3.16867194729824,3.30708297334475,34.2587666194705));
#31572=CARTESIAN_POINT('Ctrl Pts',(-3.61831459461467,2.70580138565192,34.2852239161549));
#31573=CARTESIAN_POINT('Ctrl Pts',(-4.06795724193109,2.10451979795912,34.3116812128394));
#31574=CARTESIAN_POINT('Ctrl Pts',(-4.36448108455674,1.38873487920764,34.3381385095239));
#31575=CARTESIAN_POINT('Ctrl Pts',(-4.47176984663203,0.645628440319887,
34.3645958062084));
#31576=CARTESIAN_POINT('Ctrl Pts',(-4.57905860870732,-0.0974779985678242,
34.3910531028928));
#31577=CARTESIAN_POINT('Ctrl Pts',(-4.49711229023226,-0.86790595759181,
34.4175103995773));
#31578=CARTESIAN_POINT('Ctrl Pts',(-4.23591186210457,-1.57181816399963,
34.4439676962618));
#31579=CARTESIAN_POINT('Ctrl Pts',(-3.97471143397686,-2.27573037040753,
34.4704249929462));
#31580=CARTESIAN_POINT('Ctrl Pts',(-3.53425689619645,-2.91312682419928,
34.4968822896307));
#31581=CARTESIAN_POINT('Ctrl Pts',(-2.96819512400025,-3.40637334272956,
34.5233395863152));
#31582=CARTESIAN_POINT('Ctrl Pts',(-2.40213335180411,-3.89961986125978,
34.5497968829996));
#31583=CARTESIAN_POINT('Ctrl Pts',(-1.71046434519219,-4.24871644452859,
34.5762541796841));
#31584=CARTESIAN_POINT('Ctrl Pts',(-0.977432623678127,-4.41114351504993,
34.6027114763686));
#31585=CARTESIAN_POINT('Ctrl Pts',(-0.244400902164024,-4.57357058557128,
34.629168773053));
#31586=CARTESIAN_POINT('Ctrl Pts',(0.529993534252376,-4.54932814334514,
34.6556260697375));
#31587=CARTESIAN_POINT('Ctrl Pts',(1.25143030026179,-4.34136889100478,34.682083366422));
#31588=CARTESIAN_POINT('Ctrl Pts',(1.97286706627129,-4.13340963866439,34.7085406631064));
#31589=CARTESIAN_POINT('Ctrl Pts',(2.64134616187382,-3.74173357620983,34.7349979597909));
#31590=CARTESIAN_POINT('Ctrl Pts',(3.17544757305189,-3.21404641456781,34.7614552564754));
#31591=CARTESIAN_POINT('Ctrl Pts',(3.70954898422987,-2.68635925292589,34.7879125531598));
#31592=CARTESIAN_POINT('Ctrl Pts',(4.10927271098332,-2.0226609920966,34.8143698498443));
#31593=CARTESIAN_POINT('Ctrl Pts',(4.3259328457804,-1.30378934571338,34.8408271465288));
#31594=CARTESIAN_POINT('Ctrl Pts',(4.45310757210366,-0.881827525298336,
34.8563569968552));
#31595=CARTESIAN_POINT('Ctrl Pts',(4.51720899391685,-0.440856093465167,
34.8718868471816));
#31596=CARTESIAN_POINT('Ctrl Pts',(4.51740954388543,5.82741782004033E-5,
34.887416697508));
#31597=CARTESIAN_POINT('Ctrl Pts',(4.51806911322653,-6.09724841136444E-5,
34.6125833024919));
#31598=CARTESIAN_POINT('Ctrl Pts',(4.51810965670567,-0.0609750645635587,
34.6104368894226));
#31599=CARTESIAN_POINT('Ctrl Pts',(4.51690328345783,-0.121887549168861,
34.6082904763533));
#31600=CARTESIAN_POINT('Ctrl Pts',(4.51443954418555,-0.182749134310292,
34.606144063284));
#31601=CARTESIAN_POINT('Ctrl Pts',(4.48407079466025,-0.932946306416683,
34.5796867665996));
#31602=CARTESIAN_POINT('Ctrl Pts',(4.26266128049739,-1.67540995279661,34.5532294699151));
#31603=CARTESIAN_POINT('Ctrl Pts',(3.87717843548116,-2.3197088230287,34.5267721732306));
#31604=CARTESIAN_POINT('Ctrl Pts',(3.49169559046496,-2.96400769326076,34.5003148765461));
#31605=CARTESIAN_POINT('Ctrl Pts',(2.94213941459544,-3.51014178734499,34.4738575798616));
#31606=CARTESIAN_POINT('Ctrl Pts',(2.2954452418825,-3.8915925770456,34.4474002831772));
#31607=CARTESIAN_POINT('Ctrl Pts',(1.64875106916955,-4.2730433667462,34.4209429864927));
#31608=CARTESIAN_POINT('Ctrl Pts',(0.904918899613214,-4.48981085206318,
34.3944856898083));
#31609=CARTESIAN_POINT('Ctrl Pts',(0.154546668243127,-4.51549299318827,
34.3680283931238));
#31610=CARTESIAN_POINT('Ctrl Pts',(-0.595825563126962,-4.54117513431336,
34.3415710964393));
#31611=CARTESIAN_POINT('Ctrl Pts',(-1.35273785631077,-4.37577193124655,
34.3151137997548));
#31612=CARTESIAN_POINT('Ctrl Pts',(-2.02399913169702,-4.03942931106451,
34.2886565030704));
#31613=CARTESIAN_POINT('Ctrl Pts',(-2.69526040708323,-3.70308669088248,
34.2621992063859));
#31614=CARTESIAN_POINT('Ctrl Pts',(-3.28087066467185,-3.19580465358524,
34.2357419097014));
#31615=CARTESIAN_POINT('Ctrl Pts',(-3.7095032232018,-2.57936958989069,34.209284613017));
#31616=CARTESIAN_POINT('Ctrl Pts',(-4.13813578173176,-1.9629345261961,34.1828273163325));
#31617=CARTESIAN_POINT('Ctrl Pts',(-4.40979064120305,-1.23734643610409,
34.1563700196481));
#31618=CARTESIAN_POINT('Ctrl Pts',(-4.49138054038088,-0.490981145957072,
34.1299127229636));
#31619=CARTESIAN_POINT('Ctrl Pts',(-4.57297043955872,0.255384144190028,
34.1034554262791));
#31620=CARTESIAN_POINT('Ctrl Pts',(-4.46449537844313,1.02252663439224,34.0769981295946));
#31621=CARTESIAN_POINT('Ctrl Pts',(-4.17916749942524,1.71700921836348,34.0505408329102));
#31622=CARTESIAN_POINT('Ctrl Pts',(-3.89383962040737,2.41149180233465,34.0240835362257));
#31623=CARTESIAN_POINT('Ctrl Pts',(-3.43165892348727,3.03331448007484,33.9976262395413));
#31624=CARTESIAN_POINT('Ctrl Pts',(-2.84891850603996,3.50673993762589,33.9711689428568));
#31625=CARTESIAN_POINT('Ctrl Pts',(-2.26617808859268,3.98016539517692,33.9447116461723));
#31626=CARTESIAN_POINT('Ctrl Pts',(-1.56287795061823,4.30519363253881,33.9182543494878));
#31627=CARTESIAN_POINT('Ctrl Pts',(-0.824679270557638,4.44223657011982,
33.8917970528033));
#31628=CARTESIAN_POINT('Ctrl Pts',(-0.0864805904969625,4.57927950770084,
33.8653397561189));
#31629=CARTESIAN_POINT('Ctrl Pts',(0.686616631649836,4.52833714550091,33.8388824594344));
#31630=CARTESIAN_POINT('Ctrl Pts',(1.40045000983613,4.2956142068565,33.81242516275));
#31631=CARTESIAN_POINT('Ctrl Pts',(2.11428338802235,4.0628912682121,33.7859678660655));
#31632=CARTESIAN_POINT('Ctrl Pts',(2.76885292224806,3.64838775312326,33.759510569381));
#31633=CARTESIAN_POINT('Ctrl Pts',(3.28443276767714,3.10258973098379,33.7330532726965));
#31634=CARTESIAN_POINT('Ctrl Pts',(3.80001261310627,2.55679170884426,33.7065959760121));
#31635=CARTESIAN_POINT('Ctrl Pts',(4.17660276973874,1.87969917965409,33.6801386793276));
#31636=CARTESIAN_POINT('Ctrl Pts',(4.36833497328078,1.15378126410918,33.6536813826432));
#31637=CARTESIAN_POINT('Ctrl Pts',(4.46761225473945,0.777907227895749,33.6399820225928));
#31638=CARTESIAN_POINT('Ctrl Pts',(4.51732765695876,0.388942719447438,33.6262826625424));
#31639=CARTESIAN_POINT('Ctrl Pts',(4.5173649459528,-1.24327273773317E-5,
33.6125833024919));
#31640=CARTESIAN_POINT('Origin',(0.,0.,20.5));
#31641=CARTESIAN_POINT('',(4.51800690475437,8.25810157162321E-5,32.6125833024919));
#31642=CARTESIAN_POINT('',(4.5174378855045,-7.22228901865168E-5,32.887416697508));
#31643=CARTESIAN_POINT('',(4.51775,5.53264807684796E-16,20.5));
#31644=CARTESIAN_POINT('Ctrl Pts',(4.5174378855045,-7.22228901865168E-5,
32.887416697508));
#31645=CARTESIAN_POINT('Ctrl Pts',(4.51717714450692,0.458772891828189,32.9035783934211));
#31646=CARTESIAN_POINT('Ctrl Pts',(4.44766773093088,0.917695233524441,32.9197400893341));
#31647=CARTESIAN_POINT('Ctrl Pts',(4.31009826091021,1.35521755651858,32.9359017852471));
#31648=CARTESIAN_POINT('Ctrl Pts',(4.08489192720295,2.07145785505129,32.9623590819316));
#31649=CARTESIAN_POINT('Ctrl Pts',(3.67729208498414,2.73034844367792,32.988816378616));
#31650=CARTESIAN_POINT('Ctrl Pts',(3.13694394393257,3.25163717791855,33.0152736753005));
#31651=CARTESIAN_POINT('Ctrl Pts',(2.596595802881,3.77292591215919,33.0417309719849));
#31652=CARTESIAN_POINT('Ctrl Pts',(1.92349936299679,4.15661279201376,33.0681882686694));
#31653=CARTESIAN_POINT('Ctrl Pts',(1.19963702572075,4.35596518015436,33.0946455653539));
#31654=CARTESIAN_POINT('Ctrl Pts',(0.475774688444753,4.55531756829496,33.1211028620384));
#31655=CARTESIAN_POINT('Ctrl Pts',(-0.298853546223071,4.57033546472152,
33.1475601587228));
#31656=CARTESIAN_POINT('Ctrl Pts',(-1.02989881660521,4.39918970627007,33.1740174554073));
#31657=CARTESIAN_POINT('Ctrl Pts',(-1.76094408698744,4.2280439478186,33.2004747520918));
#31658=CARTESIAN_POINT('Ctrl Pts',(-2.4484063930841,3.87073453448909,33.2269320487762));
#31659=CARTESIAN_POINT('Ctrl Pts',(-3.00855358684862,3.37078135737958,33.2533893454607));
#31660=CARTESIAN_POINT('Ctrl Pts',(-3.56870078061313,2.87082818027007,33.2798466421452));
#31661=CARTESIAN_POINT('Ctrl Pts',(-4.0015328620455,2.22823123938057,33.3063039388296));
#31662=CARTESIAN_POINT('Ctrl Pts',(-4.25433136265604,1.52125813092933,33.3327612355141));
#31663=CARTESIAN_POINT('Ctrl Pts',(-4.50712986326656,0.814285022478126,
33.3592185321986));
#31664=CARTESIAN_POINT('Ctrl Pts',(-4.57989478305528,0.0429357464651833,
33.3856758288831));
#31665=CARTESIAN_POINT('Ctrl Pts',(-4.46376343532313,-0.698840208967454,
33.4121331255675));
#31666=CARTESIAN_POINT('Ctrl Pts',(-4.34763208759097,-1.44061616440009,
33.438590422252));
#31667=CARTESIAN_POINT('Ctrl Pts',(-4.04260447233795,-2.15281879925242,
33.4650477189364));
#31668=CARTESIAN_POINT('Ctrl Pts',(-3.5858326155183,-2.74870262081633,33.4915050156209));
#31669=CARTESIAN_POINT('Ctrl Pts',(-3.12906075869862,-3.34458644238028,
33.5179623123054));
#31670=CARTESIAN_POINT('Ctrl Pts',(-2.52054466031228,-3.82415145065579,
33.5444196089899));
#31671=CARTESIAN_POINT('Ctrl Pts',(-1.83440090767899,-4.12898715838447,
33.5708769056743));
#31672=CARTESIAN_POINT('Ctrl Pts',(-1.14825715504573,-4.43382286611314,
33.5973342023588));
#31673=CARTESIAN_POINT('Ctrl Pts',(-0.384485748165517,-4.56392927329501,
33.6237914990433));
#31674=CARTESIAN_POINT('Ctrl Pts',(0.363886800893304,-4.50345956352814,
33.6502487957277));
#31675=CARTESIAN_POINT('Ctrl Pts',(1.11225934995217,-4.44298985376126,33.6767060924122));
#31676=CARTESIAN_POINT('Ctrl Pts',(1.84523304118964,-4.19194402704563,33.7031633890966));
#31677=CARTESIAN_POINT('Ctrl Pts',(2.47353249021786,-3.78089918723496,33.7296206857811));
#31678=CARTESIAN_POINT('Ctrl Pts',(3.10183193924602,-3.36985434742433,33.7560779824656));
#31679=CARTESIAN_POINT('Ctrl Pts',(3.62545714606495,-2.7988104945187,33.7825352791501));
#31680=CARTESIAN_POINT('Ctrl Pts',(3.98063113999648,-2.1373201378099,33.8089925758346));
#31681=CARTESIAN_POINT('Ctrl Pts',(4.3315640520969,-1.48372854278193,33.8351339497257));
#31682=CARTESIAN_POINT('Ctrl Pts',(4.51804463650222,-0.741837565236255,
33.8612753236169));
#31683=CARTESIAN_POINT('Ctrl Pts',(4.51813527504661,9.51052893547258E-6,
33.887416697508));
#31684=CARTESIAN_POINT('Ctrl Pts',(4.5173649459528,-1.24327273773317E-5,
33.6125833024919));
#31685=CARTESIAN_POINT('Ctrl Pts',(4.51739967243793,-0.362238490490815,
33.5998253658579));
#31686=CARTESIAN_POINT('Ctrl Pts',(4.47434946667155,-0.724456433726874,
33.5870674292238));
#31687=CARTESIAN_POINT('Ctrl Pts',(4.38812044853862,-1.07608576485082,33.5743094925897));
#31688=CARTESIAN_POINT('Ctrl Pts',(4.20929946980279,-1.80529157636637,33.5478521959053));
#31689=CARTESIAN_POINT('Ctrl Pts',(3.84478326187951,-2.48895989749788,33.5213948992208));
#31690=CARTESIAN_POINT('Ctrl Pts',(3.33896949547234,-3.04382068336861,33.4949376025364));
#31691=CARTESIAN_POINT('Ctrl Pts',(2.83315572906515,-3.59868146923937,33.4684803058519));
#31692=CARTESIAN_POINT('Ctrl Pts',(2.18604440417407,-4.02473471984934,33.4420230091674));
#31693=CARTESIAN_POINT('Ctrl Pts',(1.47645296399252,-4.27008762080067,33.4155657124829));
#31694=CARTESIAN_POINT('Ctrl Pts',(0.766861523811012,-4.51544052175197,
33.3891084157985));
#31695=CARTESIAN_POINT('Ctrl Pts',(-0.00521003166095199,-4.58009307304465,
33.362651119114));
#31696=CARTESIAN_POINT('Ctrl Pts',(-0.745724241442587,-4.45617066548424,
33.3361938224295));
#31697=CARTESIAN_POINT('Ctrl Pts',(-1.48623845122422,-4.33224825792383,
33.3097365257451));
#31698=CARTESIAN_POINT('Ctrl Pts',(-2.19519531531565,-4.01975089151028,
33.2832792290606));
#31699=CARTESIAN_POINT('Ctrl Pts',(-2.78624467229499,-3.55674039962226,
33.2568219323761));
#31700=CARTESIAN_POINT('Ctrl Pts',(-3.37729402927434,-3.09372990773425,
33.2303646356917));
#31701=CARTESIAN_POINT('Ctrl Pts',(-3.85043587914167,-2.48020629037183,
33.2039073390072));
#31702=CARTESIAN_POINT('Ctrl Pts',(-4.14804206822415,-1.7908960451238,33.1774500423227));
#31703=CARTESIAN_POINT('Ctrl Pts',(-4.44564825730663,-1.10158579987578,
33.1509927456383));
#31704=CARTESIAN_POINT('Ctrl Pts',(-4.56771878560417,-0.33648892674225,
33.1245354489538));
#31705=CARTESIAN_POINT('Ctrl Pts',(-4.49938559786941,0.411206621885727,
33.0980781522693));
#31706=CARTESIAN_POINT('Ctrl Pts',(-4.43105241013465,1.15890217051366,33.0716208555848));
#31707=CARTESIAN_POINT('Ctrl Pts',(-4.17231550636761,1.88919639463604,33.0451635589004));
#31708=CARTESIAN_POINT('Ctrl Pts',(-3.75468875509488,2.51314026599421,33.0187062622159));
#31709=CARTESIAN_POINT('Ctrl Pts',(-3.33706200382211,3.13708413735244,32.9922489655315));
#31710=CARTESIAN_POINT('Ctrl Pts',(-2.76054540504362,3.65467765594643,32.965791668847));
#31711=CARTESIAN_POINT('Ctrl Pts',(-2.09535804244172,4.00287850404833,32.9393343721625));
#31712=CARTESIAN_POINT('Ctrl Pts',(-1.43017067983982,4.35107935215023,32.912877075478));
#31713=CARTESIAN_POINT('Ctrl Pts',(-0.676312553414512,4.52988752976003,
32.8864197787936));
#31714=CARTESIAN_POINT('Ctrl Pts',(0.0743972513539278,4.51752439873747,
32.8599624821091));
#31715=CARTESIAN_POINT('Ctrl Pts',(0.825107056122282,4.50516126771491,32.8335051854247));
#31716=CARTESIAN_POINT('Ctrl Pts',(1.57266853923377,4.30162682806002,32.8070478887402));
#31717=CARTESIAN_POINT('Ctrl Pts',(2.22602953939506,3.93171134926485,32.7805905920557));
#31718=CARTESIAN_POINT('Ctrl Pts',(2.87939053955642,3.56179587046963,32.7541332953712));
#31719=CARTESIAN_POINT('Ctrl Pts',(3.43855105676757,3.02549935253409,32.7276759986868));
#31720=CARTESIAN_POINT('Ctrl Pts',(3.83540595887257,2.38814211780667,32.7012187020023));
#31721=CARTESIAN_POINT('Ctrl Pts',(4.23226086097758,1.75078488307926,32.6747614053179));
#31722=CARTESIAN_POINT('Ctrl Pts',(4.46681014797645,1.01236693155997,32.6483041086334));
#31723=CARTESIAN_POINT('Ctrl Pts',(4.51048597629574,0.262826752513661,32.6218468119489));
#31724=CARTESIAN_POINT('Ctrl Pts',(4.51558339111607,0.175347765528612,32.6187589754633));
#31725=CARTESIAN_POINT('Ctrl Pts',(4.51808086670496,0.0877172796610649,
32.6156711389776));
#31726=CARTESIAN_POINT('Ctrl Pts',(4.51800690475437,8.25810157162321E-5,
32.6125833024919));
#31727=CARTESIAN_POINT('Origin',(0.,0.,20.5));
#31728=CARTESIAN_POINT('',(4.51762600826661,-0.000112987348963034,31.612583302492));
#31729=CARTESIAN_POINT('',(4.51779894817057,0.000115094980599771,31.887416697508));
#31730=CARTESIAN_POINT('',(4.51775,5.53264807684796E-16,20.5));
#31731=CARTESIAN_POINT('Ctrl Pts',(4.51779894817057,0.000115094980599771,
31.887416697508));
#31732=CARTESIAN_POINT('Ctrl Pts',(4.51796156278444,0.157653334629133,31.8929668698563));
#31733=CARTESIAN_POINT('Ctrl Pts',(4.50988180917274,0.315174976505045,31.8985170422046));
#31734=CARTESIAN_POINT('Ctrl Pts',(4.49343403803756,0.471817962781026,31.9040672145528));
#31735=CARTESIAN_POINT('Ctrl Pts',(4.41502862404034,1.21852449753214,31.9305245112373));
#31736=CARTESIAN_POINT('Ctrl Pts',(4.14647135042176,1.94526477434642,31.9569818079218));
#31737=CARTESIAN_POINT('Ctrl Pts',(3.72047219588784,2.56352263181406,31.9834391046062));
#31738=CARTESIAN_POINT('Ctrl Pts',(3.29447304135392,3.1817804892817,32.0098964012907));
#31739=CARTESIAN_POINT('Ctrl Pts',(2.71103200590467,3.69155592740269,32.0363536979752));
#31740=CARTESIAN_POINT('Ctrl Pts',(2.04121156194539,4.0307588619983,32.0628109946597));
#31741=CARTESIAN_POINT('Ctrl Pts',(1.37139111798607,4.36996179659393,32.0892682913441));
#31742=CARTESIAN_POINT('Ctrl Pts',(0.615191265516699,4.53859222766416,32.1157255880286));
#31743=CARTESIAN_POINT('Ctrl Pts',(-0.135283690341923,4.51611115533319,
32.1421828847131));
#31744=CARTESIAN_POINT('Ctrl Pts',(-0.885758646200546,4.49363008300222,
32.1686401813975));
#31745=CARTESIAN_POINT('Ctrl Pts',(-1.63050870544842,4.28003750727005,32.195097478082));
#31746=CARTESIAN_POINT('Ctrl Pts',(-2.27882413510731,3.9013487674713,32.2215547747665));
#31747=CARTESIAN_POINT('Ctrl Pts',(-2.92713956476612,3.52266002767259,32.2480120714509));
#31748=CARTESIAN_POINT('Ctrl Pts',(-3.47902036483595,2.97887512380733,32.2744693681354));
#31749=CARTESIAN_POINT('Ctrl Pts',(-3.86724806465204,2.33622645534256,32.3009266648198));
#31750=CARTESIAN_POINT('Ctrl Pts',(-4.25547576446814,1.69357778687776,32.3273839615043));
#31751=CARTESIAN_POINT('Ctrl Pts',(-4.48005036403047,0.952065353813438,
32.3538412581888));
#31752=CARTESIAN_POINT('Ctrl Pts',(-4.51361892565606,0.202004549841869,
32.3802985548733));
#31753=CARTESIAN_POINT('Ctrl Pts',(-4.54718748728165,-0.548056254129699,
32.4067558515577));
#31754=CARTESIAN_POINT('Ctrl Pts',(-4.38975001097049,-1.30666542900852,
32.4332131482422));
#31755=CARTESIAN_POINT('Ctrl Pts',(-4.06048220709632,-1.98142521687081,
32.4596704449267));
#31756=CARTESIAN_POINT('Ctrl Pts',(-3.73121440322213,-2.65618500473315,
32.4861277416111));
#31757=CARTESIAN_POINT('Ctrl Pts',(-3.23011627178491,-3.24709540557894,
32.5125850382956));
#31758=CARTESIAN_POINT('Ctrl Pts',(-2.61822101061276,-3.68218418656418,
32.5390423349801));
#31759=CARTESIAN_POINT('Ctrl Pts',(-2.00632574944065,-4.11727296754938,
32.5654996316645));
#31760=CARTESIAN_POINT('Ctrl Pts',(-1.28363335853361,-4.39654012867405,
32.591956928349));
#31761=CARTESIAN_POINT('Ctrl Pts',(-0.538166971277905,-4.48597123878686,
32.6184142250335));
#31762=CARTESIAN_POINT('Ctrl Pts',(0.207299415977802,-4.57540234889968,
32.6448715217179));
#31763=CARTESIAN_POINT('Ctrl Pts',(0.975539799582185,-4.47499740800066,
32.6713288184024));
#31764=CARTESIAN_POINT('Ctrl Pts',(1.67298335104786,-4.19698562677001,32.6977861150869));
#31765=CARTESIAN_POINT('Ctrl Pts',(2.37042690251357,-3.91897384553935,32.7242434117713));
#31766=CARTESIAN_POINT('Ctrl Pts',(2.99707362184056,-3.46335522397704,32.7507007084558));
#31767=CARTESIAN_POINT('Ctrl Pts',(3.47659863214429,-2.88562360594202,32.7771580051403));
#31768=CARTESIAN_POINT('Ctrl Pts',(3.95612364244802,-2.30789198790701,32.8036153018248));
#31769=CARTESIAN_POINT('Ctrl Pts',(4.28852694372849,-1.60804737339928,32.8300725985092));
#31770=CARTESIAN_POINT('Ctrl Pts',(4.43332218177084,-0.871330061926005,
32.8565298951937));
#31771=CARTESIAN_POINT('Ctrl Pts',(4.48966784634383,-0.584643655117203,
32.8668254959651));
#31772=CARTESIAN_POINT('Ctrl Pts',(4.51760398720758,-0.292373608988289,
32.8771210967366));
#31773=CARTESIAN_POINT('Ctrl Pts',(4.5174378855045,-7.22228901865168E-5,
32.887416697508));
#31774=CARTESIAN_POINT('Ctrl Pts',(4.51800690475437,8.25810157162321E-5,
32.6125833024919));
#31775=CARTESIAN_POINT('Ctrl Pts',(4.51744714361788,-0.663157072879468,
32.5892138422931));
#31776=CARTESIAN_POINT('Ctrl Pts',(4.36960026846028,-1.32663802677704,32.5658443820943));
#31777=CARTESIAN_POINT('Ctrl Pts',(4.08682159368458,-1.92651262793442,32.5424749218955));
#31778=CARTESIAN_POINT('Ctrl Pts',(3.76667901311444,-2.60564942276291,32.516017625211));
#31779=CARTESIAN_POINT('Ctrl Pts',(3.27359148233441,-3.20326060584664,32.4895603285266));
#31780=CARTESIAN_POINT('Ctrl Pts',(2.66761651687815,-3.64655779648099,32.4631030318421));
#31781=CARTESIAN_POINT('Ctrl Pts',(2.06164155142182,-4.08985498711538,32.4366457351576));
#31782=CARTESIAN_POINT('Ctrl Pts',(1.34277915128922,-4.37883818530036,32.4101884384731));
#31783=CARTESIAN_POINT('Ctrl Pts',(0.598585961229044,-4.47830955732371,
32.3837311417887));
#31784=CARTESIAN_POINT('Ctrl Pts',(-0.14560722883109,-4.57778092934705,
32.3572738451042));
#31785=CARTESIAN_POINT('Ctrl Pts',(-0.915131208818801,-4.4877404752088,
32.3308165484198));
#31786=CARTESIAN_POINT('Ctrl Pts',(-1.6162588096278,-4.2191550225724,32.3043592517353));
#31787=CARTESIAN_POINT('Ctrl Pts',(-2.31738641043684,-3.95056956993598,
32.2779019550508));
#31788=CARTESIAN_POINT('Ctrl Pts',(-2.95011763206717,-3.5034391188014,32.2514446583663));
#31789=CARTESIAN_POINT('Ctrl Pts',(-3.4373865119876,-2.93222366326361,32.2249873616819));
#31790=CARTESIAN_POINT('Ctrl Pts',(-3.924655391908,-2.36100820772586,32.1985300649974));
#31791=CARTESIAN_POINT('Ctrl Pts',(-4.26646193011853,-1.66570774778492,
32.172072768313));
#31792=CARTESIAN_POINT('Ctrl Pts',(-4.42117446855311,-0.931009109950869,
32.1456154716285));
#31793=CARTESIAN_POINT('Ctrl Pts',(-4.57588700698769,-0.196310472116814,
32.119158174944));
#31794=CARTESIAN_POINT('Ctrl Pts',(-4.54350554564632,0.577786343610359,
32.0927008782595));
#31795=CARTESIAN_POINT('Ctrl Pts',(-4.3279741106828,1.2969972017922,32.0662435815751));
#31796=CARTESIAN_POINT('Ctrl Pts',(-4.11244267571929,2.01620805997403,32.0397862848906));
#31797=CARTESIAN_POINT('Ctrl Pts',(-3.71376126713363,2.68053296061054,32.0133289882062));
#31798=CARTESIAN_POINT('Ctrl Pts',(-3.18048883925839,3.2090578660333,31.9868716915217));
#31799=CARTESIAN_POINT('Ctrl Pts',(-2.64721641138316,3.73758277145606,31.9604143948372));
#31800=CARTESIAN_POINT('Ctrl Pts',(-1.97935296421834,4.13030768166508,31.9339570981527));
#31801=CARTESIAN_POINT('Ctrl Pts',(-1.25824352648329,4.33939913723781,31.9074998014683));
#31802=CARTESIAN_POINT('Ctrl Pts',(-0.537134088748201,4.54849059281056,
31.8810425047838));
#31803=CARTESIAN_POINT('Ctrl Pts',(0.237221339557133,4.57394859374701,31.8545852080993));
#31804=CARTESIAN_POINT('Ctrl Pts',(0.970507124268449,4.41267238370826,31.8281279114149));
#31805=CARTESIAN_POINT('Ctrl Pts',(1.70379290897972,4.25139617366952,31.8016706147304));
#31806=CARTESIAN_POINT('Ctrl Pts',(2.39600905009698,3.90338575265561,31.7752133180459));
#31807=CARTESIAN_POINT('Ctrl Pts',(2.96284438772936,3.41102840479202,31.7487560213615));
#31808=CARTESIAN_POINT('Ctrl Pts',(3.52967972536174,2.91867105692843,31.722298724677));
#31809=CARTESIAN_POINT('Ctrl Pts',(3.97113425950925,2.28196678221515,31.6958414279925));
#31810=CARTESIAN_POINT('Ctrl Pts',(4.23343931648423,1.57846545665177,31.669384131308));
#31811=CARTESIAN_POINT('Ctrl Pts',(4.42115243039411,1.07501948430126,31.6504505217027));
#31812=CARTESIAN_POINT('Ctrl Pts',(4.5171186342718,0.537365078236716,31.6315169120973));
#31813=CARTESIAN_POINT('Ctrl Pts',(4.51762600826661,-0.000112987348963034,
31.612583302492));
#31814=CARTESIAN_POINT('Origin',(0.,0.,20.5));
#31815=CARTESIAN_POINT('',(4.5175628644093,0.000105298910395568,30.612583302492));
#31816=CARTESIAN_POINT('',(4.51784283093286,-0.000111697445491984,30.8874166975081));
#31817=CARTESIAN_POINT('',(4.51775,5.53264807684796E-16,20.5));
#31818=CARTESIAN_POINT('Ctrl Pts',(4.51784283093286,-0.000111697445491984,
30.8874166975081));
#31819=CARTESIAN_POINT('Ctrl Pts',(4.51722105684837,0.607182099716009,30.908812642976));
#31820=CARTESIAN_POINT('Ctrl Pts',(4.39393696701912,1.21472067967305,30.930208588444));
#31821=CARTESIAN_POINT('Ctrl Pts',(4.15564368858641,1.77318560159654,30.951604533912));
#31822=CARTESIAN_POINT('Ctrl Pts',(3.86098057239723,2.46375906325124,30.9780618305965));
#31823=CARTESIAN_POINT('Ctrl Pts',(3.3904601122214,3.07929536251675,31.0045191272809));
#31824=CARTESIAN_POINT('Ctrl Pts',(2.80139117936865,3.54482285937575,31.0309764239654));
#31825=CARTESIAN_POINT('Ctrl Pts',(2.21232224651588,4.01035035623478,31.0574337206499));
#31826=CARTESIAN_POINT('Ctrl Pts',(1.50470484098616,4.32586905068731,31.0838910173343));
#31827=CARTESIAN_POINT('Ctrl Pts',(0.764725979630773,4.45294911494339,31.1103483140188));
#31828=CARTESIAN_POINT('Ctrl Pts',(0.0247471182753856,4.58002917919947,
31.1368056107033));
#31829=CARTESIAN_POINT('Ctrl Pts',(-0.747593198905696,4.51867061325911,
31.1632629073878));
#31830=CARTESIAN_POINT('Ctrl Pts',(-1.45822477605293,4.27634682254641,31.1897202040722));
#31831=CARTESIAN_POINT('Ctrl Pts',(-2.16885635320013,4.03402303183372,31.2161775007567));
#31832=CARTESIAN_POINT('Ctrl Pts',(-2.81777919031341,3.61073401634878,31.2426347974411));
#31833=CARTESIAN_POINT('Ctrl Pts',(-3.32595520401574,3.05803590971036,31.2690920941256));
#31834=CARTESIAN_POINT('Ctrl Pts',(-3.83413121771806,2.50533780307193,31.2955493908101));
#31835=CARTESIAN_POINT('Ctrl Pts',(-4.20156040800938,1.82323060527995,31.3220066874946));
#31836=CARTESIAN_POINT('Ctrl Pts',(-4.38349030615745,1.09479421811638,31.348463984179));
#31837=CARTESIAN_POINT('Ctrl Pts',(-4.56542020430551,0.366357830952816,
31.3749212808635));
#31838=CARTESIAN_POINT('Ctrl Pts',(-4.56185081031042,-0.408407745582352,
31.4013785775479));
#31839=CARTESIAN_POINT('Ctrl Pts',(-4.3732168724104,-1.13513692172461,31.4278358742324));
#31840=CARTESIAN_POINT('Ctrl Pts',(-4.18458293451036,-1.86186609786691,
31.4542931709169));
#31841=CARTESIAN_POINT('Ctrl Pts',(-3.81088445270536,-2.54055887361621,
31.4807504676013));
#31842=CARTESIAN_POINT('Ctrl Pts',(-3.29763748849549,-3.08855122001668,
31.5072077642858));
#31843=CARTESIAN_POINT('Ctrl Pts',(-2.78439052428562,-3.63654356641715,
31.5336650609703));
#31844=CARTESIAN_POINT('Ctrl Pts',(-2.13159507767086,-4.05383548346882,
31.5601223576548));
#31845=CARTESIAN_POINT('Ctrl Pts',(-1.4187609115798,-4.28960127750478,31.5865796543392));
#31846=CARTESIAN_POINT('Ctrl Pts',(-0.705926745488817,-4.52536707154071,
31.6130369510237));
#31847=CARTESIAN_POINT('Ctrl Pts',(0.0669461400784679,-4.57960674256098,
31.6394942477081));
#31848=CARTESIAN_POINT('Ctrl Pts',(0.805722683022508,-4.44571395866405,
31.6659515443926));
#31849=CARTESIAN_POINT('Ctrl Pts',(1.54449922596663,-4.31182117476711,31.6924088410771));
#31850=CARTESIAN_POINT('Ctrl Pts',(2.24917942628753,-3.98979593595292,31.7188661377616));
#31851=CARTESIAN_POINT('Ctrl Pts',(2.83393401547767,-3.51886055991368,31.745323434446));
#31852=CARTESIAN_POINT('Ctrl Pts',(3.41868860466777,-3.04792518387447,31.7717807311305));
#31853=CARTESIAN_POINT('Ctrl Pts',(3.88351758272714,-2.42807967061021,31.798238027815));
#31854=CARTESIAN_POINT('Ctrl Pts',(4.1718052945689,-1.73482051763412,31.8246953244994));
#31855=CARTESIAN_POINT('Ctrl Pts',(4.39961643899369,-1.18699223867807,31.8456024488356));
#31856=CARTESIAN_POINT('Ctrl Pts',(4.51718638990429,-0.593320812476893,
31.8665095731718));
#31857=CARTESIAN_POINT('Ctrl Pts',(4.51779894817057,0.000115094980599771,
31.887416697508));
#31858=CARTESIAN_POINT('Ctrl Pts',(4.51762600826661,-0.000112987348963034,
31.612583302492));
#31859=CARTESIAN_POINT('Ctrl Pts',(4.51782762450612,-0.213691742886314,
31.6050596154129));
#31860=CARTESIAN_POINT('Ctrl Pts',(4.50295585827573,-0.42724265346175,31.5975359283338));
#31861=CARTESIAN_POINT('Ctrl Pts',(4.47277779830256,-0.638608182854815,
31.5900122412547));
#31862=CARTESIAN_POINT('Ctrl Pts',(4.36665564334343,-1.38188212038452,31.5635549445702));
#31863=CARTESIAN_POINT('Ctrl Pts',(4.07125575362272,-2.09813161903045,31.5370976478857));
#31864=CARTESIAN_POINT('Ctrl Pts',(3.62255750878013,-2.70011828255321,31.5106403512012));
#31865=CARTESIAN_POINT('Ctrl Pts',(3.17385926393751,-3.302104946076,31.4841830545168));
#31866=CARTESIAN_POINT('Ctrl Pts',(2.57186266397298,-3.78982877447561,31.4577257578323));
#31867=CARTESIAN_POINT('Ctrl Pts',(1.88989022851381,-4.10388554523215,31.4312684611479));
#31868=CARTESIAN_POINT('Ctrl Pts',(1.20791779305463,-4.4179423159887,31.4048111644634));
#31869=CARTESIAN_POINT('Ctrl Pts',(0.44596952210079,-4.55833202910217,31.3783538677789));
#31870=CARTESIAN_POINT('Ctrl Pts',(-0.303150128217454,-4.50795537288904,
31.3518965710945));
#31871=CARTESIAN_POINT('Ctrl Pts',(-1.05226977853561,-4.45757871667591,
31.32543927441));
#31872=CARTESIAN_POINT('Ctrl Pts',(-1.7885608082182,-4.2164356911362,31.2989819777255));
#31873=CARTESIAN_POINT('Ctrl Pts',(-2.42234378472615,-3.81389724990016,
31.272524681041));
#31874=CARTESIAN_POINT('Ctrl Pts',(-3.05612676123416,-3.41135880866406,
31.2460673843566));
#31875=CARTESIAN_POINT('Ctrl Pts',(-3.58740168456753,-2.84742495173157,
31.2196100876721));
#31876=CARTESIAN_POINT('Ctrl Pts',(-3.95145985704278,-2.19078219875388,
31.1931527909876));
#31877=CARTESIAN_POINT('Ctrl Pts',(-4.31551802951802,-1.53413944577618,
31.1666954943032));
#31878=CARTESIAN_POINT('Ctrl Pts',(-4.51235945113515,-0.784787796753247,
31.1402381976187));
#31879=CARTESIAN_POINT('Ctrl Pts',(-4.51800905459174,-0.0339974532052471,
31.1137809009342));
#31880=CARTESIAN_POINT('Ctrl Pts',(-4.52365865804833,0.716792890342667,
31.0873236042498));
#31881=CARTESIAN_POINT('Ctrl Pts',(-4.33811644334446,1.46902192841556,31.0608663075653));
#31882=CARTESIAN_POINT('Ctrl Pts',(-3.98398124688566,2.13106899669175,31.0344090108808));
#31883=CARTESIAN_POINT('Ctrl Pts',(-3.62984605042683,2.79311606496798,31.0079517141964));
#31884=CARTESIAN_POINT('Ctrl Pts',(-3.10711787221305,3.36498116344739,30.9814944175119));
#31885=CARTESIAN_POINT('Ctrl Pts',(-2.47946442583117,3.77701175603613,30.9550371208274));
#31886=CARTESIAN_POINT('Ctrl Pts',(-1.85181097944929,4.18904234862487,30.928579824143));
#31887=CARTESIAN_POINT('Ctrl Pts',(-1.11923226489916,4.44123843532298,30.9021225274585));
#31888=CARTESIAN_POINT('Ctrl Pts',(-0.370955558845505,4.50288281188385,
30.875665230774));
#31889=CARTESIAN_POINT('Ctrl Pts',(0.377321147208236,4.56452718844472,30.8492079340895));
#31890=CARTESIAN_POINT('Ctrl Pts',(1.14129584476551,4.43561985486838,30.8227506374051));
#31891=CARTESIAN_POINT('Ctrl Pts',(1.82791726117872,4.13186158171862,30.7962933407206));
#31892=CARTESIAN_POINT('Ctrl Pts',(2.51453867759182,3.82810330856891,30.7698360440361));
#31893=CARTESIAN_POINT('Ctrl Pts',(3.12380681286076,3.34949409584584,30.7433787473517));
#31894=CARTESIAN_POINT('Ctrl Pts',(3.58151348240585,2.75432801596732,30.7169214506672));
#31895=CARTESIAN_POINT('Ctrl Pts',(4.039220151951,2.15916193608874,30.6904641539828));
#31896=CARTESIAN_POINT('Ctrl Pts',(4.34536535577227,1.44743898905468,30.6640068572983));
#31897=CARTESIAN_POINT('Ctrl Pts',(4.4626609468647,0.705846242127884,30.6375495606138));
#31898=CARTESIAN_POINT('Ctrl Pts',(4.49955602397321,0.47257983095123,30.6292274745732));
#31899=CARTESIAN_POINT('Ctrl Pts',(4.5177662531821,0.236358091141789,30.6209053885326));
#31900=CARTESIAN_POINT('Ctrl Pts',(4.5175628644093,0.000105298910395568,
30.612583302492));
#31901=CARTESIAN_POINT('Origin',(0.,0.,20.5));
#31902=CARTESIAN_POINT('',(4.51806064718817,-6.4525231641549E-5,29.612583302492));
#31903=CARTESIAN_POINT('',(4.51741540695923,6.15435095971417E-5,29.887416697508));
#31904=CARTESIAN_POINT('',(4.51775,5.53264807684796E-16,20.5));
#31905=CARTESIAN_POINT('Ctrl Pts',(4.51741540695923,6.15435095971417E-5,
29.887416697508));
#31906=CARTESIAN_POINT('Ctrl Pts',(4.51756272899121,0.306245363704865,29.8982011194113));
#31907=CARTESIAN_POINT('Ctrl Pts',(4.48689091473443,0.612400072796405,29.9089855413145));
#31908=CARTESIAN_POINT('Ctrl Pts',(4.42510561599225,0.912141398858333,29.9197699632178));
#31909=CARTESIAN_POINT('Ctrl Pts',(4.27352846199847,1.64749330398352,29.9462272599022));
#31910=CARTESIAN_POINT('Ctrl Pts',(3.93469095105298,2.34424546963053,29.9726845565867));
#31911=CARTESIAN_POINT('Ctrl Pts',(3.44986311698689,2.91753425314097,29.9991418532711));
#31912=CARTESIAN_POINT('Ctrl Pts',(2.96503528292081,3.49082303665141,30.0255991499556));
#31913=CARTESIAN_POINT('Ctrl Pts',(2.33421712573414,3.94064843802526,30.0520564466401));
#31914=CARTESIAN_POINT('Ctrl Pts',(1.63424159882604,4.21222222121102,30.0785137433246));
#31915=CARTESIAN_POINT('Ctrl Pts',(0.934266071917943,4.48379600439678,30.104971040009));
#31916=CARTESIAN_POINT('Ctrl Pts',(0.165133175288441,4.57711816939443,30.1314283366935));
#31917=CARTESIAN_POINT('Ctrl Pts',(-0.579477555476409,4.48082217978983,
30.157885633378));
#31918=CARTESIAN_POINT('Ctrl Pts',(-1.32408828624126,4.38452619018523,30.1843429300624));
#31919=CARTESIAN_POINT('Ctrl Pts',(-2.04417685114143,4.09861204597837,30.2108002267469));
#31920=CARTESIAN_POINT('Ctrl Pts',(-2.65203725991661,3.65790377350353,30.2372575234314));
#31921=CARTESIAN_POINT('Ctrl Pts',(-3.2598976686918,3.21719550102869,30.2637148201158));
#31922=CARTESIAN_POINT('Ctrl Pts',(-3.75552992134198,2.62169310028588,30.2901721168003));
#31923=CARTESIAN_POINT('Ctrl Pts',(-4.07856655802606,1.94392810462446,30.3166294134847));
#31924=CARTESIAN_POINT('Ctrl Pts',(-4.40160319471017,1.26616310896299,30.3430867101692));
#31925=CARTESIAN_POINT('Ctrl Pts',(-4.55204421542814,0.506135518382923,
30.3695440068537));
#31926=CARTESIAN_POINT('Ctrl Pts',(-4.51156607035432,-0.243584147729374,
30.3960013035382));
#31927=CARTESIAN_POINT('Ctrl Pts',(-4.47108792528051,-0.993303813841587,
30.4224586002227));
#31928=CARTESIAN_POINT('Ctrl Pts',(-4.2396906144149,-1.73271555548614,30.4489158969071));
#31929=CARTESIAN_POINT('Ctrl Pts',(-3.84555807412635,-2.37175984086058,
30.4753731935916));
#31930=CARTESIAN_POINT('Ctrl Pts',(-3.45142553383776,-3.01080412623509,
30.501830490276));
#31931=CARTESIAN_POINT('Ctrl Pts',(-2.89455776412619,-3.54948095533957,
30.5282877869605));
#31932=CARTESIAN_POINT('Ctrl Pts',(-2.24278064303953,-3.92218008655959,
30.554745083645));
#31933=CARTESIAN_POINT('Ctrl Pts',(-1.59100352195292,-4.29487921777957,
30.5812023803295));
#31934=CARTESIAN_POINT('Ctrl Pts',(-0.844317049491253,-4.5016006511151,
30.6076596770139));
#31935=CARTESIAN_POINT('Ctrl Pts',(-0.0936668116191134,-4.51716594477096,
30.6341169736984));
#31936=CARTESIAN_POINT('Ctrl Pts',(0.656983426253069,-4.53273123842682,
30.6605742703828));
#31937=CARTESIAN_POINT('Ctrl Pts',(1.4115974295357,-4.35714039240299,30.6870315670673));
#31938=CARTESIAN_POINT('Ctrl Pts',(2.07826404778386,-4.01178017741331,30.7134888637518));
#31939=CARTESIAN_POINT('Ctrl Pts',(2.74493066603195,-3.66641996242367,30.7399461604362));
#31940=CARTESIAN_POINT('Ctrl Pts',(3.32364989924556,-3.15129037846822,30.7664034571207));
#31941=CARTESIAN_POINT('Ctrl Pts',(3.74393438530595,-2.52913363876272,30.7928607538052));
#31942=CARTESIAN_POINT('Ctrl Pts',(4.16421887136636,-1.90697689905718,30.8193180504897));
#31943=CARTESIAN_POINT('Ctrl Pts',(4.42606861027353,-1.17779300360159,30.8457753471741));
#31944=CARTESIAN_POINT('Ctrl Pts',(4.49759059362584,-0.430395743851834,
30.8722326438586));
#31945=CARTESIAN_POINT('Ctrl Pts',(4.51127293924728,-0.287416660427361,
30.8772939950751));
#31946=CARTESIAN_POINT('Ctrl Pts',(4.51798991567019,-0.143771027837287,
30.8823553462916));
#31947=CARTESIAN_POINT('Ctrl Pts',(4.51784283093286,-0.000111697445491984,
30.8874166975081));
#31948=CARTESIAN_POINT('Ctrl Pts',(4.5175628644093,0.000105298910395568,
30.612583302492));
#31949=CARTESIAN_POINT('Ctrl Pts',(4.51711964642055,-0.514728858223211,
30.5944480918481));
#31950=CARTESIAN_POINT('Ctrl Pts',(4.42923445822943,-1.02971047605454,30.5763128812042));
#31951=CARTESIAN_POINT('Ctrl Pts',(4.25671408259971,-1.51457811392965,30.5581776705604));
#31952=CARTESIAN_POINT('Ctrl Pts',(4.00502564887872,-2.22194717624094,30.5317203738759));
#31953=CARTESIAN_POINT('Ctrl Pts',(3.57320280307314,-2.86522275404404,30.5052630771915));
#31954=CARTESIAN_POINT('Ctrl Pts',(3.01384108989026,-3.36605459389572,30.478805780507));
#31955=CARTESIAN_POINT('Ctrl Pts',(2.45447937670739,-3.86688643374739,30.4523484838226));
#31956=CARTESIAN_POINT('Ctrl Pts',(1.7675787961471,-4.22527453564767,30.425891187138));
#31957=CARTESIAN_POINT('Ctrl Pts',(1.03680307870754,-4.3975676254243,30.3994338904536));
#31958=CARTESIAN_POINT('Ctrl Pts',(0.306027361267937,-4.56986071520095,
30.3729765937691));
#31959=CARTESIAN_POINT('Ctrl Pts',(-0.468623493050924,-4.55605879285401,
30.3465192970847));
#31960=CARTESIAN_POINT('Ctrl Pts',(-1.19279786752355,-4.35784291725031,
30.3200620004002));
#31961=CARTESIAN_POINT('Ctrl Pts',(-1.91697224199613,-4.15962704164662,
30.2936047037158));
#31962=CARTESIAN_POINT('Ctrl Pts',(-2.59067013662245,-3.77699721278612,
30.2671474070313));
#31963=CARTESIAN_POINT('Ctrl Pts',(-3.1318358934393,-3.25655732035575,30.2406901103468));
#31964=CARTESIAN_POINT('Ctrl Pts',(-3.67300165025612,-2.73611742792542,
30.2142328136623));
#31965=CARTESIAN_POINT('Ctrl Pts',(-4.08163526926355,-2.0778674719253,30.1877755169779));
#31966=CARTESIAN_POINT('Ctrl Pts',(-4.30796562791422,-1.3619815684902,30.1613182202934));
#31967=CARTESIAN_POINT('Ctrl Pts',(-4.5342959865649,-0.64609566505506,30.1348609236089));
#31968=CARTESIAN_POINT('Ctrl Pts',(-4.5783230848587,0.127426185815075,30.1084036269244));
#31969=CARTESIAN_POINT('Ctrl Pts',(-4.4346844709496,0.864369878764792,30.08194633024));
#31970=CARTESIAN_POINT('Ctrl Pts',(-4.29104585704049,1.60131357171455,30.0554890335555));
#31971=CARTESIAN_POINT('Ctrl Pts',(-3.95974153092847,2.30167910674398,30.029031736871));
#31972=CARTESIAN_POINT('Ctrl Pts',(-3.48112399286914,2.88016273680294,30.0025744401866));
#31973=CARTESIAN_POINT('Ctrl Pts',(-3.00250645480984,3.45864636686186,29.9761171435021));
#31974=CARTESIAN_POINT('Ctrl Pts',(-2.37657570480325,3.91524809195029,29.9496598468177));
#31975=CARTESIAN_POINT('Ctrl Pts',(-1.67956941546306,4.19435432728787,29.9232025501332));
#31976=CARTESIAN_POINT('Ctrl Pts',(-0.982563126122875,4.47346056262544,
29.8967452534487));
#31977=CARTESIAN_POINT('Ctrl Pts',(-0.214481297449103,4.57507130821215,
29.8702879567642));
#31978=CARTESIAN_POINT('Ctrl Pts',(0.53112455388596,4.48681048769132,29.8438306600798));
#31979=CARTESIAN_POINT('Ctrl Pts',(1.27673040522102,4.39854966717049,29.8173733633953));
#31980=CARTESIAN_POINT('Ctrl Pts',(1.99986027921735,4.12041728054213,29.7909160667108));
#31981=CARTESIAN_POINT('Ctrl Pts',(2.61243775753263,3.68628954467976,29.7644587700264));
#31982=CARTESIAN_POINT('Ctrl Pts',(3.22501523584791,3.25216180881739,29.7380014733419));
#31983=CARTESIAN_POINT('Ctrl Pts',(3.72704031848211,2.66203872372102,29.7115441766574));
#31984=CARTESIAN_POINT('Ctrl Pts',(4.05736690597726,1.98779662804773,29.685086879973));
#31985=CARTESIAN_POINT('Ctrl Pts',(4.35910923962182,1.37189893439675,29.6609190208126));
#31986=CARTESIAN_POINT('Ctrl Pts',(4.51758267646005,0.685810539097339,29.6367511616523));
#31987=CARTESIAN_POINT('Ctrl Pts',(4.51806064718817,-6.4525231641549E-5,
29.612583302492));
#31988=CARTESIAN_POINT('Origin',(0.,0.,20.5));
#31989=CARTESIAN_POINT('',(4.51736349586412,-8.67285085925565E-6,28.612583302492));
#31990=CARTESIAN_POINT('',(4.51813672578305,5.21363961469835E-6,28.8874166975081));
#31991=CARTESIAN_POINT('',(4.51775,5.53264807684796E-16,20.5));
#31992=CARTESIAN_POINT('Ctrl Pts',(4.51813645424719,5.20997890686523E-6,
28.8874166975081));
#31993=CARTESIAN_POINT('Ctrl Pts',(4.51813678764949,0.00491176269805106,
28.8875895958466));
#31994=CARTESIAN_POINT('Ctrl Pts',(4.51812896220818,0.00981831434884656,
28.887762494185));
#31995=CARTESIAN_POINT('Ctrl Pts',(4.51811297150728,0.0147248393885022,
28.8879353925235));
#31996=CARTESIAN_POINT('Ctrl Pts',(4.51566603811481,0.7655324515643,28.914392689208));
#31997=CARTESIAN_POINT('Ctrl Pts',(4.32202288903541,1.51571694218793,28.9408499858924));
#31998=CARTESIAN_POINT('Ctrl Pts',(3.96076904551605,2.17390667055403,28.9673072825769));
#31999=CARTESIAN_POINT('Ctrl Pts',(3.59951520199672,2.83209639892005,28.9937645792614));
#32000=CARTESIAN_POINT('Ctrl Pts',(3.07065066403746,3.39829136502856,29.0202218759458));
#32001=CARTESIAN_POINT('Ctrl Pts',(2.43859054705081,3.8035296486332,29.0466791726303));
#32002=CARTESIAN_POINT('Ctrl Pts',(1.80653043006408,4.20876793223789,29.0731364693148));
#32003=CARTESIAN_POINT('Ctrl Pts',(1.07127473404993,4.45304953333867,29.0995937659992));
#32004=CARTESIAN_POINT('Ctrl Pts',(0.32237678905244,4.50662122327555,29.1260510626837));
#32005=CARTESIAN_POINT('Ctrl Pts',(-0.426521155945046,4.56019291321243,
29.1525083593682));
#32006=CARTESIAN_POINT('Ctrl Pts',(-1.18906134992587,4.42305469198539,29.1789656560527));
#32007=CARTESIAN_POINT('Ctrl Pts',(-1.87236724119019,4.11190984316476,29.2054229527371));
#32008=CARTESIAN_POINT('Ctrl Pts',(-2.55567313245444,3.80076499434415,29.2318802494216));
#32009=CARTESIAN_POINT('Ctrl Pts',(-3.15974472100221,3.31561351792999,29.258337546106));
#32010=CARTESIAN_POINT('Ctrl Pts',(-3.61100675589329,2.7155463268172,29.2847948427905));
#32011=CARTESIAN_POINT('Ctrl Pts',(-4.06226879078437,2.11547913570442,29.311252139475));
#32012=CARTESIAN_POINT('Ctrl Pts',(-4.36072127201875,1.40049622989302,29.3377094361595));
#32013=CARTESIAN_POINT('Ctrl Pts',(-4.47001301768878,0.657681736016911,
29.3641667328439));
#32014=CARTESIAN_POINT('Ctrl Pts',(-4.57930476335883,-0.0851327578592831,
29.3906240295284));
#32015=CARTESIAN_POINT('Ctrl Pts',(-4.49943577346447,-0.855778839800193,
29.4170813262128));
#32016=CARTESIAN_POINT('Ctrl Pts',(-4.24013400258134,-1.56039266992349,
29.4435386228973));
#32017=CARTESIAN_POINT('Ctrl Pts',(-3.98083223169821,-2.26500650004679,
29.4699959195818));
#32018=CARTESIAN_POINT('Ctrl Pts',(-3.54209767982631,-2.90358807835248,
29.4964532162663));
#32019=CARTESIAN_POINT('Ctrl Pts',(-2.97736772982241,-3.39835887534109,
29.5229105129507));
#32020=CARTESIAN_POINT('Ctrl Pts',(-2.41263777981851,-3.8931296723297,29.5493678096352));
#32021=CARTESIAN_POINT('Ctrl Pts',(-1.72191243168261,-4.24408968800123,
29.5758251063197));
#32022=CARTESIAN_POINT('Ctrl Pts',(-0.989321268370363,-4.40849238086531,
29.6022824030041));
#32023=CARTESIAN_POINT('Ctrl Pts',(-0.256730105058199,-4.57289507372936,
29.6287396996886));
#32024=CARTESIAN_POINT('Ctrl Pts',(0.517726873430306,-4.55074044378599,
29.655196996373));
#32025=CARTESIAN_POINT('Ctrl Pts',(1.23972166423099,-4.34472690044308,29.6816542930575));
#32026=CARTESIAN_POINT('Ctrl Pts',(1.96171645503171,-4.13871335710016,29.708111589742));
#32027=CARTESIAN_POINT('Ctrl Pts',(2.63124905814461,-3.74884090035768,29.7345688864265));
#32028=CARTESIAN_POINT('Ctrl Pts',(3.16677114350317,-3.22259556396285,29.761026183111));
#32029=CARTESIAN_POINT('Ctrl Pts',(3.70229322886173,-2.69635022756802,29.7874834797954));
#32030=CARTESIAN_POINT('Ctrl Pts',(4.10380479646594,-2.03373201152084,29.8139407764799));
#32031=CARTESIAN_POINT('Ctrl Pts',(4.32240218174702,-1.31544708119558,29.8403980731643));
#32032=CARTESIAN_POINT('Ctrl Pts',(4.45189573839702,-0.889946702056473,
29.8560709479456));
#32033=CARTESIAN_POINT('Ctrl Pts',(4.51720130556553,-0.444911837263118,
29.8717438227268));
#32034=CARTESIAN_POINT('Ctrl Pts',(4.51741540695923,6.15435095971417E-5,
29.887416697508));
#32035=CARTESIAN_POINT('Ctrl Pts',(4.51806064718817,-6.4525231641549E-5,
29.612583302492));
#32036=CARTESIAN_POINT('Ctrl Pts',(4.51810592567614,-0.065037930559881,
29.6102938649678));
#32037=CARTESIAN_POINT('Ctrl Pts',(4.51673336863491,-0.130009421477303,
29.6080044274437));
#32038=CARTESIAN_POINT('Ctrl Pts',(4.51393045695516,-0.194919147263631,
29.6057149899196));
#32039=CARTESIAN_POINT('Ctrl Pts',(4.48153932808183,-0.945031720651385,
29.5792576932351));
#32040=CARTESIAN_POINT('Ctrl Pts',(4.25812897797913,-1.68689576117669,29.5528003965506));
#32041=CARTESIAN_POINT('Ctrl Pts',(3.87091054003435,-2.33015304974767,29.5263430998662));
#32042=CARTESIAN_POINT('Ctrl Pts',(3.48369210208957,-2.97341033831866,29.4998858031817));
#32043=CARTESIAN_POINT('Ctrl Pts',(2.9326655763027,-3.51806087493531,29.4734285064972));
#32044=CARTESIAN_POINT('Ctrl Pts',(2.28494538367634,-3.89776682701949,29.4469712098128));
#32045=CARTESIAN_POINT('Ctrl Pts',(1.63722519105001,-4.27747277910364,29.4205139131283));
#32046=CARTESIAN_POINT('Ctrl Pts',(0.892811331584192,-4.49223414665534,
29.3940566164438));
#32047=CARTESIAN_POINT('Ctrl Pts',(0.142372589495739,-4.5158932327899,29.3675993197594));
#32048=CARTESIAN_POINT('Ctrl Pts',(-0.608066152592799,-4.53955231892447,
29.3411420230749));
#32049=CARTESIAN_POINT('Ctrl Pts',(-1.36452977730397,-4.37210912364185,
29.3146847263904));
#32050=CARTESIAN_POINT('Ctrl Pts',(-2.03488185234987,-4.03395804281286,
29.288227429706));
#32051=CARTESIAN_POINT('Ctrl Pts',(-2.70523392739576,-3.69580696198387,
29.2617701330215));
#32052=CARTESIAN_POINT('Ctrl Pts',(-3.28947445277638,-3.18694799560851,
29.235312836337));
#32053=CARTESIAN_POINT('Ctrl Pts',(-3.71644357909758,-2.56935960262119,
29.2088555396525));
#32054=CARTESIAN_POINT('Ctrl Pts',(-4.14341270541876,-1.95177120963391,
29.1823982429681));
#32055=CARTESIAN_POINT('Ctrl Pts',(-4.41311043268056,-1.22545339003468,
29.1559409462836));
#32056=CARTESIAN_POINT('Ctrl Pts',(-4.49268787618537,-0.478870850412086,
29.1294836495992));
#32057=CARTESIAN_POINT('Ctrl Pts',(-4.57226531969018,0.267711689210511,
29.1030263529147));
#32058=CARTESIAN_POINT('Ctrl Pts',(-4.46172247943801,1.03455894885648,29.0765690562302));
#32059=CARTESIAN_POINT('Ctrl Pts',(-4.17452335103036,1.72826978099475,29.0501117595457));
#32060=CARTESIAN_POINT('Ctrl Pts',(-3.88732422262269,2.42198061313306,29.0236544628612));
#32061=CARTESIAN_POINT('Ctrl Pts',(-3.42346880605953,3.04255501776367,28.9971971661768));
#32062=CARTESIAN_POINT('Ctrl Pts',(-2.83945417771499,3.51440771921163,28.9707398694923));
#32063=CARTESIAN_POINT('Ctrl Pts',(-2.25543954937045,3.98626042065959,28.9442825728079));
#32064=CARTESIAN_POINT('Ctrl Pts',(-1.55126570924453,4.3093914189249,28.9178252761234));
#32065=CARTESIAN_POINT('Ctrl Pts',(-0.812700251733401,4.44444371603802,
28.8913679794389));
#32066=CARTESIAN_POINT('Ctrl Pts',(-0.0741347942223568,4.57949601315112,
28.8649106827545));
#32067=CARTESIAN_POINT('Ctrl Pts',(0.698822280673891,4.52646960911207,28.83845338607));
#32068=CARTESIAN_POINT('Ctrl Pts',(1.41202565668872,4.29182306124684,28.8119960893855));
#32069=CARTESIAN_POINT('Ctrl Pts',(2.12522903270359,4.05717651338159,28.785538792701));
#32070=CARTESIAN_POINT('Ctrl Pts',(2.77867870983704,3.64090982169015,28.7590814960166));
#32071=CARTESIAN_POINT('Ctrl Pts',(3.29278524060738,3.09372380852518,28.7326241993321));
#32072=CARTESIAN_POINT('Ctrl Pts',(3.80689177137772,2.54653779536021,28.7061669026477));
#32073=CARTESIAN_POINT('Ctrl Pts',(4.18165515578495,1.86843246072172,28.6797096059632));
#32074=CARTESIAN_POINT('Ctrl Pts',(4.37142962837061,1.14200028388831,28.6532523092787));
#32075=CARTESIAN_POINT('Ctrl Pts',(4.46866731930057,0.769786958618117,28.6396959736831));
#32076=CARTESIAN_POINT('Ctrl Pts',(4.517338221792,0.384885956569512,28.6261396380875));
#32077=CARTESIAN_POINT('Ctrl Pts',(4.51736392670147,-8.66318320566495E-6,
28.612583302492));
#32078=CARTESIAN_POINT('Origin',(0.,0.,20.5));
#32079=CARTESIAN_POINT('',(4.51801726226543,7.95831363512023E-5,27.612583302492));
#32080=CARTESIAN_POINT('',(4.51743092439869,-6.91819792334251E-5,27.8874166975081));
#32081=CARTESIAN_POINT('',(4.51775,5.53264807684796E-16,20.5));
#32082=CARTESIAN_POINT('Ctrl Pts',(4.51743092439869,-6.91819792334251E-5,
27.8874166975081));
#32083=CARTESIAN_POINT('Ctrl Pts',(4.51718386244179,0.454717345983238,27.9034353689663));
#32084=CARTESIAN_POINT('Ctrl Pts',(4.44891863177309,0.909576397762494,27.9194540404245));
#32085=CARTESIAN_POINT('Ctrl Pts',(4.31373618863887,1.34359284719174,27.9354727118827));
#32086=CARTESIAN_POINT('Ctrl Pts',(4.09046161721975,2.06043768656892,27.9619300085671));
#32087=CARTESIAN_POINT('Ctrl Pts',(3.68463958850139,2.72042474717273,27.9883873052516));
#32088=CARTESIAN_POINT('Ctrl Pts',(3.14569877644576,3.24316833544992,28.0148446019361));
#32089=CARTESIAN_POINT('Ctrl Pts',(2.60675796439011,3.76591192372714,28.0413018986205));
#32090=CARTESIAN_POINT('Ctrl Pts',(1.93469836899718,4.15141203967772,28.067759195305));
#32091=CARTESIAN_POINT('Ctrl Pts',(1.21137610519651,4.3527151958239,28.0942164919895));
#32092=CARTESIAN_POINT('Ctrl Pts',(0.48805384139591,4.55401835197006,28.1206737886739));
#32093=CARTESIAN_POINT('Ctrl Pts',(-0.286531090812426,4.57112454831186,
28.1471310853584));
#32094=CARTESIAN_POINT('Ctrl Pts',(-1.01803510394287,4.40195026906682,28.1735883820429));
#32095=CARTESIAN_POINT('Ctrl Pts',(-1.7495391170734,4.23277598982176,28.2000456787273));
#32096=CARTESIAN_POINT('Ctrl Pts',(-2.43796221112602,3.87732123498983,28.2265029754118));
#32097=CARTESIAN_POINT('Ctrl Pts',(-2.99945521514446,3.37888000031668,28.2529602720963));
#32098=CARTESIAN_POINT('Ctrl Pts',(-3.56094821916288,2.88043876564355,28.2794175687807));
#32099=CARTESIAN_POINT('Ctrl Pts',(-3.99551113314713,2.23901105112923,28.3058748654652));
#32100=CARTESIAN_POINT('Ctrl Pts',(-4.25021467511827,1.53272204251347,28.3323321621497));
#32101=CARTESIAN_POINT('Ctrl Pts',(-4.50491821708942,0.826433033897707,
28.3587894588341));
#32102=CARTESIAN_POINT('Ctrl Pts',(-4.57976238704747,0.0552827311804979,
28.3852467555186));
#32103=CARTESIAN_POINT('Ctrl Pts',(-4.4656312479239,-0.686803612223317,
28.4117040522031));
#32104=CARTESIAN_POINT('Ctrl Pts',(-4.35150010880033,-1.42888995562718,
28.4381613488875));
#32105=CARTESIAN_POINT('Ctrl Pts',(-4.04839366059513,-2.14191233971764,
28.464618645572));
#32106=CARTESIAN_POINT('Ctrl Pts',(-3.59322993324233,-2.73902542723662,
28.4910759422565));
#32107=CARTESIAN_POINT('Ctrl Pts',(-3.13806620588952,-3.3361385147556,28.517533238941));
#32108=CARTESIAN_POINT('Ctrl Pts',(-2.5308451993891,-3.8173423057031,28.5439905356254));
#32109=CARTESIAN_POINT('Ctrl Pts',(-1.84552576030239,-4.12402671090497,
28.5704478323099));
#32110=CARTESIAN_POINT('Ctrl Pts',(-1.16020632121576,-4.4307111161068,28.5969051289944));
#32111=CARTESIAN_POINT('Ctrl Pts',(-0.396788449542842,-4.56287613556305,
28.6233624256788));
#32112=CARTESIAN_POINT('Ctrl Pts',(0.351744402845005,-4.50442421617509,
28.6498197223633));
#32113=CARTESIAN_POINT('Ctrl Pts',(1.10027725523294,-4.44597229678712,28.6762770190477));
#32114=CARTESIAN_POINT('Ctrl Pts',(1.8339250883358,-4.19690343855492,28.7027343157322));
#32115=CARTESIAN_POINT('Ctrl Pts',(2.46333040803262,-3.78755395275886,28.7291916124167));
#32116=CARTESIAN_POINT('Ctrl Pts',(3.09273572772936,-3.37820446696285,28.7556489091012));
#32117=CARTESIAN_POINT('Ctrl Pts',(3.61789853402009,-2.80857435360303,28.7821062057856));
#32118=CARTESIAN_POINT('Ctrl Pts',(3.97485457831268,-2.14804393005918,28.8085635024701));
#32119=CARTESIAN_POINT('Ctrl Pts',(4.32947791614233,-1.49183007045257,28.8348479008161));
#32120=CARTESIAN_POINT('Ctrl Pts',(4.51808576967277,-0.745900085055985,
28.8611322991621));
#32121=CARTESIAN_POINT('Ctrl Pts',(4.51813645424719,5.20997890686523E-6,
28.8874166975081));
#32122=CARTESIAN_POINT('Ctrl Pts',(4.51736392670147,-8.66318320566495E-6,
28.612583302492));
#32123=CARTESIAN_POINT('Ctrl Pts',(4.5173883889195,-0.366295738162854,28.5996823414031));
#32124=CARTESIAN_POINT('Ctrl Pts',(4.47335741760473,-0.732577033027994,
28.5867813803142));
#32125=CARTESIAN_POINT('Ctrl Pts',(4.38520343465814,-1.08791198212899,28.5738804192253));
#32126=CARTESIAN_POINT('Ctrl Pts',(4.20441720759592,-1.81663305228457,28.5474231225409));
#32127=CARTESIAN_POINT('Ctrl Pts',(3.8380591927074,-2.49931617356742,28.5209658258564));
#32128=CARTESIAN_POINT('Ctrl Pts',(3.33075139074614,-3.05281129735201,28.4945085291719));
#32129=CARTESIAN_POINT('Ctrl Pts',(2.82344358878484,-3.60630642113663,28.4680512324875));
#32130=CARTESIAN_POINT('Ctrl Pts',(2.17518599975079,-4.03061354742298,28.441593935803));
#32131=CARTESIAN_POINT('Ctrl Pts',(1.46493568054142,-4.27405253782332,28.4151366391185));
#32132=CARTESIAN_POINT('Ctrl Pts',(0.754685361332094,-4.51749152822365,
28.388679342434));
#32133=CARTESIAN_POINT('Ctrl Pts',(-0.0175576880525484,-4.580062382738,
28.3622220457496));
#32134=CARTESIAN_POINT('Ctrl Pts',(-0.757735118862955,-4.45414404053564,
28.3357647490651));
#32135=CARTESIAN_POINT('Ctrl Pts',(-1.49791254967336,-4.32822569833327,
28.3093074523807));
#32136=CARTESIAN_POINT('Ctrl Pts',(-2.20602436190953,-4.01381815941419,
28.2828501556962));
#32137=CARTESIAN_POINT('Ctrl Pts',(-2.79582332053056,-3.54921591405409,
28.2563928590117));
#32138=CARTESIAN_POINT('Ctrl Pts',(-3.38562227915162,-3.08461366869397,
28.2299355623272));
#32139=CARTESIAN_POINT('Ctrl Pts',(-3.85710838415752,-2.46981671689283,
28.2034782656428));
#32140=CARTESIAN_POINT('Ctrl Pts',(-4.15285514976694,-1.77970664696505,
28.1770209689583));
#32141=CARTESIAN_POINT('Ctrl Pts',(-4.44860191537634,-1.08959657703732,
28.1505636722738));
#32142=CARTESIAN_POINT('Ctrl Pts',(-4.56860934158928,-0.32417338898296,
28.1241063755894));
#32143=CARTESIAN_POINT('Ctrl Pts',(-4.49826065670898,0.423335220010742,
28.0976490789049));
#32144=CARTESIAN_POINT('Ctrl Pts',(-4.42791197182868,1.17084382900444,28.0711917822204));
#32145=CARTESIAN_POINT('Ctrl Pts',(-4.16720717585513,1.90043785893749,28.0447344855359));
#32146=CARTESIAN_POINT('Ctrl Pts',(-3.7478998244078,2.52325356442854,28.0182771888515));
#32147=CARTESIAN_POINT('Ctrl Pts',(-3.32859247296047,3.14606926991958,27.991819892167));
#32148=CARTESIAN_POINT('Ctrl Pts',(-2.75068256603934,3.66210665096863,27.9653625954826));
#32149=CARTESIAN_POINT('Ctrl Pts',(-2.08455889071647,4.00851292567859,27.9389052987981));
#32150=CARTESIAN_POINT('Ctrl Pts',(-1.41843521539359,4.35491920038855,27.9124480021136));
#32151=CARTESIAN_POINT('Ctrl Pts',(-0.664097771668966,4.53169436875941,
27.8859907054291));
#32152=CARTESIAN_POINT('Ctrl Pts',(0.0865759746605513,4.51730741092622,
27.8595334087447));
#32153=CARTESIAN_POINT('Ctrl Pts',(0.837249720990026,4.50292045309303,27.8330761120602));
#32154=CARTESIAN_POINT('Ctrl Pts',(1.58425976992439,4.2973713690558,27.8066188153758));
#32155=CARTESIAN_POINT('Ctrl Pts',(2.23662112424281,3.92569580976267,27.7801615186913));
#32156=CARTESIAN_POINT('Ctrl Pts',(2.88898247856131,3.5540202504695,27.7537042220068));
#32157=CARTESIAN_POINT('Ctrl Pts',(3.44669513826383,3.0162182159204,27.7272469253223));
#32158=CARTESIAN_POINT('Ctrl Pts',(3.84183031863663,2.37779339872113,27.7007896286379));
#32159=CARTESIAN_POINT('Ctrl Pts',(4.23696549900942,1.73936858152187,27.6743323319534));
#32160=CARTESIAN_POINT('Ctrl Pts',(4.46952320005248,1.00032098167245,27.647875035269));
#32161=CARTESIAN_POINT('Ctrl Pts',(4.51117815115764,0.250665778907488,27.6214177385845));
#32162=CARTESIAN_POINT('Ctrl Pts',(4.51581452813225,0.167225898922454,27.6184729265537));
#32163=CARTESIAN_POINT('Ctrl Pts',(4.51808587645197,0.0836546049852204,
27.6155281145228));
#32164=CARTESIAN_POINT('Ctrl Pts',(4.51801726226543,7.95831363512023E-5,
27.612583302492));
#32165=CARTESIAN_POINT('Origin',(0.,0.,20.5));
#32166=CARTESIAN_POINT('',(4.51761428595877,-0.000111883206665997,26.612583302492));
#32167=CARTESIAN_POINT('',(4.51781182322151,0.000114263439177032,26.8874166975081));
#32168=CARTESIAN_POINT('',(4.51775,5.53264807684796E-16,20.5));
#32169=CARTESIAN_POINT('Ctrl Pts',(4.51781182322151,0.000114263439177032,
26.8874166975081));
#32170=CARTESIAN_POINT('Ctrl Pts',(4.51797007849026,0.153591581624792,26.8928238454015));
#32171=CARTESIAN_POINT('Ctrl Pts',(4.51030214935632,0.307053160819986,26.898230993295));
#32172=CARTESIAN_POINT('Ctrl Pts',(4.49468970350708,0.459702200761322,26.9036381411884));
#32173=CARTESIAN_POINT('Ctrl Pts',(4.41829765358665,1.20661739855353,26.9300954378729));
#32174=CARTESIAN_POINT('Ctrl Pts',(4.1517006071518,1.93407904976938,26.9565527345573));
#32175=CARTESIAN_POINT('Ctrl Pts',(3.727369789407,2.55348313039531,26.9830100312418));
#32176=CARTESIAN_POINT('Ctrl Pts',(3.30303897166215,3.17288721102131,27.0094673279263));
#32177=CARTESIAN_POINT('Ctrl Pts',(2.72097438260733,3.68423372105737,27.0359246246107));
#32178=CARTESIAN_POINT('Ctrl Pts',(2.05207084500035,4.02524122150424,27.0623819212952));
#32179=CARTESIAN_POINT('Ctrl Pts',(1.38316730739341,4.36624872195109,27.0888392179797));
#32180=CARTESIAN_POINT('Ctrl Pts',(0.627424821234327,4.53691721280878,27.1152965146642));
#32181=CARTESIAN_POINT('Ctrl Pts',(-0.123108015066531,4.51645946077497,
27.1417538113486));
#32182=CARTESIAN_POINT('Ctrl Pts',(-0.873640851367389,4.49600170874117,
27.1682111080331));
#32183=CARTESIAN_POINT('Ctrl Pts',(-1.61896403781002,4.28441771381588,27.1946684047176));
#32184=CARTESIAN_POINT('Ctrl Pts',(-2.26829803515817,3.9074781724144,27.221125701402));
#32185=CARTESIAN_POINT('Ctrl Pts',(-2.91763203250632,3.53053863101291,27.2475829980865));
#32186=CARTESIAN_POINT('Ctrl Pts',(-3.47097684075998,2.98824354313522,27.274040294771));
#32187=CARTESIAN_POINT('Ctrl Pts',(-3.86093567467783,2.34664385030993,27.3004975914554));
#32188=CARTESIAN_POINT('Ctrl Pts',(-4.25089450859569,1.70504415748464,27.3269548881399));
#32189=CARTESIAN_POINT('Ctrl Pts',(-4.47746736817774,0.96413985971173,27.3534121848244));
#32190=CARTESIAN_POINT('Ctrl Pts',(-4.51305792988216,0.214172280478033,
27.3798694815088));
#32191=CARTESIAN_POINT('Ctrl Pts',(-4.54864849158657,-0.535795298755707,
27.4063267781933));
#32192=CARTESIAN_POINT('Ctrl Pts',(-4.39325675541333,-1.29482615945024,
27.4327840748778));
#32193=CARTESIAN_POINT('Ctrl Pts',(-4.06580926285144,-1.97047118281612,
27.4592413715622));
#32194=CARTESIAN_POINT('Ctrl Pts',(-3.73836177028958,-2.64611620618197,
27.4856986682467));
#32195=CARTESIAN_POINT('Ctrl Pts',(-3.23885852133909,-3.23837539221917,
27.5121559649312));
#32196=CARTESIAN_POINT('Ctrl Pts',(-2.62813845890629,-3.67511222754014,
27.5386132616156));
#32197=CARTESIAN_POINT('Ctrl Pts',(-2.0174183964735,-4.11184906286111,27.5650705583001));
#32198=CARTESIAN_POINT('Ctrl Pts',(-1.29548152055841,-4.39306354746584,
27.5915278549846));
#32199=CARTESIAN_POINT('Ctrl Pts',(-0.550258943657392,-4.48450406835833,
27.617985151669));
#32200=CARTESIAN_POINT('Ctrl Pts',(0.194963633243671,-4.57594458925083,
27.6444424483535));
#32201=CARTESIAN_POINT('Ctrl Pts',(0.963471911130666,-4.47761114643107,
27.670899745038));
#32202=CARTESIAN_POINT('Ctrl Pts',(1.66166243228906,-4.20148064440581,27.6973570417224));
#32203=CARTESIAN_POINT('Ctrl Pts',(2.35985295344741,-3.92535014238055,27.7238143384069));
#32204=CARTESIAN_POINT('Ctrl Pts',(2.98772571787716,-3.47142258114982,27.7502716350914));
#32205=CARTESIAN_POINT('Ctrl Pts',(3.46880651775718,-2.89498583529569,27.7767289317758));
#32206=CARTESIAN_POINT('Ctrl Pts',(3.94988731763719,-2.31854908944157,27.8031862284603));
#32207=CARTESIAN_POINT('Ctrl Pts',(4.28417615296746,-1.61960315896406,27.8296435251448));
#32208=CARTESIAN_POINT('Ctrl Pts',(4.43095701357266,-0.883278884650025,
27.8561008218292));
#32209=CARTESIAN_POINT('Ctrl Pts',(4.48886884079068,-0.592764958142916,
27.8665394470555));
#32210=CARTESIAN_POINT('Ctrl Pts',(4.517591923217,-0.296432468768919,27.8769780722818));
#32211=CARTESIAN_POINT('Ctrl Pts',(4.51743092439869,-6.91819792334251E-5,
27.8874166975081));
#32212=CARTESIAN_POINT('Ctrl Pts',(4.51801726226543,7.95831363512023E-5,
27.612583302492));
#32213=CARTESIAN_POINT('Ctrl Pts',(4.5174694208443,-0.667214763012837,27.5890708178383));
#32214=CARTESIAN_POINT('Ctrl Pts',(4.36774838447631,-1.33474676446109,27.5655583331847));
#32215=CARTESIAN_POINT('Ctrl Pts',(4.08161297138008,-1.93752346980862,27.5420458485311));
#32216=CARTESIAN_POINT('Ctrl Pts',(3.7596406393301,-2.61579471007933,27.5155885518466));
#32217=CARTESIAN_POINT('Ctrl Pts',(3.26494377406285,-3.21207438494031,27.4891312551621));
#32218=CARTESIAN_POINT('Ctrl Pts',(2.65777590627143,-3.65373628991481,27.4626739584777));
#32219=CARTESIAN_POINT('Ctrl Pts',(2.05060803847998,-4.09539819488933,27.4362166617932));
#32220=CARTESIAN_POINT('Ctrl Pts',(1.33096916816432,-4.38244232997737,27.4097593651087));
#32221=CARTESIAN_POINT('Ctrl Pts',(0.586510513282131,-4.47990703720589,
27.3833020684243));
#32222=CARTESIAN_POINT('Ctrl Pts',(-0.15794814160006,-4.57737174443442,
27.3568447717398));
#32223=CARTESIAN_POINT('Ctrl Pts',(-0.927226581048814,-4.48525702380344,
27.3303874750553));
#32224=CARTESIAN_POINT('Ctrl Pts',(-1.62762754252371,-4.21478234633956,
27.3039301783709));
#32225=CARTESIAN_POINT('Ctrl Pts',(-2.32802850399852,-3.94430766887572,
27.2774728816864));
#32226=CARTESIAN_POINT('Ctrl Pts',(-2.95955198749952,-3.49547303457901,
27.2510155850019));
#32227=CARTESIAN_POINT('Ctrl Pts',(-3.44527913166303,-2.92294600516749,
27.2245582883174));
#32228=CARTESIAN_POINT('Ctrl Pts',(-3.93100627582659,-2.35041897575591,
27.198100991633));
#32229=CARTESIAN_POINT('Ctrl Pts',(-4.27093708065265,-1.65419955122946,
27.1716436949485));
#32230=CARTESIAN_POINT('Ctrl Pts',(-4.42366835032541,-0.919086486967716,
27.1451863982641));
#32231=CARTESIAN_POINT('Ctrl Pts',(-4.57639961999816,-0.183973422706017,
27.1187291015796));
#32232=CARTESIAN_POINT('Ctrl Pts',(-4.54193135451766,0.590033281290875,
27.0922718048951));
#32233=CARTESIAN_POINT('Ctrl Pts',(-4.32446175047231,1.30866046509374,27.0658145082107));
#32234=CARTESIAN_POINT('Ctrl Pts',(-4.10699214642695,2.02728764889665,27.0393572115262));
#32235=CARTESIAN_POINT('Ctrl Pts',(-3.7065212038167,2.69053531250543,27.0128999148417));
#32236=CARTESIAN_POINT('Ctrl Pts',(-3.17182584023783,3.21762062452939,26.9864426181572));
#32237=CARTESIAN_POINT('Ctrl Pts',(-2.63713047665899,3.74470593655333,26.9599853214728));
#32238=CARTESIAN_POINT('Ctrl Pts',(-1.96821069211152,4.13562889699249,26.9335280247883));
#32239=CARTESIAN_POINT('Ctrl Pts',(-1.2465401760389,4.34277552191203,26.9070707281038));
#32240=CARTESIAN_POINT('Ctrl Pts',(-0.524869659966319,4.54992214683155,
26.8806134314194));
#32241=CARTESIAN_POINT('Ctrl Pts',(0.249551587631431,4.57329243623147,26.8541561347349));
#32242=CARTESIAN_POINT('Ctrl Pts',(0.982399915873105,4.41003991472752,26.8276988380504));
#32243=CARTESIAN_POINT('Ctrl Pts',(1.71524824411482,4.24678739322355,26.801241541366));
#32244=CARTESIAN_POINT('Ctrl Pts',(2.40652365300059,3.89691206081561,26.7747842446815));
#32245=CARTESIAN_POINT('Ctrl Pts',(2.97202956278397,3.40302834577314,26.748326947997));
#32246=CARTESIAN_POINT('Ctrl Pts',(3.53753547256739,2.90914463073064,26.7218696513126));
#32247=CARTESIAN_POINT('Ctrl Pts',(3.97727188324847,2.27125253305366,26.6954123546281));
#32248=CARTESIAN_POINT('Ctrl Pts',(4.23767938667642,1.56704660426395,26.6689550579436));
#32249=CARTESIAN_POINT('Ctrl Pts',(4.42262682954492,1.06690323639616,26.6501644727931));
#32250=CARTESIAN_POINT('Ctrl Pts',(4.5171177314681,0.533310047910147,26.6313738876425));
#32251=CARTESIAN_POINT('Ctrl Pts',(4.51761428595877,-0.000111883206665997,
26.612583302492));
#32252=CARTESIAN_POINT('Origin',(0.,0.,20.5));
#32253=CARTESIAN_POINT('',(4.51757373878986,0.000106944042679857,25.612583302492));
#32254=CARTESIAN_POINT('',(4.51783003468408,-0.000112853895665516,25.8874166975081));
#32255=CARTESIAN_POINT('',(4.51775,5.53264807684796E-16,20.5));
#32256=CARTESIAN_POINT('Ctrl Pts',(4.51783003468408,-0.000112853895665516,
25.8874166975081));
#32257=CARTESIAN_POINT('Ctrl Pts',(4.51721010591009,0.603126320584693,25.9086696185212));
#32258=CARTESIAN_POINT('Ctrl Pts',(4.39561298077165,1.20660788106352,25.9299225395344));
#32259=CARTESIAN_POINT('Ctrl Pts',(4.16040899613699,1.76197577425452,25.9511754605476));
#32260=CARTESIAN_POINT('Ctrl Pts',(3.86760869828648,2.45334112163804,25.977632757232));
#32261=CARTESIAN_POINT('Ctrl Pts',(3.39874939952398,3.0701436809076,26.0040900539165));
#32262=CARTESIAN_POINT('Ctrl Pts',(2.81093764353751,3.53725758297881,26.030547350601));
#32263=CARTESIAN_POINT('Ctrl Pts',(2.22312588755105,4.00437148505003,26.0570046472854));
#32264=CARTESIAN_POINT('Ctrl Pts',(1.51636167434063,4.32179672992291,26.0834619439699));
#32265=CARTESIAN_POINT('Ctrl Pts',(0.776728102877261,4.45087127407636,26.1099192406544));
#32266=CARTESIAN_POINT('Ctrl Pts',(0.0370945314138876,4.57994581822981,
26.1363765373388));
#32267=CARTESIAN_POINT('Ctrl Pts',(-0.735408398302442,4.52066966166383,
26.1628338340233));
#32268=CARTESIAN_POINT('Ctrl Pts',(-1.4466906843854,4.28026257464538,26.1892911307078));
#32269=CARTESIAN_POINT('Ctrl Pts',(-2.15797297046839,4.03985548762692,26.2157484273923));
#32270=CARTESIAN_POINT('Ctrl Pts',(-2.80803461291801,3.61831747015598,26.2422057240767));
#32271=CARTESIAN_POINT('Ctrl Pts',(-3.31769882312739,3.06699138623123,26.2686630207612));
#32272=CARTESIAN_POINT('Ctrl Pts',(-3.82736303333674,2.51566530230651,26.2951203174456));
#32273=CARTESIAN_POINT('Ctrl Pts',(-4.19662981130587,1.834551151928,26.3215776141301));
#32274=CARTESIAN_POINT('Ctrl Pts',(-4.38052287215722,1.1066078848015,26.3480349108146));
#32275=CARTESIAN_POINT('Ctrl Pts',(-4.56441593300857,0.378664617674993,
26.3744922074991));
#32276=CARTESIAN_POINT('Ctrl Pts',(-4.56293527674215,-0.396107766199503,
26.4009495041835));
#32277=CARTESIAN_POINT('Ctrl Pts',(-4.3762612456525,-1.12334284793087,26.427406800868));
#32278=CARTESIAN_POINT('Ctrl Pts',(-4.18958721456285,-1.85057792966224,
26.4538640975524));
#32279=CARTESIAN_POINT('Ctrl Pts',(-3.81771980864998,-2.53027570925048,
26.4803213942369));
#32280=CARTESIAN_POINT('Ctrl Pts',(-3.30595206639681,-3.0796497493845,26.5067786909214));
#32281=CARTESIAN_POINT('Ctrl Pts',(-2.79418432414364,-3.62902378951853,
26.5332359876059));
#32282=CARTESIAN_POINT('Ctrl Pts',(-2.14251624555017,-4.04807409019834,
26.5596932842903));
#32283=CARTESIAN_POINT('Ctrl Pts',(-1.43032028136767,-4.28576078857718,
26.5861505809748));
#32284=CARTESIAN_POINT('Ctrl Pts',(-0.718124317185119,-4.52344748695604,
26.6126078776593));
#32285=CARTESIAN_POINT('Ctrl Pts',(0.0545995325864684,-4.57977058303392,
26.6390651743437));
#32286=CARTESIAN_POINT('Ctrl Pts',(0.793734358242524,-4.44786998604306,
26.6655224710282));
#32287=CARTESIAN_POINT('Ctrl Pts',(1.53286918389854,-4.31596938905221,26.6919797677127));
#32288=CARTESIAN_POINT('Ctrl Pts',(2.23841498543902,-3.99584509899264,26.7184370643971));
#32289=CARTESIAN_POINT('Ctrl Pts',(2.82443706508592,-3.52648790010206,26.7448943610816));
#32290=CARTESIAN_POINT('Ctrl Pts',(3.41045914473281,-3.05713070121148,26.7713516577661));
#32291=CARTESIAN_POINT('Ctrl Pts',(3.87695750248613,-2.43854059348989,26.7978089544505));
#32292=CARTESIAN_POINT('Ctrl Pts',(4.1671131546598,-1.74606116744478,26.824266251135));
#32293=CARTESIAN_POINT('Ctrl Pts',(4.39796892664792,-1.19510559829445,26.845316399926));
#32294=CARTESIAN_POINT('Ctrl Pts',(4.51719573188836,-0.59737640031138,26.8663665487171));
#32295=CARTESIAN_POINT('Ctrl Pts',(4.51781182322151,0.000114263439177032,
26.8874166975081));
#32296=CARTESIAN_POINT('Ctrl Pts',(4.51761428595877,-0.000111883206665997,
26.612583302492));
#32297=CARTESIAN_POINT('Ctrl Pts',(4.51781688422861,-0.217752368533235,
26.604916590958));
#32298=CARTESIAN_POINT('Ctrl Pts',(4.50237218377303,-0.435364344536763,
26.5972498794241));
#32299=CARTESIAN_POINT('Ctrl Pts',(4.47103989191871,-0.65066422144523,26.5895831678902));
#32300=CARTESIAN_POINT('Ctrl Pts',(4.36291429755835,-1.39364935846232,26.5631258712058));
#32301=CARTESIAN_POINT('Ctrl Pts',(4.06558451266292,-2.10909987259421,26.5366685745213));
#32302=CARTESIAN_POINT('Ctrl Pts',(3.61526497596852,-2.70987468303106,26.5102112778368));
#32303=CARTESIAN_POINT('Ctrl Pts',(3.16494543927413,-3.31064949346792,26.4837539811524));
#32304=CARTESIAN_POINT('Ctrl Pts',(2.56163615078078,-3.79674860020972,26.4572966844679));
#32305=CARTESIAN_POINT('Ctrl Pts',(1.87881951412572,-4.10896567003641,26.4308393877834));
#32306=CARTESIAN_POINT('Ctrl Pts',(1.19600287747066,-4.4211827398631,26.4043820910989));
#32307=CARTESIAN_POINT('Ctrl Pts',(0.433678892653904,-4.55951777277466,
26.3779247944145));
#32308=CARTESIAN_POINT('Ctrl Pts',(-0.315302222661645,-4.50712171486216,
26.35146749773));
#32309=CARTESIAN_POINT('Ctrl Pts',(-1.06428333797715,-4.45472565694967,
26.3250102010456));
#32310=CARTESIAN_POINT('Ctrl Pts',(-1.79992158379143,-4.21159850821314,
26.2985529043611));
#32311=CARTESIAN_POINT('Ctrl Pts',(-2.43261703591816,-3.80735288629228,
26.2720956076766));
#32312=CARTESIAN_POINT('Ctrl Pts',(-3.06531248804499,-3.40310726437134,
26.2456383109922));
#32313=CARTESIAN_POINT('Ctrl Pts',(-3.59506514648422,-2.83774316926603,
26.2191810143077));
#32314=CARTESIAN_POINT('Ctrl Pts',(-3.95735172373175,-2.18012132205405,
26.1927237176232));
#32315=CARTESIAN_POINT('Ctrl Pts',(-4.31963830097924,-1.52249947484215,
26.1662664209387));
#32316=CARTESIAN_POINT('Ctrl Pts',(-4.51445879703509,-0.772619875523507,
26.1398091242543));
#32317=CARTESIAN_POINT('Ctrl Pts',(-4.51808429109356,-0.0218170293801812,
26.1133518275698));
#32318=CARTESIAN_POINT('Ctrl Pts',(-4.52170978515203,0.728985816763102,
26.0868945308853));
#32319=CARTESIAN_POINT('Ctrl Pts',(-4.33414027721319,1.48071190973118,26.0604372342009));
#32320=CARTESIAN_POINT('Ctrl Pts',(-3.97822152575495,2.1418018433593,26.0339799375164));
#32321=CARTESIAN_POINT('Ctrl Pts',(-3.62230277429665,2.80289177698754,26.0075226408319));
#32322=CARTESIAN_POINT('Ctrl Pts',(-3.09803477931891,3.37334555127578,25.9810653441475));
#32323=CARTESIAN_POINT('Ctrl Pts',(-2.46927280238623,3.78368252785471,25.954608047463));
#32324=CARTESIAN_POINT('Ctrl Pts',(-1.84051082545367,4.19401950443358,25.9281507507785));
#32325=CARTESIAN_POINT('Ctrl Pts',(-1.10725486656624,4.44423968330318,25.9016934540941));
#32326=CARTESIAN_POINT('Ctrl Pts',(-0.358814689999135,4.50386652360371,
25.8752361574096));
#32327=CARTESIAN_POINT('Ctrl Pts',(0.389625486568016,4.56349336390425,25.8487788607251));
#32328=CARTESIAN_POINT('Ctrl Pts',(1.15324988081482,4.43252686563568,25.8223215640406));
#32329=CARTESIAN_POINT('Ctrl Pts',(1.83904988664902,4.1269186033424,25.7958642673562));
#32330=CARTESIAN_POINT('Ctrl Pts',(2.52484989248321,3.82131034104913,25.7694069706717));
#32331=CARTESIAN_POINT('Ctrl Pts',(3.13282550990476,3.34106031473115,25.7429496739873));
#32332=CARTESIAN_POINT('Ctrl Pts',(3.58892598157735,2.74466244608629,25.7164923773028));
#32333=CARTESIAN_POINT('Ctrl Pts',(4.04502645324994,2.14826457744144,25.6900350806183));
#32334=CARTESIAN_POINT('Ctrl Pts',(4.34925177917356,1.43571886646971,25.6635777839338));
#32335=CARTESIAN_POINT('Ctrl Pts',(4.46454765134638,0.693812592170858,25.6371204872494));
#32336=CARTESIAN_POINT('Ctrl Pts',(4.50019044774909,0.464458203445785,25.6289414256636));
#32337=CARTESIAN_POINT('Ctrl Pts',(4.51777748758952,0.232297861633777,25.6207623640778));
#32338=CARTESIAN_POINT('Ctrl Pts',(4.51757373878986,0.000106944042679857,
25.612583302492));
#32339=CARTESIAN_POINT('Origin',(0.,0.,20.5));
#32340=CARTESIAN_POINT('',(4.51805179992706,-6.79869438786201E-5,24.612583302492));
#32341=CARTESIAN_POINT('',(4.51742159705025,6.47500723078405E-5,24.8874166975081));
#32342=CARTESIAN_POINT('',(4.51775,5.53264807684796E-16,20.5));
#32343=CARTESIAN_POINT('Ctrl Pts',(4.51742159705025,6.47500723078405E-5,
24.8874166975081));
#32344=CARTESIAN_POINT('Ctrl Pts',(4.51757480489056,0.3021867342129,24.8980580949565));
#32345=CARTESIAN_POINT('Ctrl Pts',(4.4877169204789,0.604278844221435,24.9086994924049));
#32346=CARTESIAN_POINT('Ctrl Pts',(4.42754861718235,0.90020824628754,24.9193408898533));
#32347=CARTESIAN_POINT('Ctrl Pts',(4.27795448172836,1.63596612264488,24.9457981865378));
#32348=CARTESIAN_POINT('Ctrl Pts',(3.94099660709531,2.33362924326996,24.9722554832222));
#32349=CARTESIAN_POINT('Ctrl Pts',(3.4577160894917,2.90822301219621,24.9987127799067));
#32350=CARTESIAN_POINT('Ctrl Pts',(2.97443557188809,3.48281678112246,25.0251700765912));
#32351=CARTESIAN_POINT('Ctrl Pts',(2.34483241131392,3.93434119834988,25.0516273732757));
#32352=CARTESIAN_POINT('Ctrl Pts',(1.64559157592564,4.20780108957635,25.0780846699601));
#32353=CARTESIAN_POINT('Ctrl Pts',(0.946350740537367,4.48126098080282,25.1045419666446));
#32354=CARTESIAN_POINT('Ctrl Pts',(0.177472230334982,4.57665634602833,25.1309992633291));
#32355=CARTESIAN_POINT('Ctrl Pts',(-0.567395403080719,4.48236813534545,
25.1574565600135));
#32356=CARTESIAN_POINT('Ctrl Pts',(-1.31226303649646,4.38807992466257,25.183913856698));
#32357=CARTESIAN_POINT('Ctrl Pts',(-2.03311979312552,4.10410813807126,25.2103711533825));
#32358=CARTESIAN_POINT('Ctrl Pts',(-2.64216611780515,3.66504022489793,25.2368284500669));
#32359=CARTESIAN_POINT('Ctrl Pts',(-3.25121244248478,3.22597231172459,25.2632857467514));
#32360=CARTESIAN_POINT('Ctrl Pts',(-3.74844833521498,2.63180827196922,25.2897430434359));
#32361=CARTESIAN_POINT('Ctrl Pts',(-4.07331101456769,1.95491662809413,25.3162003401203));
#32362=CARTESIAN_POINT('Ctrl Pts',(-4.39817369392037,1.27802498421911,25.3426576368048));
#32363=CARTESIAN_POINT('Ctrl Pts',(-4.55066315989561,0.518405736224393,
25.3691149334893));
#32364=CARTESIAN_POINT('Ctrl Pts',(-4.51220636430247,-0.231420332178628,
25.3955722301737));
#32365=CARTESIAN_POINT('Ctrl Pts',(-4.47374956870933,-0.981246400581734,
25.4220295268582));
#32366=CARTESIAN_POINT('Ctrl Pts',(-4.24434651154778,-1.72127928939314,
25.4484868235427));
#32367=CARTESIAN_POINT('Ctrl Pts',(-3.85193823129256,-2.36138381177311,
25.4749441202271));
#32368=CARTESIAN_POINT('Ctrl Pts',(-3.45952995103737,-3.00148833415305,
25.5014014169116));
#32369=CARTESIAN_POINT('Ctrl Pts',(-2.90411644768853,-3.54166449010157,
25.5278587135961));
#32370=CARTESIAN_POINT('Ctrl Pts',(-2.25334647126047,-3.91611942165396,
25.5543160102806));
#32371=CARTESIAN_POINT('Ctrl Pts',(-1.60257649483241,-4.29057435320635,
25.580773306965));
#32372=CARTESIAN_POINT('Ctrl Pts',(-0.856450045325122,-4.49930806036262,
25.6072306036495));
#32373=CARTESIAN_POINT('Ctrl Pts',(-0.105844498527155,-4.51689700860324,
25.6336879003339));
#32374=CARTESIAN_POINT('Ctrl Pts',(0.644761048270813,-4.53448595684386,
25.6601451970184));
#32375=CARTESIAN_POINT('Ctrl Pts',(1.39984569235946,-4.36093014616883,25.6866024937029));
#32376=CARTESIAN_POINT('Ctrl Pts',(2.06744095976455,-4.01736848223874,25.7130597903874));
#32377=CARTESIAN_POINT('Ctrl Pts',(2.73503622716964,-3.67380681830865,25.7395170870718));
#32378=CARTESIAN_POINT('Ctrl Pts',(3.31514211789117,-3.16023930112349,25.7659743837563));
#32379=CARTESIAN_POINT('Ctrl Pts',(3.73710237646057,-2.53921788589521,25.7924316804407));
#32380=CARTESIAN_POINT('Ctrl Pts',(4.15906263502999,-1.9181964706669,25.8188889771252));
#32381=CARTESIAN_POINT('Ctrl Pts',(4.42287726144725,-1.18972115739545,25.8453462738097));
#32382=CARTESIAN_POINT('Ctrl Pts',(4.49641392618663,-0.442519433010954,
25.8718035704942));
#32383=CARTESIAN_POINT('Ctrl Pts',(4.51087921466574,-0.295538487742104,
25.8770079461655));
#32384=CARTESIAN_POINT('Ctrl Pts',(4.51798184168639,-0.147832938193592,
25.8822123218368));
#32385=CARTESIAN_POINT('Ctrl Pts',(4.51783003468408,-0.000112853895665516,
25.8874166975081));
#32386=CARTESIAN_POINT('Ctrl Pts',(4.51757373878986,0.000106944042679857,
25.612583302492));
#32387=CARTESIAN_POINT('Ctrl Pts',(4.51711840923619,-0.518783901194552,
25.5943050673933));
#32388=CARTESIAN_POINT('Ctrl Pts',(4.42781321686835,-1.03782744645157,25.5760268322946));
#32389=CARTESIAN_POINT('Ctrl Pts',(4.25261539535607,-1.52604847346927,25.557748597196));
#32390=CARTESIAN_POINT('Ctrl Pts',(3.99902084877091,-2.2327364271846,25.5312913005115));
#32391=CARTESIAN_POINT('Ctrl Pts',(3.56546533717857,-2.87484549698929,25.504834003827));
#32392=CARTESIAN_POINT('Ctrl Pts',(3.00475544206156,-3.3741675088233,25.4783767071426));
#32393=CARTESIAN_POINT('Ctrl Pts',(2.44404554694452,-3.87348952065733,25.4519194104581));
#32394=CARTESIAN_POINT('Ctrl Pts',(1.7561812683028,-4.23002447452067,25.4254621137736));
#32395=CARTESIAN_POINT('Ctrl Pts',(1.0249437139941,-4.40034680762112,25.3990048170892));
#32396=CARTESIAN_POINT('Ctrl Pts',(0.293706159685441,-4.57066914072155,
25.3725475204047));
#32397=CARTESIAN_POINT('Ctrl Pts',(-0.4809046702902,-4.55477885305912,25.3460902237202));
#32398=CARTESIAN_POINT('Ctrl Pts',(-1.20454203412779,-4.35461136408482,
25.3196329270358));
#32399=CARTESIAN_POINT('Ctrl Pts',(-1.92817939796537,-4.15444387511052,
25.2931756303513));
#32400=CARTESIAN_POINT('Ctrl Pts',(-2.60084329566491,-3.76999918482436,
25.2667183336669));
#32401=CARTESIAN_POINT('Ctrl Pts',(-3.14060400894472,-3.24810223102625,
25.2402610369824));
#32402=CARTESIAN_POINT('Ctrl Pts',(-3.68036472222457,-2.72620527722811,
25.2138037402979));
#32403=CARTESIAN_POINT('Ctrl Pts',(-4.08722225108469,-2.066856059918,25.1873464436134));
#32404=CARTESIAN_POINT('Ctrl Pts',(-4.31162179879184,-1.35036258404192,
25.1608891469289));
#32405=CARTESIAN_POINT('Ctrl Pts',(-4.53602134649897,-0.633869108165933,
25.1344318502445));
#32406=CARTESIAN_POINT('Ctrl Pts',(-4.57796291305318,0.139768626276003,
25.1079745535601));
#32407=CARTESIAN_POINT('Ctrl Pts',(-4.4323380620662,0.876322399437911,25.0815172568756));
#32408=CARTESIAN_POINT('Ctrl Pts',(-4.28671321107921,1.6128761725999,25.0550599601911));
#32409=CARTESIAN_POINT('Ctrl Pts',(-3.95352194255099,2.31234598448186,25.0286026635066));
#32410=CARTESIAN_POINT('Ctrl Pts',(-3.4733465842351,2.88953718612163,25.0021453668221));
#32411=CARTESIAN_POINT('Ctrl Pts',(-2.99317122591925,3.46672838776137,24.9756880701377));
#32412=CARTESIAN_POINT('Ctrl Pts',(-2.36601177781574,3.92164097915893,24.9492307734532));
#32413=CARTESIAN_POINT('Ctrl Pts',(-1.66825556660664,4.19886711014808,24.9227734767688));
#32414=CARTESIAN_POINT('Ctrl Pts',(-0.970499355397546,4.47609324113723,
24.8963161800843));
#32415=CARTESIAN_POINT('Ctrl Pts',(-0.202146381082855,4.57563291171796,
24.8698588833998));
#32416=CARTESIAN_POINT('Ctrl Pts',(0.543218814426126,4.4853623001772,24.8434015867153));
#32417=CARTESIAN_POINT('Ctrl Pts',(1.28858400993515,4.39509168863642,24.8169442900309));
#32418=CARTESIAN_POINT('Ctrl Pts',(2.01096142663846,4.11501079497414,24.7904869933464));
#32419=CARTESIAN_POINT('Ctrl Pts',(2.62236629465924,3.67923316206414,24.7640296966619));
#32420=CARTESIAN_POINT('Ctrl Pts',(3.23377116267999,3.24345552915417,24.7375723999775));
#32421=CARTESIAN_POINT('Ctrl Pts',(3.73420348201823,2.65198115699651,24.711115103293));
#32422=CARTESIAN_POINT('Ctrl Pts',(4.06271115002261,1.97685096951678,24.6846578066085));
#32423=CARTESIAN_POINT('Ctrl Pts',(4.36101609468216,1.3637916931913,24.660632971903));
#32424=CARTESIAN_POINT('Ctrl Pts',(4.51755636187948,0.681751967669245,24.6366081371975));
#32425=CARTESIAN_POINT('Ctrl Pts',(4.51805179992706,-6.79869438786201E-5,
24.612583302492));
#32426=CARTESIAN_POINT('Origin',(0.,0.,20.5));
#32427=CARTESIAN_POINT('',(4.5173631353831,-4.88662610135722E-6,23.612583302492));
#32428=CARTESIAN_POINT('',(4.51813699104787,9.0065690785813E-7,23.8874166975081));
#32429=CARTESIAN_POINT('',(4.51775,5.53264807684796E-16,20.5));
#32430=CARTESIAN_POINT('Ctrl Pts',(4.51813695063288,9.0056284873609E-7,
23.8874166975081));
#32431=CARTESIAN_POINT('Ctrl Pts',(4.51814591729222,0.751660275924123,23.9139038680762));
#32432=CARTESIAN_POINT('Ctrl Pts',(4.32649937043261,1.5033152188212,23.9403910386443));
#32433=CARTESIAN_POINT('Ctrl Pts',(3.96661538289285,2.16322075812818,23.9668782092125));
#32434=CARTESIAN_POINT('Ctrl Pts',(3.6071372949696,2.8223820147924,23.9933355058969));
#32435=CARTESIAN_POINT('Ctrl Pts',(3.07980110896882,3.39000071259223,24.0197928025814));
#32436=CARTESIAN_POINT('Ctrl Pts',(2.44883578872663,3.7969415223372,24.0462500992659));
#32437=CARTESIAN_POINT('Ctrl Pts',(1.81787046848448,4.20388233208215,24.0727073959503));
#32438=CARTESIAN_POINT('Ctrl Pts',(1.08327601400093,4.45014525377226,24.0991646926348));
#32439=CARTESIAN_POINT('Ctrl Pts',(0.334525216833109,4.50573573609242,24.1256219893193));
#32440=CARTESIAN_POINT('Ctrl Pts',(-0.414225580334709,4.56132621841258,
24.1520792860037));
#32441=CARTESIAN_POINT('Ctrl Pts',(-1.17713272018679,4.4262442613628,24.1785365826882));
#32442=CARTESIAN_POINT('Ctrl Pts',(-1.86127495742213,4.11694269781237,24.2049938793727));
#32443=CARTESIAN_POINT('Ctrl Pts',(-2.54541719465748,3.80764113426195,24.2314511760572));
#32444=CARTESIAN_POINT('Ctrl Pts',(-3.15079452927609,3.32411996421088,24.2579084727416));
#32445=CARTESIAN_POINT('Ctrl Pts',(-3.6036726719115,2.72527153104338,24.2843657694261));
#32446=CARTESIAN_POINT('Ctrl Pts',(-4.05655081454692,2.12642309787588,24.3108230661106));
#32447=CARTESIAN_POINT('Ctrl Pts',(-4.35692976519914,1.41224740159195,24.337280362795));
#32448=CARTESIAN_POINT('Ctrl Pts',(-4.46822370011745,0.669730251598438,
24.3637376594795));
#32449=CARTESIAN_POINT('Ctrl Pts',(-4.57951763503577,-0.0727868983951169,
24.390194956164));
#32450=CARTESIAN_POINT('Ctrl Pts',(-4.50172655422016,-0.843645502098255,
24.4166522528484));
#32451=CARTESIAN_POINT('Ctrl Pts',(-4.24432532522016,-1.54895583471323,
24.4431095495329));
#32452=CARTESIAN_POINT('Ctrl Pts',(-3.98692409622017,-2.25426616732816,
24.4695668462174));
#32453=CARTESIAN_POINT('Ctrl Pts',(-3.54991271903582,-2.89402822885493,
24.4960241429018));
#32454=CARTESIAN_POINT('Ctrl Pts',(-2.98651869575401,-3.39031970824422,
24.5224814395863));
#32455=CARTESIAN_POINT('Ctrl Pts',(-2.42312467247219,-3.88661118763352,
24.5489387362708));
#32456=CARTESIAN_POINT('Ctrl Pts',(-1.73334800309291,-4.23943208488534,
24.5753960329552));
#32457=CARTESIAN_POINT('Ctrl Pts',(-1.00120272254919,-4.40580920519233,
24.6018533296397));
#32458=CARTESIAN_POINT('Ctrl Pts',(-0.269057442005433,-4.57218632549932,
24.6283106263242));
#32459=CARTESIAN_POINT('Ctrl Pts',(0.505456449702776,-4.55211966886146,
24.6547679230086));
#32460=CARTESIAN_POINT('Ctrl Pts',(1.22800401774408,-4.34805333184884,24.6812252196931));
#32461=CARTESIAN_POINT('Ctrl Pts',(1.95055158578534,-4.14398699483623,24.7076825163776));
#32462=CARTESIAN_POINT('Ctrl Pts',(2.6211328301597,-3.75592097744887,24.7341398130621));
#32463=CARTESIAN_POINT('Ctrl Pts',(3.15807169745557,-3.23112129111977,24.7605971097465));
#32464=CARTESIAN_POINT('Ctrl Pts',(3.69501056475143,-2.70632160479067,24.787054406431));
#32465=CARTESIAN_POINT('Ctrl Pts',(4.0983070549688,-2.04478824951983,24.8135117031154));
#32466=CARTESIAN_POINT('Ctrl Pts',(4.31884010194003,-1.32709525583961,24.8399689997999));
#32467=CARTESIAN_POINT('Ctrl Pts',(4.45067248416388,-0.898065782199879,
24.855784899036));
#32468=CARTESIAN_POINT('Ctrl Pts',(4.51719389013711,-0.448967520484957,
24.871600798272));
#32469=CARTESIAN_POINT('Ctrl Pts',(4.51742159705025,6.47500723078405E-5,
24.8874166975081));
#32470=CARTESIAN_POINT('Ctrl Pts',(4.51805179992706,-6.79869438786201E-5,
24.612583302492));
#32471=CARTESIAN_POINT('Ctrl Pts',(4.51810196194601,-0.0691007664161157,
24.610150840513));
#32472=CARTESIAN_POINT('Ctrl Pts',(4.51655248974293,-0.13813129299046,24.6077183785341));
#32473=CARTESIAN_POINT('Ctrl Pts',(4.51338856189906,-0.207087743519482,
24.6052859165551));
#32474=CARTESIAN_POINT('Ctrl Pts',(4.47897528910062,-0.957110266274211,
24.5788286198707));
#32475=CARTESIAN_POINT('Ctrl Pts',(4.25356572683319,-1.69836930898188,24.5523713231862));
#32476=CARTESIAN_POINT('Ctrl Pts',(3.8646145103131,-2.3405803406153,24.5259140265017));
#32477=CARTESIAN_POINT('Ctrl Pts',(3.47566329379301,-2.98279137224871,24.4994567298173));
#32478=CARTESIAN_POINT('Ctrl Pts',(2.92317042302025,-3.52595439280789,24.4729994331328));
#32479=CARTESIAN_POINT('Ctrl Pts',(2.27442891819395,-3.90391274752403,24.4465421364483));
#32480=CARTESIAN_POINT('Ctrl Pts',(1.62568741336761,-4.2818711022402,24.4200848397639));
#32481=CARTESIAN_POINT('Ctrl Pts',(0.88069727448771,-4.49462479111332,24.3936275430794));
#32482=CARTESIAN_POINT('Ctrl Pts',(0.130197475965773,-4.51626065030008,
24.3671702463949));
#32483=CARTESIAN_POINT('Ctrl Pts',(-0.620302322556121,-4.53789650948684,
24.3407129497104));
#32484=CARTESIAN_POINT('Ctrl Pts',(-1.37631178072007,-4.36841453898727,
24.314255653026));
#32485=CARTESIAN_POINT('Ctrl Pts',(-2.04574978322055,-4.02845745523667,
24.2877983563415));
#32486=CARTESIAN_POINT('Ctrl Pts',(-2.71518778572104,-3.68850037148608,
24.2613410596571));
#32487=CARTESIAN_POINT('Ctrl Pts',(-3.29805433255807,-3.17806817448446,
24.2348837629726));
#32488=CARTESIAN_POINT('Ctrl Pts',(-3.72335692340428,-2.55933094091641,
24.2084264662881));
#32489=CARTESIAN_POINT('Ctrl Pts',(-4.14865951425051,-1.94059370734831,
24.1819691696036));
#32490=CARTESIAN_POINT('Ctrl Pts',(-4.41639814910591,-1.21355143721374,
24.1555118729192));
#32491=CARTESIAN_POINT('Ctrl Pts',(-4.49396255855832,-0.466757074372799,
24.1290545762347));
#32492=CARTESIAN_POINT('Ctrl Pts',(-4.57152696801073,0.280037288468098,
24.1025972795502));
#32493=CARTESIAN_POINT('Ctrl Pts',(-4.4589171520602,1.04658374401527,24.0761399828658));
#32494=CARTESIAN_POINT('Ctrl Pts',(-4.16984886166344,1.73951778234053,24.0496826861813));
#32495=CARTESIAN_POINT('Ctrl Pts',(-3.88078057126667,2.43245182066584,24.0232253894968));
#32496=CARTESIAN_POINT('Ctrl Pts',(-3.41525380642364,3.05177344176913,23.9967680928124));
#32497=CARTESIAN_POINT('Ctrl Pts',(-2.82996921187404,3.52204995762946,23.9703107961279));
#32498=CARTESIAN_POINT('Ctrl Pts',(-2.24468461732448,3.99232647348976,23.9438534994434));
#32499=CARTESIAN_POINT('Ctrl Pts',(-1.53964219306833,4.31355788410714,23.917396202759));
#32500=CARTESIAN_POINT('Ctrl Pts',(-0.800715326097399,4.44661855917222,
23.8909389060745));
#32501=CARTESIAN_POINT('Ctrl Pts',(-0.0617884591264724,4.5796792342373,
23.86448160939));
#32502=CARTESIAN_POINT('Ctrl Pts',(0.711022850559258,4.5245691737501,23.8380243127056));
#32503=CARTESIAN_POINT('Ctrl Pts',(1.42359104075306,4.28800072211045,23.8115670160211));
#32504=CARTESIAN_POINT('Ctrl Pts',(2.13615923094691,4.05143227047079,23.7851097193366));
#32505=CARTESIAN_POINT('Ctrl Pts',(2.78848430164884,3.63340542767864,23.7586524226522));
#32506=CARTESIAN_POINT('Ctrl Pts',(3.30111378116074,3.08483540049647,23.7321951259677));
#32507=CARTESIAN_POINT('Ctrl Pts',(3.81374326067261,2.53626537331434,23.7057378292832));
#32508=CARTESIAN_POINT('Ctrl Pts',(4.18667714899447,1.85715216174218,23.6792805325988));
#32509=CARTESIAN_POINT('Ctrl Pts',(4.37449251133263,1.13021100344109,23.6528232359143));
#32510=CARTESIAN_POINT('Ctrl Pts',(4.46971107890219,0.761666625925485,23.6394099247735));
#32511=CARTESIAN_POINT('Ctrl Pts',(4.51734893340559,0.380829109202114,23.6259966136328));
#32512=CARTESIAN_POINT('Ctrl Pts',(4.51736327228765,-4.88489681080284E-6,
23.612583302492));
#32513=CARTESIAN_POINT('Origin',(0.,0.,20.5));
#32514=CARTESIAN_POINT('',(4.51802736372575,7.65320072124154E-5,22.612583302492));
#32515=CARTESIAN_POINT('',(4.51742427980126,-6.60698246896739E-5,22.8874166975081));
#32516=CARTESIAN_POINT('',(4.51775,5.53264807684796E-16,20.5));
#32517=CARTESIAN_POINT('Ctrl Pts',(4.51742427980126,-6.60698246896739E-5,
22.8874166975081));
#32518=CARTESIAN_POINT('Ctrl Pts',(4.51719087600353,0.450661745130009,22.9032923445115));
#32519=CARTESIAN_POINT('Ctrl Pts',(4.450158091451,0.901457458944964,22.9191679915148));
#32520=CARTESIAN_POINT('Ctrl Pts',(4.31734276296,1.3319583722546,22.9350436385182));
#32521=CARTESIAN_POINT('Ctrl Pts',(4.09600157608532,2.04940254217993,22.9615009352027));
#32522=CARTESIAN_POINT('Ctrl Pts',(3.69196031163168,2.71048127828687,22.9879582318872));
#32523=CARTESIAN_POINT('Ctrl Pts',(3.15443074594463,3.23467592132643,23.0144155285716));
#32524=CARTESIAN_POINT('Ctrl Pts',(2.61690118025762,3.75887056436596,23.0408728252561));
#32525=CARTESIAN_POINT('Ctrl Pts',(1.94588331333721,4.14618111433815,23.0673301219406));
#32526=CARTESIAN_POINT('Ctrl Pts',(1.22310638006181,4.34943357534335,23.093787418625));
#32527=CARTESIAN_POINT('Ctrl Pts',(0.500329446786407,4.55268603634856,23.1202447153095));
#32528=CARTESIAN_POINT('Ctrl Pts',(-0.274206552844009,4.5718804083868,23.146702011994));
#32529=CARTESIAN_POINT('Ctrl Pts',(-1.00616399197876,4.4046788379547,23.1731593086784));
#32530=CARTESIAN_POINT('Ctrl Pts',(-1.73812143111355,4.23747726752258,23.1996166053629));
#32531=CARTESIAN_POINT('Ctrl Pts',(-2.4275003097527,3.88387975462009,23.2260739020474));
#32532=CARTESIAN_POINT('Ctrl Pts',(-2.99033504306372,3.38695408510429,23.2525311987318));
#32533=CARTESIAN_POINT('Ctrl Pts',(-3.55316977637471,2.89002841558852,23.2789884954163));
#32534=CARTESIAN_POINT('Ctrl Pts',(-3.98946036435762,2.24977458945944,23.3054457921008));
#32535=CARTESIAN_POINT('Ctrl Pts',(-4.24606709644918,1.54417481408558,23.3319030887853));
#32536=CARTESIAN_POINT('Ctrl Pts',(-4.50267382854076,0.838575038711681,
23.3583603854697));
#32537=CARTESIAN_POINT('Ctrl Pts',(-4.57959670474098,0.0676293140930979,
23.3848176821541));
#32538=CARTESIAN_POINT('Ctrl Pts',(-4.46746660375748,-0.674762023707061,
23.4112749788386));
#32539=CARTESIAN_POINT('Ctrl Pts',(-4.35533650277398,-1.41715336150718,
23.4377322755231));
#32540=CARTESIAN_POINT('Ctrl Pts',(-4.05415342460676,-2.13099031248878,
23.4641895722076));
#32541=CARTESIAN_POINT('Ctrl Pts',(-3.60060113490302,-2.72932832606618,
23.4906468688921));
#32542=CARTESIAN_POINT('Ctrl Pts',(-3.14704884519929,-3.32766633964359,
23.5171041655765));
#32543=CARTESIAN_POINT('Ctrl Pts',(-2.54112734395902,-3.81050541581682,
23.543561462261));
#32544=CARTESIAN_POINT('Ctrl Pts',(-1.85663719941186,-4.11903628947138,
23.5700187589454));
#32545=CARTESIAN_POINT('Ctrl Pts',(-1.17214705486469,-4.42756716312594,
23.5964760556299));
#32546=CARTESIAN_POINT('Ctrl Pts',(-0.409088267010601,-4.56178983426184,
23.6229333523144));
#32547=CARTESIAN_POINT('Ctrl Pts',(0.339599448275288,-4.50535613008826,
23.6493906489989));
#32548=CARTESIAN_POINT('Ctrl Pts',(1.08828716356118,-4.44892242591468,23.6758479456834));
#32549=CARTESIAN_POINT('Ctrl Pts',(1.82260380627889,-4.20183234643162,23.7023052423678));
#32550=CARTESIAN_POINT('Ctrl Pts',(2.45311042204474,-3.7941811898551,23.7287625390522));
#32551=CARTESIAN_POINT('Ctrl Pts',(3.08361703781062,-3.38653003327857,23.7552198357367));
#32552=CARTESIAN_POINT('Ctrl Pts',(3.61031362662464,-2.81831779960855,23.7816771324212));
#32553=CARTESIAN_POINT('Ctrl Pts',(3.96904912687646,-2.15875211004929,23.8081344291057));
#32554=CARTESIAN_POINT('Ctrl Pts',(4.32737956599415,-1.49993115979256,23.8345618519065));
#32555=CARTESIAN_POINT('Ctrl Pts',(4.51812800419987,-0.749962938110063,
23.8609892747073));
#32556=CARTESIAN_POINT('Ctrl Pts',(4.51813695063288,9.0056284873609E-7,
23.8874166975081));
#32557=CARTESIAN_POINT('Ctrl Pts',(4.51736327228765,-4.88489681080284E-6,
23.612583302492));
#32558=CARTESIAN_POINT('Ctrl Pts',(4.51737721635919,-0.370352896766723,
23.5995393169483));
#32559=CARTESIAN_POINT('Ctrl Pts',(4.47235409625982,-0.740697577327283,
23.5864953314046));
#32560=CARTESIAN_POINT('Ctrl Pts',(4.38225454858748,-1.09973029228254,23.5734513458609));
#32561=CARTESIAN_POINT('Ctrl Pts',(4.19950438714968,-1.82796132467507,23.5469940491764));
#32562=CARTESIAN_POINT('Ctrl Pts',(3.83130722791959,-2.50965428443002,23.5205367524919));
#32563=CARTESIAN_POINT('Ctrl Pts',(3.3225090776327,-3.06177972318861,23.4940794558075));
#32564=CARTESIAN_POINT('Ctrl Pts',(2.81371092734586,-3.61390516194714,23.467622159123));
#32565=CARTESIAN_POINT('Ctrl Pts',(2.16431178600224,-4.03646307970933,23.4411648624385));
#32566=CARTESIAN_POINT('Ctrl Pts',(1.45340774986053,-4.27798639033802,23.4147075657541));
#32567=CARTESIAN_POINT('Ctrl Pts',(0.742503713718783,-4.51950970096672,
23.3882502690696));
#32568=CARTESIAN_POINT('Ctrl Pts',(-0.0299052172210591,-4.5799984044619,
23.3617929723851));
#32569=CARTESIAN_POINT('Ctrl Pts',(-0.769740489176251,-4.4520850425719,
23.3353356757007));
#32570=CARTESIAN_POINT('Ctrl Pts',(-1.50957576113144,-4.32417168068191,
23.3088783790162));
#32571=CARTESIAN_POINT('Ctrl Pts',(-2.21683737410199,-4.00785625340675,
23.2824210823318));
#32572=CARTESIAN_POINT('Ctrl Pts',(-2.80538164796902,-3.54166563180954,
23.2559637856473));
#32573=CARTESIAN_POINT('Ctrl Pts',(-3.39392592183609,-3.0754750102123,23.2295064889628));
#32574=CARTESIAN_POINT('Ctrl Pts',(-3.86375285659963,-2.459409194293,23.2030491922783));
#32575=CARTESIAN_POINT('Ctrl Pts',(-4.15763804857074,-1.76850431465145,
23.1765918955939));
#32576=CARTESIAN_POINT('Ctrl Pts',(-4.45152324054182,-1.07759943500997,
23.1501345989094));
#32577=CARTESIAN_POINT('Ctrl Pts',(-4.56946668972051,-0.311855491646258,
23.123677302225));
#32578=CARTESIAN_POINT('Ctrl Pts',(-4.49710302020607,0.435460743133651,
23.0972200055405));
#32579=CARTESIAN_POINT('Ctrl Pts',(-4.42473935069162,1.18277697791365,23.070762708856));
#32580=CARTESIAN_POINT('Ctrl Pts',(-4.162068562484,1.91166550410983,23.0443054121715));
#32581=CARTESIAN_POINT('Ctrl Pts',(-3.74108365616062,2.53334852003347,23.017848115487));
#32582=CARTESIAN_POINT('Ctrl Pts',(-3.32009874983724,3.15503153595711,22.9913908188026));
#32583=CARTESIAN_POINT('Ctrl Pts',(-2.74079972539808,3.66950904160819,22.9649335221181));
#32584=CARTESIAN_POINT('Ctrl Pts',(-2.07374458313369,4.01411821952858,22.9384762254337));
#32585=CARTESIAN_POINT('Ctrl Pts',(-1.40668944086933,4.35872739744894,22.9120189287492));
#32586=CARTESIAN_POINT('Ctrl Pts',(-0.651878180779734,4.53346824763863,
22.8855616320647));
#32587=CARTESIAN_POINT('Ctrl Pts',(0.0987540592506666,4.51705757827173,
22.8591043353802));
#32588=CARTESIAN_POINT('Ctrl Pts',(0.849386299281067,4.50064690890482,22.8326470386958));
#32589=CARTESIAN_POINT('Ctrl Pts',(1.59583951925228,4.29308471998132,22.8061897420113));
#32590=CARTESIAN_POINT('Ctrl Pts',(2.24719647092532,3.91965176135188,22.7797324453269));
#32591=CARTESIAN_POINT('Ctrl Pts',(2.89855342259837,3.54621880272245,22.7532751486424));
#32592=CARTESIAN_POINT('Ctrl Pts',(3.45481410597325,3.00691507438708,22.7268178519579));
#32593=CARTESIAN_POINT('Ctrl Pts',(3.8482267217168,2.3674273530564,22.7003605552734));
#32594=CARTESIAN_POINT('Ctrl Pts',(4.24163933746037,1.72793963172568,22.673903258589));
#32595=CARTESIAN_POINT('Ctrl Pts',(4.47220388557259,0.988267917399649,22.6474459619045));
#32596=CARTESIAN_POINT('Ctrl Pts',(4.51183760195935,0.238503067401548,22.6209886652201));
#32597=CARTESIAN_POINT('Ctrl Pts',(4.51603475238966,0.159104107382582,22.618186877644));
#32598=CARTESIAN_POINT('Ctrl Pts',(4.51809071117569,0.0795919580082339,
22.615385090068));
#32599=CARTESIAN_POINT('Ctrl Pts',(4.51802736372575,7.65320072124154E-5,
22.612583302492));
#32600=CARTESIAN_POINT('Origin',(0.,0.,20.5));
#32601=CARTESIAN_POINT('',(4.51732076945549,-0.00048196737157627,21.612583302492));
#32602=CARTESIAN_POINT('',(4.51782520267197,0.000113471772791779,21.8874166975081));
#32603=CARTESIAN_POINT('',(4.51775,5.53264807684796E-16,20.5));
#32604=CARTESIAN_POINT('Ctrl Pts',(4.51782520267197,0.000113471772791779,
21.8874166975081));
#32605=CARTESIAN_POINT('Ctrl Pts',(4.51797972979194,0.149530198200455,21.8926808209467));
#32606=CARTESIAN_POINT('Ctrl Pts',(4.51071347097486,0.298931999583376,21.8979449443854));
#32607=CARTESIAN_POINT('Ctrl Pts',(4.49591510340165,0.447583892947329,21.903209067824));
#32608=CARTESIAN_POINT('Ctrl Pts',(4.4215390356869,1.19470300808371,21.9296663645084));
#32609=CARTESIAN_POINT('Ctrl Pts',(4.15689950898611,1.92287920852908,21.9561236611929));
#32610=CARTESIAN_POINT('Ctrl Pts',(3.73423901960025,2.54342464869698,21.9825809578774));
#32611=CARTESIAN_POINT('Ctrl Pts',(3.3115785302144,3.16397008886483,22.0090382545618));
#32612=CARTESIAN_POINT('Ctrl Pts',(2.7308970781435,3.67688476875521,22.0354955512463));
#32613=CARTESIAN_POINT('Ctrl Pts',(2.06291588716907,4.0196945481291,22.0619528479308));
#32614=CARTESIAN_POINT('Ctrl Pts',(1.39493469619467,4.36250432750298,22.0884101446153));
#32615=CARTESIAN_POINT('Ctrl Pts',(0.639653766316767,4.53520920636039,22.1148674412997));
#32616=CARTESIAN_POINT('Ctrl Pts',(-0.110931801888053,4.51677482186132,
22.1413247379842));
#32617=CARTESIAN_POINT('Ctrl Pts',(-0.861517370093001,4.49834043736225,
22.1677820346687));
#32618=CARTESIAN_POINT('Ctrl Pts',(-1.60740757662484,4.28876678950664,22.1942393313531));
#32619=CARTESIAN_POINT('Ctrl Pts',(-2.25775525993264,3.91357923987666,22.2206966280376));
#32620=CARTESIAN_POINT('Ctrl Pts',(-2.90810294324037,3.53839169024672,22.2471539247221));
#32621=CARTESIAN_POINT('Ctrl Pts',(-3.46290810332406,2.99759023884246,22.2736112214065));
#32622=CARTESIAN_POINT('Ctrl Pts',(-3.85459532302061,2.35704415643024,22.300068518091));
#32623=CARTESIAN_POINT('Ctrl Pts',(-4.24628254271713,1.71649807401806,22.3265258147755));
#32624=CARTESIAN_POINT('Ctrl Pts',(-4.4748518220265,0.976207360597959,22.3529831114599));
#32625=CARTESIAN_POINT('Ctrl Pts',(-4.51246407961468,0.226338472032797,
22.3794404081444));
#32626=CARTESIAN_POINT('Ctrl Pts',(-4.55007633720287,-0.523530416532452,
22.4058977048289));
#32627=CARTESIAN_POINT('Ctrl Pts',(-4.39673157306978,-1.28297748024285,
22.4323550015133));
#32628=CARTESIAN_POINT('Ctrl Pts',(-4.07110679585725,-1.95950283641873,
22.4588122981978));
#32629=CARTESIAN_POINT('Ctrl Pts',(-3.74548201864475,-2.63602819259453,
22.4852695948823));
#32630=CARTESIAN_POINT('Ctrl Pts',(-3.24757722835284,-3.22963184123592,
22.5117268915668));
#32631=CARTESIAN_POINT('Ctrl Pts',(-2.63803679068419,-3.66801355240642,
22.5381841882512));
#32632=CARTESIAN_POINT('Ctrl Pts',(-2.02849635301547,-4.10639526357697,
22.5646414849357));
#32633=CARTESIAN_POINT('Ctrl Pts',(-1.30732026797,-4.38955503727659,22.5910987816201));
#32634=CARTESIAN_POINT('Ctrl Pts',(-0.562346924558367,-4.48300430658586,
22.6175560783046));
#32635=CARTESIAN_POINT('Ctrl Pts',(0.182626418853268,-4.57645357589513,
22.6440133749891));
#32636=CARTESIAN_POINT('Ctrl Pts',(0.951397020631046,-4.48019234081406,
22.6704706716736));
#32637=CARTESIAN_POINT('Ctrl Pts',(1.65032944052472,-4.20594512376056,22.696927968358));
#32638=CARTESIAN_POINT('Ctrl Pts',(2.34926186041832,-3.93169790670708,22.7233852650425));
#32639=CARTESIAN_POINT('Ctrl Pts',(2.97835609842781,-3.47946470768123,22.749842561727));
#32640=CARTESIAN_POINT('Ctrl Pts',(3.46098918943069,-2.90432702425209,22.7762998584114));
#32641=CARTESIAN_POINT('Ctrl Pts',(3.94362228043359,-2.32918934082292,22.8027571550959));
#32642=CARTESIAN_POINT('Ctrl Pts',(4.27979422442984,-1.63114717299047,22.8292144517804));
#32643=CARTESIAN_POINT('Ctrl Pts',(4.42855964178011,-0.89522128720241,22.8556717484648));
#32644=CARTESIAN_POINT('Ctrl Pts',(4.48805867336429,-0.600886230695128,
22.8662533981459));
#32645=CARTESIAN_POINT('Ctrl Pts',(4.51757985123852,-0.300491232865703,
22.876835047827));
#32646=CARTESIAN_POINT('Ctrl Pts',(4.51742427980126,-6.60698246896739E-5,
22.8874166975081));
#32647=CARTESIAN_POINT('Ctrl Pts',(4.51802736372575,7.65320072124154E-5,
22.612583302492));
#32648=CARTESIAN_POINT('Ctrl Pts',(4.51749252083047,-0.671272680948583,
22.5889277933835));
#32649=CARTESIAN_POINT('Ctrl Pts',(4.36588431242158,-1.34285546610394,22.5652722842751));
#32650=CARTESIAN_POINT('Ctrl Pts',(4.07637456299432,-1.94852038806885,22.5416167751666));
#32651=CARTESIAN_POINT('Ctrl Pts',(3.75257492298122,-2.62592100787102,22.5151594784822));
#32652=CARTESIAN_POINT('Ctrl Pts',(3.2562727582937,-3.22086426180528,22.4887021817977));
#32653=CARTESIAN_POINT('Ctrl Pts',(2.64791620593777,-3.66088792814019,22.4622448851133));
#32654=CARTESIAN_POINT('Ctrl Pts',(2.03955965358178,-4.10091159447515,22.4357875884288));
#32655=CARTESIAN_POINT('Ctrl Pts',(1.31914871355735,-4.38601567321071,22.4093302917443));
#32656=CARTESIAN_POINT('Ctrl Pts',(0.574430373257849,-4.48147252184727,
22.3828729950598));
#32657=CARTESIAN_POINT('Ctrl Pts',(-0.17028796704161,-4.57692937048383,
22.3564156983754));
#32658=CARTESIAN_POINT('Ctrl Pts',(-0.939313707616121,-4.48273898902142,
22.3299584016909));
#32659=CARTESIAN_POINT('Ctrl Pts',(-1.63898363511379,-4.21037796912979,
22.3035011050064));
#32660=CARTESIAN_POINT('Ctrl Pts',(-2.33865356261146,-3.93801694923817,
22.277043808322));
#32661=CARTESIAN_POINT('Ctrl Pts',(-2.96896767703227,-3.48748529091735,
22.2505865116375));
#32662=CARTESIAN_POINT('Ctrl Pts',(-3.4531482409959,-2.91364911818973,22.224129214953));
#32663=CARTESIAN_POINT('Ctrl Pts',(-3.93732880495957,-2.33981294546208,
22.1976719182685));
#32664=CARTESIAN_POINT('Ctrl Pts',(-4.27537581846602,-1.64267225832765,
22.1712146215841));
#32665=CARTESIAN_POINT('Ctrl Pts',(-4.42612719062429,-0.907153378338295,
22.1447573248996));
#32666=CARTESIAN_POINT('Ctrl Pts',(-4.57687856278254,-0.171634498348981,
22.1183000282152));
#32667=CARTESIAN_POINT('Ctrl Pts',(-4.5403342935926,0.602262574495347,22.0918427315307));
#32668=CARTESIAN_POINT('Ctrl Pts',(-4.32092341583129,1.32030703112007,22.0653854348462));
#32669=CARTESIAN_POINT('Ctrl Pts',(-4.10151253806998,2.03835148774475,22.0389281381617));
#32670=CARTESIAN_POINT('Ctrl Pts',(-3.69923505173734,2.70054332814993,22.0124708414773));
#32671=CARTESIAN_POINT('Ctrl Pts',(-3.16312948534619,3.2261735651419,21.9860135447928));
#32672=CARTESIAN_POINT('Ctrl Pts',(-2.62702391895502,3.7518038021339,21.9595562481083));
#32673=CARTESIAN_POINT('Ctrl Pts',(-1.95709027250536,4.14087243571266,21.9330989514239));
#32674=CARTESIAN_POINT('Ctrl Pts',(-1.23484721910289,4.34609472311248,21.9066416547394));
#32675=CARTESIAN_POINT('Ctrl Pts',(-0.512604165700429,4.5513170105123,21.880184358055));
#32676=CARTESIAN_POINT('Ctrl Pts',(0.261948294654812,4.57269295173318,21.8537270613705));
#32677=CARTESIAN_POINT('Ctrl Pts',(0.994322299916156,4.40742376897541,21.827269764686));
#32678=CARTESIAN_POINT('Ctrl Pts',(1.72669630517754,4.24215458621763,21.8008124680015));
#32679=CARTESIAN_POINT('Ctrl Pts',(2.41689185534501,3.89024027948119,21.7743551713171));
#32680=CARTESIAN_POINT('Ctrl Pts',(2.9811237744369,3.39491220205643,21.7478978746326));
#32681=CARTESIAN_POINT('Ctrl Pts',(3.54535569352876,2.8995841246317,21.7214405779481));
#32682=CARTESIAN_POINT('Ctrl Pts',(3.98362398154505,2.26084227651867,21.6949832812637));
#32683=CARTESIAN_POINT('Ctrl Pts',(4.24201965646871,1.55578891217676,21.6685259845792));
#32684=CARTESIAN_POINT('Ctrl Pts',(4.42414140114732,1.05885509606931,21.6498784238835));
#32685=CARTESIAN_POINT('Ctrl Pts',(4.51690828804801,0.528979877711725,21.6312308631877));
#32686=CARTESIAN_POINT('Ctrl Pts',(4.51732076945549,-0.00048196737157627,
21.612583302492));
#32687=CARTESIAN_POINT('Origin',(0.,0.,20.5));
#32688=CARTESIAN_POINT('',(4.52133925202235,0.00376432143610439,20.612583302492));
#32689=CARTESIAN_POINT('',(4.50983715083838,-0.000439487622834945,20.8874166975081));
#32690=CARTESIAN_POINT('',(4.51775,5.53264807684796E-16,20.5));
#32691=CARTESIAN_POINT('Ctrl Pts',(4.50983715083838,-0.000439487622834945,
20.8874166975081));
#32692=CARTESIAN_POINT('Ctrl Pts',(4.51223989494407,0.600272225419278,20.9085265940664));
#32693=CARTESIAN_POINT('Ctrl Pts',(4.40045147683232,1.20075832380094,20.9296364906248));
#32694=CARTESIAN_POINT('Ctrl Pts',(4.16995632188889,1.7527710518725,20.9507463871831));
#32695=CARTESIAN_POINT('Ctrl Pts',(3.88107386896856,2.44461548985082,20.9772036838676));
#32696=CARTESIAN_POINT('Ctrl Pts',(3.40572780474968,3.06031833788172,21.0036609805521));
#32697=CARTESIAN_POINT('Ctrl Pts',(2.81753981467946,3.528620768205,21.0301182772365));
#32698=CARTESIAN_POINT('Ctrl Pts',(2.22935182460931,3.99692319852822,21.056575573921));
#32699=CARTESIAN_POINT('Ctrl Pts',(1.52832190868785,4.31782521114387,21.0830328706055));
#32700=CARTESIAN_POINT('Ctrl Pts',(0.790149843231595,4.44924273175288,21.1094901672899));
#32701=CARTESIAN_POINT('Ctrl Pts',(0.051977777775257,4.58066025236192,21.1359474639744));
#32702=CARTESIAN_POINT('Ctrl Pts',(-0.723336437215882,4.52259328096428,
21.1624047606589));
#32703=CARTESIAN_POINT('Ctrl Pts',(-1.43588412720356,4.28390166798379,21.1888620573433));
#32704=CARTESIAN_POINT('Ctrl Pts',(-2.14843181719121,4.04521005500332,21.2153193540278));
#32705=CARTESIAN_POINT('Ctrl Pts',(-2.7982129821754,3.62589380044002,21.2417766507123));
#32706=CARTESIAN_POINT('Ctrl Pts',(-3.30902952393807,3.07605344225317,21.2682339473967));
#32707=CARTESIAN_POINT('Ctrl Pts',(-3.81984606570073,2.52621308406631,21.2946912440812));
#32708=CARTESIAN_POINT('Ctrl Pts',(-4.19169798424187,1.84584862225589,21.3211485407657));
#32709=CARTESIAN_POINT('Ctrl Pts',(-4.37772925931563,1.11834540158705,21.3476058374502));
#32710=CARTESIAN_POINT('Ctrl Pts',(-4.56376053438938,0.390842180918212,
21.3740631341346));
#32711=CARTESIAN_POINT('Ctrl Pts',(-4.56397116599575,-0.383799798609046,
21.4005204308191));
#32712=CARTESIAN_POINT('Ctrl Pts',(-4.37916492462626,-1.11150455739398,
21.4269777275035));
#32713=CARTESIAN_POINT('Ctrl Pts',(-4.19435868325677,-1.83920931617892,
21.453435024188));
#32714=CARTESIAN_POINT('Ctrl Pts',(-3.82453556891143,-2.51997685422154,
21.4798923208725));
#32715=CARTESIAN_POINT('Ctrl Pts',(-3.31430027943462,-3.07074498667336,
21.5063496175569));
#32716=CARTESIAN_POINT('Ctrl Pts',(-2.80406498995777,-3.62151311912521,
21.5328069142414));
#32717=CARTESIAN_POINT('Ctrl Pts',(-2.15341752534944,-4.04228184598626,
21.5592642109259));
#32718=CARTESIAN_POINT('Ctrl Pts',(-1.44183871719702,-4.28187903967218,
21.5857215076104));
#32719=CARTESIAN_POINT('Ctrl Pts',(-0.730259909044641,-4.5214762333581,
21.6121788042948));
#32720=CARTESIAN_POINT('Ctrl Pts',(0.0422502426518133,-4.57990189386891,
21.6386361009793));
#32721=CARTESIAN_POINT('Ctrl Pts',(0.781724091400323,-4.44999904027082,
21.6650933976638));
#32722=CARTESIAN_POINT('Ctrl Pts',(1.52119794014883,-4.32009618667273,21.6915506943482));
#32723=CARTESIAN_POINT('Ctrl Pts',(2.2276354859494,-4.00186481896572,21.7180079910327));
#32724=CARTESIAN_POINT('Ctrl Pts',(2.81492815165366,-3.53408677354305,21.7444652877172));
#32725=CARTESIAN_POINT('Ctrl Pts',(3.40222081735796,-3.06630872812035,21.7709225844016));
#32726=CARTESIAN_POINT('Ctrl Pts',(3.87036860296593,-2.44898400498197,21.7973798810861));
#32727=CARTESIAN_POINT('Ctrl Pts',(4.16238619140555,-1.75729062849908,21.8238371777706));
#32728=CARTESIAN_POINT('Ctrl Pts',(4.39630197715038,-1.20322126398217,21.8450303510164));
#32729=CARTESIAN_POINT('Ctrl Pts',(4.51720308199739,-0.601432940640185,
21.8662235242623));
#32730=CARTESIAN_POINT('Ctrl Pts',(4.51782520267197,0.000113471772791779,
21.8874166975081));
#32731=CARTESIAN_POINT('Ctrl Pts',(4.51732076945549,-0.00048196737157627,
21.612583302492));
#32732=CARTESIAN_POINT('Ctrl Pts',(4.51749351971195,-0.222224494111391,
21.6047735665033));
#32733=CARTESIAN_POINT('Ctrl Pts',(4.50146734240306,-0.44389451533626,21.5969638305145));
#32734=CARTESIAN_POINT('Ctrl Pts',(4.46902189478939,-0.663041834113329,
21.5891540945258));
#32735=CARTESIAN_POINT('Ctrl Pts',(4.35910539635538,-1.40545433549076,21.5626967978413));
#32736=CARTESIAN_POINT('Ctrl Pts',(4.06074933765633,-2.11891445767478,21.5362395011569));
#32737=CARTESIAN_POINT('Ctrl Pts',(3.60841564297682,-2.71899122382358,21.5097822044724));
#32738=CARTESIAN_POINT('Ctrl Pts',(3.15608194829734,-3.31906798997234,21.4833249077879));
#32739=CARTESIAN_POINT('Ctrl Pts',(2.54977061763742,-3.80576140008588,21.4568676111035));
#32740=CARTESIAN_POINT('Ctrl Pts',(1.86683275295722,-4.11521969441498,21.430410314419));
#32741=CARTESIAN_POINT('Ctrl Pts',(1.18389488827701,-4.42467798874409,21.4039530177345));
#32742=CARTESIAN_POINT('Ctrl Pts',(0.424330489576522,-4.55690116728877,
21.37749572105));
#32743=CARTESIAN_POINT('Ctrl Pts',(-0.325633495564533,-4.50373822059831,
21.3510384243656));
#32744=CARTESIAN_POINT('Ctrl Pts',(-1.07559748070559,-4.45057527390784,
21.3245811276811));
#32745=CARTESIAN_POINT('Ctrl Pts',(-1.81596105228721,-4.21202620198225,
21.2981238309967));
#32746=CARTESIAN_POINT('Ctrl Pts',(-2.44569775560519,-3.80516814017082,
21.2716665343122));
#32747=CARTESIAN_POINT('Ctrl Pts',(-3.70517116224116,-2.99145201654798,
21.2187519409433));
#32748=CARTESIAN_POINT('Ctrl Pts',(-4.52213709582257,-1.50449993338184,
21.1658373475743));
#32749=CARTESIAN_POINT('Ctrl Pts',(-4.5251392293927,-0.0110172863203392,
21.1129227542054));
#32750=CARTESIAN_POINT('Ctrl Pts',(-4.52814136296284,1.4824653607412,21.0600081608364));
#32751=CARTESIAN_POINT('Ctrl Pts',(-3.71717969652165,2.98247857169809,21.0070935674675));
#32752=CARTESIAN_POINT('Ctrl Pts',(-2.46290199004371,3.79700220422752,20.9541789740986));
#32753=CARTESIAN_POINT('Ctrl Pts',(-1.20862428356581,4.61152583675692,20.9012643807296));
#32754=CARTESIAN_POINT('Ctrl Pts',(0.488969462948824,4.7405598908589,20.8483497873607));
#32755=CARTESIAN_POINT('Ctrl Pts',(1.85305394748095,4.12790602103174,20.7954351939918));
#32756=CARTESIAN_POINT('Ctrl Pts',(3.21713843201311,3.51525215120457,20.7425206006228));
#32757=CARTESIAN_POINT('Ctrl Pts',(4.24771365456276,2.16091035744822,20.6896060072539));
#32758=CARTESIAN_POINT('Ctrl Pts',(4.47332054780559,0.68305737845925,20.636691413885));
#32759=CARTESIAN_POINT('Ctrl Pts',(4.5075830310957,0.458618699879782,20.628655376754));
#32760=CARTESIAN_POINT('Ctrl Pts',(4.52327979691323,0.231331370382945,20.620619339623));
#32761=CARTESIAN_POINT('Ctrl Pts',(4.52133925202235,0.00376432143610439,
20.612583302492));
#32762=CARTESIAN_POINT('Origin',(0.,0.,20.5));
#32763=CARTESIAN_POINT('',(4.51048356578783,0.00141370502139415,19.612583302492));
#32764=CARTESIAN_POINT('',(4.51474283421141,-0.0038924084009401,19.8874166975081));
#32765=CARTESIAN_POINT('',(4.51775,5.53264807684796E-16,20.5));
#32766=CARTESIAN_POINT('Ctrl Pts',(4.51474283421141,-0.00389240840094011,
19.8874166975081));
#32767=CARTESIAN_POINT('Ctrl Pts',(4.50621483686762,1.04654996357473,19.9243723671861));
#32768=CARTESIAN_POINT('Ctrl Pts',(4.14085607956887,2.10234645737149,19.9613280368642));
#32769=CARTESIAN_POINT('Ctrl Pts',(3.4708839066554,2.90334883526624,19.9982837065423));
#32770=CARTESIAN_POINT('Ctrl Pts',(2.51159118088301,4.05025580469952,20.0511982999112));
#32771=CARTESIAN_POINT('Ctrl Pts',(0.927790752426727,4.6747928461432,20.1041128932802));
#32772=CARTESIAN_POINT('Ctrl Pts',(-0.556105607180406,4.49092827001162,
20.1570274866491));
#32773=CARTESIAN_POINT('Ctrl Pts',(-2.04000196678754,4.30706369388004,20.209942080018));
#32774=CARTESIAN_POINT('Ctrl Pts',(-3.42399425754553,3.3147975001732,20.262856673387));
#32775=CARTESIAN_POINT('Ctrl Pts',(-4.07445610293379,1.9687487323051,20.3157712667559));
#32776=CARTESIAN_POINT('Ctrl Pts',(-4.72491794832207,0.622699964436965,
20.3686858601248));
#32777=CARTESIAN_POINT('Ctrl Pts',(-4.64184934834058,-1.07713137759245,
20.4216004534938));
#32778=CARTESIAN_POINT('Ctrl Pts',(-3.86404219126196,-2.3542716484918,20.4745150468627));
#32779=CARTESIAN_POINT('Ctrl Pts',(-3.08623503418336,-3.63141191939111,
20.5274296402316));
#32780=CARTESIAN_POINT('Ctrl Pts',(-1.61368932000766,-4.48586111916038,
20.5803442336006));
#32781=CARTESIAN_POINT('Ctrl Pts',(-0.118635503777389,-4.52427204848619,
20.6332588269695));
#32782=CARTESIAN_POINT('Ctrl Pts',(1.37641831245292,-4.56268297781199,20.6861734203384));
#32783=CARTESIAN_POINT('Ctrl Pts',(2.89398023073781,-3.78505563669429,20.7390880137074));
#32784=CARTESIAN_POINT('Ctrl Pts',(3.73680595955696,-2.55211434826229,20.7920026070763));
#32785=CARTESIAN_POINT('Ctrl Pts',(4.24339242394412,-1.81104612176332,20.8238073038869));
#32786=CARTESIAN_POINT('Ctrl Pts',(4.50621711662441,-0.905486741220779,
20.8556120006975));
#32787=CARTESIAN_POINT('Ctrl Pts',(4.50983715083838,-0.000439487622834945,
20.8874166975081));
#32788=CARTESIAN_POINT('Ctrl Pts',(4.52133925202235,0.00376432143610439,
20.612583302492));
#32789=CARTESIAN_POINT('Ctrl Pts',(4.51050196349347,-1.26712087204873,20.567704746254));
#32790=CARTESIAN_POINT('Ctrl Pts',(3.94958417430038,-2.54673008347757,20.5228261900161));
#32791=CARTESIAN_POINT('Ctrl Pts',(3.00029299713898,-3.38761451526673,20.4779476337781));
#32792=CARTESIAN_POINT('Ctrl Pts',(1.88101998929342,-4.37906926578227,20.4250330404092));
#32793=CARTESIAN_POINT('Ctrl Pts',(0.221835409666229,-4.76061460259175,
20.3721184470403));
#32794=CARTESIAN_POINT('Ctrl Pts',(-1.21815646492133,-4.35804593593179,
20.3192038536714));
#32795=CARTESIAN_POINT('Ctrl Pts',(-2.65814833950885,-3.95547726927185,
20.2662892603024));
#32796=CARTESIAN_POINT('Ctrl Pts',(-3.87894750905677,-2.76879459914251,
20.2133746669335));
#32797=CARTESIAN_POINT('Ctrl Pts',(-4.32195458228653,-1.34081481536639,
20.1604600735645));
#32798=CARTESIAN_POINT('Ctrl Pts',(-4.76496165551631,0.0871649684097867,
20.1075454801956));
#32799=CARTESIAN_POINT('Ctrl Pts',(-4.43017663242789,1.75644186583272,20.0546308868267));
#32800=CARTESIAN_POINT('Ctrl Pts',(-3.47088390665552,2.90334883526609,20.0017162934577));
#32801=CARTESIAN_POINT('Ctrl Pts',(-2.51159118088318,4.05025580469941,19.9488017000888));
#32802=CARTESIAN_POINT('Ctrl Pts',(-0.927790752426926,4.67479284614316,
19.8958871067198));
#32803=CARTESIAN_POINT('Ctrl Pts',(0.556105607180211,4.49092827001165,19.8429725133509));
#32804=CARTESIAN_POINT('Ctrl Pts',(2.04000196678735,4.30706369388013,19.790057919982));
#32805=CARTESIAN_POINT('Ctrl Pts',(3.42399425754539,3.31479750017334,19.737143326613));
#32806=CARTESIAN_POINT('Ctrl Pts',(4.07445610293371,1.96874873230528,19.6842287332441));
#32807=CARTESIAN_POINT('Ctrl Pts',(4.36802741054216,1.36123992961467,19.6603469229934));
#32808=CARTESIAN_POINT('Ctrl Pts',(4.51218113590681,0.681666855829588,19.6364651127427));
#32809=CARTESIAN_POINT('Ctrl Pts',(4.51048356578783,0.00141370502139415,
19.612583302492));
#32810=CARTESIAN_POINT('Origin',(0.,0.,20.5));
#32811=CARTESIAN_POINT('',(4.51751172608841,-5.0340792907555E-5,18.612583302492));
#32812=CARTESIAN_POINT('',(4.52514732618828,-0.0014363825736758,18.8874166975081));
#32813=CARTESIAN_POINT('',(4.51775,5.53264807684796E-16,20.5));
#32814=CARTESIAN_POINT('Ctrl Pts',(4.52514732618828,-0.0014363825736758,
18.8874166975081));
#32815=CARTESIAN_POINT('Ctrl Pts',(4.52467107616349,1.48887736965158,18.9402181403059));
#32816=CARTESIAN_POINT('Ctrl Pts',(3.71449759637046,2.98422031831989,18.9930195831037));
#32817=CARTESIAN_POINT('Ctrl Pts',(2.46290199004355,3.79700220422763,19.0458210259014));
#32818=CARTESIAN_POINT('Ctrl Pts',(1.20862428356557,4.611525836757,19.0987356192704));
#32819=CARTESIAN_POINT('Ctrl Pts',(-0.488969462949119,4.74055989085888,
19.1516502126393));
#32820=CARTESIAN_POINT('Ctrl Pts',(-1.85305394748124,4.12790602103161,19.2045648060083));
#32821=CARTESIAN_POINT('Ctrl Pts',(-3.21713843201331,3.51525215120436,19.2574793993772));
#32822=CARTESIAN_POINT('Ctrl Pts',(-4.24771365456286,2.16091035744797,19.3103939927461));
#32823=CARTESIAN_POINT('Ctrl Pts',(-4.47332054780562,0.683057378459056,
19.3633085861151));
#32824=CARTESIAN_POINT('Ctrl Pts',(-4.69892744104839,-0.794795600529883,
19.416223179484));
#32825=CARTESIAN_POINT('Ctrl Pts',(-4.1195660049844,-2.3961597647514,19.4691377728529));
#32826=CARTESIAN_POINT('Ctrl Pts',(-3.00029299713883,-3.38761451526686,
19.5220523662219));
#32827=CARTESIAN_POINT('Ctrl Pts',(-1.8810199892932,-4.37906926578239,19.5749669595908));
#32828=CARTESIAN_POINT('Ctrl Pts',(-0.221835409665938,-4.76061460259178,
19.6278815529597));
#32829=CARTESIAN_POINT('Ctrl Pts',(1.21815646492164,-4.35804593593171,19.6807961463287));
#32830=CARTESIAN_POINT('Ctrl Pts',(2.6581483395091,-3.95547726927166,19.7337107396976));
#32831=CARTESIAN_POINT('Ctrl Pts',(3.8789475090569,-2.76879459914231,19.7866253330665));
#32832=CARTESIAN_POINT('Ctrl Pts',(4.32195458228659,-1.3408148153662,19.8395399264355));
#32833=CARTESIAN_POINT('Ctrl Pts',(4.45556453043254,-0.910139288059504,
19.8554988501263));
#32834=CARTESIAN_POINT('Ctrl Pts',(4.51842556165299,-0.457515081242471,
19.8714577738172));
#32835=CARTESIAN_POINT('Ctrl Pts',(4.51474283421141,-0.00389240840094011,
19.8874166975081));
#32836=CARTESIAN_POINT('Ctrl Pts',(4.51048356578783,0.00141370502139415,
19.612583302492));
#32837=CARTESIAN_POINT('Ctrl Pts',(4.50841985350745,-0.825560548001291,
19.5835505193738));
#32838=CARTESIAN_POINT('Ctrl Pts',(4.29080360170741,-1.65353988177363,19.5545177362555));
#32839=CARTESIAN_POINT('Ctrl Pts',(3.86404219126206,-2.35427164849163,19.5254849531373));
#32840=CARTESIAN_POINT('Ctrl Pts',(3.08623503418352,-3.63141191939097,19.4725703597684));
#32841=CARTESIAN_POINT('Ctrl Pts',(1.61368932000785,-4.48586111916031,19.4196557663994));
#32842=CARTESIAN_POINT('Ctrl Pts',(0.118635503777585,-4.52427204848618,
19.3667411730305));
#32843=CARTESIAN_POINT('Ctrl Pts',(-1.37641831245272,-4.56268297781205,
19.3138265796616));
#32844=CARTESIAN_POINT('Ctrl Pts',(-2.89398023073765,-3.78505563669441,
19.2609119862926));
#32845=CARTESIAN_POINT('Ctrl Pts',(-3.73680595955685,-2.55211434826245,
19.2079973929237));
#32846=CARTESIAN_POINT('Ctrl Pts',(-4.57963168837605,-1.3191730598305,19.1550827995547));
#32847=CARTESIAN_POINT('Ctrl Pts',(-4.74772122772955,0.369082175915713,
19.1021682061858));
#32848=CARTESIAN_POINT('Ctrl Pts',(-4.16995632188897,1.75277105187232,19.0492536128169));
#32849=CARTESIAN_POINT('Ctrl Pts',(-3.88107386896868,2.44461548985061,19.0227963161324));
#32850=CARTESIAN_POINT('Ctrl Pts',(-3.40572780474986,3.0603183378815,18.9963390194479));
#32851=CARTESIAN_POINT('Ctrl Pts',(-2.81753981467971,3.5286207682048,18.9698817227635));
#32852=CARTESIAN_POINT('Ctrl Pts',(-2.22935182460953,3.99692319852811,18.943424426079));
#32853=CARTESIAN_POINT('Ctrl Pts',(-1.52832190868799,4.31782521114383,18.9169671293945));
#32854=CARTESIAN_POINT('Ctrl Pts',(-0.790149843231659,4.44924273175287,
18.8905098327101));
#32855=CARTESIAN_POINT('Ctrl Pts',(-0.0519777777753676,4.58066025236191,
18.8640525360256));
#32856=CARTESIAN_POINT('Ctrl Pts',(0.72333643721573,4.5225932809643,18.8375952393411));
#32857=CARTESIAN_POINT('Ctrl Pts',(1.43588412720338,4.28390166798386,18.8111379426567));
#32858=CARTESIAN_POINT('Ctrl Pts',(2.14843181719103,4.04521005500342,18.7846806459722));
#32859=CARTESIAN_POINT('Ctrl Pts',(2.79821298217524,3.62589380044014,18.7582233492877));
#32860=CARTESIAN_POINT('Ctrl Pts',(3.30902952393793,3.07605344225331,18.7317660526033));
#32861=CARTESIAN_POINT('Ctrl Pts',(3.81984606570062,2.52621308406647,18.7053087559188));
#32862=CARTESIAN_POINT('Ctrl Pts',(4.19169798424179,1.84584862225607,18.6788514592343));
#32863=CARTESIAN_POINT('Ctrl Pts',(4.37772925931557,1.11834540158724,18.6523941625499));
#32864=CARTESIAN_POINT('Ctrl Pts',(4.47103767181987,0.753448850803234,18.6391238758639));
#32865=CARTESIAN_POINT('Ctrl Pts',(4.51759801973486,0.3766933068382,18.625853589178));
#32866=CARTESIAN_POINT('Ctrl Pts',(4.51751172608841,-5.0340792907555E-5,
18.612583302492));
#32867=CARTESIAN_POINT('Origin',(0.,0.,20.5));
#32868=CARTESIAN_POINT('',(4.51803700570725,7.32895604327321E-5,17.612583302492));
#32869=CARTESIAN_POINT('',(4.51742050630483,-6.62530376704942E-5,17.8874166975081));
#32870=CARTESIAN_POINT('',(4.51775,5.53264807684796E-16,20.5));
#32871=CARTESIAN_POINT('Ctrl Pts',(4.51742050630483,-6.62530376705099E-5,
17.8874166975081));
#32872=CARTESIAN_POINT('Ctrl Pts',(4.5172038153436,0.446598657046559,17.9031493200567));
#32873=CARTESIAN_POINT('Ctrl Pts',(4.4513943616742,0.893327565156709,17.9188819426052));
#32874=CARTESIAN_POINT('Ctrl Pts',(4.32092341583127,1.32030703112013,17.9346145651538));
#32875=CARTESIAN_POINT('Ctrl Pts',(4.10151253806993,2.03835148774488,17.9610718618383));
#32876=CARTESIAN_POINT('Ctrl Pts',(3.6992350517372,2.70054332815014,17.9875291585227));
#32877=CARTESIAN_POINT('Ctrl Pts',(3.16312948534596,3.22617356514213,18.0139864552072));
#32878=CARTESIAN_POINT('Ctrl Pts',(2.62702391895476,3.75180380213408,18.0404437518917));
#32879=CARTESIAN_POINT('Ctrl Pts',(1.95709027250505,4.1408724357128,18.0669010485761));
#32880=CARTESIAN_POINT('Ctrl Pts',(1.23484721910258,4.34609472311257,18.0933583452606));
#32881=CARTESIAN_POINT('Ctrl Pts',(0.51260416570011,4.55131701051233,18.1198156419451));
#32882=CARTESIAN_POINT('Ctrl Pts',(-0.261948294655145,4.57269295173316,
18.1462729386295));
#32883=CARTESIAN_POINT('Ctrl Pts',(-0.994322299916471,4.40742376897534,
18.172730235314));
#32884=CARTESIAN_POINT('Ctrl Pts',(-1.72669630517784,4.24215458621751,18.1991875319985));
#32885=CARTESIAN_POINT('Ctrl Pts',(-2.41689185534529,3.89024027948101,18.225644828683));
#32886=CARTESIAN_POINT('Ctrl Pts',(-2.98112377443714,3.39491220205621,18.2521021253674));
#32887=CARTESIAN_POINT('Ctrl Pts',(-3.54535569352893,2.89958412463147,18.2785594220519));
#32888=CARTESIAN_POINT('Ctrl Pts',(-3.98362398154516,2.26084227651845,18.3050167187363));
#32889=CARTESIAN_POINT('Ctrl Pts',(-4.24201965646877,1.55578891217658,18.3314740154208));
#32890=CARTESIAN_POINT('Ctrl Pts',(-4.50041533139241,0.85073554783464,18.3579313121053));
#32891=CARTESIAN_POINT('Ctrl Pts',(-4.5789383932234,0.0793706672638789,
18.3843886087897));
#32892=CARTESIAN_POINT('Ctrl Pts',(-4.46902189478936,-0.663041834113523,
18.4108459054742));
#32893=CARTESIAN_POINT('Ctrl Pts',(-4.35910539635533,-1.4054543354909,18.4373032021587));
#32894=CARTESIAN_POINT('Ctrl Pts',(-4.06074933765627,-2.11891445767488,
18.4637604988432));
#32895=CARTESIAN_POINT('Ctrl Pts',(-3.60841564297678,-2.71899122382363,
18.4902177955276));
#32896=CARTESIAN_POINT('Ctrl Pts',(-3.15608194829727,-3.31906798997241,
18.5166750922121));
#32897=CARTESIAN_POINT('Ctrl Pts',(-2.54977061763729,-3.80576140008597,
18.5431323888965));
#32898=CARTESIAN_POINT('Ctrl Pts',(-1.86683275295704,-4.11521969441507,
18.569589685581));
#32899=CARTESIAN_POINT('Ctrl Pts',(-1.18389488827682,-4.42467798874415,
18.5960469822655));
#32900=CARTESIAN_POINT('Ctrl Pts',(-0.424330489576326,-4.55690116728879,
18.62250427895));
#32901=CARTESIAN_POINT('Ctrl Pts',(0.325633495564726,-4.5037382205983,18.6489615756344));
#32902=CARTESIAN_POINT('Ctrl Pts',(1.07559748070578,-4.4505752739078,18.6754188723189));
#32903=CARTESIAN_POINT('Ctrl Pts',(1.8159610522874,-4.21202620198217,18.7018761690034));
#32904=CARTESIAN_POINT('Ctrl Pts',(2.44569775560536,-3.80516814017072,18.7283334656878));
#32905=CARTESIAN_POINT('Ctrl Pts',(3.70517116224129,-2.99145201654782,18.7812480590567));
#32906=CARTESIAN_POINT('Ctrl Pts',(4.52213709582263,-1.50449993338164,18.8341626524257));
#32907=CARTESIAN_POINT('Ctrl Pts',(4.5251392293927,-0.0110172863201459,
18.8870772457947));
#32908=CARTESIAN_POINT('Ctrl Pts',(4.52514564904193,-0.00782367934410926,
18.8871903963658));
#32909=CARTESIAN_POINT('Ctrl Pts',(4.52514834676573,-0.00463004250646042,
18.887303546937));
#32910=CARTESIAN_POINT('Ctrl Pts',(4.52514732618828,-0.00143638257367575,
18.8874166975081));
#32911=CARTESIAN_POINT('Ctrl Pts',(4.51751172608841,-5.0340792907555E-5,
18.612583302492));
#32912=CARTESIAN_POINT('Ctrl Pts',(4.51742597397124,-0.374429761958339,
18.5993962924935));
#32913=CARTESIAN_POINT('Ctrl Pts',(4.47127719829474,-0.748797435630456,
18.586209282495));
#32914=CARTESIAN_POINT('Ctrl Pts',(4.37916492462631,-1.11150455739379,18.5730222724965));
#32915=CARTESIAN_POINT('Ctrl Pts',(4.19435868325684,-1.83920931617878,18.546564975812));
#32916=CARTESIAN_POINT('Ctrl Pts',(3.8245355689115,-2.51997685422145,18.5201076791275));
#32917=CARTESIAN_POINT('Ctrl Pts',(3.31430027943466,-3.07074498667331,18.493650382443));
#32918=CARTESIAN_POINT('Ctrl Pts',(2.80406498995785,-3.62151311912514,18.4671930857586));
#32919=CARTESIAN_POINT('Ctrl Pts',(2.15341752534957,-4.04228184598617,18.4407357890741));
#32920=CARTESIAN_POINT('Ctrl Pts',(1.4418387171972,-4.28187903967212,18.4142784923896));
#32921=CARTESIAN_POINT('Ctrl Pts',(0.730259909044834,-4.52147623335806,
18.3878211957052));
#32922=CARTESIAN_POINT('Ctrl Pts',(-0.0422502426516132,-4.57990189386892,
18.3613638990207));
#32923=CARTESIAN_POINT('Ctrl Pts',(-0.781724091400131,-4.44999904027085,
18.3349066023362));
#32924=CARTESIAN_POINT('Ctrl Pts',(-1.52119794014869,-4.32009618667279,
18.3084493056518));
#32925=CARTESIAN_POINT('Ctrl Pts',(-2.2276354859493,-4.00186481896578,18.2819920089673));
#32926=CARTESIAN_POINT('Ctrl Pts',(-2.81492815165361,-3.53408677354309,
18.2555347122828));
#32927=CARTESIAN_POINT('Ctrl Pts',(-3.40222081735788,-3.06630872812042,
18.2290774155984));
#32928=CARTESIAN_POINT('Ctrl Pts',(-3.87036860296584,-2.4489840049821,18.2026201189139));
#32929=CARTESIAN_POINT('Ctrl Pts',(-4.16238619140547,-1.75729062849926,
18.1761628222294));
#32930=CARTESIAN_POINT('Ctrl Pts',(-4.45440377984509,-1.06559725201643,
18.149705525545));
#32931=CARTESIAN_POINT('Ctrl Pts',(-4.57029117111638,-0.299535222189059,
18.1232482288605));
#32932=CARTESIAN_POINT('Ctrl Pts',(-4.49591510340165,0.447583892947263,
18.096790932176));
#32933=CARTESIAN_POINT('Ctrl Pts',(-4.42153903568692,1.19470300808361,18.0703336354916));
#32934=CARTESIAN_POINT('Ctrl Pts',(-4.15689950898618,1.92287920852894,18.0438763388071));
#32935=CARTESIAN_POINT('Ctrl Pts',(-3.73423901960036,2.54342464869681,18.0174190421226));
#32936=CARTESIAN_POINT('Ctrl Pts',(-3.31157853021454,3.16397008886469,17.9909617454381));
#32937=CARTESIAN_POINT('Ctrl Pts',(-2.73089707814366,3.67688476875509,17.9645044487537));
#32938=CARTESIAN_POINT('Ctrl Pts',(-2.06291588716924,4.01969454812901,17.9380471520692));
#32939=CARTESIAN_POINT('Ctrl Pts',(-1.39493469619478,4.36250432750296,17.9115898553848));
#32940=CARTESIAN_POINT('Ctrl Pts',(-0.639653766316788,4.53520920636039,
17.8851325587003));
#32941=CARTESIAN_POINT('Ctrl Pts',(0.110931801888114,4.51677482186132,17.8586752620158));
#32942=CARTESIAN_POINT('Ctrl Pts',(0.861517370092973,4.49834043736224,17.8322179653313));
#32943=CARTESIAN_POINT('Ctrl Pts',(1.60740757662473,4.28876678950667,17.8057606686469));
#32944=CARTESIAN_POINT('Ctrl Pts',(2.25775525993247,3.91357923987676,17.7793033719624));
#32945=CARTESIAN_POINT('Ctrl Pts',(2.90810294324022,3.53839169024685,17.7528460752779));
#32946=CARTESIAN_POINT('Ctrl Pts',(3.46290810332394,2.99759023884261,17.7263887785935));
#32947=CARTESIAN_POINT('Ctrl Pts',(3.8545953230205,2.35704415643041,17.699931481909));
#32948=CARTESIAN_POINT('Ctrl Pts',(4.24628254271708,1.71649807401819,17.6734741852245));
#32949=CARTESIAN_POINT('Ctrl Pts',(4.47485182202649,0.976207360598019,17.6470168885401));
#32950=CARTESIAN_POINT('Ctrl Pts',(4.51246407961468,0.226338472032798,17.6205595918556));
#32951=CARTESIAN_POINT('Ctrl Pts',(4.51624383400808,0.150982181084616,17.6179008287344));
#32952=CARTESIAN_POINT('Ctrl Pts',(4.5180951579083,0.0755291623761646,17.6152420656132));
#32953=CARTESIAN_POINT('Ctrl Pts',(4.51803700570725,7.32895604327322E-5,
17.612583302492));
#32954=CARTESIAN_POINT('Origin',(0.,0.,20.5));
#32955=CARTESIAN_POINT('',(4.51759135405446,-0.000109312323752775,16.612583302492));
#32956=CARTESIAN_POINT('',(4.51783748975292,0.000112199089269072,16.8874166975081));
#32957=CARTESIAN_POINT('',(4.51775,5.53264807684796E-16,20.5));
#32958=CARTESIAN_POINT('Ctrl Pts',(4.51783748975292,0.000112199089269072,
16.8874166975081));
#32959=CARTESIAN_POINT('Ctrl Pts',(4.5179865637855,0.145467881021208,16.8925377964919));
#32960=CARTESIAN_POINT('Ctrl Pts',(4.51110979946378,0.290809516813962,16.8976588954757));
#32961=CARTESIAN_POINT('Ctrl Pts',(4.49710302020602,0.435460743134165,16.9027799944596));
#32962=CARTESIAN_POINT('Ctrl Pts',(4.42473935069149,1.18277697791411,16.929237291144));
#32963=CARTESIAN_POINT('Ctrl Pts',(4.16206856248382,1.91166550411022,16.9556945878285));
#32964=CARTESIAN_POINT('Ctrl Pts',(3.7410836561604,2.53334852003379,16.9821518845129));
#32965=CARTESIAN_POINT('Ctrl Pts',(3.320098749837,3.15503153595733,17.0086091811974));
#32966=CARTESIAN_POINT('Ctrl Pts',(2.74079972539787,3.66950904160833,17.0350664778819));
#32967=CARTESIAN_POINT('Ctrl Pts',(2.07374458313351,4.01411821952866,17.0615237745663));
#32968=CARTESIAN_POINT('Ctrl Pts',(1.40668944086914,4.358727397449,17.0879810712508));
#32969=CARTESIAN_POINT('Ctrl Pts',(0.651878180779539,4.53346824763866,17.1144383679353));
#32970=CARTESIAN_POINT('Ctrl Pts',(-0.0987540592508608,4.51705757827172,
17.1408956646198));
#32971=CARTESIAN_POINT('Ctrl Pts',(-0.849386299281262,4.50064690890479,
17.1673529613042));
#32972=CARTESIAN_POINT('Ctrl Pts',(-1.59583951925246,4.29308471998125,17.1938102579887));
#32973=CARTESIAN_POINT('Ctrl Pts',(-2.24719647092549,3.91965176135179,17.2202675546731));
#32974=CARTESIAN_POINT('Ctrl Pts',(-2.89855342259852,3.54621880272232,17.2467248513576));
#32975=CARTESIAN_POINT('Ctrl Pts',(-3.45481410597338,3.00691507438693,17.2731821480421));
#32976=CARTESIAN_POINT('Ctrl Pts',(-3.8482267217169,2.36742735305624,17.2996394447266));
#32977=CARTESIAN_POINT('Ctrl Pts',(-4.24163933746045,1.7279396317255,17.326096741411));
#32978=CARTESIAN_POINT('Ctrl Pts',(-4.47220388557264,0.988267917399458,
17.3525540380955));
#32979=CARTESIAN_POINT('Ctrl Pts',(-4.51183760195937,0.238503067401354,
17.37901133478));
#32980=CARTESIAN_POINT('Ctrl Pts',(-4.55147131834609,-0.511261782596708,
17.4054686314644));
#32981=CARTESIAN_POINT('Ctrl Pts',(-4.40017420300738,-1.27111976826683,
17.4319259281489));
#32982=CARTESIAN_POINT('Ctrl Pts',(-4.07637456299423,-1.94852038806902,
17.4583832248334));
#32983=CARTESIAN_POINT('Ctrl Pts',(-3.75257492298108,-2.62592100787122,
17.4848405215178));
#32984=CARTESIAN_POINT('Ctrl Pts',(-3.25627275829351,-3.22086426180549,
17.5112978182023));
#32985=CARTESIAN_POINT('Ctrl Pts',(-2.64791620593751,-3.66088792814038,
17.5377551148868));
#32986=CARTESIAN_POINT('Ctrl Pts',(-2.0395596535815,-4.10091159447528,17.5642124115712));
#32987=CARTESIAN_POINT('Ctrl Pts',(-1.31914871355708,-4.38601567321079,
17.5906697082557));
#32988=CARTESIAN_POINT('Ctrl Pts',(-0.574430373257593,-4.48147252184731,
17.6171270049402));
#32989=CARTESIAN_POINT('Ctrl Pts',(0.17028796704189,-4.57692937048383,17.6435843016246));
#32990=CARTESIAN_POINT('Ctrl Pts',(0.939313707616428,-4.48273898902136,
17.6700415983091));
#32991=CARTESIAN_POINT('Ctrl Pts',(1.63898363511409,-4.21037796912968,17.6964988949936));
#32992=CARTESIAN_POINT('Ctrl Pts',(2.33865356261174,-3.93801694923801,17.7229561916781));
#32993=CARTESIAN_POINT('Ctrl Pts',(2.96896767703252,-3.48748529091713,17.7494134883625));
#32994=CARTESIAN_POINT('Ctrl Pts',(3.45314824099611,-2.91364911818949,17.775870785047));
#32995=CARTESIAN_POINT('Ctrl Pts',(3.9373288049597,-2.33981294546184,17.8023280817315));
#32996=CARTESIAN_POINT('Ctrl Pts',(4.27537581846611,-1.64267225832742,17.8287853784159));
#32997=CARTESIAN_POINT('Ctrl Pts',(4.42612719062433,-0.907153378338104,
17.8552426751004));
#32998=CARTESIAN_POINT('Ctrl Pts',(4.48723544976425,-0.609004992176015,
17.8659673492363));
#32999=CARTESIAN_POINT('Ctrl Pts',(4.51756822102564,-0.304550492318464,
17.8766920233722));
#33000=CARTESIAN_POINT('Ctrl Pts',(4.51742050630483,-6.62530376704943E-5,
17.8874166975081));
#33001=CARTESIAN_POINT('Ctrl Pts',(4.51803700570725,7.32895604327322E-5,
17.612583302492));
#33002=CARTESIAN_POINT('Ctrl Pts',(4.5175164865615,-0.675330663287972,17.5887847689287));
#33003=CARTESIAN_POINT('Ctrl Pts',(4.36400868534142,-1.35096328729663,17.5649862353655));
#33004=CARTESIAN_POINT('Ctrl Pts',(4.07110679585739,-1.95950283641844,17.5411877018022));
#33005=CARTESIAN_POINT('Ctrl Pts',(3.74548201864491,-2.63602819259433,17.5147304051177));
#33006=CARTESIAN_POINT('Ctrl Pts',(3.24757722835295,-3.22963184123583,17.4882731084333));
#33007=CARTESIAN_POINT('Ctrl Pts',(2.63803679068424,-3.66801355240638,17.4618158117488));
#33008=CARTESIAN_POINT('Ctrl Pts',(2.02849635301557,-4.10639526357692,17.4353585150643));
#33009=CARTESIAN_POINT('Ctrl Pts',(1.30732026797015,-4.38955503727653,17.4089012183799));
#33010=CARTESIAN_POINT('Ctrl Pts',(0.562346924558562,-4.48300430658583,
17.3824439216954));
#33011=CARTESIAN_POINT('Ctrl Pts',(-0.182626418853022,-4.57645357589513,
17.3559866250109));
#33012=CARTESIAN_POINT('Ctrl Pts',(-0.95139702063077,-4.48019234081411,
17.3295293283265));
#33013=CARTESIAN_POINT('Ctrl Pts',(-1.65032944052442,-4.20594512376068,
17.303072031642));
#33014=CARTESIAN_POINT('Ctrl Pts',(-2.34926186041808,-3.93169790670724,
17.2766147349575));
#33015=CARTESIAN_POINT('Ctrl Pts',(-2.97835609842763,-3.47946470768139,
17.2501574382731));
#33016=CARTESIAN_POINT('Ctrl Pts',(-3.46098918943056,-2.90432702425224,
17.2237001415886));
#33017=CARTESIAN_POINT('Ctrl Pts',(-3.94362228043348,-2.32918934082309,
17.1972428449041));
#33018=CARTESIAN_POINT('Ctrl Pts',(-4.27979422442977,-1.63114717299066,
17.1707855482197));
#33019=CARTESIAN_POINT('Ctrl Pts',(-4.42855964178007,-0.895221287202602,
17.1443282515352));
#33020=CARTESIAN_POINT('Ctrl Pts',(-4.57732505913038,-0.159295401414506,
17.1178709548507));
#33021=CARTESIAN_POINT('Ctrl Pts',(-4.53868394983468,0.614514202329214,
17.0914136581662));
#33022=CARTESIAN_POINT('Ctrl Pts',(-4.31734276296002,1.33195837225454,17.0649563614818));
#33023=CARTESIAN_POINT('Ctrl Pts',(-4.09600157608536,2.04940254217985,17.0384990647973));
#33024=CARTESIAN_POINT('Ctrl Pts',(-3.69196031163174,2.71048127828677,17.0120417681128));
#33025=CARTESIAN_POINT('Ctrl Pts',(-3.15443074594472,3.23467592132634,16.9855844714284));
#33026=CARTESIAN_POINT('Ctrl Pts',(-2.61690118025774,3.75887056436587,16.9591271747439));
#33027=CARTESIAN_POINT('Ctrl Pts',(-1.94588331333737,4.14618111433807,16.9326698780594));
#33028=CARTESIAN_POINT('Ctrl Pts',(-1.223106380062,4.3494335753433,16.906212581375));
#33029=CARTESIAN_POINT('Ctrl Pts',(-0.500329446786581,4.55268603634855,
16.8797552846905));
#33030=CARTESIAN_POINT('Ctrl Pts',(0.274206552843852,4.57188040838682,16.853297988006));
#33031=CARTESIAN_POINT('Ctrl Pts',(1.00616399197863,4.40467883795473,16.8268406913216));
#33032=CARTESIAN_POINT('Ctrl Pts',(1.73812143111341,4.23747726752264,16.8003833946371));
#33033=CARTESIAN_POINT('Ctrl Pts',(2.42750030975254,3.88387975462018,16.7739260979526));
#33034=CARTESIAN_POINT('Ctrl Pts',(2.99033504306357,3.38695408510442,16.7474688012682));
#33035=CARTESIAN_POINT('Ctrl Pts',(3.55316977637459,2.89002841558867,16.7210115045837));
#33036=CARTESIAN_POINT('Ctrl Pts',(3.98946036435752,2.24977458945961,16.6945542078992));
#33037=CARTESIAN_POINT('Ctrl Pts',(4.24606709644911,1.54417481408576,16.6680969112148));
#33038=CARTESIAN_POINT('Ctrl Pts',(4.42554078305754,1.05067025197154,16.6495923749738));
#33039=CARTESIAN_POINT('Ctrl Pts',(4.51711737210933,0.525199995180907,16.6310878387329));
#33040=CARTESIAN_POINT('Ctrl Pts',(4.51759135405446,-0.000109312323752775,
16.612583302492));
#33041=CARTESIAN_POINT('Origin',(0.,0.,20.5));
#33042=CARTESIAN_POINT('',(4.51759608459634,0.0001098887360651,15.612583302492));
#33043=CARTESIAN_POINT('',(4.5178043285159,-0.000114763987914418,15.8874166975081));
#33044=CARTESIAN_POINT('',(4.51775,5.53264807684796E-16,20.5));
#33045=CARTESIAN_POINT('Ctrl Pts',(4.5178043285159,-0.000114763987914418,
15.8874166975081));
#33046=CARTESIAN_POINT('Ctrl Pts',(4.51719021324072,0.595015005655344,15.9083835696116));
#33047=CARTESIAN_POINT('Ctrl Pts',(4.39892963080694,1.19038158256103,15.9293504417152));
#33048=CARTESIAN_POINT('Ctrl Pts',(4.16984886166331,1.73951778234083,15.9503173138187));
#33049=CARTESIAN_POINT('Ctrl Pts',(3.88078057126651,2.43245182066608,15.9767746105032));
#33050=CARTESIAN_POINT('Ctrl Pts',(3.41525380642348,3.05177344176931,16.0032319071877));
#33051=CARTESIAN_POINT('Ctrl Pts',(2.82996921187389,3.52204995762958,16.0296892038721));
#33052=CARTESIAN_POINT('Ctrl Pts',(2.2446846173243,3.99232647348986,16.0561465005566));
#33053=CARTESIAN_POINT('Ctrl Pts',(1.53964219306814,4.3135578841072,16.082603797241));
#33054=CARTESIAN_POINT('Ctrl Pts',(0.800715326097207,4.44661855917225,16.1090610939255));
#33055=CARTESIAN_POINT('Ctrl Pts',(0.0617884591262693,4.57967923423731,
16.13551839061));
#33056=CARTESIAN_POINT('Ctrl Pts',(-0.711022850559448,4.52456917375008,
16.1619756872944));
#33057=CARTESIAN_POINT('Ctrl Pts',(-1.42359104075325,4.28800072211039,16.1884329839789));
#33058=CARTESIAN_POINT('Ctrl Pts',(-2.13615923094709,4.0514322704707,16.2148902806634));
#33059=CARTESIAN_POINT('Ctrl Pts',(-2.788484301649,3.63340542767853,16.2413475773478));
#33060=CARTESIAN_POINT('Ctrl Pts',(-3.30111378116087,3.08483540049633,16.2678048740323));
#33061=CARTESIAN_POINT('Ctrl Pts',(-3.81374326067272,2.53626537331417,16.2942621707168));
#33062=CARTESIAN_POINT('Ctrl Pts',(-4.18667714899455,1.857152161742,16.3207194674013));
#33063=CARTESIAN_POINT('Ctrl Pts',(-4.37449251133268,1.1302110034409,16.3471767640857));
#33064=CARTESIAN_POINT('Ctrl Pts',(-4.56230787367082,0.403269845139789,
16.3736340607702));
#33065=CARTESIAN_POINT('Ctrl Pts',(-4.56500471002526,-0.371499259890255,
16.4000913574546));
#33066=CARTESIAN_POINT('Ctrl Pts',(-4.38225454858744,-1.09973029228273,
16.4265486541391));
#33067=CARTESIAN_POINT('Ctrl Pts',(-4.19950438714961,-1.82796132467523,
16.4530059508236));
#33068=CARTESIAN_POINT('Ctrl Pts',(-3.8313072279195,-2.50965428443015,16.4794632475081));
#33069=CARTESIAN_POINT('Ctrl Pts',(-3.3225090776326,-3.06177972318871,16.5059205441925));
#33070=CARTESIAN_POINT('Ctrl Pts',(-2.81371092734571,-3.61390516194727,
16.532377840877));
#33071=CARTESIAN_POINT('Ctrl Pts',(-2.16431178600201,-4.03646307970946,
16.5588351375615));
#33072=CARTESIAN_POINT('Ctrl Pts',(-1.45340774986022,-4.27798639033812,
16.5852924342459));
#33073=CARTESIAN_POINT('Ctrl Pts',(-0.742503713718461,-4.51950970096678,
16.6117497309304));
#33074=CARTESIAN_POINT('Ctrl Pts',(0.0299052172213853,-4.5799984044619,
16.6382070276149));
#33075=CARTESIAN_POINT('Ctrl Pts',(0.769740489176569,-4.45208504257185,
16.6646643242993));
#33076=CARTESIAN_POINT('Ctrl Pts',(1.50957576113175,-4.32417168068181,16.6911216209838));
#33077=CARTESIAN_POINT('Ctrl Pts',(2.21683737410228,-4.00785625340658,16.7175789176683));
#33078=CARTESIAN_POINT('Ctrl Pts',(2.80538164796928,-3.54166563180933,16.7440362143527));
#33079=CARTESIAN_POINT('Ctrl Pts',(3.39392592183629,-3.07547501021207,16.7704935110372));
#33080=CARTESIAN_POINT('Ctrl Pts',(3.86375285659978,-2.45940919429276,16.7969508077217));
#33081=CARTESIAN_POINT('Ctrl Pts',(4.15763804857084,-1.76850431465121,16.8234081044061));
#33082=CARTESIAN_POINT('Ctrl Pts',(4.39463854911208,-1.21133162689784,16.8447443021068));
#33083=CARTESIAN_POINT('Ctrl Pts',(4.51721639786597,-0.605487805208481,
16.8660804998074));
#33084=CARTESIAN_POINT('Ctrl Pts',(4.51783748975292,0.000112199089269072,
16.8874166975081));
#33085=CARTESIAN_POINT('Ctrl Pts',(4.51759135405446,-0.000109312323752775,
16.612583302492));
#33086=CARTESIAN_POINT('Ctrl Pts',(4.51779505896309,-0.225873364281351,
16.6046305420484));
#33087=CARTESIAN_POINT('Ctrl Pts',(4.50117162820754,-0.451607688050524,
16.5966777816049));
#33088=CARTESIAN_POINT('Ctrl Pts',(4.46746660375751,-0.674762023706868,
16.5887250211614));
#33089=CARTESIAN_POINT('Ctrl Pts',(4.35533650277404,-1.417153361507,16.5622677244769));
#33090=CARTESIAN_POINT('Ctrl Pts',(4.05415342460685,-2.1309903124886,16.5358104277924));
#33091=CARTESIAN_POINT('Ctrl Pts',(3.60060113490314,-2.72932832606603,16.509353131108));
#33092=CARTESIAN_POINT('Ctrl Pts',(3.14704884519943,-3.32766633964346,16.4828958344235));
#33093=CARTESIAN_POINT('Ctrl Pts',(2.54112734395919,-3.81050541581671,16.456438537739));
#33094=CARTESIAN_POINT('Ctrl Pts',(1.85663719941204,-4.1190362894713,16.4299812410546));
#33095=CARTESIAN_POINT('Ctrl Pts',(1.17214705486486,-4.4275671631259,16.4035239443701));
#33096=CARTESIAN_POINT('Ctrl Pts',(0.409088267010757,-4.56178983426182,
16.3770666476856));
#33097=CARTESIAN_POINT('Ctrl Pts',(-0.33959944827516,-4.50535613008826,
16.3506093510012));
#33098=CARTESIAN_POINT('Ctrl Pts',(-1.08828716356108,-4.4489224259147,16.3241520543167));
#33099=CARTESIAN_POINT('Ctrl Pts',(-1.82260380627881,-4.20183234643166,
16.2976947576322));
#33100=CARTESIAN_POINT('Ctrl Pts',(-2.45311042204468,-3.79418118985514,
16.2712374609477));
#33101=CARTESIAN_POINT('Ctrl Pts',(-3.08361703781053,-3.38653003327864,
16.2447801642633));
#33102=CARTESIAN_POINT('Ctrl Pts',(-3.61031362662454,-2.81831779960867,
16.2183228675788));
#33103=CARTESIAN_POINT('Ctrl Pts',(-3.96904912687637,-2.15875211004946,
16.1918655708943));
#33104=CARTESIAN_POINT('Ctrl Pts',(-4.3277846271282,-1.49918642049025,16.1654082742099));
#33105=CARTESIAN_POINT('Ctrl Pts',(-4.51855903881786,-0.748267275041791,
16.1389509775254));
#33106=CARTESIAN_POINT('Ctrl Pts',(-4.51813624973985,0.00254420544672257,
16.1124936808409));
#33107=CARTESIAN_POINT('Ctrl Pts',(-4.51771346066184,0.753355685935258,
16.0860363841565));
#33108=CARTESIAN_POINT('Ctrl Pts',(-4.32609347081614,1.50405950146385,16.059579087472));
#33109=CARTESIAN_POINT('Ctrl Pts',(-3.96661538289292,2.16322075812806,16.0331217907875));
#33110=CARTESIAN_POINT('Ctrl Pts',(-3.6071372949697,2.82238201479228,16.0066644941031));
#33111=CARTESIAN_POINT('Ctrl Pts',(-3.07980110896895,3.39000071259211,15.9802071974186));
#33112=CARTESIAN_POINT('Ctrl Pts',(-2.4488357887268,3.7969415223371,15.9537499007341));
#33113=CARTESIAN_POINT('Ctrl Pts',(-1.81787046848466,4.20388233208208,15.9272926040497));
#33114=CARTESIAN_POINT('Ctrl Pts',(-1.08327601400112,4.45014525377221,15.9008353073652));
#33115=CARTESIAN_POINT('Ctrl Pts',(-0.334525216833305,4.50573573609241,
15.8743780106807));
#33116=CARTESIAN_POINT('Ctrl Pts',(0.41422558033451,4.5613262184126,15.8479207139963));
#33117=CARTESIAN_POINT('Ctrl Pts',(1.1771327201866,4.42624426136285,15.8214634173118));
#33118=CARTESIAN_POINT('Ctrl Pts',(1.86127495742196,4.11694269781245,15.7950061206273));
#33119=CARTESIAN_POINT('Ctrl Pts',(2.54541719465734,3.80764113426205,15.7685488239429));
#33120=CARTESIAN_POINT('Ctrl Pts',(3.15079452927597,3.32411996421099,15.7420915272584));
#33121=CARTESIAN_POINT('Ctrl Pts',(3.60367267191142,2.72527153104349,15.7156342305739));
#33122=CARTESIAN_POINT('Ctrl Pts',(4.05655081454687,2.12642309787598,15.6891769338895));
#33123=CARTESIAN_POINT('Ctrl Pts',(4.35692976519912,1.41224740159204,15.662719637205));
#33124=CARTESIAN_POINT('Ctrl Pts',(4.46822370011744,0.669730251598505,15.6362623405205));
#33125=CARTESIAN_POINT('Ctrl Pts',(4.50142605066627,0.448214903788299,15.6283693278443));
#33126=CARTESIAN_POINT('Ctrl Pts',(4.51779965427679,0.224177139537577,15.6204763151682));
#33127=CARTESIAN_POINT('Ctrl Pts',(4.51759608459634,0.0001098887360651,
15.612583302492));
#33128=CARTESIAN_POINT('Origin',(0.,0.,20.5));
#33129=CARTESIAN_POINT('',(4.51803303654689,-7.46219232266102E-5,14.612583302492));
#33130=CARTESIAN_POINT('',(4.51743493951217,7.09613961932946E-5,14.8874166975081));
#33131=CARTESIAN_POINT('',(4.51775,5.53264807684796E-16,20.5));
#33132=CARTESIAN_POINT('Ctrl Pts',(4.51743493951217,7.09613961932946E-5,
14.8874166975081));
#33133=CARTESIAN_POINT('Ctrl Pts',(4.51759894908653,0.294069189408427,14.8977720460469));
#33134=CARTESIAN_POINT('Ctrl Pts',(4.48933542297813,0.588036293354993,14.9081273945857));
#33135=CARTESIAN_POINT('Ctrl Pts',(4.43233806206614,0.876322399438229,14.9184827431245));
#33136=CARTESIAN_POINT('Ctrl Pts',(4.2867132110791,1.61287617260017,14.9449400398089));
#33137=CARTESIAN_POINT('Ctrl Pts',(3.95352194255086,2.31234598448206,14.9713973364934));
#33138=CARTESIAN_POINT('Ctrl Pts',(3.47334658423498,2.88953718612178,14.9978546331779));
#33139=CARTESIAN_POINT('Ctrl Pts',(2.99317122591908,3.46672838776151,15.0243119298623));
#33140=CARTESIAN_POINT('Ctrl Pts',(2.36601177781554,3.92164097915906,15.0507692265468));
#33141=CARTESIAN_POINT('Ctrl Pts',(1.6682555666064,4.19886711014818,15.0772265232313));
#33142=CARTESIAN_POINT('Ctrl Pts',(0.97049935539727,4.4760932411373,15.1036838199157));
#33143=CARTESIAN_POINT('Ctrl Pts',(0.20214638108255,4.57563291171798,15.1301411166002));
#33144=CARTESIAN_POINT('Ctrl Pts',(-0.543218814426446,4.48536230017716,
15.1565984132847));
#33145=CARTESIAN_POINT('Ctrl Pts',(-1.28858400993542,4.39509168863634,15.1830557099691));
#33146=CARTESIAN_POINT('Ctrl Pts',(-2.01096142663867,4.11501079497402,15.2095130066536));
#33147=CARTESIAN_POINT('Ctrl Pts',(-2.6223662946594,3.67923316206403,15.2359703033381));
#33148=CARTESIAN_POINT('Ctrl Pts',(-3.23377116268013,3.24345552915403,15.2624276000225));
#33149=CARTESIAN_POINT('Ctrl Pts',(-3.73420348201834,2.65198115699635,15.288884896707));
#33150=CARTESIAN_POINT('Ctrl Pts',(-4.06271115002269,1.9768509695166,15.3153421933915));
#33151=CARTESIAN_POINT('Ctrl Pts',(-4.39121881802704,1.30172078203686,15.3417994900759));
#33152=CARTESIAN_POINT('Ctrl Pts',(-4.54780183469754,0.542934779235054,
15.3682567867604));
#33153=CARTESIAN_POINT('Ctrl Pts',(-4.51338856189906,-0.207087743519677,
15.3947140834449));
#33154=CARTESIAN_POINT('Ctrl Pts',(-4.47897528910057,-0.957110266274451,
15.4211713801293));
#33155=CARTESIAN_POINT('Ctrl Pts',(-4.2535657268331,-1.69836930898215,15.4476286768138));
#33156=CARTESIAN_POINT('Ctrl Pts',(-3.86461451031294,-2.34058034061557,
15.4740859734983));
#33157=CARTESIAN_POINT('Ctrl Pts',(-3.4756632937928,-2.98279137224897,15.5005432701827));
#33158=CARTESIAN_POINT('Ctrl Pts',(-2.92317042302,-3.5259543928081,15.5270005668672));
#33159=CARTESIAN_POINT('Ctrl Pts',(-2.27442891819367,-3.9039127475242,15.5534578635517));
#33160=CARTESIAN_POINT('Ctrl Pts',(-1.62568741336734,-4.28187110224029,
15.5799151602362));
#33161=CARTESIAN_POINT('Ctrl Pts',(-0.880697274487477,-4.49462479111335,
15.6063724569206));
#33162=CARTESIAN_POINT('Ctrl Pts',(-0.130197475965578,-4.51626065030008,
15.6328297536051));
#33163=CARTESIAN_POINT('Ctrl Pts',(0.620302322556342,-4.53789650948681,
15.6592870502896));
#33164=CARTESIAN_POINT('Ctrl Pts',(1.3763117807203,-4.3684145389872,15.685744346974));
#33165=CARTESIAN_POINT('Ctrl Pts',(2.04574978322079,-4.02845745523656,15.7122016436585));
#33166=CARTESIAN_POINT('Ctrl Pts',(2.71518778572125,-3.68850037148593,15.738658940343));
#33167=CARTESIAN_POINT('Ctrl Pts',(3.29805433255825,-3.17806817448428,15.7651162370274));
#33168=CARTESIAN_POINT('Ctrl Pts',(3.72335692340443,-2.55933094091619,15.7915735337119));
#33169=CARTESIAN_POINT('Ctrl Pts',(4.14865951425061,-1.94059370734809,15.8180308303964));
#33170=CARTESIAN_POINT('Ctrl Pts',(4.41639814910596,-1.21355143721353,15.8444881270808));
#33171=CARTESIAN_POINT('Ctrl Pts',(4.49396255855834,-0.466757074372606,
15.8709454237653));
#33172=CARTESIAN_POINT('Ctrl Pts',(4.51005874349141,-0.311782128309925,
15.8764358483462));
#33173=CARTESIAN_POINT('Ctrl Pts',(4.51796514189739,-0.155956565280692,
15.8819262729272));
#33174=CARTESIAN_POINT('Ctrl Pts',(4.5178043285159,-0.000114763987914418,
15.8874166975081));
#33175=CARTESIAN_POINT('Ctrl Pts',(4.51759608459634,0.0001098887360651,
15.612583302492));
#33176=CARTESIAN_POINT('Ctrl Pts',(4.5171172908178,-0.526893962833933,15.5940190184837));
#33177=CARTESIAN_POINT('Ctrl Pts',(4.42493597400368,-1.05406092973462,15.5754547344754));
#33178=CARTESIAN_POINT('Ctrl Pts',(4.24432532522022,-1.54895583471304,15.5568904504671));
#33179=CARTESIAN_POINT('Ctrl Pts',(3.98692409622027,-2.25426616732798,15.5304331537826));
#33180=CARTESIAN_POINT('Ctrl Pts',(3.54991271903595,-2.89402822885477,15.5039758570982));
#33181=CARTESIAN_POINT('Ctrl Pts',(2.98651869575415,-3.39031970824409,15.4775185604137));
#33182=CARTESIAN_POINT('Ctrl Pts',(2.42312467247236,-3.88661118763341,15.4510612637292));
#33183=CARTESIAN_POINT('Ctrl Pts',(1.73334800309309,-4.23943208488526,15.4246039670448));
#33184=CARTESIAN_POINT('Ctrl Pts',(1.00120272254938,-4.40580920519228,15.3981466703603));
#33185=CARTESIAN_POINT('Ctrl Pts',(0.269057442005672,-4.5721863254993,15.3716893736758));
#33186=CARTESIAN_POINT('Ctrl Pts',(-0.505456449702493,-4.55211966886149,
15.3452320769914));
#33187=CARTESIAN_POINT('Ctrl Pts',(-1.22800401774377,-4.34805333184893,
15.3187747803069));
#33188=CARTESIAN_POINT('Ctrl Pts',(-1.95055158578508,-4.14398699483636,
15.2923174836224));
#33189=CARTESIAN_POINT('Ctrl Pts',(-2.62113283015951,-3.75592097744901,
15.265860186938));
#33190=CARTESIAN_POINT('Ctrl Pts',(-3.15807169745543,-3.23112129111991,
15.2394028902535));
#33191=CARTESIAN_POINT('Ctrl Pts',(-3.69501056475133,-2.70632160479082,
15.212945593569));
#33192=CARTESIAN_POINT('Ctrl Pts',(-4.09830705496871,-2.04478824952003,
15.1864882968846));
#33193=CARTESIAN_POINT('Ctrl Pts',(-4.31884010193997,-1.3270952558398,15.1600310002001));
#33194=CARTESIAN_POINT('Ctrl Pts',(-4.53937314891122,-0.609402262159613,
15.1335737035156));
#33195=CARTESIAN_POINT('Ctrl Pts',(-4.57714275263633,0.164450369930026,
15.1071164068312));
#33196=CARTESIAN_POINT('Ctrl Pts',(-4.42754861718238,0.90020824628735,15.0806591101467));
#33197=CARTESIAN_POINT('Ctrl Pts',(-4.27795448172842,1.63596612264472,15.0542018134622));
#33198=CARTESIAN_POINT('Ctrl Pts',(-3.94099660709542,2.33362924326977,15.0277445167778));
#33199=CARTESIAN_POINT('Ctrl Pts',(-3.45771608949183,2.90822301219606,15.0012872200933));
#33200=CARTESIAN_POINT('Ctrl Pts',(-2.97443557188824,3.48281678112233,14.9748299234088));
#33201=CARTESIAN_POINT('Ctrl Pts',(-2.34483241131409,3.93434119834979,14.9483726267244));
#33202=CARTESIAN_POINT('Ctrl Pts',(-1.64559157592583,4.20780108957628,14.9219153300399));
#33203=CARTESIAN_POINT('Ctrl Pts',(-0.946350740537523,4.4812609808028,14.8954580333554));
#33204=CARTESIAN_POINT('Ctrl Pts',(-0.17747223033509,4.57665634602833,14.8690007366709));
#33205=CARTESIAN_POINT('Ctrl Pts',(0.567395403080653,4.48236813534546,14.8425434399865));
#33206=CARTESIAN_POINT('Ctrl Pts',(1.31226303649637,4.38807992466259,14.816086143302));
#33207=CARTESIAN_POINT('Ctrl Pts',(2.03311979312542,4.10410813807131,14.7896288466175));
#33208=CARTESIAN_POINT('Ctrl Pts',(2.64216611780504,3.665040224898,14.7631715499331));
#33209=CARTESIAN_POINT('Ctrl Pts',(3.25121244248463,3.22597231172472,14.7367142532486));
#33210=CARTESIAN_POINT('Ctrl Pts',(3.74844833521482,2.63180827196943,14.7102569565641));
#33211=CARTESIAN_POINT('Ctrl Pts',(4.07331101456755,1.95491662809442,14.6837996598797));
#33212=CARTESIAN_POINT('Ctrl Pts',(4.36479376317213,1.347576205805,14.6600608740838));
#33213=CARTESIAN_POINT('Ctrl Pts',(4.51750642932664,0.673635432917883,14.6363220882879));
#33214=CARTESIAN_POINT('Ctrl Pts',(4.51803303654689,-7.46219232266102E-5,
14.612583302492));
#33215=CARTESIAN_POINT('Origin',(0.,0.,20.5));
#33216=CARTESIAN_POINT('',(4.51736301819297,2.68279993319077E-6,13.612583302492));
#33217=CARTESIAN_POINT('',(4.51813640225623,-7.72658854479727E-6,13.8874166975081));
#33218=CARTESIAN_POINT('',(4.51775,5.53264807684796E-16,20.5));
#33219=CARTESIAN_POINT('Ctrl Pts',(4.51813584929441,-7.71553139285741E-6,
13.8874166975081));
#33220=CARTESIAN_POINT('Ctrl Pts',(4.5180616865618,0.743534623094937,13.9136178191666));
#33221=CARTESIAN_POINT('Ctrl Pts',(4.33069406362294,1.48711296925487,13.9398189408251));
#33222=CARTESIAN_POINT('Ctrl Pts',(3.97822152575483,2.14180184335953,13.9660200624836));
#33223=CARTESIAN_POINT('Ctrl Pts',(3.62230277429653,2.80289177698769,13.9924773591681));
#33224=CARTESIAN_POINT('Ctrl Pts',(3.0980347793188,3.37334555127586,14.0189346558525));
#33225=CARTESIAN_POINT('Ctrl Pts',(2.46927280238618,3.78368252785474,14.045391952537));
#33226=CARTESIAN_POINT('Ctrl Pts',(1.84051082545358,4.19401950443362,14.0718492492215));
#33227=CARTESIAN_POINT('Ctrl Pts',(1.10725486656609,4.44423968330323,14.0983065459059));
#33228=CARTESIAN_POINT('Ctrl Pts',(0.358814689998941,4.50386652360373,14.1247638425904));
#33229=CARTESIAN_POINT('Ctrl Pts',(-0.389625486568206,4.56349336390423,
14.1512211392749));
#33230=CARTESIAN_POINT('Ctrl Pts',(-1.15324988081502,4.43252686563563,14.1776784359594));
#33231=CARTESIAN_POINT('Ctrl Pts',(-1.83904988664919,4.12691860334233,14.2041357326438));
#33232=CARTESIAN_POINT('Ctrl Pts',(-2.52484989248339,3.82131034104901,14.2305930293283));
#33233=CARTESIAN_POINT('Ctrl Pts',(-3.13282550990494,3.34106031473099,14.2570503260128));
#33234=CARTESIAN_POINT('Ctrl Pts',(-3.58892598157751,2.74466244608609,14.2835076226972));
#33235=CARTESIAN_POINT('Ctrl Pts',(-4.04502645325008,2.14826457744119,14.3099649193817));
#33236=CARTESIAN_POINT('Ctrl Pts',(-4.34925177917366,1.43571886646941,14.3364222160662));
#33237=CARTESIAN_POINT('Ctrl Pts',(-4.46454765134644,0.693812592170538,
14.3628795127506));
#33238=CARTESIAN_POINT('Ctrl Pts',(-4.57984352351921,-0.0480936821283345,
14.3893368094351));
#33239=CARTESIAN_POINT('Ctrl Pts',(-4.50620994194118,-0.819360519754252,
14.4157941061196));
#33240=CARTESIAN_POINT('Ctrl Pts',(-4.25261539535597,-1.52604847346958,
14.442251402804));
#33241=CARTESIAN_POINT('Ctrl Pts',(-3.99902084877075,-2.23273642718488,
14.4687086994885));
#33242=CARTESIAN_POINT('Ctrl Pts',(-3.56546533717836,-2.87484549698955,
14.495165996173));
#33243=CARTESIAN_POINT('Ctrl Pts',(-3.00475544206132,-3.37416750882351,
14.5216232928574));
#33244=CARTESIAN_POINT('Ctrl Pts',(-2.44404554694427,-3.87348952065748,
14.5480805895419));
#33245=CARTESIAN_POINT('Ctrl Pts',(-1.75618126830258,-4.23002447452076,
14.5745378862264));
#33246=CARTESIAN_POINT('Ctrl Pts',(-1.02494371399391,-4.40034680762116,
14.6009951829108));
#33247=CARTESIAN_POINT('Ctrl Pts',(-0.293706159685227,-4.57066914072157,
14.6274524795953));
#33248=CARTESIAN_POINT('Ctrl Pts',(0.480904670290444,-4.5547788530591,14.6539097762798));
#33249=CARTESIAN_POINT('Ctrl Pts',(1.20454203412804,-4.35461136408475,14.6803670729642));
#33250=CARTESIAN_POINT('Ctrl Pts',(1.92817939796561,-4.15444387511041,14.7068243696487));
#33251=CARTESIAN_POINT('Ctrl Pts',(2.60084329566512,-3.76999918482422,14.7332816663332));
#33252=CARTESIAN_POINT('Ctrl Pts',(3.14060400894491,-3.24810223102607,14.7597389630176));
#33253=CARTESIAN_POINT('Ctrl Pts',(3.68036472222471,-2.72620527722791,14.7861962597021));
#33254=CARTESIAN_POINT('Ctrl Pts',(4.08722225108478,-2.0668560599178,14.8126535563866));
#33255=CARTESIAN_POINT('Ctrl Pts',(4.3116217987919,-1.35036258404174,14.839110853071));
#33256=CARTESIAN_POINT('Ctrl Pts',(4.44819168059748,-0.91430364223594,14.8552128012167));
#33257=CARTESIAN_POINT('Ctrl Pts',(4.51717991442519,-0.457078713927616,
14.8713147493624));
#33258=CARTESIAN_POINT('Ctrl Pts',(4.51743493951217,7.09613961932946E-5,
14.8874166975081));
#33259=CARTESIAN_POINT('Ctrl Pts',(4.51803303654689,-7.46219232266102E-5,
14.612583302492));
#33260=CARTESIAN_POINT('Ctrl Pts',(4.51809334238876,-0.0772263404472327,
14.6098647916034));
#33261=CARTESIAN_POINT('Ctrl Pts',(4.51615783443211,-0.154375033265316,
14.6071462807148));
#33262=CARTESIAN_POINT('Ctrl Pts',(4.51220636430248,-0.231420332178498,
14.6044277698263));
#33263=CARTESIAN_POINT('Ctrl Pts',(4.47374956870936,-0.981246400581585,
14.5779704731418));
#33264=CARTESIAN_POINT('Ctrl Pts',(4.24434651154784,-1.72127928939297,14.5515131764573));
#33265=CARTESIAN_POINT('Ctrl Pts',(3.85193823129266,-2.36138381177295,14.5250558797729));
#33266=CARTESIAN_POINT('Ctrl Pts',(3.4595299510375,-3.0014883341529,14.4985985830884));
#33267=CARTESIAN_POINT('Ctrl Pts',(2.90411644768869,-3.54166449010144,14.4721412864039));
#33268=CARTESIAN_POINT('Ctrl Pts',(2.25334647126064,-3.91611942165386,14.4456839897195));
#33269=CARTESIAN_POINT('Ctrl Pts',(1.60257649483259,-4.29057435320629,14.419226693035));
#33270=CARTESIAN_POINT('Ctrl Pts',(0.856450045325319,-4.49930806036259,
14.3927693963505));
#33271=CARTESIAN_POINT('Ctrl Pts',(0.10584449852735,-4.51689700860324,14.3663120996661));
#33272=CARTESIAN_POINT('Ctrl Pts',(-0.644761048270598,-4.53448595684389,
14.3398548029816));
#33273=CARTESIAN_POINT('Ctrl Pts',(-1.39984569235923,-4.36093014616891,
14.3133975062971));
#33274=CARTESIAN_POINT('Ctrl Pts',(-2.06744095976432,-4.01736848223886,
14.2869402096127));
#33275=CARTESIAN_POINT('Ctrl Pts',(-2.73503622716945,-3.67380681830879,
14.2604829129282));
#33276=CARTESIAN_POINT('Ctrl Pts',(-3.31514211789102,-3.16023930112366,
14.2340256162437));
#33277=CARTESIAN_POINT('Ctrl Pts',(-3.73710237646046,-2.53921788589538,
14.2075683195593));
#33278=CARTESIAN_POINT('Ctrl Pts',(-4.15906263502989,-1.91819647066709,
14.1811110228748));
#33279=CARTESIAN_POINT('Ctrl Pts',(-4.42287726144721,-1.18972115739562,
14.1546537261903));
#33280=CARTESIAN_POINT('Ctrl Pts',(-4.49641392618661,-0.442519433011148,
14.1281964295058));
#33281=CARTESIAN_POINT('Ctrl Pts',(-4.56995059092601,0.3046822913733,14.1017391328214));
#33282=CARTESIAN_POINT('Ctrl Pts',(-4.45320929398754,1.07061042687079,14.0752818361369));
#33283=CARTESIAN_POINT('Ctrl Pts',(-4.16040899613706,1.76197577425433,14.0488245394525));
#33284=CARTESIAN_POINT('Ctrl Pts',(-3.86760869828659,2.45334112163787,14.022367242768));
#33285=CARTESIAN_POINT('Ctrl Pts',(-3.39874939952411,3.07014368090745,13.9959099460835));
#33286=CARTESIAN_POINT('Ctrl Pts',(-2.81093764353767,3.53725758297869,13.969452649399));
#33287=CARTESIAN_POINT('Ctrl Pts',(-2.22312588755121,4.00437148504995,13.9429953527146));
#33288=CARTESIAN_POINT('Ctrl Pts',(-1.51636167434084,4.32179672992284,13.9165380560301));
#33289=CARTESIAN_POINT('Ctrl Pts',(-0.776728102877452,4.45087127407632,
13.8900807593456));
#33290=CARTESIAN_POINT('Ctrl Pts',(-0.0370945314140622,4.5799458182298,
13.8636234626612));
#33291=CARTESIAN_POINT('Ctrl Pts',(0.735408398302354,4.52066966166384,13.8371661659767));
#33292=CARTESIAN_POINT('Ctrl Pts',(1.44669068438533,4.2802625746454,13.8107088692922));
#33293=CARTESIAN_POINT('Ctrl Pts',(2.15797297046829,4.03985548762697,13.7842515726078));
#33294=CARTESIAN_POINT('Ctrl Pts',(2.80803461291788,3.61831747015607,13.7577942759233));
#33295=CARTESIAN_POINT('Ctrl Pts',(3.31769882312725,3.06699138623137,13.7313369792388));
#33296=CARTESIAN_POINT('Ctrl Pts',(3.82736303333661,2.51566530230669,13.7048796825544));
#33297=CARTESIAN_POINT('Ctrl Pts',(4.19662981130577,1.83455115192822,13.6784223858699));
#33298=CARTESIAN_POINT('Ctrl Pts',(4.38052287215716,1.10660788480175,13.6519650891854));
#33299=CARTESIAN_POINT('Ctrl Pts',(4.47176471220886,0.745425777992701,13.6388378269543));
#33300=CARTESIAN_POINT('Ctrl Pts',(4.5173707651647,0.372715156596874,13.6257105647231));
#33301=CARTESIAN_POINT('Ctrl Pts',(4.51736305946108,2.68251383689355E-6,
13.612583302492));
#33302=CARTESIAN_POINT('Origin',(0.,0.,20.5));
#33303=CARTESIAN_POINT('',(4.51804648040592,6.99590604930078E-5,12.612583302492));
#33304=CARTESIAN_POINT('',(4.51741195309898,-5.96473381690886E-5,12.8874166975081));
#33305=CARTESIAN_POINT('',(4.51775,5.53264807684796E-16,20.5));
#33306=CARTESIAN_POINT('Ctrl Pts',(4.51741195309898,-5.96473381690886E-5,
12.8874166975081));
#33307=CARTESIAN_POINT('Ctrl Pts',(4.51720574953279,0.442550368129689,12.9030062956018));
#33308=CARTESIAN_POINT('Ctrl Pts',(4.45260272288938,0.885219283315433,12.9185958936956));
#33309=CARTESIAN_POINT('Ctrl Pts',(4.32446175047221,1.30866046509405,12.9341854917894));
#33310=CARTESIAN_POINT('Ctrl Pts',(4.10699214642681,2.02728764889691,12.9606427884738));
#33311=CARTESIAN_POINT('Ctrl Pts',(3.70652120381657,2.69053531250561,12.9871000851583));
#33312=CARTESIAN_POINT('Ctrl Pts',(3.1718258402377,3.21762062452953,13.0135573818428));
#33313=CARTESIAN_POINT('Ctrl Pts',(2.63713047665883,3.74470593655345,13.0400146785272));
#33314=CARTESIAN_POINT('Ctrl Pts',(1.96821069211135,4.13562889699258,13.0664719752117));
#33315=CARTESIAN_POINT('Ctrl Pts',(1.24654017603871,4.34277552191208,13.0929292718962));
#33316=CARTESIAN_POINT('Ctrl Pts',(0.524869659966072,4.54992214683159,13.1193865685806));
#33317=CARTESIAN_POINT('Ctrl Pts',(-0.249551587631711,4.57329243623147,
13.1458438652651));
#33318=CARTESIAN_POINT('Ctrl Pts',(-0.98239991587342,4.41003991472745,13.1723011619496));
#33319=CARTESIAN_POINT('Ctrl Pts',(-1.71524824411517,4.24678739322342,13.198758458634));
#33320=CARTESIAN_POINT('Ctrl Pts',(-2.40652365300083,3.89691206081547,13.2252157553185));
#33321=CARTESIAN_POINT('Ctrl Pts',(-2.97202956278422,3.40302834577293,13.251673052003));
#33322=CARTESIAN_POINT('Ctrl Pts',(-3.53753547256757,2.90914463073042,13.2781303486874));
#33323=CARTESIAN_POINT('Ctrl Pts',(-3.97727188324865,2.27125253305334,13.3045876453719));
#33324=CARTESIAN_POINT('Ctrl Pts',(-4.23767938667653,1.56704660426365,13.3310449420564));
#33325=CARTESIAN_POINT('Ctrl Pts',(-4.49808689010441,0.862840675473956,
13.3575022387408));
#33326=CARTESIAN_POINT('Ctrl Pts',(-4.57916548627907,0.0923209155716644,
13.3839595354253));
#33327=CARTESIAN_POINT('Ctrl Pts',(-4.47103989191868,-0.650664221445422,
13.4104168321098));
#33328=CARTESIAN_POINT('Ctrl Pts',(-4.36291429755829,-1.39364935846249,
13.4368741287942));
#33329=CARTESIAN_POINT('Ctrl Pts',(-4.06558451266282,-2.1090998725944,13.4633314254787));
#33330=CARTESIAN_POINT('Ctrl Pts',(-3.61526497596841,-2.70987468303122,
13.4897887221632));
#33331=CARTESIAN_POINT('Ctrl Pts',(-3.16494543927398,-3.31064949346807,
13.5162460188477));
#33332=CARTESIAN_POINT('Ctrl Pts',(-2.56163615078063,-3.79674860020983,
13.5427033155321));
#33333=CARTESIAN_POINT('Ctrl Pts',(-1.87881951412554,-4.10896567003649,
13.5691606122166));
#33334=CARTESIAN_POINT('Ctrl Pts',(-1.19600287747047,-4.42118273986315,
13.5956179089011));
#33335=CARTESIAN_POINT('Ctrl Pts',(-0.43367889265364,-4.55951777277468,
13.6220752055855));
#33336=CARTESIAN_POINT('Ctrl Pts',(0.315302222661903,-4.50712171486214,
13.64853250227));
#33337=CARTESIAN_POINT('Ctrl Pts',(1.06428333797747,-4.4547256569496,13.6749897989545));
#33338=CARTESIAN_POINT('Ctrl Pts',(1.7999215837918,-4.211598508213,13.7014470956389));
#33339=CARTESIAN_POINT('Ctrl Pts',(2.43261703591854,-3.80735288629203,13.7279043923234));
#33340=CARTESIAN_POINT('Ctrl Pts',(3.06531248804526,-3.40310726437108,13.7543616890079));
#33341=CARTESIAN_POINT('Ctrl Pts',(3.59506514648438,-2.8377431692658,13.7808189856923));
#33342=CARTESIAN_POINT('Ctrl Pts',(3.95735172373184,-2.18012132205388,13.8072762823768));
#33343=CARTESIAN_POINT('Ctrl Pts',(4.3196383009793,-1.52249947484199,13.8337335790613));
#33344=CARTESIAN_POINT('Ctrl Pts',(4.51445879703509,-0.772619875523486,
13.8601908757457));
#33345=CARTESIAN_POINT('Ctrl Pts',(4.51808429109356,-0.0218170293801791,
13.8866481724302));
#33346=CARTESIAN_POINT('Ctrl Pts',(4.51811939524822,-0.0145473169490636,
13.8869043474562));
#33347=CARTESIAN_POINT('Ctrl Pts',(4.5181365744023,-0.0072775179612929,
13.8871605224821));
#33348=CARTESIAN_POINT('Ctrl Pts',(4.51813584929441,-7.71553139285741E-6,
13.8874166975081));
#33349=CARTESIAN_POINT('Ctrl Pts',(4.51736305946108,2.68251383689355E-6,
13.612583302492));
#33350=CARTESIAN_POINT('Ctrl Pts',(4.51735523473014,-0.378466950622669,
13.5992532680387));
#33351=CARTESIAN_POINT('Ctrl Pts',(4.47031360843327,-0.756938494124053,
13.5859232335853));
#33352=CARTESIAN_POINT('Ctrl Pts',(4.37626124565255,-1.12334284793068,13.572593199132));
#33353=CARTESIAN_POINT('Ctrl Pts',(4.18958721456293,-1.85057792966208,13.5461359024476));
#33354=CARTESIAN_POINT('Ctrl Pts',(3.81771980865007,-2.53027570925035,13.5196786057631));
#33355=CARTESIAN_POINT('Ctrl Pts',(3.3059520663969,-3.07964974938441,13.4932213090786));
#33356=CARTESIAN_POINT('Ctrl Pts',(2.79418432414376,-3.62902378951843,13.4667640123941));
#33357=CARTESIAN_POINT('Ctrl Pts',(2.14251624555032,-4.04807409019825,13.4403067157097));
#33358=CARTESIAN_POINT('Ctrl Pts',(1.43032028136785,-4.28576078857712,13.4138494190252));
#33359=CARTESIAN_POINT('Ctrl Pts',(0.718124317185353,-4.523447486956,13.3873921223408));
#33360=CARTESIAN_POINT('Ctrl Pts',(-0.0545995325861841,-4.57977058303392,
13.3609348256563));
#33361=CARTESIAN_POINT('Ctrl Pts',(-0.793734358242206,-4.44786998604312,
13.3344775289718));
#33362=CARTESIAN_POINT('Ctrl Pts',(-1.53286918389827,-4.31596938905231,
13.3080202322873));
#33363=CARTESIAN_POINT('Ctrl Pts',(-2.23841498543881,-3.99584509899276,
13.2815629356029));
#33364=CARTESIAN_POINT('Ctrl Pts',(-2.82443706508576,-3.52648790010218,
13.2551056389184));
#33365=CARTESIAN_POINT('Ctrl Pts',(-3.41045914473268,-3.05713070121163,
13.2286483422339));
#33366=CARTESIAN_POINT('Ctrl Pts',(-3.87695750248602,-2.43854059349005,
13.2021910455495));
#33367=CARTESIAN_POINT('Ctrl Pts',(-4.16711315465972,-1.74606116744496,
13.175733748865));
#33368=CARTESIAN_POINT('Ctrl Pts',(-4.45726880683343,-1.05358174139987,
13.1492764521805));
#33369=CARTESIAN_POINT('Ctrl Pts',(-4.57108175342749,-0.287212997031258,
13.1228191554961));
#33370=CARTESIAN_POINT('Ctrl Pts',(-4.49468970350711,0.459702200761001,
13.0963618588116));
#33371=CARTESIAN_POINT('Ctrl Pts',(-4.41829765358673,1.20661739855328,13.0699045621271));
#33372=CARTESIAN_POINT('Ctrl Pts',(-4.15170060715189,1.93407904976921,13.0434472654427));
#33373=CARTESIAN_POINT('Ctrl Pts',(-3.72736978940707,2.5534831303952,13.0169899687582));
#33374=CARTESIAN_POINT('Ctrl Pts',(-3.30303897166226,3.1728872110212,12.9905326720737));
#33375=CARTESIAN_POINT('Ctrl Pts',(-2.72097438260746,3.68423372105726,12.9640753753893));
#33376=CARTESIAN_POINT('Ctrl Pts',(-2.05207084500052,4.02524122150415,12.9376180787048));
#33377=CARTESIAN_POINT('Ctrl Pts',(-1.3831673073936,4.36624872195103,12.9111607820203));
#33378=CARTESIAN_POINT('Ctrl Pts',(-0.627424821234523,4.53691721280875,
12.8847034853359));
#33379=CARTESIAN_POINT('Ctrl Pts',(0.123108015066336,4.51645946077498,12.8582461886514));
#33380=CARTESIAN_POINT('Ctrl Pts',(0.873640851367194,4.49600170874121,12.8317888919669));
#33381=CARTESIAN_POINT('Ctrl Pts',(1.61896403780984,4.28441771381596,12.8053315952824));
#33382=CARTESIAN_POINT('Ctrl Pts',(2.268298035158,3.9074781724145,12.778874298598));
#33383=CARTESIAN_POINT('Ctrl Pts',(2.91763203250619,3.53053863101303,12.7524170019135));
#33384=CARTESIAN_POINT('Ctrl Pts',(3.47097684075988,2.98824354313534,12.7259597052291));
#33385=CARTESIAN_POINT('Ctrl Pts',(3.86093567467777,2.34664385031004,12.6995024085446));
#33386=CARTESIAN_POINT('Ctrl Pts',(4.25089450859566,1.70504415748472,12.6730451118601));
#33387=CARTESIAN_POINT('Ctrl Pts',(4.47746736817774,0.964139859711776,12.6465878151756));
#33388=CARTESIAN_POINT('Ctrl Pts',(4.51305792988216,0.214172280478037,12.6201305184912));
#33389=CARTESIAN_POINT('Ctrl Pts',(4.51644212114351,0.142860291950876,12.6176147798248));
#33390=CARTESIAN_POINT('Ctrl Pts',(4.51809954743677,0.0714663578345357,
12.6150990411584));
#33391=CARTESIAN_POINT('Ctrl Pts',(4.51804648040592,6.99590604930078E-5,
12.612583302492));
#33392=CARTESIAN_POINT('Origin',(0.,0.,20.5));
#33393=CARTESIAN_POINT('',(4.5175801641472,-0.000107849321499542,11.612583302492));
#33394=CARTESIAN_POINT('',(4.5178502562812,0.000110962492481057,11.8874166975081));
#33395=CARTESIAN_POINT('',(4.51775,5.53264807684796E-16,20.5));
#33396=CARTESIAN_POINT('Ctrl Pts',(4.5178502562812,0.000110962492481057,
11.8874166975081));
#33397=CARTESIAN_POINT('Ctrl Pts',(4.51799453028332,0.141405931765494,11.8923947720371));
#33398=CARTESIAN_POINT('Ctrl Pts',(4.51149711848843,0.282687684813822,11.8973728465661));
#33399=CARTESIAN_POINT('Ctrl Pts',(4.49826065670895,0.423335220010937,11.9023509210951));
#33400=CARTESIAN_POINT('Ctrl Pts',(4.42791197182862,1.17084382900464,11.9288082177796));
#33401=CARTESIAN_POINT('Ctrl Pts',(4.16720717585505,1.90043785893767,11.955265514464));
#33402=CARTESIAN_POINT('Ctrl Pts',(3.7478998244077,2.5232535644287,11.9817228111485));
#33403=CARTESIAN_POINT('Ctrl Pts',(3.32859247296032,3.14606926991974,12.008180107833));
#33404=CARTESIAN_POINT('Ctrl Pts',(2.75068256603915,3.66210665096878,12.0346374045175));
#33405=CARTESIAN_POINT('Ctrl Pts',(2.08455889071624,4.00851292567871,12.0610947012019));
#33406=CARTESIAN_POINT('Ctrl Pts',(1.41843521539332,4.35491920038864,12.0875519978864));
#33407=CARTESIAN_POINT('Ctrl Pts',(0.664097771668666,4.53169436875946,12.1140092945709));
#33408=CARTESIAN_POINT('Ctrl Pts',(-0.0865759746608722,4.51730741092621,
12.1404665912553));
#33409=CARTESIAN_POINT('Ctrl Pts',(-0.83724972099039,4.50292045309296,12.1669238879398));
#33410=CARTESIAN_POINT('Ctrl Pts',(-1.58425976992479,4.29737136905566,12.1933811846243));
#33411=CARTESIAN_POINT('Ctrl Pts',(-2.23662112424321,3.92569580976245,12.2198384813087));
#33412=CARTESIAN_POINT('Ctrl Pts',(-2.88898247856163,3.55402025046923,12.2462957779932));
#33413=CARTESIAN_POINT('Ctrl Pts',(-3.44669513826407,3.01621821592011,12.2727530746777));
#33414=CARTESIAN_POINT('Ctrl Pts',(-3.84183031863679,2.37779339872086,12.2992103713621));
#33415=CARTESIAN_POINT('Ctrl Pts',(-4.23696549900952,1.7393685815216,12.3256676680466));
#33416=CARTESIAN_POINT('Ctrl Pts',(-4.46952320005253,1.00032098167222,12.3521249647311));
#33417=CARTESIAN_POINT('Ctrl Pts',(-4.51117815115765,0.250665778907295,
12.3785822614155));
#33418=CARTESIAN_POINT('Ctrl Pts',(-4.55283310226278,-0.498989423857626,
12.4050395581));
#33419=CARTESIAN_POINT('Ctrl Pts',(-4.40358530343001,-1.25925222953809,
12.4314968547845));
#33420=CARTESIAN_POINT('Ctrl Pts',(-4.08161297138,-1.93752346980879,12.4579541514689));
#33421=CARTESIAN_POINT('Ctrl Pts',(-3.75964063932998,-2.61579471007952,
12.4844114481534));
#33422=CARTESIAN_POINT('Ctrl Pts',(-3.26494377406269,-3.21207438494048,
12.5108687448379));
#33423=CARTESIAN_POINT('Ctrl Pts',(-2.65777590627122,-3.65373628991496,
12.5373260415223));
#33424=CARTESIAN_POINT('Ctrl Pts',(-2.05060803847976,-4.09539819488944,
12.5637833382068));
#33425=CARTESIAN_POINT('Ctrl Pts',(-1.33096916816412,-4.38244232997743,
12.5902406348913));
#33426=CARTESIAN_POINT('Ctrl Pts',(-0.586510513281939,-4.47990703720592,
12.6166979315757));
#33427=CARTESIAN_POINT('Ctrl Pts',(0.15794814160022,-4.57737174443441,12.6431552282602));
#33428=CARTESIAN_POINT('Ctrl Pts',(0.927226581048916,-4.48525702380341,
12.6696125249447));
#33429=CARTESIAN_POINT('Ctrl Pts',(1.62762754252377,-4.21478234633953,12.6960698216291));
#33430=CARTESIAN_POINT('Ctrl Pts',(2.32802850399863,-3.94430766887566,12.7225271183136));
#33431=CARTESIAN_POINT('Ctrl Pts',(2.95955198749964,-3.49547303457892,12.7489844149981));
#33432=CARTESIAN_POINT('Ctrl Pts',(3.44527913166315,-2.92294600516735,12.7754417116826));
#33433=CARTESIAN_POINT('Ctrl Pts',(3.93100627582668,-2.35041897575576,12.801899008367));
#33434=CARTESIAN_POINT('Ctrl Pts',(4.2709370806527,-1.65419955122932,12.8283563050515));
#33435=CARTESIAN_POINT('Ctrl Pts',(4.42366835032544,-0.919086486967588,
12.854813601736));
#33436=CARTESIAN_POINT('Ctrl Pts',(4.48640482049374,-0.617128682745771,
12.8656813003267));
#33437=CARTESIAN_POINT('Ctrl Pts',(4.51755570011492,-0.308608476653881,
12.8765489989174));
#33438=CARTESIAN_POINT('Ctrl Pts',(4.51741195309898,-5.96473381690886E-5,
12.8874166975081));
#33439=CARTESIAN_POINT('Ctrl Pts',(4.51804648040592,6.99590604930078E-5,
12.612583302492));
#33440=CARTESIAN_POINT('Ctrl Pts',(4.51754145680588,-0.679388939577024,
12.5886417444739));
#33441=CARTESIAN_POINT('Ctrl Pts',(4.36212083370235,-1.35907105681478,12.5647001864558));
#33442=CARTESIAN_POINT('Ctrl Pts',(4.06580926285153,-1.97047118281595,12.5407586284378));
#33443=CARTESIAN_POINT('Ctrl Pts',(3.73836177028969,-2.64611620618181,12.5143013317533));
#33444=CARTESIAN_POINT('Ctrl Pts',(3.23885852133923,-3.23837539221903,12.4878440350688));
#33445=CARTESIAN_POINT('Ctrl Pts',(2.62813845890645,-3.67511222754003,12.4613867383844));
#33446=CARTESIAN_POINT('Ctrl Pts',(2.01741839647366,-4.11184906286103,12.4349294416999));
#33447=CARTESIAN_POINT('Ctrl Pts',(1.29548152055856,-4.3930635474658,12.4084721450154));
#33448=CARTESIAN_POINT('Ctrl Pts',(0.550258943657521,-4.48450406835832,
12.382014848331));
#33449=CARTESIAN_POINT('Ctrl Pts',(-0.194963633243496,-4.57594458925083,
12.3555575516465));
#33450=CARTESIAN_POINT('Ctrl Pts',(-0.963471911130448,-4.47761114643111,
12.329100254962));
#33451=CARTESIAN_POINT('Ctrl Pts',(-1.66166243228881,-4.2014806444059,12.3026429582776));
#33452=CARTESIAN_POINT('Ctrl Pts',(-2.35985295344718,-3.92535014238069,
12.2761856615931));
#33453=CARTESIAN_POINT('Ctrl Pts',(-2.98772571787696,-3.47142258114999,
12.2497283649086));
#33454=CARTESIAN_POINT('Ctrl Pts',(-3.46880651775701,-2.89498583529589,
12.2232710682242));
#33455=CARTESIAN_POINT('Ctrl Pts',(-3.94988731763707,-2.31854908944178,
12.1968137715397));
#33456=CARTESIAN_POINT('Ctrl Pts',(-4.28417615296739,-1.61960315896426,
12.1703564748552));
#33457=CARTESIAN_POINT('Ctrl Pts',(-4.43095701357263,-0.883278884650216,
12.1438991781708));
#33458=CARTESIAN_POINT('Ctrl Pts',(-4.57773787417786,-0.146954610336191,
12.1174418814863));
#33459=CARTESIAN_POINT('Ctrl Pts',(-4.53701076005802,0.626748007814359,
12.0909845848018));
#33460=CARTESIAN_POINT('Ctrl Pts',(-4.31373618863893,1.34359284719155,12.0645272881174));
#33461=CARTESIAN_POINT('Ctrl Pts',(-4.09046161721984,2.06043768656874,12.0380699914329));
#33462=CARTESIAN_POINT('Ctrl Pts',(-3.6846395885015,2.72042474717257,12.0116126947484));
#33463=CARTESIAN_POINT('Ctrl Pts',(-3.1456987764459,3.24316833544978,11.985155398064));
#33464=CARTESIAN_POINT('Ctrl Pts',(-2.60675796439029,3.76591192372701,11.9586981013795));
#33465=CARTESIAN_POINT('Ctrl Pts',(-1.9346983689974,4.15141203967762,11.932240804695));
#33466=CARTESIAN_POINT('Ctrl Pts',(-1.21137610519676,4.35271519582384,11.9057835080105));
#33467=CARTESIAN_POINT('Ctrl Pts',(-0.488053841396109,4.55401835197005,
11.8793262113261));
#33468=CARTESIAN_POINT('Ctrl Pts',(0.286531090812296,4.57112454831187,11.8528689146416));
#33469=CARTESIAN_POINT('Ctrl Pts',(1.0180351039428,4.40195026906683,11.8264116179572));
#33470=CARTESIAN_POINT('Ctrl Pts',(1.74953911707329,4.2327759898218,11.7999543212727));
#33471=CARTESIAN_POINT('Ctrl Pts',(2.43796221112589,3.8773212349899,11.7734970245882));
#33472=CARTESIAN_POINT('Ctrl Pts',(2.99945521514432,3.37888000031681,11.7470397279037));
#33473=CARTESIAN_POINT('Ctrl Pts',(3.56094821916276,2.88043876564371,11.7205824312193));
#33474=CARTESIAN_POINT('Ctrl Pts',(3.99551113314703,2.23901105112941,11.6941251345348));
#33475=CARTESIAN_POINT('Ctrl Pts',(4.2502146751182,1.53272204251365,11.6676678378503));
#33476=CARTESIAN_POINT('Ctrl Pts',(4.42698035695052,1.0425535226241,11.6493063260642));
#33477=CARTESIAN_POINT('Ctrl Pts',(4.51711789485057,0.521144965264365,11.6309448142781));
#33478=CARTESIAN_POINT('Ctrl Pts',(4.5175801641472,-0.000107849321499542,
11.612583302492));
#33479=CARTESIAN_POINT('Origin',(0.,0.,20.5));
#33480=CARTESIAN_POINT('',(4.517607537138,0.000111184246189833,10.612583302492));
#33481=CARTESIAN_POINT('',(4.51779144669394,-0.000115517084662978,10.8874166975081));
#33482=CARTESIAN_POINT('',(4.51775,5.53264807684796E-16,20.5));
#33483=CARTESIAN_POINT('Ctrl Pts',(4.51779144669394,-0.000115517084662978,
10.8874166975081));
#33484=CARTESIAN_POINT('Ctrl Pts',(4.51718124885461,0.590959459307199,10.9082405451568));
#33485=CARTESIAN_POINT('Ctrl Pts',(4.40057028871007,1.18226809182004,10.9290643928055));
#33486=CARTESIAN_POINT('Ctrl Pts',(4.17452335103026,1.72826978099499,10.9498882404543));
#33487=CARTESIAN_POINT('Ctrl Pts',(3.88732422262257,2.42198061313325,10.9763455371387));
#33488=CARTESIAN_POINT('Ctrl Pts',(3.42346880605941,3.0425550177638,11.0028028338232));
#33489=CARTESIAN_POINT('Ctrl Pts',(2.83945417771489,3.51440771921171,11.0292601305077));
#33490=CARTESIAN_POINT('Ctrl Pts',(2.25543954937037,3.98626042065963,11.0557174271921));
#33491=CARTESIAN_POINT('Ctrl Pts',(1.55126570924448,4.30939141892491,11.0821747238766));
#33492=CARTESIAN_POINT('Ctrl Pts',(0.812700251733397,4.44444371603802,11.1086320205611));
#33493=CARTESIAN_POINT('Ctrl Pts',(0.0741347942222902,4.57949601315113,
11.1350893172455));
#33494=CARTESIAN_POINT('Ctrl Pts',(-0.698822280674023,4.52646960911206,
11.16154661393));
#33495=CARTESIAN_POINT('Ctrl Pts',(-1.41202565668891,4.29182306124677,11.1880039106145));
#33496=CARTESIAN_POINT('Ctrl Pts',(-2.12522903270377,4.0571765133815,11.2144612072989));
#33497=CARTESIAN_POINT('Ctrl Pts',(-2.7786787098372,3.64090982169003,11.2409185039834));
#33498=CARTESIAN_POINT('Ctrl Pts',(-3.29278524060752,3.09372380852504,11.2673758006679));
#33499=CARTESIAN_POINT('Ctrl Pts',(-3.80689177137783,2.54653779536005,11.2938330973523));
#33500=CARTESIAN_POINT('Ctrl Pts',(-4.18165515578503,1.86843246072154,11.3202903940368));
#33501=CARTESIAN_POINT('Ctrl Pts',(-4.37142962837066,1.14200028388812,11.3467476907213));
#33502=CARTESIAN_POINT('Ctrl Pts',(-4.56120410095629,0.415568107054687,
11.3732049874058));
#33503=CARTESIAN_POINT('Ctrl Pts',(-4.56598966172034,-0.359190911973653,
11.3996622840902));
#33504=CARTESIAN_POINT('Ctrl Pts',(-4.38520343465808,-1.08791198212924,
11.4261195807747));
#33505=CARTESIAN_POINT('Ctrl Pts',(-4.20441720759582,-1.81663305228484,
11.4525768774592));
#33506=CARTESIAN_POINT('Ctrl Pts',(-3.83805919270723,-2.49931617356768,
11.4790341741436));
#33507=CARTESIAN_POINT('Ctrl Pts',(-3.33075139074592,-3.05281129735225,
11.5054914708281));
#33508=CARTESIAN_POINT('Ctrl Pts',(-2.82344358878461,-3.6063064211368,11.5319487675126));
#33509=CARTESIAN_POINT('Ctrl Pts',(-2.17518599975058,-4.03061354742309,
11.558406064197));
#33510=CARTESIAN_POINT('Ctrl Pts',(-1.46493568054124,-4.27405253782339,
11.5848633608815));
#33511=CARTESIAN_POINT('Ctrl Pts',(-0.7546853613319,-4.51749152822369,11.611320657566));
#33512=CARTESIAN_POINT('Ctrl Pts',(0.017557688052746,-4.580062382738,11.6377779542504));
#33513=CARTESIAN_POINT('Ctrl Pts',(0.757735118863148,-4.4541440405356,11.6642352509349));
#33514=CARTESIAN_POINT('Ctrl Pts',(1.49791254967357,-4.3282256983332,11.6906925476194));
#33515=CARTESIAN_POINT('Ctrl Pts',(2.20602436190975,-4.01381815941408,11.7171498443038));
#33516=CARTESIAN_POINT('Ctrl Pts',(2.79582332053076,-3.54921591405394,11.7436071409883));
#33517=CARTESIAN_POINT('Ctrl Pts',(3.38562227915178,-3.0846136686938,11.7700644376728));
#33518=CARTESIAN_POINT('Ctrl Pts',(3.85710838415764,-2.46981671689265,11.7965217343572));
#33519=CARTESIAN_POINT('Ctrl Pts',(4.15285514976701,-1.77970664696488,11.8229790310417));
#33520=CARTESIAN_POINT('Ctrl Pts',(4.39295566177474,-1.21944428605644,11.8444582531972));
#33521=CARTESIAN_POINT('Ctrl Pts',(4.51722774785459,-0.609543637247958,
11.8659374753526));
#33522=CARTESIAN_POINT('Ctrl Pts',(4.5178502562812,0.000110962492481057,
11.8874166975081));
#33523=CARTESIAN_POINT('Ctrl Pts',(4.5175801641472,-0.000107849321499542,
11.612583302492));
#33524=CARTESIAN_POINT('Ctrl Pts',(4.51778398357309,-0.229933732598545,
11.6044875175936));
#33525=CARTESIAN_POINT('Ctrl Pts',(4.50055473854231,-0.45972933914648,11.5963917326953));
#33526=CARTESIAN_POINT('Ctrl Pts',(4.46563124792392,-0.686803612223187,
11.5882959477969));
#33527=CARTESIAN_POINT('Ctrl Pts',(4.35150010880038,-1.42888995562703,11.5618386511125));
#33528=CARTESIAN_POINT('Ctrl Pts',(4.04839366059521,-2.14191233971748,11.535381354428));
#33529=CARTESIAN_POINT('Ctrl Pts',(3.59322993324244,-2.73902542723646,11.5089240577435));
#33530=CARTESIAN_POINT('Ctrl Pts',(3.13806620588969,-3.33613851475543,11.4824667610591));
#33531=CARTESIAN_POINT('Ctrl Pts',(2.53084519938934,-3.81734230570294,11.4560094643746));
#33532=CARTESIAN_POINT('Ctrl Pts',(1.84552576030269,-4.12402671090484,11.4295521676901));
#33533=CARTESIAN_POINT('Ctrl Pts',(1.16020632121604,-4.43071111610674,11.4030948710056));
#33534=CARTESIAN_POINT('Ctrl Pts',(0.396788449543078,-4.56287613556304,
11.3766375743212));
#33535=CARTESIAN_POINT('Ctrl Pts',(-0.351744402844812,-4.50442421617511,
11.3501802776367));
#33536=CARTESIAN_POINT('Ctrl Pts',(-1.10027725523272,-4.44597229678718,
11.3237229809523));
#33537=CARTESIAN_POINT('Ctrl Pts',(-1.83392508833558,-4.196903438555,11.2972656842678));
#33538=CARTESIAN_POINT('Ctrl Pts',(-2.4633304080324,-3.787553952759,11.2708083875833));
#33539=CARTESIAN_POINT('Ctrl Pts',(-3.0927357277292,-3.378204466963,11.2443510908988));
#33540=CARTESIAN_POINT('Ctrl Pts',(-3.61789853401999,-2.80857435360317,
11.2178937942144));
#33541=CARTESIAN_POINT('Ctrl Pts',(-3.97485457831262,-2.1480439300593,11.1914364975299));
#33542=CARTESIAN_POINT('Ctrl Pts',(-4.33181062260526,-1.48751350651541,
11.1649792008454));
#33543=CARTESIAN_POINT('Ctrl Pts',(-4.52055990489972,-0.736082772787468,
11.138521904161));
#33544=CARTESIAN_POINT('Ctrl Pts',(-4.51811297150728,0.0147248393883086,
11.1120646074765));
#33545=CARTESIAN_POINT('Ctrl Pts',(-4.51566603811484,0.765532451564064,
11.085607310792));
#33546=CARTESIAN_POINT('Ctrl Pts',(-4.32202288903552,1.5157169421876,11.0591500141076));
#33547=CARTESIAN_POINT('Ctrl Pts',(-3.96076904551623,2.17390667055369,11.0326927174231));
#33548=CARTESIAN_POINT('Ctrl Pts',(-3.59951520199693,2.83209639891979,11.0062354207386));
#33549=CARTESIAN_POINT('Ctrl Pts',(-3.07065066403766,3.3982913650284,10.9797781240542));
#33550=CARTESIAN_POINT('Ctrl Pts',(-2.43859054705097,3.8035296486331,10.9533208273697));
#33551=CARTESIAN_POINT('Ctrl Pts',(-1.8065304300643,4.20876793223779,10.9268635306852));
#33552=CARTESIAN_POINT('Ctrl Pts',(-1.0712747340502,4.4530495333386,10.9004062340008));
#33553=CARTESIAN_POINT('Ctrl Pts',(-0.322376789052762,4.50662122327553,
10.8739489373163));
#33554=CARTESIAN_POINT('Ctrl Pts',(0.426521155944698,4.56019291321245,10.8474916406318));
#33555=CARTESIAN_POINT('Ctrl Pts',(1.18906134992551,4.42305469198549,10.8210343439474));
#33556=CARTESIAN_POINT('Ctrl Pts',(1.87236724118984,4.11190984316492,10.7945770472629));
#33557=CARTESIAN_POINT('Ctrl Pts',(2.55567313245417,3.80076499434435,10.7681197505784));
#33558=CARTESIAN_POINT('Ctrl Pts',(3.15974472100203,3.31561351793017,10.741662453894));
#33559=CARTESIAN_POINT('Ctrl Pts',(3.61100675589317,2.71554632681736,10.7152051572095));
#33560=CARTESIAN_POINT('Ctrl Pts',(4.0622687907843,2.11547913570456,10.688747860525));
#33561=CARTESIAN_POINT('Ctrl Pts',(4.36072127201872,1.40049622989312,10.6622905638405));
#33562=CARTESIAN_POINT('Ctrl Pts',(4.47001301768877,0.657681736016976,10.6358332671561));
#33563=CARTESIAN_POINT('Ctrl Pts',(4.5020272386327,0.440093233047143,10.6280832789347));
#33564=CARTESIAN_POINT('Ctrl Pts',(4.51781057668589,0.220116648612125,10.6203332907133));
#33565=CARTESIAN_POINT('Ctrl Pts',(4.517607537138,0.000111184246189833,
10.612583302492));
#33566=CARTESIAN_POINT('Origin',(0.,0.,20.5));
#33567=CARTESIAN_POINT('',(4.51802315729813,-7.77880120685776E-5,9.61258330249199));
#33568=CARTESIAN_POINT('',(4.5174420818448,7.39595355181285E-5,9.88741669750808));
#33569=CARTESIAN_POINT('',(4.51775,5.53264807684796E-16,20.5));
#33570=CARTESIAN_POINT('Ctrl Pts',(4.5174420818448,7.39595355181285E-5,
9.88741669750808));
#33571=CARTESIAN_POINT('Ctrl Pts',(4.51761100468578,0.290010274247371,9.89762902159206));
#33572=CARTESIAN_POINT('Ctrl Pts',(4.49012793116805,0.579914973420611,9.90784134567604));
#33573=CARTESIAN_POINT('Ctrl Pts',(4.43468447094956,0.864369878764984,9.91805366976002));
#33574=CARTESIAN_POINT('Ctrl Pts',(4.29104585704042,1.60131357171471,9.94451096644449));
#33575=CARTESIAN_POINT('Ctrl Pts',(3.95974153092839,2.30167910674412,9.97096826312895));
#33576=CARTESIAN_POINT('Ctrl Pts',(3.48112399286906,2.88016273680304,9.99742555981342));
#33577=CARTESIAN_POINT('Ctrl Pts',(3.00250645480973,3.45864636686196,10.0238828564979));
#33578=CARTESIAN_POINT('Ctrl Pts',(2.3765757048031,3.91524809195038,10.0503401531824));
#33579=CARTESIAN_POINT('Ctrl Pts',(1.67956941546288,4.19435432728793,10.0767974498668));
#33580=CARTESIAN_POINT('Ctrl Pts',(0.982563126122689,4.47346056262548,10.1032547465513));
#33581=CARTESIAN_POINT('Ctrl Pts',(0.214481297448898,4.57507130821216,10.1297120432358));
#33582=CARTESIAN_POINT('Ctrl Pts',(-0.531124553886154,4.4868104876913,10.1561693399202));
#33583=CARTESIAN_POINT('Ctrl Pts',(-1.27673040522121,4.39854966717044,10.1826266366047));
#33584=CARTESIAN_POINT('Ctrl Pts',(-1.99986027921753,4.12041728054204,10.2090839332892));
#33585=CARTESIAN_POINT('Ctrl Pts',(-2.61243775753278,3.68628954467964,10.2355412299736));
#33586=CARTESIAN_POINT('Ctrl Pts',(-3.22501523584806,3.25216180881724,10.2619985266581));
#33587=CARTESIAN_POINT('Ctrl Pts',(-3.72704031848226,2.66203872372082,10.2884558233426));
#33588=CARTESIAN_POINT('Ctrl Pts',(-4.05736690597737,1.9877966280475,10.314913120027));
#33589=CARTESIAN_POINT('Ctrl Pts',(-4.38769349347249,1.31355453237416,10.3413704167115));
#33590=CARTESIAN_POINT('Ctrl Pts',(-4.54632158582851,0.555193426123966,
10.367827713396));
#33591=CARTESIAN_POINT('Ctrl Pts',(-4.51393045695515,-0.194919147263826,
10.3942850100804));
#33592=CARTESIAN_POINT('Ctrl Pts',(-4.48153932808179,-0.945031720651576,
10.4207423067649));
#33593=CARTESIAN_POINT('Ctrl Pts',(-4.25812897797905,-1.68689576117688,
10.4471996034494));
#33594=CARTESIAN_POINT('Ctrl Pts',(-3.87091054003425,-2.33015304974784,
10.4736569001339));
#33595=CARTESIAN_POINT('Ctrl Pts',(-3.48369210208944,-2.9734103383188,10.5001141968183));
#33596=CARTESIAN_POINT('Ctrl Pts',(-2.93266557630255,-3.51806087493544,
10.5265714935028));
#33597=CARTESIAN_POINT('Ctrl Pts',(-2.28494538367617,-3.89776682701959,
10.5530287901872));
#33598=CARTESIAN_POINT('Ctrl Pts',(-1.63722519104977,-4.27747277910375,
10.5794860868717));
#33599=CARTESIAN_POINT('Ctrl Pts',(-0.892811331583869,-4.49223414665542,
10.6059433835562));
#33600=CARTESIAN_POINT('Ctrl Pts',(-0.142372589495352,-4.51589323278992,
10.6324006802407));
#33601=CARTESIAN_POINT('Ctrl Pts',(0.608066152593165,-4.53955231892441,
10.6588579769251));
#33602=CARTESIAN_POINT('Ctrl Pts',(1.36452977730431,-4.37210912364174,10.6853152736096));
#33603=CARTESIAN_POINT('Ctrl Pts',(2.03488185235016,-4.03395804281271,10.7117725702941));
#33604=CARTESIAN_POINT('Ctrl Pts',(2.70523392739599,-3.6958069619837,10.7382298669785));
#33605=CARTESIAN_POINT('Ctrl Pts',(3.28947445277654,-3.18694799560833,10.764687163663));
#33606=CARTESIAN_POINT('Ctrl Pts',(3.71644357909769,-2.56935960262103,10.7911444603475));
#33607=CARTESIAN_POINT('Ctrl Pts',(4.14341270541885,-1.95177120963373,10.8176017570319));
#33608=CARTESIAN_POINT('Ctrl Pts',(4.41311043268061,-1.22545339003449,10.8440590537164));
#33609=CARTESIAN_POINT('Ctrl Pts',(4.49268787618539,-0.478870850411892,
10.8705163504009));
#33610=CARTESIAN_POINT('Ctrl Pts',(4.50963199098762,-0.319903940901298,
10.8761497994366));
#33611=CARTESIAN_POINT('Ctrl Pts',(4.51795652273981,-0.160018279147252,
10.8817832484723));
#33612=CARTESIAN_POINT('Ctrl Pts',(4.51779144669394,-0.000115517084662978,
10.8874166975081));
#33613=CARTESIAN_POINT('Ctrl Pts',(4.517607537138,0.000111184246189833,
10.612583302492));
#33614=CARTESIAN_POINT('Ctrl Pts',(4.51711743014117,-0.530948988737395,
10.5938759940289));
#33615=CARTESIAN_POINT('Ctrl Pts',(4.42347995325767,-1.06217743558981,10.5751686855658));
#33616=CARTESIAN_POINT('Ctrl Pts',(4.24013400258143,-1.56039266992325,10.5564613771027));
#33617=CARTESIAN_POINT('Ctrl Pts',(3.98083223169834,-2.26500650004656,10.5300040804182));
#33618=CARTESIAN_POINT('Ctrl Pts',(3.54209767982647,-2.90358807835227,10.5035467837338));
#33619=CARTESIAN_POINT('Ctrl Pts',(2.9773677298226,-3.39835887534092,10.4770894870493));
#33620=CARTESIAN_POINT('Ctrl Pts',(2.41263777981875,-3.89312967232955,10.4506321903648));
#33621=CARTESIAN_POINT('Ctrl Pts',(1.7219124316829,-4.24408968800111,10.4241748936803));
#33622=CARTESIAN_POINT('Ctrl Pts',(0.989321268370679,-4.40849238086523,
10.3977175969959));
#33623=CARTESIAN_POINT('Ctrl Pts',(0.256730105058482,-4.57289507372935,
10.3712603003114));
#33624=CARTESIAN_POINT('Ctrl Pts',(-0.517726873430066,-4.55074044378602,
10.3448030036269));
#33625=CARTESIAN_POINT('Ctrl Pts',(-1.2397216642308,-4.34472690044313,10.3183457069425));
#33626=CARTESIAN_POINT('Ctrl Pts',(-1.96171645503154,-4.13871335710024,
10.291888410258));
#33627=CARTESIAN_POINT('Ctrl Pts',(-2.63124905814445,-3.74884090035779,
10.2654311135735));
#33628=CARTESIAN_POINT('Ctrl Pts',(-3.16677114350303,-3.22259556396298,
10.2389738168891));
#33629=CARTESIAN_POINT('Ctrl Pts',(-3.70229322886161,-2.69635022756818,
10.2125165202046));
#33630=CARTESIAN_POINT('Ctrl Pts',(-4.10380479646586,-2.033732011521,10.1860592235201));
#33631=CARTESIAN_POINT('Ctrl Pts',(-4.32240218174696,-1.31544708119576,
10.1596019268357));
#33632=CARTESIAN_POINT('Ctrl Pts',(-4.54099956702807,-0.597162150870509,
10.1331446301512));
#33633=CARTESIAN_POINT('Ctrl Pts',(-4.57668276998605,0.176789493732823,
10.1066873334667));
#33634=CARTESIAN_POINT('Ctrl Pts',(-4.42510561599232,0.912141398858014,
10.0802300367823));
#33635=CARTESIAN_POINT('Ctrl Pts',(-4.27352846199858,1.64749330398323,10.0537727400978));
#33636=CARTESIAN_POINT('Ctrl Pts',(-3.93469095105313,2.34424546963029,10.0273154434133));
#33637=CARTESIAN_POINT('Ctrl Pts',(-3.44986311698706,2.91753425314077,10.0008581467289));
#33638=CARTESIAN_POINT('Ctrl Pts',(-2.965035282921,3.49082303665126,9.97440085004439));
#33639=CARTESIAN_POINT('Ctrl Pts',(-2.33421712573433,3.94064843802516,9.94794355335992));
#33640=CARTESIAN_POINT('Ctrl Pts',(-1.63424159882622,4.21222222121095,9.92148625667545));
#33641=CARTESIAN_POINT('Ctrl Pts',(-0.93426607191815,4.48379600439673,9.89502895999098));
#33642=CARTESIAN_POINT('Ctrl Pts',(-0.165133175288626,4.57711816939442,
9.86857166330652));
#33643=CARTESIAN_POINT('Ctrl Pts',(0.579477555476215,4.48082217978985,9.84211436662205));
#33644=CARTESIAN_POINT('Ctrl Pts',(1.32408828624107,4.38452619018528,9.81565706993759));
#33645=CARTESIAN_POINT('Ctrl Pts',(2.04417685114126,4.09861204597845,9.78919977325312));
#33646=CARTESIAN_POINT('Ctrl Pts',(2.65203725991646,3.65790377350364,9.76274247656865));
#33647=CARTESIAN_POINT('Ctrl Pts',(3.25989766869166,3.21719550102883,9.73628517988418));
#33648=CARTESIAN_POINT('Ctrl Pts',(3.75552992134187,2.62169310028604,9.70982788319971));
#33649=CARTESIAN_POINT('Ctrl Pts',(4.07856655802598,1.94392810462463,9.68337058651525));
#33650=CARTESIAN_POINT('Ctrl Pts',(4.36666460048778,1.33946797123696,9.65977482517416));
#33651=CARTESIAN_POINT('Ctrl Pts',(4.51748278690866,0.669577455247932,9.63617906383307));
#33652=CARTESIAN_POINT('Ctrl Pts',(4.51802315729813,-7.77880120685776E-5,
9.61258330249199));
#33653=CARTESIAN_POINT('Origin',(0.,0.,20.5));
#33654=CARTESIAN_POINT('',(4.51736326149566,6.46810088806768E-6,8.61258330249198));
#33655=CARTESIAN_POINT('',(4.51813428255233,-1.20076389504314E-5,8.88741669750808));
#33656=CARTESIAN_POINT('',(4.51775,5.53264807684796E-16,20.5));
#33657=CARTESIAN_POINT('Ctrl Pts',(4.51813428255233,-1.20076389504314E-5,
8.88741669750808));
#33658=CARTESIAN_POINT('Ctrl Pts',(4.51802118875718,0.73947229319191,8.91347479471178));
#33659=CARTESIAN_POINT('Ctrl Pts',(4.3327730937107,1.47901118956561,8.93953289191547));
#33660=CARTESIAN_POINT('Ctrl Pts',(3.9839812468855,2.13106899669204,8.96559098911917));
#33661=CARTESIAN_POINT('Ctrl Pts',(3.62984605042663,2.79311606496825,8.99204828580364));
#33662=CARTESIAN_POINT('Ctrl Pts',(3.10711787221281,3.36498116344761,9.01850558248812));
#33663=CARTESIAN_POINT('Ctrl Pts',(2.47946442583089,3.77701175603631,9.04496287917258));
#33664=CARTESIAN_POINT('Ctrl Pts',(1.85181097944898,4.189042348625,9.07142017585705));
#33665=CARTESIAN_POINT('Ctrl Pts',(1.11923226489897,4.44123843532303,9.09787747254152));
#33666=CARTESIAN_POINT('Ctrl Pts',(0.370955558845314,4.50288281188386,9.12433476922598));
#33667=CARTESIAN_POINT('Ctrl Pts',(-0.377321147208358,4.5645271884447,9.15079206591045));
#33668=CARTESIAN_POINT('Ctrl Pts',(-1.14129584476571,4.43561985486832,9.17724936259492));
#33669=CARTESIAN_POINT('Ctrl Pts',(-1.82791726117885,4.13186158171856,9.20370665927939));
#33670=CARTESIAN_POINT('Ctrl Pts',(-2.51453867759199,3.82810330856881,9.23016395596386));
#33671=CARTESIAN_POINT('Ctrl Pts',(-3.12380681286095,3.34949409584567,9.25662125264832));
#33672=CARTESIAN_POINT('Ctrl Pts',(-3.58151348240605,2.75432801596707,9.28307854933279));
#33673=CARTESIAN_POINT('Ctrl Pts',(-4.03922015195113,2.15916193608848,9.30953584601726));
#33674=CARTESIAN_POINT('Ctrl Pts',(-4.34536535577235,1.44743898905445,9.33599314270173));
#33675=CARTESIAN_POINT('Ctrl Pts',(-4.46266094686473,0.705846242127692,
9.3624504393862));
#33676=CARTESIAN_POINT('Ctrl Pts',(-4.57995653795712,-0.0357465047990668,
9.38890773607066));
#33677=CARTESIAN_POINT('Ctrl Pts',(-4.50840251632067,-0.807209051618545,
9.41536503275513));
#33678=CARTESIAN_POINT('Ctrl Pts',(-4.25671408259964,-1.51457811392983,
9.4418223294396));
#33679=CARTESIAN_POINT('Ctrl Pts',(-4.00502564887861,-2.22194717624114,
9.46827962612407));
#33680=CARTESIAN_POINT('Ctrl Pts',(-3.57320280307299,-2.86522275404424,
9.49473692280854));
#33681=CARTESIAN_POINT('Ctrl Pts',(-3.01384108989007,-3.36605459389589,
9.521194219493));
#33682=CARTESIAN_POINT('Ctrl Pts',(-2.45447937670717,-3.86688643374753,
9.54765151617747));
#33683=CARTESIAN_POINT('Ctrl Pts',(-1.76757879614698,-4.22527453564772,
9.57410881286193));
#33684=CARTESIAN_POINT('Ctrl Pts',(-1.03680307870741,-4.39756762542433,
9.6005661095464));
#33685=CARTESIAN_POINT('Ctrl Pts',(-0.306027361267855,-4.56986071520094,
9.62702340623087));
#33686=CARTESIAN_POINT('Ctrl Pts',(0.468623493051109,-4.55605879285398,
9.65348070291534));
#33687=CARTESIAN_POINT('Ctrl Pts',(1.19279786752367,-4.35784291725027,9.67993799959981));
#33688=CARTESIAN_POINT('Ctrl Pts',(1.91697224199627,-4.15962704164656,9.70639529628428));
#33689=CARTESIAN_POINT('Ctrl Pts',(2.59067013662248,-3.7769972127861,9.73285259296875));
#33690=CARTESIAN_POINT('Ctrl Pts',(3.13183589343935,-3.25655732035571,9.75930988965321));
#33691=CARTESIAN_POINT('Ctrl Pts',(3.67300165025619,-2.73611742792533,9.78576718633768));
#33692=CARTESIAN_POINT('Ctrl Pts',(4.08163526926369,-2.07786747192505,9.81222448302215));
#33693=CARTESIAN_POINT('Ctrl Pts',(4.30796562791432,-1.3619815684899,9.83868177970662));
#33694=CARTESIAN_POINT('Ctrl Pts',(4.44693411433176,-0.922422416809593,
9.8549267523071));
#33695=CARTESIAN_POINT('Ctrl Pts',(4.51717337249904,-0.461134228693464,
9.87117172490759));
#33696=CARTESIAN_POINT('Ctrl Pts',(4.5174420818448,7.39595355181285E-5,
9.88741669750808));
#33697=CARTESIAN_POINT('Ctrl Pts',(4.51802315729813,-7.77880120685776E-5,
9.61258330249199));
#33698=CARTESIAN_POINT('Ctrl Pts',(4.51808868978702,-0.081289075021137,
9.60972176714861));
#33699=CARTESIAN_POINT('Ctrl Pts',(4.51594405515544,-0.162496901825208,
9.60686023180522));
#33700=CARTESIAN_POINT('Ctrl Pts',(4.51156607035433,-0.243584147729178,
9.60399869646184));
#33701=CARTESIAN_POINT('Ctrl Pts',(4.47108792528055,-0.993303813841435,
9.57754139977738));
#33702=CARTESIAN_POINT('Ctrl Pts',(4.23969061441499,-1.73271555548592,9.5510841030929));
#33703=CARTESIAN_POINT('Ctrl Pts',(3.84555807412645,-2.37175984086041,9.52462680640843));
#33704=CARTESIAN_POINT('Ctrl Pts',(3.45142553383792,-3.0108041262349,9.49816950972396));
#33705=CARTESIAN_POINT('Ctrl Pts',(2.8945577641264,-3.54948095533939,9.47171221303951));
#33706=CARTESIAN_POINT('Ctrl Pts',(2.24278064303981,-3.92218008655942,9.44525491635504));
#33707=CARTESIAN_POINT('Ctrl Pts',(1.59100352195321,-4.29487921777947,9.41879761967057));
#33708=CARTESIAN_POINT('Ctrl Pts',(0.844317049491529,-4.50160065111505,
9.3923403229861));
#33709=CARTESIAN_POINT('Ctrl Pts',(0.0936668116193721,-4.51716594477095,
9.36588302630163));
#33710=CARTESIAN_POINT('Ctrl Pts',(-0.656983426252764,-4.53273123842686,
9.33942572961716));
#33711=CARTESIAN_POINT('Ctrl Pts',(-1.41159742953537,-4.3571403924031,9.3129684329327));
#33712=CARTESIAN_POINT('Ctrl Pts',(-2.07826404778352,-4.01178017741349,
9.28651113624823));
#33713=CARTESIAN_POINT('Ctrl Pts',(-2.74493066603167,-3.66641996242389,
9.26005383956376));
#33714=CARTESIAN_POINT('Ctrl Pts',(-3.32364989924536,-3.15129037846845,
9.23359654287929));
#33715=CARTESIAN_POINT('Ctrl Pts',(-3.7439343853058,-2.52913363876293,9.20713924619482));
#33716=CARTESIAN_POINT('Ctrl Pts',(-4.16421887136626,-1.9069768990574,9.18068194951035));
#33717=CARTESIAN_POINT('Ctrl Pts',(-4.42606861027347,-1.1777930036018,9.15422465282589));
#33718=CARTESIAN_POINT('Ctrl Pts',(-4.49759059362582,-0.430395743852028,
9.12776735614142));
#33719=CARTESIAN_POINT('Ctrl Pts',(-4.56911257697816,0.317001515897712,
9.10131005945695));
#33720=CARTESIAN_POINT('Ctrl Pts',(-4.45030680477565,1.08261213994165,9.07485276277248));
#33721=CARTESIAN_POINT('Ctrl Pts',(-4.15564368858649,1.77318560159636,9.04839546608801));
#33722=CARTESIAN_POINT('Ctrl Pts',(-3.86098057239734,2.46375906325108,9.02193816940354));
#33723=CARTESIAN_POINT('Ctrl Pts',(-3.39046011222153,3.0792953625166,8.99548087271908));
#33724=CARTESIAN_POINT('Ctrl Pts',(-2.8013911793688,3.54482285937563,8.96902357603462));
#33725=CARTESIAN_POINT('Ctrl Pts',(-2.21232224651606,4.01035035623468,8.94256627935015));
#33726=CARTESIAN_POINT('Ctrl Pts',(-1.50470484098639,4.32586905068723,8.91610898266568));
#33727=CARTESIAN_POINT('Ctrl Pts',(-0.76472597963103,4.45294911494335,8.88965168598121));
#33728=CARTESIAN_POINT('Ctrl Pts',(-0.0247471182756658,4.58002917919947,
8.86319438929674));
#33729=CARTESIAN_POINT('Ctrl Pts',(0.747593198905389,4.51867061325916,8.83673709261227));
#33730=CARTESIAN_POINT('Ctrl Pts',(1.45822477605263,4.27634682254651,8.8102797959278));
#33731=CARTESIAN_POINT('Ctrl Pts',(2.16885635319985,4.03402303183387,8.78382249924334));
#33732=CARTESIAN_POINT('Ctrl Pts',(2.81777919031325,3.6107340163489,8.75736520255887));
#33733=CARTESIAN_POINT('Ctrl Pts',(3.3259552040156,3.0580359097105,8.7309079058744));
#33734=CARTESIAN_POINT('Ctrl Pts',(3.83413121771795,2.5053378030721,8.70445060918993));
#33735=CARTESIAN_POINT('Ctrl Pts',(4.20156040800925,1.82323060528026,8.67799331250546));
#33736=CARTESIAN_POINT('Ctrl Pts',(4.38349030615737,1.0947942181167,8.65153601582099));
#33737=CARTESIAN_POINT('Ctrl Pts',(4.47277460017851,0.737305266442263,8.63855177804465));
#33738=CARTESIAN_POINT('Ctrl Pts',(4.51738186963902,0.368658049377594,8.62556754026832));
#33739=CARTESIAN_POINT('Ctrl Pts',(4.51736350124836,6.46409108656654E-6,
8.61258330249198));
#33740=CARTESIAN_POINT('Origin',(0.,0.,20.5));
#33741=CARTESIAN_POINT('',(4.51805554098247,6.65521552928316E-5,7.61258330249197));
#33742=CARTESIAN_POINT('',(4.51740628246061,-5.63430382605529E-5,7.88741669750807));
#33743=CARTESIAN_POINT('',(4.51775,5.53264807684796E-16,20.5));
#33744=CARTESIAN_POINT('Ctrl Pts',(4.51740628246061,-5.63430382605529E-5,
7.88741669750807));
#33745=CARTESIAN_POINT('Ctrl Pts',(4.51721359264065,0.438494588092411,7.90286327114702));
#33746=CARTESIAN_POINT('Ctrl Pts',(4.45380791076361,0.877100051477632,7.91830984478598));
#33747=CARTESIAN_POINT('Ctrl Pts',(4.32797411068275,1.29699720179238,7.93375641842493));
#33748=CARTESIAN_POINT('Ctrl Pts',(4.1124426757192,2.01620805997421,7.9602137151094));
#33749=CARTESIAN_POINT('Ctrl Pts',(3.71376126713352,2.68053296061069,7.98667101179386));
#33750=CARTESIAN_POINT('Ctrl Pts',(3.18048883925826,3.20905786603343,8.01312830847833));
#33751=CARTESIAN_POINT('Ctrl Pts',(2.64721641138298,3.73758277145619,8.0395856051628));
#33752=CARTESIAN_POINT('Ctrl Pts',(1.97935296421813,4.13030768166519,8.06604290184727));
#33753=CARTESIAN_POINT('Ctrl Pts',(1.25824352648304,4.33939913723789,8.09250019853174));
#33754=CARTESIAN_POINT('Ctrl Pts',(0.53713408874796,4.54849059281059,8.11895749521621));
#33755=CARTESIAN_POINT('Ctrl Pts',(-0.237221339557352,4.57394859374699,
8.14541479190067));
#33756=CARTESIAN_POINT('Ctrl Pts',(-0.970507124268639,4.41267238370822,
8.17187208858514));
#33757=CARTESIAN_POINT('Ctrl Pts',(-1.70379290897991,4.25139617366945,8.19832938526961));
#33758=CARTESIAN_POINT('Ctrl Pts',(-2.39600905009715,3.90338575265551,8.22478668195408));
#33759=CARTESIAN_POINT('Ctrl Pts',(-2.96284438772951,3.4110284047919,8.25124397863854));
#33760=CARTESIAN_POINT('Ctrl Pts',(-3.52967972536187,2.91867105692828,8.27770127532301));
#33761=CARTESIAN_POINT('Ctrl Pts',(-3.97113425950935,2.28196678221498,8.30415857200748));
#33762=CARTESIAN_POINT('Ctrl Pts',(-4.2334393164843,1.57846545665159,8.33061586869195));
#33763=CARTESIAN_POINT('Ctrl Pts',(-4.49574437345926,0.874964131088192,
8.35707316537641));
#33764=CARTESIAN_POINT('Ctrl Pts',(-4.57889995326168,0.104665754674698,
8.38353046206088));
#33765=CARTESIAN_POINT('Ctrl Pts',(-4.47277779830253,-0.638608182855007,
8.40998775874535));
#33766=CARTESIAN_POINT('Ctrl Pts',(-4.36665564334337,-1.38188212038471,
8.43644505542982));
#33767=CARTESIAN_POINT('Ctrl Pts',(-4.07125575362263,-2.09813161903063,
8.46290235211428));
#33768=CARTESIAN_POINT('Ctrl Pts',(-3.62255750878001,-2.70011828255337,
8.48935964879875));
#33769=CARTESIAN_POINT('Ctrl Pts',(-3.17385926393738,-3.30210494607612,
8.51581694548322));
#33770=CARTESIAN_POINT('Ctrl Pts',(-2.57186266397286,-3.78982877447569,
8.54227424216769));
#33771=CARTESIAN_POINT('Ctrl Pts',(-1.88989022851369,-4.10388554523221,
8.56873153885216));
#33772=CARTESIAN_POINT('Ctrl Pts',(-1.20791779305452,-4.41794231598872,
8.59518883553663));
#33773=CARTESIAN_POINT('Ctrl Pts',(-0.445969522100707,-4.55833202910218,
8.62164613222109));
#33774=CARTESIAN_POINT('Ctrl Pts',(0.30315012821752,-4.50795537288903,8.64810342890556));
#33775=CARTESIAN_POINT('Ctrl Pts',(1.05226977853573,-4.45757871667589,8.67456072559003));
#33776=CARTESIAN_POINT('Ctrl Pts',(1.78856080821834,-4.21643569113615,8.7010180222745));
#33777=CARTESIAN_POINT('Ctrl Pts',(2.42234378472631,-3.81389724990005,8.72747531895897));
#33778=CARTESIAN_POINT('Ctrl Pts',(3.05612676123428,-3.41135880866395,8.75393261564343));
#33779=CARTESIAN_POINT('Ctrl Pts',(3.58740168456759,-2.84742495173149,8.78038991232789));
#33780=CARTESIAN_POINT('Ctrl Pts',(3.95145985704281,-2.19078219875382,8.80684720901236));
#33781=CARTESIAN_POINT('Ctrl Pts',(4.31551802951803,-1.53413944577613,8.83330450569683));
#33782=CARTESIAN_POINT('Ctrl Pts',(4.51235945113515,-0.78478779675323,8.85976180238131));
#33783=CARTESIAN_POINT('Ctrl Pts',(4.51800905459174,-0.0339974532052447,
8.88621909906578));
#33784=CARTESIAN_POINT('Ctrl Pts',(4.51809429832594,-0.0226691939774265,
8.88661829854654));
#33785=CARTESIAN_POINT('Ctrl Pts',(4.5181360151034,-0.0113406072147017,
8.88701749802731));
#33786=CARTESIAN_POINT('Ctrl Pts',(4.51813428255233,-1.20076389504314E-5,
8.88741669750808));
#33787=CARTESIAN_POINT('Ctrl Pts',(4.51736350124836,6.46409108656654E-6,
8.61258330249198));
#33788=CARTESIAN_POINT('Ctrl Pts',(4.5173444413379,-0.382523847714403,8.59911024358385));
#33789=CARTESIAN_POINT('Ctrl Pts',(4.46927642784078,-0.765058862836159,
8.58563718467573));
#33790=CARTESIAN_POINT('Ctrl Pts',(4.37321687241043,-1.13513692172449,8.5721641257676));
#33791=CARTESIAN_POINT('Ctrl Pts',(4.18458293451042,-1.86186609786678,8.54570682908313));
#33792=CARTESIAN_POINT('Ctrl Pts',(3.81088445270546,-2.54055887361605,8.51924953239865));
#33793=CARTESIAN_POINT('Ctrl Pts',(3.29763748849563,-3.08855122001653,8.49279223571418));
#33794=CARTESIAN_POINT('Ctrl Pts',(2.78439052428581,-3.636543566417,8.46633493902971));
#33795=CARTESIAN_POINT('Ctrl Pts',(2.13159507767111,-4.05383548346868,8.43987764234525));
#33796=CARTESIAN_POINT('Ctrl Pts',(1.4187609115801,-4.28960127750468,8.41342034566079));
#33797=CARTESIAN_POINT('Ctrl Pts',(0.705926745489094,-4.52536707154067,
8.38696304897632));
#33798=CARTESIAN_POINT('Ctrl Pts',(-0.0669461400782259,-4.57960674256099,
8.36050575229184));
#33799=CARTESIAN_POINT('Ctrl Pts',(-0.805722683022316,-4.44571395866409,
8.33404845560738));
#33800=CARTESIAN_POINT('Ctrl Pts',(-1.54449922596642,-4.31182117476718,
8.30759115892291));
#33801=CARTESIAN_POINT('Ctrl Pts',(-2.24917942628729,-3.98979593595305,
8.28113386223845));
#33802=CARTESIAN_POINT('Ctrl Pts',(-2.83393401547744,-3.51886055991386,
8.25467656555398));
#33803=CARTESIAN_POINT('Ctrl Pts',(-3.41868860466758,-3.04792518387468,
8.22821926886951));
#33804=CARTESIAN_POINT('Ctrl Pts',(-3.88351758272698,-2.42807967061047,
8.20176197218504));
#33805=CARTESIAN_POINT('Ctrl Pts',(-4.17180529456878,-1.73482051763438,
8.17530467550057));
#33806=CARTESIAN_POINT('Ctrl Pts',(-4.46009300641058,-1.0415613646583,8.1488473788161));
#33807=CARTESIAN_POINT('Ctrl Pts',(-4.57183945203477,-0.274888571970355,
8.12239008213164));
#33808=CARTESIAN_POINT('Ctrl Pts',(-4.49343403803759,0.471817962780769,
8.09593278544718));
#33809=CARTESIAN_POINT('Ctrl Pts',(-4.41502862404041,1.21852449753188,8.06947548876271));
#33810=CARTESIAN_POINT('Ctrl Pts',(-4.14647135042187,1.94526477434618,8.04301819207824));
#33811=CARTESIAN_POINT('Ctrl Pts',(-3.72047219588799,2.56352263181385,8.01656089539377));
#33812=CARTESIAN_POINT('Ctrl Pts',(-3.2944730413541,3.18178048928153,7.9901035987093));
#33813=CARTESIAN_POINT('Ctrl Pts',(-2.71103200590485,3.69155592740257,7.96364630202483));
#33814=CARTESIAN_POINT('Ctrl Pts',(-2.04121156194556,4.03075886199821,7.93718900534037));
#33815=CARTESIAN_POINT('Ctrl Pts',(-1.37139111798628,4.36996179659386,7.9107317086559));
#33816=CARTESIAN_POINT('Ctrl Pts',(-0.615191265516958,4.53859222766412,
7.88427441197143));
#33817=CARTESIAN_POINT('Ctrl Pts',(0.135283690341632,4.5161111553332,7.85781711528696));
#33818=CARTESIAN_POINT('Ctrl Pts',(0.885758646200222,4.49363008300228,7.83135981860249));
#33819=CARTESIAN_POINT('Ctrl Pts',(1.63050870544808,4.28003750727018,7.80490252191802));
#33820=CARTESIAN_POINT('Ctrl Pts',(2.27882413510697,3.90134876747149,7.77844522523355));
#33821=CARTESIAN_POINT('Ctrl Pts',(2.92713956476585,3.52266002767282,7.75198792854908));
#33822=CARTESIAN_POINT('Ctrl Pts',(3.47902036483576,2.97887512380756,7.72553063186463));
#33823=CARTESIAN_POINT('Ctrl Pts',(3.8672480646519,2.33622645534278,7.69907333518016));
#33824=CARTESIAN_POINT('Ctrl Pts',(4.25547576446805,1.69357778687799,7.67261603849569));
#33825=CARTESIAN_POINT('Ctrl Pts',(4.48005036403042,0.952065353813674,7.64615874181121));
#33826=CARTESIAN_POINT('Ctrl Pts',(4.51361892565605,0.202004549842097,7.61970144512674));
#33827=CARTESIAN_POINT('Ctrl Pts',(4.51662938451667,0.134738420941428,7.61732873091515));
#33828=CARTESIAN_POINT('Ctrl Pts',(4.51810364598245,0.0674035403653694,
7.61495601670356));
#33829=CARTESIAN_POINT('Ctrl Pts',(4.51805554098247,6.65521552928316E-5,
7.61258330249197));
#33830=CARTESIAN_POINT('Origin',(0.,0.,20.5));
#33831=CARTESIAN_POINT('',(4.51756917096255,-0.000106270599391639,6.61258330249198));
#33832=CARTESIAN_POINT('',(4.5178629555887,0.000109594847417262,6.88741669750807));
#33833=CARTESIAN_POINT('',(4.51775,5.53264807684796E-16,20.5));
#33834=CARTESIAN_POINT('Ctrl Pts',(4.5178629555887,0.000109594847417262,
6.88741669750807));
#33835=CARTESIAN_POINT('Ctrl Pts',(4.51800230500779,0.137343923060939,6.89225174758228));
#33836=CARTESIAN_POINT('Ctrl Pts',(4.5118734339612,0.274565850873291,6.89708679765648));
#33837=CARTESIAN_POINT('Ctrl Pts',(4.4993855978694,0.411206621885887,6.90192184773068));
#33838=CARTESIAN_POINT('Ctrl Pts',(4.43105241013461,1.15890217051388,6.92837914441515));
#33839=CARTESIAN_POINT('Ctrl Pts',(4.17231550636749,1.88919639463632,6.95483644109962));
#33840=CARTESIAN_POINT('Ctrl Pts',(3.75468875509468,2.51314026599451,6.98129373778408));
#33841=CARTESIAN_POINT('Ctrl Pts',(3.33706200382187,3.13708413735269,7.00775103446855));
#33842=CARTESIAN_POINT('Ctrl Pts',(2.76054540504339,3.6546776559466,7.03420833115302));
#33843=CARTESIAN_POINT('Ctrl Pts',(2.09535804244149,4.00287850404845,7.06066562783749));
#33844=CARTESIAN_POINT('Ctrl Pts',(1.4301706798396,4.35107935215029,7.08712292452196));
#33845=CARTESIAN_POINT('Ctrl Pts',(0.676312553414283,4.52988752976006,7.11358022120642));
#33846=CARTESIAN_POINT('Ctrl Pts',(-0.074397251354124,4.51752439873747,
7.14003751789089));
#33847=CARTESIAN_POINT('Ctrl Pts',(-0.82510705612252,4.50516126771487,7.16649481457536));
#33848=CARTESIAN_POINT('Ctrl Pts',(-1.57266853923404,4.30162682805993,7.19295211125983));
#33849=CARTESIAN_POINT('Ctrl Pts',(-2.22602953939534,3.93171134926469,7.2194094079443));
#33850=CARTESIAN_POINT('Ctrl Pts',(-2.87939053955664,3.56179587046945,7.24586670462877));
#33851=CARTESIAN_POINT('Ctrl Pts',(-3.43855105676772,3.0254993525339,7.27232400131323));
#33852=CARTESIAN_POINT('Ctrl Pts',(-3.83540595887268,2.38814211780651,7.2987812979977));
#33853=CARTESIAN_POINT('Ctrl Pts',(-4.23226086097764,1.7507848830791,7.32523859468216));
#33854=CARTESIAN_POINT('Ctrl Pts',(-4.46681014797648,1.01236693155982,7.35169589136664));
#33855=CARTESIAN_POINT('Ctrl Pts',(-4.51048597629575,0.26282675251353,7.37815318805111));
#33856=CARTESIAN_POINT('Ctrl Pts',(-4.55416180461501,-0.486713426532748,
7.40461048473557));
#33857=CARTESIAN_POINT('Ctrl Pts',(-4.40696417425471,-1.24737583310602,
7.43106778142003));
#33858=CARTESIAN_POINT('Ctrl Pts',(-4.08682159368453,-1.92651262793454,
7.4575250781045));
#33859=CARTESIAN_POINT('Ctrl Pts',(-3.76667901311434,-2.60564942276306,
7.48398237478897));
#33860=CARTESIAN_POINT('Ctrl Pts',(-3.27359148233425,-3.20326060584682,
7.51043967147344));
#33861=CARTESIAN_POINT('Ctrl Pts',(-2.66761651687792,-3.64655779648116,
7.53689696815791));
#33862=CARTESIAN_POINT('Ctrl Pts',(-2.06164155142159,-4.0898549871155,7.56335426484238));
#33863=CARTESIAN_POINT('Ctrl Pts',(-1.342779151289,-4.37883818530042,7.58981156152685));
#33864=CARTESIAN_POINT('Ctrl Pts',(-0.59858596122885,-4.47830955732374,
7.61626885821132));
#33865=CARTESIAN_POINT('Ctrl Pts',(0.145607228831289,-4.57778092934705,
7.64272615489578));
#33866=CARTESIAN_POINT('Ctrl Pts',(0.915131208818995,-4.48774047520876,
7.66918345158024));
#33867=CARTESIAN_POINT('Ctrl Pts',(1.61625880962798,-4.21915502257233,7.69564074826471));
#33868=CARTESIAN_POINT('Ctrl Pts',(2.31738641043699,-3.95056956993589,7.72209804494918));
#33869=CARTESIAN_POINT('Ctrl Pts',(2.95011763206728,-3.5034391188013,7.74855534163365));
#33870=CARTESIAN_POINT('Ctrl Pts',(3.43738651198769,-2.93222366326352,7.77501263831812));
#33871=CARTESIAN_POINT('Ctrl Pts',(3.92465539190809,-2.36100820772573,7.80146993500259));
#33872=CARTESIAN_POINT('Ctrl Pts',(4.2664619301186,-1.66570774778476,7.82792723168706));
#33873=CARTESIAN_POINT('Ctrl Pts',(4.42117446855315,-0.931009109950678,
7.85438452837153));
#33874=CARTESIAN_POINT('Ctrl Pts',(4.4855611265208,-0.625249858747316,7.86539525141704));
#33875=CARTESIAN_POINT('Ctrl Pts',(4.51754363682092,-0.312666955391513,
7.87640597446256));
#33876=CARTESIAN_POINT('Ctrl Pts',(4.51740628246061,-5.63430382605529E-5,
7.88741669750807));
#33877=CARTESIAN_POINT('Ctrl Pts',(4.51805554098247,6.65521552928316E-5,
7.61258330249197));
#33878=CARTESIAN_POINT('Ctrl Pts',(4.51756724414766,-0.683447390694716,
7.58849872001909));
#33879=CARTESIAN_POINT('Ctrl Pts',(4.36022097756292,-1.36717849491845,7.56441413754622));
#33880=CARTESIAN_POINT('Ctrl Pts',(4.06048220709641,-1.98142521687064,7.54032955507335));
#33881=CARTESIAN_POINT('Ctrl Pts',(3.73121440322227,-2.65618500473295,7.51387225838888));
#33882=CARTESIAN_POINT('Ctrl Pts',(3.23011627178511,-3.24709540557874,7.48741496170441));
#33883=CARTESIAN_POINT('Ctrl Pts',(2.61822101061302,-3.68218418656399,7.46095766501995));
#33884=CARTESIAN_POINT('Ctrl Pts',(2.00632574944092,-4.11727296754925,7.43450036833548));
#33885=CARTESIAN_POINT('Ctrl Pts',(1.28363335853389,-4.39654012867397,7.40804307165101));
#33886=CARTESIAN_POINT('Ctrl Pts',(0.538166971278164,-4.48597123878683,
7.38158577496654));
#33887=CARTESIAN_POINT('Ctrl Pts',(-0.207299415977548,-4.57540234889969,
7.35512847828207));
#33888=CARTESIAN_POINT('Ctrl Pts',(-0.975539799581951,-4.47499740800071,
7.3286711815976));
#33889=CARTESIAN_POINT('Ctrl Pts',(-1.67298335104765,-4.1969856267701,7.30221388491313));
#33890=CARTESIAN_POINT('Ctrl Pts',(-2.37042690251334,-3.91897384553948,
7.27575658822867));
#33891=CARTESIAN_POINT('Ctrl Pts',(-2.99707362184033,-3.46335522397723,
7.2492992915442));
#33892=CARTESIAN_POINT('Ctrl Pts',(-3.47659863214408,-2.88562360594227,
7.22284199485973));
#33893=CARTESIAN_POINT('Ctrl Pts',(-3.95612364244783,-2.30789198790732,
7.19638469817527));
#33894=CARTESIAN_POINT('Ctrl Pts',(-4.28852694372834,-1.60804737339967,
7.1699274014908));
#33895=CARTESIAN_POINT('Ctrl Pts',(-4.43332218177076,-0.871330061926449,
7.14347010480633));
#33896=CARTESIAN_POINT('Ctrl Pts',(-4.57811741981318,-0.134612750453221,
7.11701280812186));
#33897=CARTESIAN_POINT('Ctrl Pts',(-4.53530459461751,0.63897725798557,7.09055551143739));
#33898=CARTESIAN_POINT('Ctrl Pts',(-4.31009826091029,1.3552175565183,7.06409821475293));
#33899=CARTESIAN_POINT('Ctrl Pts',(-4.08489192720307,2.07145785505103,7.03764091806846));
#33900=CARTESIAN_POINT('Ctrl Pts',(-3.67729208498431,2.7303484436777,7.01118362138399));
#33901=CARTESIAN_POINT('Ctrl Pts',(-3.13694394393276,3.25163717791837,6.98472632469952));
#33902=CARTESIAN_POINT('Ctrl Pts',(-2.59659580288121,3.77292591215904,6.95826902801505));
#33903=CARTESIAN_POINT('Ctrl Pts',(-1.92349936299689,4.15661279201372,6.93181173133059));
#33904=CARTESIAN_POINT('Ctrl Pts',(-1.19963702572085,4.35596518015434,6.90535443464612));
#33905=CARTESIAN_POINT('Ctrl Pts',(-0.475774688444814,4.55531756829496,
6.87889713796165));
#33906=CARTESIAN_POINT('Ctrl Pts',(0.298853546222961,4.57033546472154,6.85243984127718));
#33907=CARTESIAN_POINT('Ctrl Pts',(1.02989881660515,4.39918970627009,6.82598254459271));
#33908=CARTESIAN_POINT('Ctrl Pts',(1.76094408698735,4.22804394781863,6.79952524790824));
#33909=CARTESIAN_POINT('Ctrl Pts',(2.44840639308396,3.87073453448917,6.77306795122378));
#33910=CARTESIAN_POINT('Ctrl Pts',(3.00855358684847,3.37078135737971,6.74661065453931));
#33911=CARTESIAN_POINT('Ctrl Pts',(3.56870078061298,2.87082818027025,6.72015335785485));
#33912=CARTESIAN_POINT('Ctrl Pts',(4.00153286204536,2.22823123938082,6.69369606117038));
#33913=CARTESIAN_POINT('Ctrl Pts',(4.25433136265593,1.52125813092963,6.66723876448591));
#33914=CARTESIAN_POINT('Ctrl Pts',(4.42840834170919,1.03443663992461,6.6490202771546));
#33915=CARTESIAN_POINT('Ctrl Pts',(4.51711887209743,0.517089928133967,6.63080178982329));
#33916=CARTESIAN_POINT('Ctrl Pts',(4.51756917096255,-0.000106270599391639,
6.61258330249198));
#33917=CARTESIAN_POINT('Origin',(0.,0.,20.5));
#33918=CARTESIAN_POINT('',(4.51761916309611,0.000112359330087797,5.61258330249198));
#33919=CARTESIAN_POINT('',(4.51777856404949,-0.00011613542669066,5.88741669750807));
#33920=CARTESIAN_POINT('',(4.51775,5.53264807684796E-16,20.5));
#33921=CARTESIAN_POINT('Ctrl Pts',(4.51777856404949,-0.00011613542669066,
5.88741669750807));
#33922=CARTESIAN_POINT('Ctrl Pts',(4.51717292408202,0.586903980160037,5.90809752070199));
#33923=CARTESIAN_POINT('Ctrl Pts',(4.40219918284471,1.17415437942607,5.92877834389592));
#33924=CARTESIAN_POINT('Ctrl Pts',(4.17916749942524,1.71700921836349,5.94945916708984));
#33925=CARTESIAN_POINT('Ctrl Pts',(3.89383962040738,2.41149180233464,5.97591646377431));
#33926=CARTESIAN_POINT('Ctrl Pts',(3.43165892348727,3.03331448007484,6.00237376045877));
#33927=CARTESIAN_POINT('Ctrl Pts',(2.84891850603996,3.50673993762589,6.02883105714324));
#33928=CARTESIAN_POINT('Ctrl Pts',(2.26617808859264,3.98016539517695,6.05528835382771));
#33929=CARTESIAN_POINT('Ctrl Pts',(1.56287795061812,4.30519363253886,6.08174565051218));
#33930=CARTESIAN_POINT('Ctrl Pts',(0.82467927055748,4.44223657011985,6.10820294719664));
#33931=CARTESIAN_POINT('Ctrl Pts',(0.086480590496836,4.57927950770083,6.13466024388111));
#33932=CARTESIAN_POINT('Ctrl Pts',(-0.686616631649936,4.5283371455009,6.16111754056558));
#33933=CARTESIAN_POINT('Ctrl Pts',(-1.4004500098362,4.29561420685648,6.18757483725005));
#33934=CARTESIAN_POINT('Ctrl Pts',(-2.11428338802246,4.06289126821206,6.21403213393451));
#33935=CARTESIAN_POINT('Ctrl Pts',(-2.76885292224821,3.64838775312316,6.24048943061899));
#33936=CARTESIAN_POINT('Ctrl Pts',(-3.28443276767729,3.10258973098363,6.26694672730345));
#33937=CARTESIAN_POINT('Ctrl Pts',(-3.80001261310638,2.5567917088441,6.29340402398792));
#33938=CARTESIAN_POINT('Ctrl Pts',(-4.1766027697388,1.87969917965394,6.31986132067238));
#33939=CARTESIAN_POINT('Ctrl Pts',(-4.36833497328082,1.15378126410905,6.34631861735685));
#33940=CARTESIAN_POINT('Ctrl Pts',(-4.56006717682283,0.427863348564182,
6.37277591404132));
#33941=CARTESIAN_POINT('Ctrl Pts',(-4.56694142727444,-0.346879953335408,
6.39923321072579));
#33942=CARTESIAN_POINT('Ctrl Pts',(-4.38812044853859,-1.07608576485095,
6.42569050741026));
#33943=CARTESIAN_POINT('Ctrl Pts',(-4.20929946980274,-1.80529157636651,
6.45214780409473));
#33944=CARTESIAN_POINT('Ctrl Pts',(-3.84478326187941,-2.48895989749803,
6.4786051007792));
#33945=CARTESIAN_POINT('Ctrl Pts',(-3.33896949547221,-3.04382068336875,
6.50506239746367));
#33946=CARTESIAN_POINT('Ctrl Pts',(-2.83315572906502,-3.59868146923946,
6.53151969414813));
#33947=CARTESIAN_POINT('Ctrl Pts',(-2.18604440417397,-4.02473471984939,
6.55797699083259));
#33948=CARTESIAN_POINT('Ctrl Pts',(-1.47645296399246,-4.27008762080069,
6.58443428751706));
#33949=CARTESIAN_POINT('Ctrl Pts',(-0.766861523810935,-4.51544052175199,
6.61089158420153));
#33950=CARTESIAN_POINT('Ctrl Pts',(0.00521003166104095,-4.58009307304465,
6.637348880886));
#33951=CARTESIAN_POINT('Ctrl Pts',(0.745724241442684,-4.45617066548422,
6.66380617757047));
#33952=CARTESIAN_POINT('Ctrl Pts',(1.48623845122433,-4.3322482579238,6.69026347425494));
#33953=CARTESIAN_POINT('Ctrl Pts',(2.19519531531564,-4.01975089151029,6.7167207709394));
#33954=CARTESIAN_POINT('Ctrl Pts',(2.78624467229499,-3.55674039962227,6.74317806762387));
#33955=CARTESIAN_POINT('Ctrl Pts',(3.37729402927435,-3.09372990773424,6.76963536430834));
#33956=CARTESIAN_POINT('Ctrl Pts',(3.85043587914176,-2.4802062903717,6.79609266099281));
#33957=CARTESIAN_POINT('Ctrl Pts',(4.14804206822422,-1.79089604512366,6.82254995767728));
#33958=CARTESIAN_POINT('Ctrl Pts',(4.39126096128897,-1.22755670280584,6.84417220428754));
#33959=CARTESIAN_POINT('Ctrl Pts',(4.51723978779142,-0.613599558623174,
6.86579445089781));
#33960=CARTESIAN_POINT('Ctrl Pts',(4.5178629555887,0.000109594847417262,
6.88741669750807));
#33961=CARTESIAN_POINT('Ctrl Pts',(4.51756917096255,-0.000106270599391639,
6.61258330249198));
#33962=CARTESIAN_POINT('Ctrl Pts',(4.51777280622788,-0.233994013420898,
6.60434449313882));
#33963=CARTESIAN_POINT('Ctrl Pts',(4.49992676845961,-0.467850975545092,
6.59610568378566));
#33964=CARTESIAN_POINT('Ctrl Pts',(4.46376343532316,-0.698840208967197,
6.5878668744325));
#33965=CARTESIAN_POINT('Ctrl Pts',(4.34763208759105,-1.44061616439985,6.56140957774804));
#33966=CARTESIAN_POINT('Ctrl Pts',(4.04260447233807,-2.15281879925221,6.53495228106357));
#33967=CARTESIAN_POINT('Ctrl Pts',(3.58583261551844,-2.74870262081615,6.5084949843791));
#33968=CARTESIAN_POINT('Ctrl Pts',(3.1290607586988,-3.3445864423801,6.48203768769463));
#33969=CARTESIAN_POINT('Ctrl Pts',(2.52054466031253,-3.82415145065562,6.45558039101016));
#33970=CARTESIAN_POINT('Ctrl Pts',(1.83440090767928,-4.12898715838434,6.42912309432569));
#33971=CARTESIAN_POINT('Ctrl Pts',(1.14825715504604,-4.43382286611306,6.40266579764122));
#33972=CARTESIAN_POINT('Ctrl Pts',(0.384485748165844,-4.56392927329498,
6.37620850095676));
#33973=CARTESIAN_POINT('Ctrl Pts',(-0.363886800892981,-4.50345956352816,
6.34975120427229));
#33974=CARTESIAN_POINT('Ctrl Pts',(-1.11225934995183,-4.44298985376135,
6.32329390758782));
#33975=CARTESIAN_POINT('Ctrl Pts',(-1.84523304118933,-4.19194402704577,
6.29683661090335));
#33976=CARTESIAN_POINT('Ctrl Pts',(-2.47353249021757,-3.78089918723516,
6.27037931421889));
#33977=CARTESIAN_POINT('Ctrl Pts',(-3.10183193924579,-3.36985434742456,
6.24392201753442));
#33978=CARTESIAN_POINT('Ctrl Pts',(-3.62545714606476,-2.79881049451895,
6.21746472084996));
#33979=CARTESIAN_POINT('Ctrl Pts',(-3.98063113999636,-2.13732013781012,
6.19100742416549));
#33980=CARTESIAN_POINT('Ctrl Pts',(-4.33580513392796,-1.47582978110128,
6.16455012748102));
#33981=CARTESIAN_POINT('Ctrl Pts',(-4.52252791497214,-0.723892920589236,
6.13809283079655));
#33982=CARTESIAN_POINT('Ctrl Pts',(-4.51805685504966,0.0269053663076428,
6.11163553411208));
#33983=CARTESIAN_POINT('Ctrl Pts',(-4.51358579512718,0.777703653204501,
6.08517823742761));
#33984=CARTESIAN_POINT('Ctrl Pts',(-4.31792089423804,1.52736336648619,6.05872094074314));
#33985=CARTESIAN_POINT('Ctrl Pts',(-3.95489392076209,2.18457678274683,6.03226364405868));
#33986=CARTESIAN_POINT('Ctrl Pts',(-3.59186694728612,2.84179019900748,6.00580634737421));
#33987=CARTESIAN_POINT('Ctrl Pts',(-3.06147790122333,3.40655731824708,5.97934905068974));
#33988=CARTESIAN_POINT('Ctrl Pts',(-2.42832758138604,3.81009013038763,5.95289175400527));
#33989=CARTESIAN_POINT('Ctrl Pts',(-1.79517726154877,4.21362294252816,5.9264344573208));
#33990=CARTESIAN_POINT('Ctrl Pts',(-1.05926566793702,4.45592144756967,5.89997716063634));
#33991=CARTESIAN_POINT('Ctrl Pts',(-0.310226018196338,4.50747395575742,
5.87351986395187));
#33992=CARTESIAN_POINT('Ctrl Pts',(0.438813631544363,4.55902646394516,5.8470625672674));
#33993=CARTESIAN_POINT('Ctrl Pts',(1.20098133741399,4.41983297527914,5.82060527058293));
#33994=CARTESIAN_POINT('Ctrl Pts',(1.88344591635241,4.10684710262907,5.79414797389846));
#33995=CARTESIAN_POINT('Ctrl Pts',(2.56591049529081,3.79386122997902,5.767690677214));
#33996=CARTESIAN_POINT('Ctrl Pts',(3.16867194729802,3.30708297334494,5.74123338052953));
#33997=CARTESIAN_POINT('Ctrl Pts',(3.61831459461448,2.70580138565218,5.71477608384506));
#33998=CARTESIAN_POINT('Ctrl Pts',(4.06795724193093,2.10451979795941,5.68831878716059));
#33999=CARTESIAN_POINT('Ctrl Pts',(4.36448108455665,1.38873487920795,5.66186149047613));
#34000=CARTESIAN_POINT('Ctrl Pts',(4.47176984663199,0.645628440320207,5.63540419379166));
#34001=CARTESIAN_POINT('Ctrl Pts',(4.50261735669319,0.431971549265432,5.6277972300251));
#34002=CARTESIAN_POINT('Ctrl Pts',(4.51782138536506,0.216056072273327,5.62019026625854));
#34003=CARTESIAN_POINT('Ctrl Pts',(4.51761916309611,0.000112359330087797,
5.61258330249198));
#34004=CARTESIAN_POINT('Origin',(0.,0.,20.5));
#34005=CARTESIAN_POINT('',(4.51801297056466,-8.08487039419617E-5,4.61258330249197));
#34006=CARTESIAN_POINT('',(4.51744953111884,7.68816669171638E-5,4.88741669750807));
#34007=CARTESIAN_POINT('',(4.51775,5.53264807684796E-16,20.5));
#34008=CARTESIAN_POINT('Ctrl Pts',(4.51744953111884,7.68816669171638E-5,
4.88741669750807));
#34009=CARTESIAN_POINT('Ctrl Pts',(4.51762304095457,0.28595126409645,4.89748599713724));
#34010=CARTESIAN_POINT('Ctrl Pts',(4.49090928481679,0.571793625338861,4.90755529676642));
#34011=CARTESIAN_POINT('Ctrl Pts',(4.43699864797727,0.852411075740623,4.91762459639559));
#34012=CARTESIAN_POINT('Ctrl Pts',(4.2953473151299,1.58973933227679,4.94408189308006));
#34013=CARTESIAN_POINT('Ctrl Pts',(3.96593233939643,2.29099550010712,4.97053918976452));
#34014=CARTESIAN_POINT('Ctrl Pts',(3.48887610024735,2.87076735409198,4.99699648644899));
#34015=CARTESIAN_POINT('Ctrl Pts',(3.01181986109827,3.45053920807684,5.02345378313346));
#34016=CARTESIAN_POINT('Ctrl Pts',(2.38712235853358,3.90882674821622,5.04991107981793));
#34017=CARTESIAN_POINT('Ctrl Pts',(1.69087105699343,4.18981105932229,5.0763683765024));
#34018=CARTESIAN_POINT('Ctrl Pts',(0.994619755453274,4.47079537042835,5.10282567318686));
#34019=CARTESIAN_POINT('Ctrl Pts',(0.226814654937662,4.57447645250109,5.12928296987133));
#34020=CARTESIAN_POINT('Ctrl Pts',(-0.519026433064492,4.48822606449115,
5.1557402665558));
#34021=CARTESIAN_POINT('Ctrl Pts',(-1.26486752106665,4.40197567648121,5.18219756324027));
#34022=CARTESIAN_POINT('Ctrl Pts',(-1.98874459655534,4.12579381838858,5.20865485992474));
#34023=CARTESIAN_POINT('Ctrl Pts',(-2.60249023287342,3.69331913486986,5.2351121566092));
#34024=CARTESIAN_POINT('Ctrl Pts',(-3.21623586919149,3.26084445135114,5.26156945329367));
#34025=CARTESIAN_POINT('Ctrl Pts',(-3.71985006633895,2.67207694240634,5.28802674997814));
#34026=CARTESIAN_POINT('Ctrl Pts',(-4.05199317246879,1.99872783901753,5.31448404666261));
#34027=CARTESIAN_POINT('Ctrl Pts',(-4.38413627859864,1.32537873562872,5.34094134334707));
#34028=CARTESIAN_POINT('Ctrl Pts',(-4.54480829371086,0.567448037795898,
5.36739864003154));
#34029=CARTESIAN_POINT('Ctrl Pts',(-4.51443954418554,-0.182749134310455,
5.39385593671601));
#34030=CARTESIAN_POINT('Ctrl Pts',(-4.48407079466022,-0.932946306416809,
5.42031323340048));
#34031=CARTESIAN_POINT('Ctrl Pts',(-4.26266128049735,-1.6754099527967,5.44677053008495));
#34032=CARTESIAN_POINT('Ctrl Pts',(-3.87717843548113,-2.31970882302876,
5.47322782676942));
#34033=CARTESIAN_POINT('Ctrl Pts',(-3.49169559046492,-2.96400769326083,
5.49968512345388));
#34034=CARTESIAN_POINT('Ctrl Pts',(-2.94213941459537,-3.51014178734505,
5.52614242013835));
#34035=CARTESIAN_POINT('Ctrl Pts',(-2.29544524188241,-3.89159257704565,
5.55259971682282));
#34036=CARTESIAN_POINT('Ctrl Pts',(-1.64875106916946,-4.27304336674624,
5.57905701350729));
#34037=CARTESIAN_POINT('Ctrl Pts',(-0.904918899613081,-4.48981085206321,
5.60551431019175));
#34038=CARTESIAN_POINT('Ctrl Pts',(-0.154546668242997,-4.51549299318827,
5.63197160687622));
#34039=CARTESIAN_POINT('Ctrl Pts',(0.595825563127097,-4.54117513431334,
5.65842890356069));
#34040=CARTESIAN_POINT('Ctrl Pts',(1.35273785631093,-4.37577193124651,5.68488620024516));
#34041=CARTESIAN_POINT('Ctrl Pts',(2.02399913169717,-4.03942931106444,5.71134349692963));
#34042=CARTESIAN_POINT('Ctrl Pts',(2.69526040708341,-3.70308669088236,5.73780079361409));
#34043=CARTESIAN_POINT('Ctrl Pts',(3.28087066467206,-3.19580465358505,5.76425809029856));
#34044=CARTESIAN_POINT('Ctrl Pts',(3.70950322320198,-2.57936958989042,5.79071538698303));
#34045=CARTESIAN_POINT('Ctrl Pts',(4.13813578173191,-1.9629345261958,5.8171726836675));
#34046=CARTESIAN_POINT('Ctrl Pts',(4.40979064120311,-1.23734643610387,5.84362998035196));
#34047=CARTESIAN_POINT('Ctrl Pts',(4.49138054038091,-0.490981145956846,
5.87008727703643));
#34048=CARTESIAN_POINT('Ctrl Pts',(4.50919422313609,-0.328025747897277,
5.87586375052698));
#34049=CARTESIAN_POINT('Ctrl Pts',(4.51794772865112,-0.164079924696943,
5.88164022401752));
#34050=CARTESIAN_POINT('Ctrl Pts',(4.51777856404949,-0.00011613542669066,
5.88741669750807));
#34051=CARTESIAN_POINT('Ctrl Pts',(4.51761916309611,0.000112359330087797,
5.61258330249198));
#34052=CARTESIAN_POINT('Ctrl Pts',(4.51711804895781,-0.535004016325972,
5.59373296957407));
#34053=CARTESIAN_POINT('Ctrl Pts',(4.42201232003226,-1.07029377947848,5.57488263665616));
#34054=CARTESIAN_POINT('Ctrl Pts',(4.23591186210463,-1.57181816399948,5.55603230373826));
#34055=CARTESIAN_POINT('Ctrl Pts',(3.97471143397694,-2.27573037040736,5.52957500705379));
#34056=CARTESIAN_POINT('Ctrl Pts',(3.5342568961966,-2.91312682419909,5.50311771036932));
#34057=CARTESIAN_POINT('Ctrl Pts',(2.96819512400045,-3.40637334272939,5.47666041368485));
#34058=CARTESIAN_POINT('Ctrl Pts',(2.4021333518043,-3.89961986125968,5.45020311700038));
#34059=CARTESIAN_POINT('Ctrl Pts',(1.71046434519234,-4.24871644452854,5.42374582031592));
#34060=CARTESIAN_POINT('Ctrl Pts',(0.977432623678222,-4.41114351504991,
5.39728852363145));
#34061=CARTESIAN_POINT('Ctrl Pts',(0.244400902164107,-4.57357058557128,
5.37083122694698));
#34062=CARTESIAN_POINT('Ctrl Pts',(-0.529993534252169,-4.54932814334517,
5.34437393026251));
#34063=CARTESIAN_POINT('Ctrl Pts',(-1.2514303002616,-4.34136889100483,5.31791663357804));
#34064=CARTESIAN_POINT('Ctrl Pts',(-1.97286706627105,-4.1334096386645,5.29145933689358));
#34065=CARTESIAN_POINT('Ctrl Pts',(-2.64134616187366,-3.74173357620994,
5.2650020402091));
#34066=CARTESIAN_POINT('Ctrl Pts',(-3.17544757305171,-3.214046414568,5.23854474352464));
#34067=CARTESIAN_POINT('Ctrl Pts',(-3.70954898422975,-2.68635925292607,
5.21208744684017));
#34068=CARTESIAN_POINT('Ctrl Pts',(-4.10927271098324,-2.02266099209677,
5.1856301501557));
#34069=CARTESIAN_POINT('Ctrl Pts',(-4.32593284578035,-1.3037893457135,5.15917285347124));
#34070=CARTESIAN_POINT('Ctrl Pts',(-4.54259298057747,-0.584917699330228,
5.13271555678677));
#34071=CARTESIAN_POINT('Ctrl Pts',(-4.57618952341819,0.189127332607011,
5.1062582601023));
#34072=CARTESIAN_POINT('Ctrl Pts',(-4.42263045256687,0.924067921868061,
5.07980096341783));
#34073=CARTESIAN_POINT('Ctrl Pts',(-4.26907138171554,1.65900851112912,5.05334366673336));
#34074=CARTESIAN_POINT('Ctrl Pts',(-3.92835669717217,2.35484465771397,5.0268863700489));
#34075=CARTESIAN_POINT('Ctrl Pts',(-3.44198507043455,2.92682428907221,5.00042907336443));
#34076=CARTESIAN_POINT('Ctrl Pts',(-2.95561344369694,3.49880392043043,4.97397177667996));
#34077=CARTESIAN_POINT('Ctrl Pts',(-2.3235848747651,3.94692703656203,4.9475144799955));
#34078=CARTESIAN_POINT('Ctrl Pts',(-1.62287974384915,4.21661273787403,4.92105718331103));
#34079=CARTESIAN_POINT('Ctrl Pts',(-0.922174612933183,4.48629843918604,
4.89459988662656));
#34080=CARTESIAN_POINT('Ctrl Pts',(-0.152792920033106,4.57754672567842,
4.86814258994209));
#34081=CARTESIAN_POINT('Ctrl Pts',(0.591555496154586,4.47924365704375,4.84168529325762));
#34082=CARTESIAN_POINT('Ctrl Pts',(1.33590391234227,4.38094058840908,4.81522799657315));
#34083=CARTESIAN_POINT('Ctrl Pts',(2.05521905181757,4.09308616464735,4.78877069988869));
#34084=CARTESIAN_POINT('Ctrl Pts',(2.66188912668092,3.65074073599527,4.76231340320422));
#34085=CARTESIAN_POINT('Ctrl Pts',(3.26855920154427,3.20839530734318,4.73585610651975));
#34086=CARTESIAN_POINT('Ctrl Pts',(3.76258421179568,2.61155887380074,4.70939880983528));
#34087=CARTESIAN_POINT('Ctrl Pts',(4.08379245793942,1.93292545243589,4.68294151315081));
#34088=CARTESIAN_POINT('Ctrl Pts',(4.36852345568096,1.33135941704992,4.65948877626453));
#34089=CARTESIAN_POINT('Ctrl Pts',(4.51746001083452,0.665519661321642,4.63603603937825));
#34090=CARTESIAN_POINT('Ctrl Pts',(4.51801297056466,-8.08487039419617E-5,
4.61258330249197));
#34091=CARTESIAN_POINT('Origin',(0.,0.,20.5));
#34092=CARTESIAN_POINT('',(4.51736370604735,1.02551535238581E-5,3.61258330249198));
#34093=CARTESIAN_POINT('',(4.51813206731963,-1.62797693238861E-5,3.88741669750807));
#34094=CARTESIAN_POINT('',(4.51775,5.53264807684796E-16,20.5));
#34095=CARTESIAN_POINT('Ctrl Pts',(4.51813206731963,-1.62797693238861E-5,
3.88741669750807));
#34096=CARTESIAN_POINT('Ctrl Pts',(4.51798177204935,0.735410282480124,3.91333177025696));
#34097=CARTESIAN_POINT('Ctrl Pts',(4.33483992986086,1.47090898249386,3.93924684300585));
#34098=CARTESIAN_POINT('Ctrl Pts',(3.98971201192936,2.12032066114161,3.96516191575474));
#34099=CARTESIAN_POINT('Ctrl Pts',(3.63736294436994,2.78332005222287,3.99161921243921));
#34100=CARTESIAN_POINT('Ctrl Pts',(3.11617838217547,3.35659231850456,4.01807650912368));
#34101=CARTESIAN_POINT('Ctrl Pts',(2.48963802820999,3.77031353241187,4.04453380580815));
#34102=CARTESIAN_POINT('Ctrl Pts',(1.86309767424454,4.18403474631916,4.07099110249262));
#34103=CARTESIAN_POINT('Ctrl Pts',(1.13120152850809,4.4382049078521,4.09744839917709));
#34104=CARTESIAN_POINT('Ctrl Pts',(0.383093731539025,4.50186637263401,4.12390569586155));
#34105=CARTESIAN_POINT('Ctrl Pts',(-0.365014065430051,4.56552783741592,
4.15036299254602));
#34106=CARTESIAN_POINT('Ctrl Pts',(-1.12933351363175,4.43868060544681,4.17682028923049));
#34107=CARTESIAN_POINT('Ctrl Pts',(-1.81677135017129,4.13677452919472,4.20327758591496));
#34108=CARTESIAN_POINT('Ctrl Pts',(-2.50420918671083,3.83486845294263,4.22973488259942));
#34109=CARTESIAN_POINT('Ctrl Pts',(-3.11476541158823,3.35790353240755,4.25619217928389));
#34110=CARTESIAN_POINT('Ctrl Pts',(-3.57407495233505,2.7639735670387,4.28264947596836));
#34111=CARTESIAN_POINT('Ctrl Pts',(-4.03338449308186,2.17004360166985,4.30910677265283));
#34112=CARTESIAN_POINT('Ctrl Pts',(-4.3414473496981,1.45914859146723,4.3355640693373));
#34113=CARTESIAN_POINT('Ctrl Pts',(-4.4607418071907,0.717874761903797,4.36202136602176));
#34114=CARTESIAN_POINT('Ctrl Pts',(-4.5800362646833,-0.0233990676596439,
4.38847866270623));
#34115=CARTESIAN_POINT('Ctrl Pts',(-4.51056232305225,-0.795051716583895,
4.4149359593907));
#34116=CARTESIAN_POINT('Ctrl Pts',(-4.26078183149923,-1.50309674624206,
4.44139325607517));
#34117=CARTESIAN_POINT('Ctrl Pts',(-4.01100133994621,-2.21114177590023,
4.46785055275963));
#34118=CARTESIAN_POINT('Ctrl Pts',(-3.58091429847122,-2.85557918629231,
4.4943078494441));
#34119=CARTESIAN_POINT('Ctrl Pts',(-3.02290483273516,-3.35791721405156,
4.52076514612857));
#34120=CARTESIAN_POINT('Ctrl Pts',(-2.4648953669991,-3.86025524181081,4.54722244281304));
#34121=CARTESIAN_POINT('Ctrl Pts',(-1.77896347700197,-4.22049388693723,
4.57367973949751));
#34122=CARTESIAN_POINT('Ctrl Pts',(-1.04865490780318,-4.39475648114178,
4.60013703618198));
#34123=CARTESIAN_POINT('Ctrl Pts',(-0.318346338604368,-4.56901907534634,
4.62659433286644));
#34124=CARTESIAN_POINT('Ctrl Pts',(0.456338909796113,-4.55730561862902,
4.65305162955091));
#34125=CARTESIAN_POINT('Ctrl Pts',(1.18104503151144,-4.36104279705434,4.67950892623538));
#34126=CARTESIAN_POINT('Ctrl Pts',(1.90575115322676,-4.16477997547966,4.70596622291985));
#34127=CARTESIAN_POINT('Ctrl Pts',(2.58047814825693,-3.78396778904763,4.73242351960431));
#34128=CARTESIAN_POINT('Ctrl Pts',(3.1230450153487,-3.26498874060892,4.75888081628878));
#34129=CARTESIAN_POINT('Ctrl Pts',(3.66561188244045,-2.74600969217023,4.78533811297325));
#34130=CARTESIAN_POINT('Ctrl Pts',(4.07601862159381,-2.08886378172488,4.81179540965772));
#34131=CARTESIAN_POINT('Ctrl Pts',(4.30427814618986,-1.37359065388121,4.83825270634219));
#34132=CARTESIAN_POINT('Ctrl Pts',(4.4456650936749,-0.930541084129997,4.85464070339748));
#34133=CARTESIAN_POINT('Ctrl Pts',(4.51716714020965,-0.465189691975021,
4.87102870045278));
#34134=CARTESIAN_POINT('Ctrl Pts',(4.51744953111884,7.68816669171638E-5,
4.88741669750807));
#34135=CARTESIAN_POINT('Ctrl Pts',(4.51801297056466,-8.08487039419617E-5,
4.61258330249197));
#34136=CARTESIAN_POINT('Ctrl Pts',(4.51808381093537,-0.0853517722542952,
4.60957874269379));
#34137=CARTESIAN_POINT('Ctrl Pts',(4.51571930609417,-0.170618769185437,
4.6065741828956));
#34138=CARTESIAN_POINT('Ctrl Pts',(4.51089298576516,-0.255746192878958,
4.60356962309741));
#34139=CARTESIAN_POINT('Ctrl Pts',(4.46839378541107,-1.00535400764169,4.57711232641294));
#34140=CARTESIAN_POINT('Ctrl Pts',(4.23500390266681,-1.74413922797991,4.55065502972848));
#34141=CARTESIAN_POINT('Ctrl Pts',(3.83914996695076,-2.38211863169309,4.52419773304401));
#34142=CARTESIAN_POINT('Ctrl Pts',(3.44329603123471,-3.02009803540626,4.49774043635954));
#34143=CARTESIAN_POINT('Ctrl Pts',(2.88497804254688,-3.55727162249439,4.47128313967507));
#34144=CARTESIAN_POINT('Ctrl Pts',(2.23219851400147,-3.92821224455693,4.4448258429906));
#34145=CARTESIAN_POINT('Ctrl Pts',(1.57941898545608,-4.29915286661947,4.41836854630613));
#34146=CARTESIAN_POINT('Ctrl Pts',(0.832177917053118,-4.50386052365641,
4.39191124962167));
#34147=CARTESIAN_POINT('Ctrl Pts',(0.0814884439290546,-4.51740204959703,
4.3654539529372));
#34148=CARTESIAN_POINT('Ctrl Pts',(-0.66920102919502,-4.53094357553764,
4.33899665625273));
#34149=CARTESIAN_POINT('Ctrl Pts',(-1.42333890704021,-4.35331897038192,
4.31253935956826));
#34150=CARTESIAN_POINT('Ctrl Pts',(-2.08907203071289,-4.00616271445513,
4.28608206288379));
#34151=CARTESIAN_POINT('Ctrl Pts',(-2.75480515438558,-3.65900645852834,
4.25962476619933));
#34152=CARTESIAN_POINT('Ctrl Pts',(-3.33213352388578,-3.14231855183048,
4.23316746951486));
#34153=CARTESIAN_POINT('Ctrl Pts',(-3.75073918275569,-2.51903100956272,
4.20671017283039));
#34154=CARTESIAN_POINT('Ctrl Pts',(-4.1693448416256,-1.89574346729495,4.18025287614593));
#34155=CARTESIAN_POINT('Ctrl Pts',(-4.42922778986523,-1.16585628945725,
4.15379557946146));
#34156=CARTESIAN_POINT('Ctrl Pts',(-4.49873457199956,-0.418268926521358,
4.12733828277699));
#34157=CARTESIAN_POINT('Ctrl Pts',(-4.56824135413388,0.329318436414523,
4.10088098609252));
#34158=CARTESIAN_POINT('Ctrl Pts',(-4.44737197016292,1.0946059844486,4.07442368940805));
#34159=CARTESIAN_POINT('Ctrl Pts',(-4.1508481772844,1.78438254119798,4.04796639272359));
#34160=CARTESIAN_POINT('Ctrl Pts',(-3.85432438440588,2.47415909794737,4.02150909603912));
#34161=CARTESIAN_POINT('Ctrl Pts',(-3.3821461826198,3.08842466341204,3.99505179935465));
#34162=CARTESIAN_POINT('Ctrl Pts',(-2.79182435432936,3.55236237154529,3.96859450267018));
#34163=CARTESIAN_POINT('Ctrl Pts',(-2.20150252603891,4.01630007967853,3.94213720598571));
#34164=CARTESIAN_POINT('Ctrl Pts',(-1.49303707124409,4.32990993048035,3.91567990930125));
#34165=CARTESIAN_POINT('Ctrl Pts',(-0.752718298258071,4.45499459120489,
3.88922261261678));
#34166=CARTESIAN_POINT('Ctrl Pts',(-0.0123995252720613,4.58007925192944,
3.86276531593231));
#34167=CARTESIAN_POINT('Ctrl Pts',(0.759772565905157,4.51663872257671,3.83630801924784));
#34168=CARTESIAN_POINT('Ctrl Pts',(1.46974826915516,4.27239998941026,3.80985072256337));
#34169=CARTESIAN_POINT('Ctrl Pts',(2.17972397240517,4.02816125624381,3.78339342587891));
#34170=CARTESIAN_POINT('Ctrl Pts',(2.82750328772796,3.60312431926363,3.75693612919444));
#34171=CARTESIAN_POINT('Ctrl Pts',(3.33418741143483,3.04905820699226,3.73047883250997));
#34172=CARTESIAN_POINT('Ctrl Pts',(3.84087153514169,2.49499209472089,3.7040215358255));
#34173=CARTESIAN_POINT('Ctrl Pts',(4.20646046723263,1.81189680715833,3.67756423914103));
#34174=CARTESIAN_POINT('Ctrl Pts',(4.38642588038764,1.08297259432681,3.65110694245657));
#34175=CARTESIAN_POINT('Ctrl Pts',(4.47377321176399,0.729184698918257,3.63826572913504));
#34176=CARTESIAN_POINT('Ctrl Pts',(4.51739308950363,0.364600853640814,3.62542451581351));
#34177=CARTESIAN_POINT('Ctrl Pts',(4.51736430815743,1.02391689833781E-5,
3.61258330249198));
#34178=CARTESIAN_POINT('Origin',(0.,0.,20.5));
#34179=CARTESIAN_POINT('',(4.51806423128285,6.30519293007281E-5,2.61258330249198));
#34180=CARTESIAN_POINT('',(4.5174009456275,-5.29814202112051E-5,2.88741669750807));
#34181=CARTESIAN_POINT('',(4.51775,5.53264807684796E-16,20.5));
#34182=CARTESIAN_POINT('Ctrl Pts',(4.5174009456275,-5.29814202112051E-5,
2.88741669750807));
#34183=CARTESIAN_POINT('Ctrl Pts',(4.5172216944486,0.434438744202657,2.90272024669221));
#34184=CARTESIAN_POINT('Ctrl Pts',(4.45500169120217,0.868980727030553,2.91802379587635));
#34185=CARTESIAN_POINT('Ctrl Pts',(4.33145501462215,1.28532451174868,2.9333273450605));
#34186=CARTESIAN_POINT('Ctrl Pts',(4.11786331525058,2.00511381699269,2.95978464174497));
#34187=CARTESIAN_POINT('Ctrl Pts',(3.72097433835707,2.67051112625836,2.98624193842943));
#34188=CARTESIAN_POINT('Ctrl Pts',(3.18912872207782,3.2004717836931,3.0126992351139));
#34189=CARTESIAN_POINT('Ctrl Pts',(2.65728310579859,3.73043244112782,3.03915653179837));
#34190=CARTESIAN_POINT('Ctrl Pts',(1.99048085013363,4.12495644673162,3.06561382848284));
#34191=CARTESIAN_POINT('Ctrl Pts',(1.26993773185205,4.33599121325399,3.0920711251673));
#34192=CARTESIAN_POINT('Ctrl Pts',(0.54939461357047,4.54702597977637,3.11852842185177));
#34193=CARTESIAN_POINT('Ctrl Pts',(-0.22488936732773,4.57457150721731,3.14498571853624));
#34194=CARTESIAN_POINT('Ctrl Pts',(-0.958607278893408,4.41527278082,3.17144301522071));
#34195=CARTESIAN_POINT('Ctrl Pts',(-1.69232519045908,4.25597405442269,3.19790031190518));
#34196=CARTESIAN_POINT('Ctrl Pts',(-2.38547703269224,3.90983107418713,3.22435760858964));
#34197=CARTESIAN_POINT('Ctrl Pts',(-2.95363767834166,3.41900367201878,3.25081490527411));
#34198=CARTESIAN_POINT('Ctrl Pts',(-3.52179832399109,2.92817626985041,3.27727220195858));
#34199=CARTESIAN_POINT('Ctrl Pts',(-3.96496777305678,2.29266444574925,3.30372949864305));
#34200=CARTESIAN_POINT('Ctrl Pts',(-4.229168477112,1.58987283655001,3.33018679532752));
#34201=CARTESIAN_POINT('Ctrl Pts',(-4.49336918116721,0.887081227350804,
3.35664409201199));
#34202=CARTESIAN_POINT('Ctrl Pts',(-4.57860114021196,0.117009833053533,
3.38310138869645));
#34203=CARTESIAN_POINT('Ctrl Pts',(-4.47448319596347,-0.62654750277845,
3.40955868538092));
#34204=CARTESIAN_POINT('Ctrl Pts',(-4.37036525171498,-1.37010483861044,
3.43601598206539));
#34205=CARTESIAN_POINT('Ctrl Pts',(-4.07689740417324,-2.08714811597715,
3.46247327874986));
#34206=CARTESIAN_POINT('Ctrl Pts',(-3.62982371237881,-2.69034225726949,
3.48893057543432));
#34207=CARTESIAN_POINT('Ctrl Pts',(-3.18275002058438,-3.29353639856183,
3.51538787211879));
#34208=CARTESIAN_POINT('Ctrl Pts',(-2.58207048453726,-3.7828814037798,3.54184516880326));
#34209=CARTESIAN_POINT('Ctrl Pts',(-1.90094720693718,-4.09877559286125,
3.56830246548773));
#34210=CARTESIAN_POINT('Ctrl Pts',(-1.2198239293371,-4.41466978194271,3.59475976217219));
#34211=CARTESIAN_POINT('Ctrl Pts',(-0.45825691018407,-4.55711315488765,
3.62121705885666));
#34212=CARTESIAN_POINT('Ctrl Pts',(0.290995830439079,-4.5087562665179,3.64767435554113));
#34213=CARTESIAN_POINT('Ctrl Pts',(1.04024857106223,-4.46039937814816,3.6741316522256));
#34214=CARTESIAN_POINT('Ctrl Pts',(1.77718703315549,-4.22124222846373,3.70058894891007));
#34215=CARTESIAN_POINT('Ctrl Pts',(2.41205292762872,-3.8204138936135,3.72704624559453));
#34216=CARTESIAN_POINT('Ctrl Pts',(3.04691882210195,-3.41958555876328,3.753503542279));
#34217=CARTESIAN_POINT('Ctrl Pts',(3.57971214895514,-2.85708603874726,3.77996083896347));
#34218=CARTESIAN_POINT('Ctrl Pts',(3.94553927063659,-2.2014271525676,3.80641813564794));
#34219=CARTESIAN_POINT('Ctrl Pts',(4.31136639231804,-1.54576826638794,3.83287543233241));
#34220=CARTESIAN_POINT('Ctrl Pts',(4.51022730882776,-0.796950014044647,
3.85933272901687));
#34221=CARTESIAN_POINT('Ctrl Pts',(4.51790098062045,-0.0461776299325883,
3.88579002570134));
#34222=CARTESIAN_POINT('Ctrl Pts',(4.51805824719871,-0.0307910709167367,
3.88633224963692));
#34223=CARTESIAN_POINT('Ctrl Pts',(4.5181352119642,-0.0154036911331415,
3.88687447357249));
#34224=CARTESIAN_POINT('Ctrl Pts',(4.51813206731963,-1.62797693238861E-5,
3.88741669750807));
#34225=CARTESIAN_POINT('Ctrl Pts',(4.51736430815743,1.02391689833781E-5,
3.61258330249198));
#34226=CARTESIAN_POINT('Ctrl Pts',(4.51733379007481,-0.386580659657543,
3.59896721912904));
#34227=CARTESIAN_POINT('Ctrl Pts',(4.46822794652789,-0.773179169265813,
3.5853511357661));
#34228=CARTESIAN_POINT('Ctrl Pts',(4.370140714067,-1.14692274519747,3.57173505240317));
#34229=CARTESIAN_POINT('Ctrl Pts',(4.17954824037228,-1.87314073378976,3.5452777557187));
#34230=CARTESIAN_POINT('Ctrl Pts',(3.80402139876375,-2.55082357287386,3.51882045903423));
#34231=CARTESIAN_POINT('Ctrl Pts',(3.28929894294204,-3.09743024266209,3.49236316234976));
#34232=CARTESIAN_POINT('Ctrl Pts',(2.77457648712035,-3.64403691245031,3.46590586566529));
#34233=CARTESIAN_POINT('Ctrl Pts',(2.12065841708548,-4.05956741294266,3.43944856898082));
#34234=CARTESIAN_POINT('Ctrl Pts',(1.40719123005614,-4.29341058905976,3.41299127229636));
#34235=CARTESIAN_POINT('Ctrl Pts',(0.693724043026795,-4.52725376517686,
3.38653397561189));
#34236=CARTESIAN_POINT('Ctrl Pts',(-0.0792922609970231,-4.5794096169187,
3.36007667892742));
#34237=CARTESIAN_POINT('Ctrl Pts',(-0.8177051517065,-4.44352561926563,3.33361938224295));
#34238=CARTESIAN_POINT('Ctrl Pts',(-1.55611804241598,-4.30764162161257,
3.30716208555848));
#34239=CARTESIAN_POINT('Ctrl Pts',(-2.2599275198111,-3.9837177745646,3.28070478887401));
#34240=CARTESIAN_POINT('Ctrl Pts',(-2.84341036847309,-3.51120764419552,
3.25424749218955));
#34241=CARTESIAN_POINT('Ctrl Pts',(-3.42689321713508,-3.03869751382645,
3.22779019550508));
#34242=CARTESIAN_POINT('Ctrl Pts',(-3.89004943706392,-2.41760110013629,
3.20133289882062));
#34243=CARTESIAN_POINT('Ctrl Pts',(-4.17646711326174,-1.72356725892568,
3.17487560213615));
#34244=CARTESIAN_POINT('Ctrl Pts',(-4.46288478945955,-1.02953341771508,
3.14841830545168));
#34245=CARTESIAN_POINT('Ctrl Pts',(-4.57256392192634,-0.262562148984027,
3.12196100876721));
#34246=CARTESIAN_POINT('Ctrl Pts',(-4.49214571371297,0.483930295567052,
3.09550371208274));
#34247=CARTESIAN_POINT('Ctrl Pts',(-4.41172750549959,1.23042274011814,3.06904641539827));
#34248=CARTESIAN_POINT('Ctrl Pts',(-4.14121195660606,1.95643636048925,3.04258911871381));
#34249=CARTESIAN_POINT('Ctrl Pts',(-3.71354756149959,2.57354350122118,3.01613182202934));
#34250=CARTESIAN_POINT('Ctrl Pts',(-3.28588316639313,3.1906506419531,2.98967452534487));
#34251=CARTESIAN_POINT('Ctrl Pts',(-2.70106992507374,3.69885130304582,2.9632172286604));
#34252=CARTESIAN_POINT('Ctrl Pts',(-2.03033744310303,4.03624720641976,2.93675993197593));
#34253=CARTESIAN_POINT('Ctrl Pts',(-1.35960496113232,4.3736431097937,2.91030263529147));
#34254=CARTESIAN_POINT('Ctrl Pts',(-0.602953238510295,4.54023425544885,
2.883845338607));
#34255=CARTESIAN_POINT('Ctrl Pts',(0.147458382357749,4.5157300262161,2.85738804192253));
#34256=CARTESIAN_POINT('Ctrl Pts',(0.897870003225787,4.49122579698336,2.83093074523806));
#34257=CARTESIAN_POINT('Ctrl Pts',(1.64204152233985,4.27562619286271,2.80447344855359));
#34258=CARTESIAN_POINT('Ctrl Pts',(2.28933367226974,3.89519100702514,2.77801615186913));
#34259=CARTESIAN_POINT('Ctrl Pts',(2.93662582219963,3.51475582118756,2.75155885518466));
#34260=CARTESIAN_POINT('Ctrl Pts',(3.48703860294536,2.96948505363305,2.72510155850019));
#34261=CARTESIAN_POINT('Ctrl Pts',(3.873532346971,2.32579208038178,2.69864426181572));
#34262=CARTESIAN_POINT('Ctrl Pts',(4.26002609099665,1.68209910713051,2.67218696513126));
#34263=CARTESIAN_POINT('Ctrl Pts',(4.48260079830222,0.939983928182504,2.64572966844679));
#34264=CARTESIAN_POINT('Ctrl Pts',(4.51414711586846,0.189835351011121,2.61927237176232));
#34265=CARTESIAN_POINT('Ctrl Pts',(4.51680568306753,0.126616549085492,2.61704268200554));
#34266=CARTESIAN_POINT('Ctrl Pts',(4.51810751267774,0.063340691696271,2.61481299224876));
#34267=CARTESIAN_POINT('Ctrl Pts',(4.51806423128285,6.30519293007281E-5,
2.61258330249198));
#34268=CARTESIAN_POINT('Origin',(0.,0.,20.5));
#34269=CARTESIAN_POINT('',(4.51755838390264,-0.00010457874560596,1.61258330249198));
#34270=CARTESIAN_POINT('',(4.51787557461174,0.000108094638884985,1.88741669750807));
#34271=CARTESIAN_POINT('',(4.51775,5.53264807684796E-16,20.5));
#34272=CARTESIAN_POINT('Ctrl Pts',(4.51787557461174,0.000108094638884985,
1.88741669750807));
#34273=CARTESIAN_POINT('Ctrl Pts',(4.51800988663209,0.133281854142107,1.89210872312746));
#34274=CARTESIAN_POINT('Ctrl Pts',(4.5122387502371,0.266444013117212,1.89680074874686));
#34275=CARTESIAN_POINT('Ctrl Pts',(4.50047783691867,0.399075035061228,1.90149277436625));
#34276=CARTESIAN_POINT('Ctrl Pts',(4.43416064298431,1.14695208897868,1.92795007105072));
#34277=CARTESIAN_POINT('Ctrl Pts',(4.17739351195545,1.87794119941301,1.95440736773518));
#34278=CARTESIAN_POINT('Ctrl Pts',(3.76145039622174,2.50300870173296,1.98086466441965));
#34279=CARTESIAN_POINT('Ctrl Pts',(3.34550728048802,3.1280762040529,2.00732196110412));
#34280=CARTESIAN_POINT('Ctrl Pts',(2.77038818004944,3.64722209825845,2.03377925778859));
#34281=CARTESIAN_POINT('Ctrl Pts',(2.10614196483581,3.99721498898444,2.06023655447306));
#34282=CARTESIAN_POINT('Ctrl Pts',(1.44189574962217,4.34720787971043,2.08669385115753));
#34283=CARTESIAN_POINT('Ctrl Pts',(0.688522419633492,4.52804776695686,2.11315114784199));
#34284=CARTESIAN_POINT('Ctrl Pts',(-0.0622179873186998,4.51770855260139,
2.13960844452646));
#34285=CARTESIAN_POINT('Ctrl Pts',(-0.812958394270891,4.50736933824591,
2.16606574121093));
#34286=CARTESIAN_POINT('Ctrl Pts',(-1.56106587818659,4.30585102228854,2.1925230378954));
#34287=CARTESIAN_POINT('Ctrl Pts',(-2.21542177547916,3.9376983125846,2.21898033457986));
#34288=CARTESIAN_POINT('Ctrl Pts',(-2.86977767277172,3.56954560288067,2.24543763126433));
#34289=CARTESIAN_POINT('Ctrl Pts',(-3.43038198344116,3.03475849943017,2.2718949279488));
#34290=CARTESIAN_POINT('Ctrl Pts',(-3.82895372288602,2.39847347956868,2.29835222463327));
#34291=CARTESIAN_POINT('Ctrl Pts',(-4.22752546233088,1.76218845970719,2.32480952131774));
#34292=CARTESIAN_POINT('Ctrl Pts',(-4.46406463055117,1.0244055234347,2.35126681800221));
#34293=CARTESIAN_POINT('Ctrl Pts',(-4.50976101864305,0.274985815861316,
2.37772411468667));
#34294=CARTESIAN_POINT('Ctrl Pts',(-4.55545740673492,-0.474433891712066,
2.40418141137114));
#34295=CARTESIAN_POINT('Ctrl Pts',(-4.41031101469838,-1.23549037058635,
2.43063870805561));
#34296=CARTESIAN_POINT('Ctrl Pts',(-4.09200051244538,-1.91548778391935,
2.45709600474008));
#34297=CARTESIAN_POINT('Ctrl Pts',(-3.77369001019238,-2.59548519725235,
2.48355330142454));
#34298=CARTESIAN_POINT('Ctrl Pts',(-3.28221539772292,-3.19442354504408,
2.51001059810901));
#34299=CARTESIAN_POINT('Ctrl Pts',(-2.67743773890551,-3.63935279939741,
2.53646789479348));
#34300=CARTESIAN_POINT('Ctrl Pts',(-2.07266008008808,-4.08428205375076,
2.56292519147795));
#34301=CARTESIAN_POINT('Ctrl Pts',(-1.35457937492269,-4.37520221466569,
2.58938248816241));
#34302=CARTESIAN_POINT('Ctrl Pts',(-0.610657058576137,-4.47667952851314,
2.61583978484688));
#34303=CARTESIAN_POINT('Ctrl Pts',(0.133265257770398,-4.57815684236058,
2.64229708153135));
#34304=CARTESIAN_POINT('Ctrl Pts',(0.9030291852981,-4.49019130914055,2.66875437821582));
#34305=CARTESIAN_POINT('Ctrl Pts',(1.60487832955586,-4.22349703344507,2.69521167490029));
#34306=CARTESIAN_POINT('Ctrl Pts',(2.30672747381364,-3.95680275774959,2.72166897158476));
#34307=CARTESIAN_POINT('Ctrl Pts',(2.94066183480147,-3.51137973957866,2.74812626826922));
#34308=CARTESIAN_POINT('Ctrl Pts',(3.42946890894601,-2.94148000958192,2.77458356495369));
#34309=CARTESIAN_POINT('Ctrl Pts',(3.91827598309054,-2.37158027958518,2.80104086163816));
#34310=CARTESIAN_POINT('Ctrl Pts',(4.26195577039178,-1.67720383776263,2.82749815832263));
#34311=CARTESIAN_POINT('Ctrl Pts',(4.41864845311758,-0.94292496624017,2.85395545500709));
#34312=CARTESIAN_POINT('Ctrl Pts',(4.4847062457604,-0.633370999882247,2.86510920250742));
#34313=CARTESIAN_POINT('Ctrl Pts',(4.51753158998749,-0.316725338941023,
2.87626295000774));
#34314=CARTESIAN_POINT('Ctrl Pts',(4.5174009456275,-5.29814202112051E-5,
2.88741669750807));
#34315=CARTESIAN_POINT('Ctrl Pts',(4.51806423128285,6.30519293007281E-5,
2.61258330249198));
#34316=CARTESIAN_POINT('Ctrl Pts',(4.51759393956657,-0.687506049970836,
2.58835569556429));
#34317=CARTESIAN_POINT('Ctrl Pts',(4.35830909853907,-1.37528559362468,2.5641280886366));
#34318=CARTESIAN_POINT('Ctrl Pts',(4.0551256392357,-1.9923648496729,2.53990048170891));
#34319=CARTESIAN_POINT('Ctrl Pts',(3.72403991720982,-2.66623449779077,2.51344318502445));
#34320=CARTESIAN_POINT('Ctrl Pts',(3.22135054533116,-3.25579181863177,2.48698588833998));
#34321=CARTESIAN_POINT('Ctrl Pts',(2.60828453275314,-3.68922938300052,2.46052859165551));
#34322=CARTESIAN_POINT('Ctrl Pts',(1.99521852017512,-4.12266694736928,2.43407129497105));
#34323=CARTESIAN_POINT('Ctrl Pts',(1.27177586689775,-4.3999847552658,2.40761399828658));
#34324=CARTESIAN_POINT('Ctrl Pts',(0.526071087432441,-4.48740580460158,
2.38115670160211));
#34325=CARTESIAN_POINT('Ctrl Pts',(-0.219633692032863,-4.57482685393736,
2.35469940491764));
#34326=CARTESIAN_POINT('Ctrl Pts',(-0.987600597686097,-4.47235114471241,
2.32824210823317));
#34327=CARTESIAN_POINT('Ctrl Pts',(-1.68429211034942,-4.19246010490287,
2.3017848115487));
#34328=CARTESIAN_POINT('Ctrl Pts',(-2.38098362301274,-3.91256906509334,
2.27532751486424));
#34329=CARTESIAN_POINT('Ctrl Pts',(-3.00639974268614,-3.45526269469925,
2.24887021817977));
#34330=CARTESIAN_POINT('Ctrl Pts',(-3.48436547816518,-2.87624040350871,
2.2224129214953));
#34331=CARTESIAN_POINT('Ctrl Pts',(-3.96233121364423,-2.29721811231817,
2.19595562481083));
#34332=CARTESIAN_POINT('Ctrl Pts',(-4.29284656492891,-1.59647990033118,
2.16949832812637));
#34333=CARTESIAN_POINT('Ctrl Pts',(-4.43565512801646,-0.859374906258969,
2.1430410314419));
#34334=CARTESIAN_POINT('Ctrl Pts',(-4.578463691104,-0.122269912186753,2.11658373475743));
#34335=CARTESIAN_POINT('Ctrl Pts',(-4.53356546599441,0.651201863970698,
2.09012643807296));
#34336=CARTESIAN_POINT('Ctrl Pts',(-4.30642900683079,1.36683241594063,2.06366914138849));
#34337=CARTESIAN_POINT('Ctrl Pts',(-4.07929254766716,2.08246296791056,2.03721184470403));
#34338=CARTESIAN_POINT('Ctrl Pts',(-3.66991785444949,2.74025229569297,2.01075454801956));
#34339=CARTESIAN_POINT('Ctrl Pts',(-3.12816631171559,3.26008238708848,1.98429725133509));
#34340=CARTESIAN_POINT('Ctrl Pts',(-2.58641476898168,3.77991247848399,1.95783995465062));
#34341=CARTESIAN_POINT('Ctrl Pts',(-1.91228637673154,4.16178333349259,1.93138265796616));
#34342=CARTESIAN_POINT('Ctrl Pts',(-1.18788922711582,4.3591835047376,1.90492536128169));
#34343=CARTESIAN_POINT('Ctrl Pts',(-0.463492077500105,4.55658367598262,
1.87846806459722));
#34344=CARTESIAN_POINT('Ctrl Pts',(0.311173829481187,4.56951316346406,1.85201076791275));
#34345=CARTESIAN_POINT('Ctrl Pts',(1.04175504380577,4.39639716966128,1.82555347122828));
#34346=CARTESIAN_POINT('Ctrl Pts',(1.77233625813035,4.2232811758585,1.79909617454381));
#34347=CARTESIAN_POINT('Ctrl Pts',(2.45883277979823,3.86411970077152,1.77263887785935));
#34348=CARTESIAN_POINT('Ctrl Pts',(3.01763009204651,3.36265821505193,1.74618158117488));
#34349=CARTESIAN_POINT('Ctrl Pts',(3.57642740429479,2.86119672933234,1.71972428449041));
#34350=CARTESIAN_POINT('Ctrl Pts',(4.00752550712348,2.21743523298015,1.69326698780594));
#34351=CARTESIAN_POINT('Ctrl Pts',(4.2584171290782,1.50978316287142,1.66680969112148));
#34352=CARTESIAN_POINT('Ctrl Pts',(4.42982474689917,1.02631960741915,1.64873422824498));
#34353=CARTESIAN_POINT('Ctrl Pts',(4.51712029378003,0.513034879908299,1.63065876536848));
#34354=CARTESIAN_POINT('Ctrl Pts',(4.51755838390264,-0.00010457874560596,
1.61258330249198));
#34355=CARTESIAN_POINT('Origin',(0.,0.,20.5));
#34356=CARTESIAN_POINT('',(4.51763087883895,0.00011359767064345,0.612583302491977));
#34357=CARTESIAN_POINT('',(4.5177656910975,-0.000116631996953637,0.887416697508071));
#34358=CARTESIAN_POINT('',(4.51775,5.53264807684796E-16,20.5));
#34359=CARTESIAN_POINT('',(-3.4337878873619,2.93584158412996,0.));
#34360=CARTESIAN_POINT('Ctrl Pts',(4.51763087883895,0.00011359767064345,
0.612583302491977));
#34361=CARTESIAN_POINT('Ctrl Pts',(4.51711863846112,-0.539057740350668,
0.59358994511926));
#34362=CARTESIAN_POINT('Ctrl Pts',(4.42053200733307,-1.07840729234144,0.574596587746541));
#34363=CARTESIAN_POINT('Ctrl Pts',(4.23165828048039,-1.58323058504537,0.555603230373824));
#34364=CARTESIAN_POINT('Ctrl Pts',(3.96856165521391,-2.28643746765176,0.529145933689356));
#34365=CARTESIAN_POINT('Ctrl Pts',(3.52639272074203,-2.92265018460396,0.502688637004889));
#34366=CARTESIAN_POINT('Ctrl Pts',(2.95900217961999,-3.41436616507663,0.476231340320421));
#34367=CARTESIAN_POINT('Ctrl Pts',(2.39161163849795,-3.90608214554931,0.449774043635953));
#34368=CARTESIAN_POINT('Ctrl Pts',(1.69899949072575,-4.25330138954245,0.423316746951485));
#34369=CARTESIAN_POINT('Ctrl Pts',(0.965534545329656,-4.41375671437595,
0.396859450267017));
#34370=CARTESIAN_POINT('Ctrl Pts',(0.232069599933564,-4.57421203920944,
0.370402153582549));
#34371=CARTESIAN_POINT('Ctrl Pts',(-0.542248143086422,-4.54790344488329,
0.343944856898081));
#34372=CARTESIAN_POINT('Ctrl Pts',(-1.26312545635881,-4.33799038903376,
0.317487560213613));
#34373=CARTESIAN_POINT('Ctrl Pts',(-1.9840027696312,-4.12807733318424,0.291030263529145));
#34374=CARTESIAN_POINT('Ctrl Pts',(-2.651439653156,-3.73455981581135,0.264572966844678));
#34375=CARTESIAN_POINT('Ctrl Pts',(-3.18410908512135,-3.20545326780586,
0.23811567016021));
#34376=CARTESIAN_POINT('Ctrl Pts',(-3.71677851708671,-2.67634671980037,
0.211658373475742));
#34377=CARTESIAN_POINT('Ctrl Pts',(-4.11468049749262,-2.01165114116227,
0.185201076791274));
#34378=CARTESIAN_POINT('Ctrl Pts',(-4.32941757999959,-1.29215909736801,
0.158743780106806));
#34379=CARTESIAN_POINT('Ctrl Pts',(-4.54415466250656,-0.572667053573755,
0.132286483422338));
#34380=CARTESIAN_POINT('Ctrl Pts',(-4.57572684711458,0.201621455376676,
0.10582918673787));
#34381=CARTESIAN_POINT('Ctrl Pts',(-4.42014586550132,0.936043740039453,
0.0793718900534021));
#34382=CARTESIAN_POINT('Ctrl Pts',(-4.26456488388806,1.67046602470223,0.0529145933689342));
#34383=CARTESIAN_POINT('Ctrl Pts',(-3.92183073605352,2.36502208507736,0.0264572966844666));
#34384=CARTESIAN_POINT('Ctrl Pts',(-3.43378788736187,2.93584158412999,-1.38777878078145E-15));
#34385=CARTESIAN_POINT('',(3.43409108914489,2.93606647242259,-1.66533453693773E-15));
#34386=CARTESIAN_POINT('Origin',(0.,0.,0.));
#34387=CARTESIAN_POINT('Ctrl Pts',(3.43409108914489,2.93606647242259,-1.66533453693773E-15));
#34388=CARTESIAN_POINT('Ctrl Pts',(2.96705577784701,3.48188002612677,0.0253131010459874));
#34389=CARTESIAN_POINT('Ctrl Pts',(2.36757358452891,3.91460873741651,0.0506262020919764));
#34390=CARTESIAN_POINT('Ctrl Pts',(1.70215900486043,4.18523117809474,0.0759393031379656));
#34391=CARTESIAN_POINT('Ctrl Pts',(1.00666654344788,4.46808621784236,0.102396599822434));
#34392=CARTESIAN_POINT('Ctrl Pts',(0.23914646876357,4.57384880856985,0.128853896506902));
#34393=CARTESIAN_POINT('Ctrl Pts',(-0.506923795872801,4.48961228541997,
0.15531119319137));
#34394=CARTESIAN_POINT('Ctrl Pts',(-1.25299406050917,4.40537576227008,0.181768489875837));
#34395=CARTESIAN_POINT('Ctrl Pts',(-1.9776145150976,4.13114012524282,0.208225786560305));
#34396=CARTESIAN_POINT('Ctrl Pts',(-2.59252418705973,3.70032015205329,0.234683083244772));
#34397=CARTESIAN_POINT('Ctrl Pts',(-3.20743385902187,3.26950017886376,0.26114037992924));
#34398=CARTESIAN_POINT('Ctrl Pts',(-3.71263274835771,2.68209586951196,0.287597676613709));
#34399=CARTESIAN_POINT('Ctrl Pts',(-4.04658977984313,2.00964543895375,0.314054973298177));
#34400=CARTESIAN_POINT('Ctrl Pts',(-4.38054681132855,1.33719500839555,0.340512269982645));
#34401=CARTESIAN_POINT('Ctrl Pts',(-4.54326198496355,0.579698456630952,
0.366969566667112));
#34402=CARTESIAN_POINT('Ctrl Pts',(-4.51491593042486,-0.170578278221808,
0.39342686335158));
#34403=CARTESIAN_POINT('Ctrl Pts',(-4.48656987588618,-0.920855013074566,
0.419884160036048));
#34404=CARTESIAN_POINT('Ctrl Pts',(-4.26716259317382,-1.66391193101549,
0.446341456720516));
#34405=CARTESIAN_POINT('Ctrl Pts',(-3.88341809255795,-2.30924747945238,
0.472798753404984));
#34406=CARTESIAN_POINT('Ctrl Pts',(-3.49967359194208,-2.95458302788927,
0.499256050089452));
#34407=CARTESIAN_POINT('Ctrl Pts',(-2.95159187342268,-3.50219720682213,
0.52571334677392));
#34408=CARTESIAN_POINT('Ctrl Pts',(-2.30592844750098,-3.88539017854139,
0.552170643458388));
#34409=CARTESIAN_POINT('Ctrl Pts',(-1.66026502157927,-4.26858315026064,
0.578627940142856));
#34410=CARTESIAN_POINT('Ctrl Pts',(-0.91701988825525,-4.48735491476628,
0.605085236827324));
#34411=CARTESIAN_POINT('Ctrl Pts',(-0.166719607306316,-4.51505986234428,
0.631542533511792));
#34412=CARTESIAN_POINT('Ctrl Pts',(0.583580673642613,-4.54276480992227,
0.65799983019626));
#34413=CARTESIAN_POINT('Ctrl Pts',(1.34093610221646,-4.37940294057262,0.684457126880727));
#34414=CARTESIAN_POINT('Ctrl Pts',(2.01310169166318,-4.04487125838886,0.710914423565195));
#34415=CARTESIAN_POINT('Ctrl Pts',(2.68526728110991,-3.7103395762051,0.737371720249663));
#34416=CARTESIAN_POINT('Ctrl Pts',(3.27224303142951,-3.20463808118722,0.763829016934131));
#34417=CARTESIAN_POINT('Ctrl Pts',(3.70253591076623,-2.58936080975925,0.790286313618599));
#34418=CARTESIAN_POINT('Ctrl Pts',(4.13282879010294,-1.9740835383313,0.816743610303067));
#34419=CARTESIAN_POINT('Ctrl Pts',(4.40643879845678,-1.24923049049327,0.843200906987535));
#34420=CARTESIAN_POINT('Ctrl Pts',(4.49004055820744,-0.503087883691874,
0.869658203672002));
#34421=CARTESIAN_POINT('Ctrl Pts',(4.50874543387838,-0.336147561686243,
0.875577701617358));
#34422=CARTESIAN_POINT('Ctrl Pts',(4.51793876013751,-0.168141513884366,
0.881497199562714));
#34423=CARTESIAN_POINT('Ctrl Pts',(4.5177656910975,-0.000116631996953637,
0.887416697508071));
#34424=CARTESIAN_POINT('Origin',(0.,0.,-2.20833684463713));
#34425=CARTESIAN_POINT('',(5.07403060246553,1.54698778687123E-5,39.208336844637));
#34426=CARTESIAN_POINT('',(5.07396752856948,-6.48011021279027E-5,39.2916631553629));
#34427=CARTESIAN_POINT('',(5.0736,-1.85409460923845E-12,-2.20833684463713));
#34428=CARTESIAN_POINT('',(-1.31303618635666,-4.90075024188317,40.));
#34429=CARTESIAN_POINT('Ctrl Pts',(5.07396752856948,-6.48011021277175E-5,
39.2916631553629));
#34430=CARTESIAN_POINT('Ctrl Pts',(5.07347424400433,0.779307331517198,39.3161170634328));
#34431=CARTESIAN_POINT('Ctrl Pts',(4.69381943413572,2.40236770827343,39.3670282681872));
#34432=CARTESIAN_POINT('Ctrl Pts',(3.03470961035893,4.33144609848054,39.4443967696262));
#34433=CARTESIAN_POINT('Ctrl Pts',(0.593383061700927,5.25537632570972,39.5237686596795));
#34434=CARTESIAN_POINT('Ctrl Pts',(-1.99247705733066,4.8990504464678,39.603140549733));
#34435=CARTESIAN_POINT('Ctrl Pts',(-4.09299916691649,3.34943642687039,39.6825124397864));
#34436=CARTESIAN_POINT('Ctrl Pts',(-5.19642846461573,0.983699440459269,
39.7618843298398));
#34437=CARTESIAN_POINT('Ctrl Pts',(-5.03410925482033,-1.62126816458454,
39.8412562198932));
#34438=CARTESIAN_POINT('Ctrl Pts',(-3.6453165085118,-3.83208153227987,39.9206281099466));
#34439=CARTESIAN_POINT('Ctrl Pts',(-2.12771778283764,-4.68247622999901,
39.9735427033155));
#34440=CARTESIAN_POINT('Ctrl Pts',(-1.31303618635638,-4.90075024188325,
40.));
#34441=CARTESIAN_POINT('',(1.31317395760221,-4.90115117757563,40.));
#34442=CARTESIAN_POINT('Origin',(0.,0.,40.));
#34443=CARTESIAN_POINT('Ctrl Pts',(5.07403060246553,1.54698778688793E-5,
39.208336844637));
#34444=CARTESIAN_POINT('Ctrl Pts',(5.07403315687698,0.0146420671929676,
39.2087957918851));
#34445=CARTESIAN_POINT('Ctrl Pts',(5.07040151797183,0.872458469457581,39.2357120358177));
#34446=CARTESIAN_POINT('Ctrl Pts',(4.62253485344793,2.56965255248844,39.2890855764349));
#34447=CARTESIAN_POINT('Ctrl Pts',(2.83047200092405,4.46759066254981,39.3684574664882));
#34448=CARTESIAN_POINT('Ctrl Pts',(0.34891291852996,5.27723479734496,39.4478293565417));
#34449=CARTESIAN_POINT('Ctrl Pts',(-2.21764149317963,4.80135391043001,39.527201246595));
#34450=CARTESIAN_POINT('Ctrl Pts',(-4.24398161873814,3.15587819282133,39.6065731366485));
#34451=CARTESIAN_POINT('Ctrl Pts',(-5.23650047694821,0.74162931109825,39.6859450267018));
#34452=CARTESIAN_POINT('Ctrl Pts',(-4.9534132521342,-1.85326330477585,39.7653169167553));
#34453=CARTESIAN_POINT('Ctrl Pts',(-3.46369715057683,-3.99673439595749,
39.8446888068086));
#34454=CARTESIAN_POINT('Ctrl Pts',(-1.1638488125998,-5.14969078544563,39.9229165012236));
#34455=CARTESIAN_POINT('Ctrl Pts',(0.533836595431815,-5.10962665469158,
39.974686898954));
#34456=CARTESIAN_POINT('Ctrl Pts',(1.31317395760221,-4.90115117757563,40.));
#34457=CARTESIAN_POINT('Origin',(0.,0.,-2.20833684463713));
#34458=CARTESIAN_POINT('',(5.07325764975804,-8.44407784307555E-5,38.208336844637));
#34459=CARTESIAN_POINT('',(5.07316912366228,-1.81818814078922E-5,38.2916631553629));
#34460=CARTESIAN_POINT('',(5.0736,-1.85409460923845E-12,-2.20833684463713));
#34461=CARTESIAN_POINT('Ctrl Pts',(5.07316912366228,-1.81818814076751E-5,
38.2916631553629));
#34462=CARTESIAN_POINT('Ctrl Pts',(5.07311400239361,0.441352830351579,38.3055055398681));
#34463=CARTESIAN_POINT('Ctrl Pts',(4.90711571561459,1.72636801461904,38.3458052210578));
#34464=CARTESIAN_POINT('Ctrl Pts',(3.83482475204887,3.64212307300276,38.4125621989319));
#34465=CARTESIAN_POINT('Ctrl Pts',(1.62575061805696,5.03268082057242,38.4919340889853));
#34466=CARTESIAN_POINT('Ctrl Pts',(-0.979352771366501,5.19728867487039,
38.5713059790387));
#34467=CARTESIAN_POINT('Ctrl Pts',(-3.3458879870052,4.09584848370752,38.6506778690921));
#34468=CARTESIAN_POINT('Ctrl Pts',(-4.89737230716795,1.99666872129193,38.7300497591456));
#34469=CARTESIAN_POINT('Ctrl Pts',(-5.2558675504918,-0.588895222855594,
38.809421649199));
#34470=CARTESIAN_POINT('Ctrl Pts',(-4.33404513553914,-3.03100540392653,
38.8887935392523));
#34471=CARTESIAN_POINT('Ctrl Pts',(-2.35645883694701,-4.73476973691708,
38.9681654293058));
#34472=CARTESIAN_POINT('Ctrl Pts',(0.195155463808245,-5.28515396379923,
39.0475373193592));
#34473=CARTESIAN_POINT('Ctrl Pts',(2.69923061743519,-4.54808766460433,39.1269092094126));
#34474=CARTESIAN_POINT('Ctrl Pts',(4.5457786161602,-2.70311485851688,39.2062810994659));
#34475=CARTESIAN_POINT('Ctrl Pts',(5.05724155748156,-0.970965988519946,
39.2611990814494));
#34476=CARTESIAN_POINT('Ctrl Pts',(5.07400794095178,-0.063914933051532,
39.2896597667484));
#34477=CARTESIAN_POINT('Ctrl Pts',(5.07396752856948,-6.48011021277175E-5,
39.2916631553629));
#34478=CARTESIAN_POINT('Ctrl Pts',(5.07325764975804,-8.44407784305126E-5,
38.208336844637));
#34479=CARTESIAN_POINT('Ctrl Pts',(5.07294945930103,0.51977335908998,38.2246415650049));
#34480=CARTESIAN_POINT('Ctrl Pts',(4.86451980067584,1.88343404898941,38.2674035820572));
#34481=CARTESIAN_POINT('Ctrl Pts',(3.66171031660113,3.81612616476472,38.336622895794));
#34482=CARTESIAN_POINT('Ctrl Pts',(1.39049711694169,5.10269135980963,38.4159947858473));
#34483=CARTESIAN_POINT('Ctrl Pts',(-1.21943810235573,5.14625223481529,38.4953666759008));
#34484=CARTESIAN_POINT('Ctrl Pts',(-3.53232089954511,3.93619745533324,38.5747385659542));
#34485=CARTESIAN_POINT('Ctrl Pts',(-4.98473814342406,1.76729369047725,38.6541104560076));
#34486=CARTESIAN_POINT('Ctrl Pts',(-5.22288421068334,-0.832118909543577,
38.733482346061));
#34487=CARTESIAN_POINT('Ctrl Pts',(-4.18874724188046,-3.22882917750522,
38.8128542361144));
#34488=CARTESIAN_POINT('Ctrl Pts',(-2.13424072225093,-4.83900381899058,
38.8922261261678));
#34489=CARTESIAN_POINT('Ctrl Pts',(0.440162123945958,-5.27040781417516,
38.9715980162212));
#34490=CARTESIAN_POINT('Ctrl Pts',(2.90734243084964,-4.41795218255951,39.0509699062746));
#34491=CARTESIAN_POINT('Ctrl Pts',(4.65612987828293,-2.500445050276,39.1298828490799));
#34492=CARTESIAN_POINT('Ctrl Pts',(5.07388590069044,-0.828549010266373,
39.1823384952007));
#34493=CARTESIAN_POINT('Ctrl Pts',(5.07403060246553,1.54698778688793E-5,
39.208336844637));
#34494=CARTESIAN_POINT('Origin',(0.,0.,-2.20833684463713));
#34495=CARTESIAN_POINT('',(5.07364050160013,0.000130038443658109,37.208336844637));
#34496=CARTESIAN_POINT('',(5.07387656802193,9.59844669708175E-5,37.2916631553629));
#34497=CARTESIAN_POINT('',(5.0736,-1.85409460923845E-12,-2.20833684463713));
#34498=CARTESIAN_POINT('Ctrl Pts',(5.07387656802193,9.59844669710073E-5,
37.2916631553629));
#34499=CARTESIAN_POINT('Ctrl Pts',(5.07396569861154,0.103072231247123,37.2948940163033));
#34500=CARTESIAN_POINT('Ctrl Pts',(5.04574853055582,1.04926503651591,37.3245821739283));
#34501=CARTESIAN_POINT('Ctrl Pts',(4.48202491545551,2.80756015154514,37.3807276282377));
#34502=CARTESIAN_POINT('Ctrl Pts',(2.59328691715162,4.6093171199916,37.4600995182911));
#34503=CARTESIAN_POINT('Ctrl Pts',(0.0728299659736646,5.28825464055466,
37.5394714083445));
#34504=CARTESIAN_POINT('Ctrl Pts',(-2.46536820371075,4.67898503603898,37.6188432983979));
#34505=CARTESIAN_POINT('Ctrl Pts',(-4.40300813596802,2.92992503348812,37.6982151884513));
#34506=CARTESIAN_POINT('Ctrl Pts',(-5.26808503220261,0.467141778084607,
37.7775870785047));
#34507=CARTESIAN_POINT('Ctrl Pts',(-4.84986807528987,-2.10943618050861,
37.8569589685581));
#34508=CARTESIAN_POINT('Ctrl Pts',(-3.2502339902585,-4.17216015459505,37.9363308586115));
#34509=CARTESIAN_POINT('Ctrl Pts',(-0.858850099431265,-5.21855515011692,
38.0157027486649));
#34510=CARTESIAN_POINT('Ctrl Pts',(1.74174777450972,-4.99372166181591,38.0950746387183));
#34511=CARTESIAN_POINT('Ctrl Pts',(3.91805974601555,-3.55242863073569,38.1744465287717));
#34512=CARTESIAN_POINT('Ctrl Pts',(4.92684606433671,-1.64805066527608,38.2399760343199));
#34513=CARTESIAN_POINT('Ctrl Pts',(5.0732193570569,-0.402250655317197,38.2790482431836));
#34514=CARTESIAN_POINT('Ctrl Pts',(5.07316912366228,-1.81818814076751E-5,
38.2916631553629));
#34515=CARTESIAN_POINT('Ctrl Pts',(5.07364050160013,0.000130038443658265,
37.208336844637));
#34516=CARTESIAN_POINT('Ctrl Pts',(5.07382783063862,0.181611936494348,37.2140300414401));
#34517=CARTESIAN_POINT('Ctrl Pts',(5.01990561118457,1.20636170521342,37.2461805349277));
#34518=CARTESIAN_POINT('Ctrl Pts',(4.34693493313475,3.01249033764469,37.3047883250998));
#34519=CARTESIAN_POINT('Ctrl Pts',(2.37663436681862,4.72467463787371,37.3841602151531));
#34520=CARTESIAN_POINT('Ctrl Pts',(-0.17260907066365,5.28593865420645,37.4635321052065));
#34521=CARTESIAN_POINT('Ctrl Pts',(-2.67980532059584,4.55955971460153,37.54290399526));
#34522=CARTESIAN_POINT('Ctrl Pts',(-4.53420692607955,2.72248212093334,37.6222758853133));
#34523=CARTESIAN_POINT('Ctrl Pts',(-5.28408576066665,0.222213908718847,
37.7016477753668));
#34524=CARTESIAN_POINT('Ctrl Pts',(-4.74677300008161,-2.33218511979937,
37.7810196654201));
#34525=CARTESIAN_POINT('Ctrl Pts',(-3.05315684347904,-4.31846901533503,
37.8603915554736));
#34526=CARTESIAN_POINT('Ctrl Pts',(-0.615798437855754,-5.25278341751105,
37.9397634455269));
#34527=CARTESIAN_POINT('Ctrl Pts',(1.97156710418767,-4.90753140600709,38.0191353355804));
#34528=CARTESIAN_POINT('Ctrl Pts',(4.07866326363087,-3.36681560666115,38.0985072256337));
#34529=CARTESIAN_POINT('Ctrl Pts',(4.96346005639167,-1.49092415374923,38.1615743953193));
#34530=CARTESIAN_POINT('Ctrl Pts',(5.07344955290414,-0.323787998268402,
38.1981842683204));
#34531=CARTESIAN_POINT('Ctrl Pts',(5.07325764975804,-8.44407784305126E-5,
38.208336844637));
#34532=CARTESIAN_POINT('Origin',(0.,0.,-2.20833684463713));
#34533=CARTESIAN_POINT('',(5.07371855919287,-0.000123991516001801,36.208336844637));
#34534=CARTESIAN_POINT('',(5.07347409402005,-0.000127990615926579,36.2916631553629));
#34535=CARTESIAN_POINT('',(5.0736,-1.85409460923845E-12,-2.20833684463713));
#34536=CARTESIAN_POINT('Ctrl Pts',(5.07347409402005,-0.00012799061592652,
36.2916631553629));
#34537=CARTESIAN_POINT('Ctrl Pts',(5.07289252391416,0.608034774450749,36.3107397894231));
#34538=CARTESIAN_POINT('Ctrl Pts',(4.81166108430775,2.06014185956918,36.3562737201677));
#34539=CARTESIAN_POINT('Ctrl Pts',(3.45741385862894,4.002153265115,36.4282649475969));
#34540=CARTESIAN_POINT('Ctrl Pts',(1.12210854951209,5.16834729390565,36.5076368376502));
#34541=CARTESIAN_POINT('Ctrl Pts',(-1.4865399185207,5.07554336184357,36.5870087277037));
#34542=CARTESIAN_POINT('Ctrl Pts',(-3.73307055280216,3.74634830136112,36.666380617757));
#34543=CARTESIAN_POINT('Ctrl Pts',(-5.07023346343257,1.50455108706837,36.7457525078105));
#34544=CARTESIAN_POINT('Ctrl Pts',(-5.17229872514219,-1.10375144176689,
36.8251243978638));
#34545=CARTESIAN_POINT('Ctrl Pts',(-4.01440346609619,-3.44318256250012,
36.9044962879173));
#34546=CARTESIAN_POINT('Ctrl Pts',(-1.87860840844056,-4.94386203236358,
36.9838681779707));
#34547=CARTESIAN_POINT('Ctrl Pts',(0.71481149928202,-5.24022765419639,37.0632400680241));
#34548=CARTESIAN_POINT('Ctrl Pts',(3.13410490798792,-4.26008541851396,37.1426119580775));
#34549=CARTESIAN_POINT('Ctrl Pts',(4.72253605350391,-2.32433471697507,37.2187529871904));
#34550=CARTESIAN_POINT('Ctrl Pts',(5.07323581438062,-0.740193128270358,
37.2684367196189));
#34551=CARTESIAN_POINT('Ctrl Pts',(5.07387656802193,9.59844669710073E-5,
37.2916631553629));
#34552=CARTESIAN_POINT('Ctrl Pts',(5.07371855919287,-0.000123991516001801,
36.208336844637));
#34553=CARTESIAN_POINT('Ctrl Pts',(5.07301904482133,0.686442797877024,36.2298758145598));
#34554=CARTESIAN_POINT('Ctrl Pts',(4.76024594010631,2.21696867292356,36.2778720811671));
#34555=CARTESIAN_POINT('Ctrl Pts',(3.26800144929601,4.15825779320007,36.3523256444589));
#34556=CARTESIAN_POINT('Ctrl Pts',(0.881102883784141,5.2148441065383,36.4316975345123));
#34557=CARTESIAN_POINT('Ctrl Pts',(-1.72043039392939,5.00110593838543,36.5110694245656));
#34558=CARTESIAN_POINT('Ctrl Pts',(-3.90287063578981,3.56910943340206,36.5904413146191));
#34559=CARTESIAN_POINT('Ctrl Pts',(-5.13458022962944,1.26768577053169,36.6698132046725));
#34560=CARTESIAN_POINT('Ctrl Pts',(-5.11551744473188,-1.34254334006536,
36.7491850947259));
#34561=CARTESIAN_POINT('Ctrl Pts',(-3.85032593330342,-3.62573186469175,
36.8285569847793));
#34562=CARTESIAN_POINT('Ctrl Pts',(-1.64720354707418,-5.02570013250056,
36.9079288748327));
#34563=CARTESIAN_POINT('Ctrl Pts',(0.957173977199105,-5.20141897223083,
36.9873007648861));
#34564=CARTESIAN_POINT('Ctrl Pts',(3.32838603929536,-4.11008366347129,37.0666726549395));
#34565=CARTESIAN_POINT('Ctrl Pts',(4.77688430036561,-2.16763522711972,37.1403513481898));
#34566=CARTESIAN_POINT('Ctrl Pts',(5.07295727932621,-0.661766675847902,
37.1875727447556));
#34567=CARTESIAN_POINT('Ctrl Pts',(5.07364050160013,0.000130038443658265,
37.208336844637));
#34568=CARTESIAN_POINT('Origin',(0.,0.,-2.20833684463713));
#34569=CARTESIAN_POINT('',(5.07321765521711,6.54440514302745E-5,35.208336844637));
#34570=CARTESIAN_POINT('',(5.07337786466077,0.000116280867786642,35.2916631553629));
#34571=CARTESIAN_POINT('',(5.0736,-1.85409460923845E-12,-2.20833684463713));
#34572=CARTESIAN_POINT('Ctrl Pts',(5.07337786466077,0.000116280867786742,
35.2916631553629));
#34573=CARTESIAN_POINT('Ctrl Pts',(5.07360553071623,0.269998548266127,35.3001282658583));
#34574=CARTESIAN_POINT('Ctrl Pts',(4.98629871182508,1.38323904612086,35.3350506730382));
#34575=CARTESIAN_POINT('Ctrl Pts',(4.18367369924664,3.23540039647985,35.3964303769026));
#34576=CARTESIAN_POINT('Ctrl Pts',(2.12664217080567,4.8423480280398,35.4758022669559));
#34577=CARTESIAN_POINT('Ctrl Pts',(-0.448434683200953,5.2697103983248,35.5551741570095));
#34578=CARTESIAN_POINT('Ctrl Pts',(-2.91427384097317,4.41338297988397,35.6345460470627));
#34579=CARTESIAN_POINT('Ctrl Pts',(-4.67020234172003,2.48196523640092,35.7139179371163));
#34580=CARTESIAN_POINT('Ctrl Pts',(-5.28847988934142,-0.0540537449324728,
35.7932898271696));
#34581=CARTESIAN_POINT('Ctrl Pts',(-4.61849544177097,-2.57690535364626,
35.872661717223));
#34582=CARTESIAN_POINT('Ctrl Pts',(-2.82345572745135,-4.47202852209511,
35.9520336072764));
#34583=CARTESIAN_POINT('Ctrl Pts',(-0.340628447537815,-5.27777544122882,
36.0314054973298));
#34584=CARTESIAN_POINT('Ctrl Pts',(2.22517516822766,-4.79786794503694,36.1107773873833));
#34585=CARTESIAN_POINT('Ctrl Pts',(4.2489310383545,-3.14921043733466,36.1901492774366));
#34586=CARTESIAN_POINT('Ctrl Pts',(5.00002147582269,-1.31403716914749,36.2504445334299));
#34587=CARTESIAN_POINT('Ctrl Pts',(5.07369910083888,-0.235423387877496,
36.2842824927386));
#34588=CARTESIAN_POINT('Ctrl Pts',(5.07347409402005,-0.00012799061592652,
36.2916631553629));
#34589=CARTESIAN_POINT('Ctrl Pts',(5.07321765521711,6.54440514305868E-5,
35.208336844637));
#34590=CARTESIAN_POINT('Ctrl Pts',(5.07337613287412,0.348482730653562,35.2192642909951));
#34591=CARTESIAN_POINT('Ctrl Pts',(4.95236148577976,1.54037186125541,35.2566490340376));
#34592=CARTESIAN_POINT('Ctrl Pts',(4.02905439992751,3.42602714375337,35.3204910737646));
#34593=CARTESIAN_POINT('Ctrl Pts',(1.8996801667365,4.93580354262787,35.3998629638181));
#34594=CARTESIAN_POINT('Ctrl Pts',(-0.69245195020073,5.24322912373406,35.4792348538714));
#34595=CARTESIAN_POINT('Ctrl Pts',(-3.11590430478548,4.27341569598948,35.5586067439249));
#34596=CARTESIAN_POINT('Ctrl Pts',(-4.78032926766171,2.26260766374704,35.6379786339782));
#34597=CARTESIAN_POINT('Ctrl Pts',(-5.28027660201491,-0.299366587187078,
35.7173505240316));
#34598=CARTESIAN_POINT('Ctrl Pts',(-4.49396024381123,-2.78841580011912,
35.7967224140851));
#34599=CARTESIAN_POINT('Ctrl Pts',(-2.61292511742748,-4.59821309619579,
35.8760943041384));
#34600=CARTESIAN_POINT('Ctrl Pts',(-0.0953872160500441,-5.28789586001125,
35.9554661941919));
#34601=CARTESIAN_POINT('Ctrl Pts',(2.4453868000212,-4.68945889688694,36.0348380842453));
#34602=CARTESIAN_POINT('Ctrl Pts',(4.39047000437915,-2.94868012642215,36.1142099742987));
#34603=CARTESIAN_POINT('Ctrl Pts',(5.02844178521537,-1.15692185290368,36.1720428944293));
#34604=CARTESIAN_POINT('Ctrl Pts',(5.07387829014872,-0.156898425299628,
36.2034185178754));
#34605=CARTESIAN_POINT('Ctrl Pts',(5.07371855919287,-0.000123991516001801,
36.208336844637));
#34606=CARTESIAN_POINT('Origin',(0.,0.,-2.20833684463713));
#34607=CARTESIAN_POINT('',(5.07403267809782,1.0680673442065E-5,34.208336844637));
#34608=CARTESIAN_POINT('',(5.07395837593185,-6.84743504405761E-5,34.2916631553629));
#34609=CARTESIAN_POINT('',(5.0736,-1.85409460923845E-12,-2.20833684463713));
#34610=CARTESIAN_POINT('Ctrl Pts',(5.07395837593184,-6.84743504405106E-5,
34.2916631553629));
#34611=CARTESIAN_POINT('Ctrl Pts',(5.07344266957576,0.774748712740892,34.315974038978));
#34612=CARTESIAN_POINT('Ctrl Pts',(4.69722240792898,2.39327548011594,34.3667422192777));
#34613=CARTESIAN_POINT('Ctrl Pts',(3.04637426047967,4.32325632045994,34.4439676962618));
#34614=CARTESIAN_POINT('Ctrl Pts',(0.607552238322964,5.25374358196314,34.5233395863151));
#34615=CARTESIAN_POINT('Ctrl Pts',(-1.97926816429518,4.90443053586424,34.6027114763686));
#34616=CARTESIAN_POINT('Ctrl Pts',(-4.08394322312674,3.36040906700167,34.6820833664219));
#34617=CARTESIAN_POINT('Ctrl Pts',(-5.19377875245966,0.997799387556786,
34.7614552564754));
#34618=CARTESIAN_POINT('Ctrl Pts',(-5.03842127392763,-1.60787201410546,
34.8408271465287));
#34619=CARTESIAN_POINT('Ctrl Pts',(-3.65571552542313,-3.82186935209593,
34.9201990365822));
#34620=CARTESIAN_POINT('Ctrl Pts',(-1.38248556671468,-5.10486777548014,
34.9995709266355));
#34621=CARTESIAN_POINT('Ctrl Pts',(1.22751481596557,-5.14433170819057,35.078942816689));
#34622=CARTESIAN_POINT('Ctrl Pts',(3.53849530653457,-3.93064782357091,35.1583147067423));
#34623=CARTESIAN_POINT('Ctrl Pts',(4.83296736710027,-1.99102597475866,35.2292214863004));
#34624=CARTESIAN_POINT('Ctrl Pts',(5.07289397138366,-0.573505529121166,
35.2736709691739));
#34625=CARTESIAN_POINT('Ctrl Pts',(5.07337786466077,0.000116280867786742,
35.2916631553629));
#34626=CARTESIAN_POINT('Ctrl Pts',(5.07403267809783,1.06806734422689E-5,
34.208336844637));
#34627=CARTESIAN_POINT('Ctrl Pts',(5.07403390825189,0.0100790925016438,
34.2086527674304));
#34628=CARTESIAN_POINT('Ctrl Pts',(5.07154731505229,0.863336953552071,34.2354259869081));
#34629=CARTESIAN_POINT('Ctrl Pts',(4.62944563286023,2.55718096342464,34.2886565030704));
#34630=CARTESIAN_POINT('Ctrl Pts',(2.84250620674923,4.45994392474861,34.3680283931238));
#34631=CARTESIAN_POINT('Ctrl Pts',(0.363138560454883,5.27627441792225,34.4474002831772));
#34632=CARTESIAN_POINT('Ctrl Pts',(-2.20468883537271,4.80731614172534,34.5267721732306));
#34633=CARTESIAN_POINT('Ctrl Pts',(-4.23545891089946,3.1673062942179,34.606144063284));
#34634=CARTESIAN_POINT('Ctrl Pts',(-5.23448057076036,0.755747644152594,
34.6855159533374));
#34635=CARTESIAN_POINT('Ctrl Pts',(-4.95839434991029,-1.83990945920924,
34.7648878433908));
#34636=CARTESIAN_POINT('Ctrl Pts',(-3.47445424064183,-3.98736869087822,
34.8442597334442));
#34637=CARTESIAN_POINT('Ctrl Pts',(-1.14414476892706,-5.16351373534018,
34.9236316234976));
#34638=CARTESIAN_POINT('Ctrl Pts',(1.4648758359769,-5.0818382631171,35.003003513551));
#34639=CARTESIAN_POINT('Ctrl Pts',(3.71705592968454,-3.76223823845686,35.0823754036044));
#34640=CARTESIAN_POINT('Ctrl Pts',(4.87836197951498,-1.83401443292226,35.1508198472998));
#34641=CARTESIAN_POINT('Ctrl Pts',(5.07299243019996,-0.495097664945923,
35.1928069943106));
#34642=CARTESIAN_POINT('Ctrl Pts',(5.07321765521711,6.54440514305868E-5,
35.208336844637));
#34643=CARTESIAN_POINT('Origin',(0.,0.,-2.20833684463713));
#34644=CARTESIAN_POINT('',(5.07324948390142,-8.11089730112791E-5,33.208336844637));
#34645=CARTESIAN_POINT('',(5.07316757009266,-1.39624117367057E-5,33.2916631553629));
#34646=CARTESIAN_POINT('',(5.0736,-1.85409460923845E-12,-2.20833684463713));
#34647=CARTESIAN_POINT('Ctrl Pts',(5.07316757009266,-1.39624117367898E-5,
33.2916631553629));
#34648=CARTESIAN_POINT('Ctrl Pts',(5.07312569317602,0.436797029802116,33.3053625154133));
#34649=CARTESIAN_POINT('Ctrl Pts',(4.90946580291021,1.7172430470973,33.3455191721481));
#34650=CARTESIAN_POINT('Ctrl Pts',(3.84462977702742,3.63177136187071,33.4121331255675));
#34651=CARTESIAN_POINT('Ctrl Pts',(1.63931253580255,5.02827960213734,33.4915050156209));
#34652=CARTESIAN_POINT('Ctrl Pts',(-0.965337610587002,5.19991006123145,
33.5708769056743));
#34653=CARTESIAN_POINT('Ctrl Pts',(-3.33483365177614,4.1048539392153,33.6502487957277));
#34654=CARTESIAN_POINT('Ctrl Pts',(-4.89197159692173,2.00986448354636,33.7296206857811));
#34655=CARTESIAN_POINT('Ctrl Pts',(-5.25743608925264,-0.574723511554913,
33.8089925758345));
#34656=CARTESIAN_POINT('Ctrl Pts',(-4.34220078737896,-3.01931013137032,
33.888364465888));
#34657=CARTESIAN_POINT('Ctrl Pts',(-2.36921498499824,-4.72839948631349,
33.9677363559413));
#34658=CARTESIAN_POINT('Ctrl Pts',(0.18090634355963,-5.28566119252548,34.0471082459947));
#34659=CARTESIAN_POINT('Ctrl Pts',(2.68695928725581,-4.55534753185087,34.1264801360481));
#34660=CARTESIAN_POINT('Ctrl Pts',(4.53847489605999,-2.71536129550809,34.2058520261016));
#34661=CARTESIAN_POINT('Ctrl Pts',(5.05594943598948,-0.980087925357289,
34.2609130325398));
#34662=CARTESIAN_POINT('Ctrl Pts',(5.07400390775537,-0.0684772480926434,
34.2895167422936));
#34663=CARTESIAN_POINT('Ctrl Pts',(5.07395837593184,-6.84743504405106E-5,
34.2916631553629));
#34664=CARTESIAN_POINT('Ctrl Pts',(5.07324948390142,-8.1108973011175E-5,
33.208336844637));
#34665=CARTESIAN_POINT('Ctrl Pts',(5.07295666213735,0.515218890813949,33.22449854055));
#34666=CARTESIAN_POINT('Ctrl Pts',(4.86710522495599,1.87431284273704,33.2671175331475));
#34667=CARTESIAN_POINT('Ctrl Pts',(3.67198507285579,3.80624052997629,33.3361938224296));
#34668=CARTESIAN_POINT('Ctrl Pts',(1.40424863498483,5.09892411381589,33.4155657124829));
#34669=CARTESIAN_POINT('Ctrl Pts',(-1.20555966211678,5.14952106980705,33.4949376025364));
#34670=CARTESIAN_POINT('Ctrl Pts',(-3.52169629398785,3.94570609146478,33.5743094925897));
#34671=CARTESIAN_POINT('Ctrl Pts',(-4.979955503786,1.78072584291395,33.6536813826432));
#34672=CARTESIAN_POINT('Ctrl Pts',(-5.22510857580638,-0.818035279400921,
33.7330532726965));
#34673=CARTESIAN_POINT('Ctrl Pts',(-4.19743676434199,-3.2175248183441,33.81242516275));
#34674=CARTESIAN_POINT('Ctrl Pts',(-2.14727864795256,-4.83323243340904,
33.8917970528034));
#34675=CARTESIAN_POINT('Ctrl Pts',(0.425951794157462,-5.27157532587404,
33.9711689428568));
#34676=CARTESIAN_POINT('Ctrl Pts',(2.89542132203897,-4.4257741373902,34.0505408329101));
#34677=CARTESIAN_POINT('Ctrl Pts',(4.6525507987008,-2.50952187653605,34.1295968001703));
#34678=CARTESIAN_POINT('Ctrl Pts',(5.07393088766675,-0.833110966960862,
34.1821954707459));
#34679=CARTESIAN_POINT('Ctrl Pts',(5.07403267809783,1.06806734422689E-5,
34.208336844637));
#34680=CARTESIAN_POINT('Origin',(0.,0.,-2.20833684463713));
#34681=CARTESIAN_POINT('',(5.07365497060222,0.000129255909634973,32.208336844637));
#34682=CARTESIAN_POINT('',(5.0738885135215,9.2741528424134E-5,32.2916631553629));
#34683=CARTESIAN_POINT('',(5.0736,-1.85409460923845E-12,-2.20833684463713));
#34684=CARTESIAN_POINT('Ctrl Pts',(5.0738885135215,9.27415284240896E-5,
32.2916631553629));
#34685=CARTESIAN_POINT('Ctrl Pts',(5.07397157552195,0.0985097427010157,
32.2947509918485));
#34686=CARTESIAN_POINT('Ctrl Pts',(5.04713500973232,1.0401410882179,32.3242961250187));
#34687=CARTESIAN_POINT('Ctrl Pts',(4.48957765297736,2.79546665964672,32.3802985548733));
#34688=CARTESIAN_POINT('Ctrl Pts',(2.60570395470567,4.60230901263064,32.4596704449267));
#34689=CARTESIAN_POINT('Ctrl Pts',(0.0870865406955613,5.28803907717593,
32.5390423349801));
#34690=CARTESIAN_POINT('Ctrl Pts',(-2.45274496186521,4.68561452739711,32.6184142250335));
#34691=CARTESIAN_POINT('Ctrl Pts',(-4.39509322077448,2.94178465017617,32.6977861150869));
#34692=CARTESIAN_POINT('Ctrl Pts',(-5.26680649947691,0.48134254370224,32.7771580051403));
#34693=CARTESIAN_POINT('Ctrl Pts',(-4.85553737278523,-2.09635354098391,
32.8565298951937));
#34694=CARTESIAN_POINT('Ctrl Pts',(-3.26147008963279,-4.16338254328624,
32.9359017852471));
#34695=CARTESIAN_POINT('Ctrl Pts',(-0.8729159117874,-5.21622077353502,33.0152736753005));
#34696=CARTESIAN_POINT('Ctrl Pts',(1.72827865000283,-4.99839916925953,33.0946455653539));
#34697=CARTESIAN_POINT('Ctrl Pts',(3.9084683581323,-3.5629785911213,33.1740174554073));
#34698=CARTESIAN_POINT('Ctrl Pts',(4.92459807825024,-1.65717664129123,33.2396899854103));
#34699=CARTESIAN_POINT('Ctrl Pts',(5.07320656921722,-0.406807195031642,
33.2789052187288));
#34700=CARTESIAN_POINT('Ctrl Pts',(5.07316757009266,-1.39624117367898E-5,
33.2916631553629));
#34701=CARTESIAN_POINT('Ctrl Pts',(5.07365497060222,0.000129255909635077,
32.208336844637));
#34702=CARTESIAN_POINT('Ctrl Pts',(5.07383759281576,0.177050513766622,32.2138870169853));
#34703=CARTESIAN_POINT('Ctrl Pts',(5.02150924629178,1.19723596214486,32.2458944860181));
#34704=CARTESIAN_POINT('Ctrl Pts',(4.35504064192764,3.00076029606972,32.3043592517354));
#34705=CARTESIAN_POINT('Ctrl Pts',(2.3893631891323,4.71825019448202,32.3837311417886));
#34706=CARTESIAN_POINT('Ctrl Pts',(-0.158357847769981,5.28638478918814,
32.4631030318421));
#34707=CARTESIAN_POINT('Ctrl Pts',(-2.66750326347463,4.56676775046226,32.5424749218955));
#34708=CARTESIAN_POINT('Ctrl Pts',(-4.52685078861515,2.73469619609277,32.6218468119489));
#34709=CARTESIAN_POINT('Ctrl Pts',(-5.28346748166331,0.23645870150246,32.7012187020024));
#34710=CARTESIAN_POINT('Ctrl Pts',(-4.75304319093522,-2.31937960938145,
32.7805905920557));
#34711=CARTESIAN_POINT('Ctrl Pts',(-3.06478809957792,-4.3102221812797,32.8599624821091));
#34712=CARTESIAN_POINT('Ctrl Pts',(-0.629957410956834,-5.25110417033318,
32.9393343721625));
#34713=CARTESIAN_POINT('Ctrl Pts',(1.95832950858626,-4.91282880661543,33.0187062622159));
#34714=CARTESIAN_POINT('Ctrl Pts',(4.06957169452659,-3.37779921996823,33.0980781522693));
#34715=CARTESIAN_POINT('Ctrl Pts',(4.96144058461863,-1.50005120370765,33.1612883464097));
#34716=CARTESIAN_POINT('Ctrl Pts',(5.07343602224469,-0.328346354394994,
33.1980412438656));
#34717=CARTESIAN_POINT('Ctrl Pts',(5.07324948390142,-8.1108973011175E-5,
33.208336844637));
#34718=CARTESIAN_POINT('Origin',(0.,0.,-2.20833684463713));
#34719=CARTESIAN_POINT('',(5.073704252564,-0.000125440355911652,31.2083368446371));
#34720=CARTESIAN_POINT('',(5.07346075270687,-0.000126888963244813,31.2916631553629));
#34721=CARTESIAN_POINT('',(5.0736,-1.85409460923845E-12,-2.20833684463713));
#34722=CARTESIAN_POINT('Ctrl Pts',(5.07346075270687,-0.000126888963244594,
31.2916631553629));
#34723=CARTESIAN_POINT('Ctrl Pts',(5.07289095298355,0.60348081698673,31.3105967649683));
#34724=CARTESIAN_POINT('Ctrl Pts',(4.81451756387892,2.05102782258644,31.3559876712581));
#34725=CARTESIAN_POINT('Ctrl Pts',(3.46819087602115,3.99281772621712,31.4278358742324));
#34726=CARTESIAN_POINT('Ctrl Pts',(1.13603804757386,5.16530336977167,31.5072077642858));
#34727=CARTESIAN_POINT('Ctrl Pts',(-1.47285113468488,5.07953254565492,31.5865796543392));
#34728=CARTESIAN_POINT('Ctrl Pts',(-3.72295704063504,3.75639883677117,31.6659515443926));
#34729=CARTESIAN_POINT('Ctrl Pts',(-5.06615885211213,1.51821468589782,31.745323434446));
#34730=CARTESIAN_POINT('Ctrl Pts',(-5.17525558096714,-1.08980320194903,
31.8246953244994));
#34731=CARTESIAN_POINT('Ctrl Pts',(-4.02367150553249,-3.43234744203962,
31.9040672145529));
#34732=CARTESIAN_POINT('Ctrl Pts',(-1.89192995759591,-4.93877944262154,
31.9834391046062));
#34733=CARTESIAN_POINT('Ctrl Pts',(0.70068154029511,-5.24213570278371,32.0628109946597));
#34734=CARTESIAN_POINT('Ctrl Pts',(3.12260856590247,-4.26851930901834,32.142182884713));
#34735=CARTESIAN_POINT('Ctrl Pts',(4.71924613978307,-2.33342987779042,32.2184669382808));
#34736=CARTESIAN_POINT('Ctrl Pts',(5.07325988110442,-0.74474986994901,32.2682936951641));
#34737=CARTESIAN_POINT('Ctrl Pts',(5.0738885135215,9.27415284240896E-5,
32.2916631553629));
#34738=CARTESIAN_POINT('Ctrl Pts',(5.073704252564,-0.000125440355911652,
31.2083368446371));
#34739=CARTESIAN_POINT('Ctrl Pts',(5.0730059773177,0.681887909050636,31.2297327901051));
#34740=CARTESIAN_POINT('Ctrl Pts',(4.76334894417968,2.20786416800771,31.2775860322575));
#34741=CARTESIAN_POINT('Ctrl Pts',(3.27920000412114,4.14943233229341,31.3518965710945));
#34742=CARTESIAN_POINT('Ctrl Pts',(0.895158610487983,5.21244975125701,31.4312684611478));
#34743=CARTESIAN_POINT('Ctrl Pts',(-1.70694143926006,5.00572594837619,31.5106403512013));
#34744=CARTESIAN_POINT('Ctrl Pts',(-3.89323433265515,3.57961838445739,31.5900122412546));
#34745=CARTESIAN_POINT('Ctrl Pts',(-5.13114396014345,1.28152370543563,31.6693841313081));
#34746=CARTESIAN_POINT('Ctrl Pts',(-5.11911827653528,-1.32874731162563,
31.7487560213615));
#34747=CARTESIAN_POINT('Ctrl Pts',(-3.86008671173927,-3.61533842470713,
31.8281279114149));
#34748=CARTESIAN_POINT('Ctrl Pts',(-1.6607465681206,-5.02124109994587,31.9074998014683));
#34749=CARTESIAN_POINT('Ctrl Pts',(0.943147763492109,-5.20398055756647,
31.9868716915216));
#34750=CARTESIAN_POINT('Ctrl Pts',(3.31729338754031,-4.11904187017945,32.0662435815751));
#34751=CARTESIAN_POINT('Ctrl Pts',(4.77384508508688,-2.17674249303873,32.1400652992802));
#34752=CARTESIAN_POINT('Ctrl Pts',(5.07296704505946,-0.666321171863868,
32.1874297203008));
#34753=CARTESIAN_POINT('Ctrl Pts',(5.07365497060222,0.000129255909635077,
32.208336844637));
#34754=CARTESIAN_POINT('Origin',(0.,0.,-2.20833684463713));
#34755=CARTESIAN_POINT('',(5.0732242396654,6.91156314036601E-5,30.208336844637));
#34756=CARTESIAN_POINT('',(5.07338983982448,0.000118254562807938,30.2916631553629));
#34757=CARTESIAN_POINT('',(5.0736,-1.85409460923845E-12,-2.20833684463713));
#34758=CARTESIAN_POINT('Ctrl Pts',(5.07338983982448,0.000118254562808118,
30.2916631553629));
#34759=CARTESIAN_POINT('Ctrl Pts',(5.07361825292341,0.265438860321299,30.2999852414035));
#34760=CARTESIAN_POINT('Ctrl Pts',(4.98815112489718,1.37411209267241,30.3347646241286));
#34761=CARTESIAN_POINT('Ctrl Pts',(4.19238095442003,3.22410968801099,30.3960013035382));
#34762=CARTESIAN_POINT('Ctrl Pts',(2.13968914249988,4.83659712202475,30.4753731935916));
#34763=CARTESIAN_POINT('Ctrl Pts',(-0.434226208411599,5.27090020273941,
30.554745083645));
#34764=CARTESIAN_POINT('Ctrl Pts',(-2.90236501609743,4.4212236610065,30.6341169736984));
#34765=CARTESIAN_POINT('Ctrl Pts',(-4.66349413013793,2.49454682166501,30.7134888637518));
#34766=CARTESIAN_POINT('Ctrl Pts',(-5.28860639654603,-0.0397961018483339,
30.7928607538052));
#34767=CARTESIAN_POINT('Ctrl Pts',(-4.62542585088724,-2.56444478303865,
30.8722326438586));
#34768=CARTESIAN_POINT('Ctrl Pts',(-2.83550180615875,-4.46440039138299,
30.951604533912));
#34769=CARTESIAN_POINT('Ctrl Pts',(-0.354855797726762,-5.27683794616905,
31.0309764239654));
#34770=CARTESIAN_POINT('Ctrl Pts',(2.21223229757146,-4.80384945735102,31.1103483140188));
#34771=CARTESIAN_POINT('Ctrl Pts',(4.24042550187443,-3.16065387386267,31.1897202040722));
#34772=CARTESIAN_POINT('Ctrl Pts',(4.99825410162456,-1.32316383571886,31.2501584845202));
#34773=CARTESIAN_POINT('Ctrl Pts',(5.07368717518548,-0.239983714616348,
31.2841394682838));
#34774=CARTESIAN_POINT('Ctrl Pts',(5.07346075270687,-0.000126888963244594,
31.2916631553629));
#34775=CARTESIAN_POINT('Ctrl Pts',(5.0732242396654,6.91156314035213E-5,
30.208336844637));
#34776=CARTESIAN_POINT('Ctrl Pts',(5.07338968774506,0.343924846945636,30.2191212665403));
#34777=CARTESIAN_POINT('Ctrl Pts',(4.95443916911164,1.53124494231641,30.256362985128));
#34778=CARTESIAN_POINT('Ctrl Pts',(4.0382761360698,3.41515258753676,30.3200620004003));
#34779=CARTESIAN_POINT('Ctrl Pts',(1.91297991407722,4.93066417388641,30.3994338904535));
#34780=CARTESIAN_POINT('Ctrl Pts',(-0.678313980675348,5.24507688131741,
30.4788057805071));
#34781=CARTESIAN_POINT('Ctrl Pts',(-3.10437209115798,4.28180047024023,30.5581776705604));
#34782=CARTESIAN_POINT('Ctrl Pts',(-4.77421203164559,2.2754869422171,30.6375495606138));
#34783=CARTESIAN_POINT('Ctrl Pts',(-5.28106448876339,-0.285130168225216,
30.7169214506672));
#34784=CARTESIAN_POINT('Ctrl Pts',(-4.50146132585641,-2.77629020081278,
30.7962933407206));
#34785=CARTESIAN_POINT('Ctrl Pts',(-2.62531214778642,-4.59115208569648,
30.8756652307741));
#34786=CARTESIAN_POINT('Ctrl Pts',(-0.109642741545517,-5.28761948484725,
30.9550371208274));
#34787=CARTESIAN_POINT('Ctrl Pts',(2.43273539384572,-4.69603448143646,31.0344090108809));
#34788=CARTESIAN_POINT('Ctrl Pts',(4.38250457206463,-2.96050587284378,31.1137809009342));
#34789=CARTESIAN_POINT('Ctrl Pts',(5.02689419953704,-1.16604718553494,31.1717568455196));
#34790=CARTESIAN_POINT('Ctrl Pts',(5.07386943415284,-0.161460170846308,
31.2032754934206));
#34791=CARTESIAN_POINT('Ctrl Pts',(5.073704252564,-0.000125440355911652,
31.2083368446371));
#34792=CARTESIAN_POINT('Origin',(0.,0.,-2.20833684463713));
#34793=CARTESIAN_POINT('',(5.07403430731529,5.85510781675173E-6,29.2083368446371));
#34794=CARTESIAN_POINT('',(5.07394886825829,-7.2464216758803E-5,29.2916631553629));
#34795=CARTESIAN_POINT('',(5.0736,-1.85409460923845E-12,-2.20833684463713));
#34796=CARTESIAN_POINT('Ctrl Pts',(5.07394886825829,-7.24642167588933E-5,
29.2916631553629));
#34797=CARTESIAN_POINT('Ctrl Pts',(5.07341208948874,0.770190548650157,29.3158310145232));
#34798=CARTESIAN_POINT('Ctrl Pts',(4.70060969038705,2.3841859592787,29.3664561703681));
#34799=CARTESIAN_POINT('Ctrl Pts',(3.05801844753361,4.31502775447088,29.4435386228973));
#34800=CARTESIAN_POINT('Ctrl Pts',(0.621713829942241,5.25208656259286,29.5229105129507));
#34801=CARTESIAN_POINT('Ctrl Pts',(-1.96603890048284,4.90974870936366,29.6022824030042));
#34802=CARTESIAN_POINT('Ctrl Pts',(-4.07486890650364,3.37140693807791,29.6816542930575));
#34803=CARTESIAN_POINT('Ctrl Pts',(-5.19106986646947,1.01179789915904,29.7610261831109));
#34804=CARTESIAN_POINT('Ctrl Pts',(-5.04273769720158,-1.59428286841832,
29.8403980731643));
#34805=CARTESIAN_POINT('Ctrl Pts',(-3.66600578680595,-3.81199985813419,
29.9197699632177));
#34806=CARTESIAN_POINT('Ctrl Pts',(-1.39624298131062,-5.10112212012718,
29.9991418532712));
#34807=CARTESIAN_POINT('Ctrl Pts',(1.21364152390063,-5.1476223247995,30.0785137433246));
#34808=CARTESIAN_POINT('Ctrl Pts',(3.52788564023963,-3.94017312521939,30.157885633378));
#34809=CARTESIAN_POINT('Ctrl Pts',(4.83020369710336,-2.00014283583164,30.2289354373907));
#34810=CARTESIAN_POINT('Ctrl Pts',(5.07289208966392,-0.578059506409542,
30.2735279447191));
#34811=CARTESIAN_POINT('Ctrl Pts',(5.07338983982448,0.000118254562808118,
30.2916631553629));
#34812=CARTESIAN_POINT('Ctrl Pts',(5.07403400238361,5.85099688312179E-6,
29.2083368446371));
#34813=CARTESIAN_POINT('Ctrl Pts',(5.07403437680669,0.00551609080175396,
29.2085097429756));
#34814=CARTESIAN_POINT('Ctrl Pts',(5.07268078911905,0.854215563279166,29.2351399379985));
#34815=CARTESIAN_POINT('Ctrl Pts',(4.6363228263275,2.54469094339263,29.2882274297059));
#34816=CARTESIAN_POINT('Ctrl Pts',(2.85451963682592,4.45226447892365,29.3675993197594));
#34817=CARTESIAN_POINT('Ctrl Pts',(0.377361782165573,5.2752762423091,29.4469712098127));
#34818=CARTESIAN_POINT('Ctrl Pts',(-2.19172056735417,4.81324238969394,29.5263430998662));
#34819=CARTESIAN_POINT('Ctrl Pts',(-4.22690463795758,3.17871334488069,29.6057149899195));
#34820=CARTESIAN_POINT('Ctrl Pts',(-5.23242409484928,0.769856765217166,
29.6850868799731));
#34821=CARTESIAN_POINT('Ctrl Pts',(-4.96333662400999,-1.82653521840426,
29.7644587700263));
#34822=CARTESIAN_POINT('Ctrl Pts',(-3.48519133772112,-3.97798726578954,
29.8438306600798));
#34823=CARTESIAN_POINT('Ctrl Pts',(-1.15806115590354,-5.16041042035391,
29.9232025501331));
#34824=CARTESIAN_POINT('Ctrl Pts',(1.45117016016719,-5.08576901889481,30.0025744401866));
#34825=CARTESIAN_POINT('Ctrl Pts',(3.70689963733188,-3.77224554159173,30.08194633024));
#34826=CARTESIAN_POINT('Ctrl Pts',(4.87583741971579,-1.84313681714053,30.1505337983901));
#34827=CARTESIAN_POINT('Ctrl Pts',(5.07298379589765,-0.499652414928338,
30.1926639698558));
#34828=CARTESIAN_POINT('Ctrl Pts',(5.0732242396654,6.91156314035213E-5,
30.208336844637));
#34829=CARTESIAN_POINT('Origin',(0.,0.,-2.20833684463713));
#34830=CARTESIAN_POINT('',(5.07324166632265,-7.76939179139569E-5,28.2083368446371));
#34831=CARTESIAN_POINT('',(5.07316594158954,-9.7399319174236E-6,28.2916631553629));
#34832=CARTESIAN_POINT('',(5.0736,-1.85409460923845E-12,-2.20833684463713));
#34833=CARTESIAN_POINT('Ctrl Pts',(5.0731664254358,-9.72907478691276E-6,
28.2916631553629));
#34834=CARTESIAN_POINT('Ctrl Pts',(5.07313755787372,0.432241135355033,28.3052194909585));
#34835=CARTESIAN_POINT('Ctrl Pts',(4.91180237168408,1.70811792520993,28.3452331232385));
#34836=CARTESIAN_POINT('Ctrl Pts',(3.85440685831077,3.62139325645763,28.4117040522031));
#34837=CARTESIAN_POINT('Ctrl Pts',(1.6528625396316,5.02384183393471,28.4910759422564));
#34838=CARTESIAN_POINT('Ctrl Pts',(-0.951315435152638,5.20249366075061,
28.5704478323099));
#34839=CARTESIAN_POINT('Ctrl Pts',(-3.32375507563475,4.11382954733206,28.6498197223633));
#34840=CARTESIAN_POINT('Ctrl Pts',(-4.8865353366993,2.02304566199065,28.7291916124167));
#34841=CARTESIAN_POINT('Ctrl Pts',(-5.25896640590637,-0.560547668676075,
28.8085635024701));
#34842=CARTESIAN_POINT('Ctrl Pts',(-4.35032489915935,-3.00759282800452,
28.8879353925235));
#34843=CARTESIAN_POINT('Ctrl Pts',(-2.38195387625792,-4.72199503162487,
28.9673072825769));
#34844=CARTESIAN_POINT('Ctrl Pts',(0.166655838534471,-5.28612969750008,
29.0466791726303));
#34845=CARTESIAN_POINT('Ctrl Pts',(2.67466855994625,-4.56257486971391,29.1260510626837));
#34846=CARTESIAN_POINT('Ctrl Pts',(4.53113794043359,-2.72758690275364,29.2054229527372));
#34847=CARTESIAN_POINT('Ctrl Pts',(5.05464511995301,-0.989211078787786,
29.2606269836302));
#34848=CARTESIAN_POINT('Ctrl Pts',(5.07399971767151,-0.0730399965665694,
29.2893737178388));
#34849=CARTESIAN_POINT('Ctrl Pts',(5.07394886825829,-7.24642167588933E-5,
29.2916631553629));
#34850=CARTESIAN_POINT('Ctrl Pts',(5.07324166632265,-7.76939179139916E-5,
28.2083368446371));
#34851=CARTESIAN_POINT('Ctrl Pts',(5.07296420662618,0.510664363139913,28.2243555160953));
#34852=CARTESIAN_POINT('Ctrl Pts',(4.86967684263928,1.86519135610718,28.266831484238));
#34853=CARTESIAN_POINT('Ctrl Pts',(3.68223314068176,3.79632723101881,28.3357647490651));
#34854=CARTESIAN_POINT('Ctrl Pts',(1.41798994671214,5.09511980804509,28.4151366391186));
#34855=CARTESIAN_POINT('Ctrl Pts',(-1.19167245960906,5.15275247768794,28.4945085291719));
#34856=CARTESIAN_POINT('Ctrl Pts',(-3.51104609249168,3.9551860491902,28.5738804192253));
#34857=CARTESIAN_POINT('Ctrl Pts',(-4.97513666881207,1.79414505376557,28.6532523092787));
#34858=CARTESIAN_POINT('Ctrl Pts',(-5.22729496488809,-0.803945705483672,
28.7326241993322));
#34859=CARTESIAN_POINT('Ctrl Pts',(-4.2060957779385,-3.20619707038074,28.8119960893855));
#34860=CARTESIAN_POINT('Ctrl Pts',(-2.16030096951815,-4.82742592572986,
28.891367979439));
#34861=CARTESIAN_POINT('Ctrl Pts',(0.41173837333167,-5.27270451089724,28.9707398694923));
#34862=CARTESIAN_POINT('Ctrl Pts',(2.88347915980534,-4.43356394814356,29.0501117595458));
#34863=CARTESIAN_POINT('Ctrl Pts',(4.64895661344711,-2.51859756056696,29.1293107512606));
#34864=CARTESIAN_POINT('Ctrl Pts',(5.07397708173548,-0.837673326665985,
29.1820524462911));
#34865=CARTESIAN_POINT('Ctrl Pts',(5.07403400238361,5.85099688312179E-6,
29.2083368446371));
#34866=CARTESIAN_POINT('Origin',(0.,0.,-2.20833684463713));
#34867=CARTESIAN_POINT('',(5.07366942975965,0.000128322057781627,27.2083368446371));
#34868=CARTESIAN_POINT('',(5.07390014538872,8.93747992460227E-5,27.2916631553629));
#34869=CARTESIAN_POINT('',(5.0736,-1.85409460923845E-12,-2.20833684463713));
#34870=CARTESIAN_POINT('Ctrl Pts',(5.07390014538872,8.93747992459192E-5,
27.2916631553629));
#34871=CARTESIAN_POINT('Ctrl Pts',(5.07397720165276,0.0939472090868575,
27.2946079673937));
#34872=CARTESIAN_POINT('Ctrl Pts',(5.04850897709501,1.03101725778952,27.324010076109));
#34873=CARTESIAN_POINT('Ctrl Pts',(4.49709775967288,2.7833528499375,27.3798694815089));
#34874=CARTESIAN_POINT('Ctrl Pts',(2.61810205366886,4.59526745509821,27.4592413715622));
#34875=CARTESIAN_POINT('Ctrl Pts',(0.101342482461748,5.28778507964899,27.5386132616156));
#34876=CARTESIAN_POINT('Ctrl Pts',(-2.44010389315526,4.69220996311103,27.617985151669));
#34877=CARTESIAN_POINT('Ctrl Pts',(-4.38714636147802,2.95362288558985,27.6973570417224));
#34878=CARTESIAN_POINT('Ctrl Pts',(-5.26548968692851,0.495539810872365,
27.7767289317758));
#34879=CARTESIAN_POINT('Ctrl Pts',(-4.86117137960698,-2.08325566491491,
27.8561008218293));
#34880=CARTESIAN_POINT('Ctrl Pts',(-3.27268248423349,-4.15457467193712,
27.9354727118826));
#34881=CARTESIAN_POINT('Ctrl Pts',(-0.886975379660524,-5.21384848487045,
28.0148446019361));
#34882=CARTESIAN_POINT('Ctrl Pts',(1.71479696411104,-5.00304034754724,28.0942164919895));
#34883=CARTESIAN_POINT('Ctrl Pts',(3.89884856306386,-3.57350265560346,28.1735883820429));
#34884=CARTESIAN_POINT('Ctrl Pts',(4.92233667869786,-1.66630250443567,28.2394039365007));
#34885=CARTESIAN_POINT('Ctrl Pts',(5.07319389740952,-0.411363633920409,
28.278762194274));
#34886=CARTESIAN_POINT('Ctrl Pts',(5.0731664254358,-9.72907478691276E-6,
28.2916631553629));
#34887=CARTESIAN_POINT('Ctrl Pts',(5.07366942975965,0.000128322057781714,
27.2083368446371));
#34888=CARTESIAN_POINT('Ctrl Pts',(5.07384715626772,0.172489015223486,27.2137439925305));
#34889=CARTESIAN_POINT('Ctrl Pts',(5.02310017357893,1.18811030837938,27.2456084371085));
#34890=CARTESIAN_POINT('Ctrl Pts',(4.36311469772634,2.98900844458398,27.3039301783709));
#34891=CARTESIAN_POINT('Ctrl Pts',(2.40207464524773,4.7117914582426,27.3833020684242));
#34892=CARTESIAN_POINT('Ctrl Pts',(-0.144105473911181,5.28679250204684,
27.4626739584777));
#34893=CARTESIAN_POINT('Ctrl Pts',(-2.65518181859737,4.57394259446923,27.542045848531));
#34894=CARTESIAN_POINT('Ctrl Pts',(-4.51946174941854,2.74689039512913,27.6214177385845));
#34895=CARTESIAN_POINT('Ctrl Pts',(-5.28281080174027,0.25070177567431,27.7007896286378));
#34896=CARTESIAN_POINT('Ctrl Pts',(-4.75927883606144,-2.30655724141581,
27.7801615186913));
#34897=CARTESIAN_POINT('Ctrl Pts',(-3.07639708040302,-4.30194401997489,
27.8595334087447));
#34898=CARTESIAN_POINT('Ctrl Pts',(-0.644111805447875,-5.24938675745965,
27.9389052987981));
#34899=CARTESIAN_POINT('Ctrl Pts',(1.94507767959709,-4.91809050014772,28.0182771888515));
#34900=CARTESIAN_POINT('Ctrl Pts',(4.06045054724861,-3.38875828300845,28.0976490789049));
#34901=CARTESIAN_POINT('Ctrl Pts',(4.95940796121397,-1.50917823199387,28.1610022975001));
#34902=CARTESIAN_POINT('Ctrl Pts',(5.07342247393797,-0.332904603741066,
28.1978982194108));
#34903=CARTESIAN_POINT('Ctrl Pts',(5.07324166632265,-7.76939179139916E-5,
28.2083368446371));
#34904=CARTESIAN_POINT('Origin',(0.,0.,-2.20833684463713));
#34905=CARTESIAN_POINT('',(5.07368988190431,-0.000126739092140837,26.2083368446371));
#34906=CARTESIAN_POINT('',(5.07344758812249,-0.000125648970980255,26.2916631553629));
#34907=CARTESIAN_POINT('',(5.0736,-1.85409460923845E-12,-2.20833684463713));
#34908=CARTESIAN_POINT('Ctrl Pts',(5.07344758812249,-0.000125648970980205,
26.2916631553629));
#34909=CARTESIAN_POINT('Ctrl Pts',(5.0728899391017,0.598926868258771,26.3104537405135));
#34910=CARTESIAN_POINT('Ctrl Pts',(4.81735989282913,2.0419133290656,26.3557016223485));
#34911=CARTESIAN_POINT('Ctrl Pts',(3.47894268615705,3.98345316700778,26.427406800868));
#34912=CARTESIAN_POINT('Ctrl Pts',(1.14995928876529,5.16222190355009,26.5067786909214));
#34913=CARTESIAN_POINT('Ctrl Pts',(-1.45915164597797,5.08348481077201,26.5861505809748));
#34914=CARTESIAN_POINT('Ctrl Pts',(-3.71281646953845,3.76642207019263,26.6655224710282));
#34915=CARTESIAN_POINT('Ctrl Pts',(-5.06204741929919,1.53186725014815,26.7448943610816));
#34916=CARTESIAN_POINT('Ctrl Pts',(-5.17817482237054,-1.07584704130177,
26.824266251135));
#34917=CARTESIAN_POINT('Ctrl Pts',(-4.032910300408,-3.42148737483758,26.9036381411884));
#34918=CARTESIAN_POINT('Ctrl Pts',(-1.90523775596165,-4.93366095719681,
26.9830100312419));
#34919=CARTESIAN_POINT('Ctrl Pts',(0.686546488664775,-5.24400565085624,
27.0623819212952));
#34920=CARTESIAN_POINT('Ctrl Pts',(3.11108952829732,-4.27692217537667,27.1417538113486));
#34921=CARTESIAN_POINT('Ctrl Pts',(4.71594148821095,-2.34252421969056,27.2181808893712));
#34922=CARTESIAN_POINT('Ctrl Pts',(5.07328489925194,-0.749306805737992,
27.2681506707093));
#34923=CARTESIAN_POINT('Ctrl Pts',(5.07390014538872,8.93747992459192E-5,
27.2916631553629));
#34924=CARTESIAN_POINT('Ctrl Pts',(5.07368988190431,-0.000126739092140768,
26.2083368446371));
#34925=CARTESIAN_POINT('Ctrl Pts',(5.07299367900981,0.677333119387493,26.2295897656503));
#34926=CARTESIAN_POINT('Ctrl Pts',(4.76643747661854,2.19875901809265,26.2772999833479));
#34927=CARTESIAN_POINT('Ctrl Pts',(3.29037472529985,4.14057671278022,26.35146749773));
#34928=CARTESIAN_POINT('Ctrl Pts',(0.909207831064193,5.21001751122215,26.4308393877834));
#34929=CARTESIAN_POINT('Ctrl Pts',(-1.69344007832135,5.01030957610855,26.5102112778369));
#34930=CARTESIAN_POINT('Ctrl Pts',(-3.88356973299385,3.59010131838702,26.5895831678902));
#34931=CARTESIAN_POINT('Ctrl Pts',(-5.12767039684481,1.29535232606086,26.6689550579437));
#34932=CARTESIAN_POINT('Ctrl Pts',(-5.12268190193029,-1.31494162567991,
26.748326947997));
#34933=CARTESIAN_POINT('Ctrl Pts',(-3.86981943456965,-3.604918707979,26.8276988380504));
#34934=CARTESIAN_POINT('Ctrl Pts',(-1.67427751864785,-5.01674557236666,
26.9070707281038));
#34935=CARTESIAN_POINT('Ctrl Pts',(0.929114694866165,-5.20650431970375,
26.9864426181573));
#34936=CARTESIAN_POINT('Ctrl Pts',(3.30617662527125,-4.12797013916282,27.0658145082107));
#34937=CARTESIAN_POINT('Ctrl Pts',(4.77079146294434,-2.18584915384965,27.1397792503706));
#34938=CARTESIAN_POINT('Ctrl Pts',(5.07297753645236,-0.6708757466937,27.1872866958461));
#34939=CARTESIAN_POINT('Ctrl Pts',(5.07366942975965,0.000128322057781714,
27.2083368446371));
#34940=CARTESIAN_POINT('Origin',(0.,0.,-2.20833684463713));
#34941=CARTESIAN_POINT('',(5.07323119136609,7.27167192501876E-5,25.2083368446371));
#34942=CARTESIAN_POINT('',(5.07340205215522,0.00012010210694157,25.2916631553629));
#34943=CARTESIAN_POINT('',(5.0736,-1.85409460923845E-12,-2.20833684463713));
#34944=CARTESIAN_POINT('Ctrl Pts',(5.07340205215522,0.000120102106941772,
25.2916631553629));
#34945=CARTESIAN_POINT('Ctrl Pts',(5.07363086957761,0.260879072720769,25.2998422169487));
#34946=CARTESIAN_POINT('Ctrl Pts',(4.98999058102238,1.36498517337352,25.334478575219));
#34947=CARTESIAN_POINT('Ctrl Pts',(4.20105773883081,3.21279554629917,25.3955722301737));
#34948=CARTESIAN_POINT('Ctrl Pts',(2.15272056265901,4.83081106300121,25.4749441202272));
#34949=CARTESIAN_POINT('Ctrl Pts',(-0.420014577610356,5.27205169757513,
25.5543160102805));
#34950=CARTESIAN_POINT('Ctrl Pts',(-2.89043509646038,4.42903220810823,25.6336879003339));
#34951=CARTESIAN_POINT('Ctrl Pts',(-4.65675202368223,2.50711027624266,25.7130597903873));
#34952=CARTESIAN_POINT('Ctrl Pts',(-5.28869446548081,-0.0255381695211706,
25.7924316804408));
#34953=CARTESIAN_POINT('Ctrl Pts',(-4.63232264181493,-2.55196557371741,
25.8718035704942));
#34954=CARTESIAN_POINT('Ctrl Pts',(-2.84752727607513,-4.45673981283608,
25.9511754605475));
#34955=CARTESIAN_POINT('Ctrl Pts',(-0.369080568778156,-5.27586209837409,
26.030547350601));
#34956=CARTESIAN_POINT('Ctrl Pts',(2.19927334812716,-4.80979605467087,26.1099192406543));
#34957=CARTESIAN_POINT('Ctrl Pts',(4.23188914543768,-3.17207433835284,26.1892911307078));
#34958=CARTESIAN_POINT('Ctrl Pts',(4.99647384522203,-1.33229055500106,26.2498724356106));
#34959=CARTESIAN_POINT('Ctrl Pts',(5.0736751134574,-0.244543947095586,26.283996443829));
#34960=CARTESIAN_POINT('Ctrl Pts',(5.07344758812249,-0.000125648970980205,
26.2916631553629));
#34961=CARTESIAN_POINT('Ctrl Pts',(5.07323119136609,7.2716719250257E-5,
25.2083368446371));
#34962=CARTESIAN_POINT('Ctrl Pts',(5.07340324942578,0.339366856221997,25.2189782420855));
#34963=CARTESIAN_POINT('Ctrl Pts',(4.95650365046512,1.52211798561692,25.2560769362184));
#34964=CARTESIAN_POINT('Ctrl Pts',(4.04746852150308,3.40425320955296,25.3196329270358));
#34965=CARTESIAN_POINT('Ctrl Pts',(1.92626575763449,4.92548896844514,25.3990048170892));
#34966=CARTESIAN_POINT('Ctrl Pts',(-0.664171081076968,5.24688651700902,
25.4783767071426));
#34967=CARTESIAN_POINT('Ctrl Pts',(-3.09281731455583,4.2901541238158,25.5577485971959));
#34968=CARTESIAN_POINT('Ctrl Pts',(-4.76806009604388,2.2883496821561,25.6371204872494));
#34969=CARTESIAN_POINT('Ctrl Pts',(-5.28181399205765,-0.2708916769007,25.7164923773028));
#34970=CARTESIAN_POINT('Ctrl Pts',(-4.50892969070311,-2.76414442307307,
25.7958642673562));
#34971=CARTESIAN_POINT('Ctrl Pts',(-2.63768009703987,-4.58405770611471,
25.8752361574096));
#34972=CARTESIAN_POINT('Ctrl Pts',(-0.123897470143628,-5.28730467858643,
25.9546080474629));
#34973=CARTESIAN_POINT('Ctrl Pts',(2.42006630623721,-4.70257593460492,26.0339799375165));
#34974=CARTESIAN_POINT('Ctrl Pts',(4.37450728714461,-2.97231010192892,26.1133518275698));
#34975=CARTESIAN_POINT('Ctrl Pts',(5.02533394688967,-1.17517261458846,26.17147079661));
#34976=CARTESIAN_POINT('Ctrl Pts',(5.07386036677103,-0.166021846101412,
26.2031324689658));
#34977=CARTESIAN_POINT('Ctrl Pts',(5.07368988190431,-0.000126739092140768,
26.2083368446371));
#34978=CARTESIAN_POINT('Origin',(0.,0.,-2.20833684463713));
#34979=CARTESIAN_POINT('',(5.07403460521456,1.01146903839872E-6,24.2083368446371));
#34980=CARTESIAN_POINT('',(5.07393893245752,-7.63518475177419E-5,24.2916631553629));
#34981=CARTESIAN_POINT('',(5.0736,-1.85409460923845E-12,-2.20833684463713));
#34982=CARTESIAN_POINT('Ctrl Pts',(5.07393893245752,-7.63518475176573E-5,
24.2916631553629));
#34983=CARTESIAN_POINT('Ctrl Pts',(5.0733825372435,0.765632623134578,24.3156879900684));
#34984=CARTESIAN_POINT('Ctrl Pts',(4.70398212533016,2.37509554318665,24.3661701214584));
#34985=CARTESIAN_POINT('Ctrl Pts',(3.0696404085172,4.30676782630642,24.4431095495329));
#34986=CARTESIAN_POINT('Ctrl Pts',(0.635870902865647,5.25039137038364,24.5224814395863));
#34987=CARTESIAN_POINT('Ctrl Pts',(-1.95279534724764,4.9150311981795,24.6018533296397));
#34988=CARTESIAN_POINT('Ctrl Pts',(-4.06576497321052,3.38238030533593,24.6812252196931));
#34989=CARTESIAN_POINT('Ctrl Pts',(-5.18832325111748,1.02578905688434,24.7605971097465));
#34990=CARTESIAN_POINT('Ctrl Pts',(-5.04701746921096,-1.58068213527875,
24.8399689997999));
#34991=CARTESIAN_POINT('Ctrl Pts',(-3.67626940318832,-3.80210265806849,
24.9193408898533));
#34992=CARTESIAN_POINT('Ctrl Pts',(-1.40999024783327,-5.09733938916421,
24.9987127799067));
#34993=CARTESIAN_POINT('Ctrl Pts',(1.19975941093347,-5.1508755278289,25.0780846699601));
#34994=CARTESIAN_POINT('Ctrl Pts',(3.51725033281924,-3.94966978918403,25.1574565600135));
#34995=CARTESIAN_POINT('Ctrl Pts',(4.82742597758186,-2.00925929492118,25.2286493884811));
#34996=CARTESIAN_POINT('Ctrl Pts',(5.07289070026022,-0.582613469337955,
25.2733849202643));
#34997=CARTESIAN_POINT('Ctrl Pts',(5.07340205215522,0.000120102106941772,
25.2916631553629));
#34998=CARTESIAN_POINT('Ctrl Pts',(5.07403455984306,1.01136344364921E-6,
24.2083368446371));
#34999=CARTESIAN_POINT('Ctrl Pts',(5.07403457120051,0.000953086505682821,
24.2083667185208));
#35000=CARTESIAN_POINT('Ctrl Pts',(5.07380195086792,0.845094303182403,24.2348538890889));
#35001=CARTESIAN_POINT('Ctrl Pts',(4.64316632240633,2.53218242822061,24.2877983563415));
#35002=CARTESIAN_POINT('Ctrl Pts',(2.86651231988729,4.4445526734691,24.3671702463949));
#35003=CARTESIAN_POINT('Ctrl Pts',(0.391582261162602,5.27423972531146,24.4465421364484));
#35004=CARTESIAN_POINT('Ctrl Pts',(-2.1787363696294,4.81913365439931,24.5259140265017));
#35005=CARTESIAN_POINT('Ctrl Pts',(-4.21831964333045,3.19009729224708,24.6052859165552));
#35006=CARTESIAN_POINT('Ctrl Pts',(-5.23032958900859,0.783960290863936,
24.6846578066085));
#35007=CARTESIAN_POINT('Ctrl Pts',(-4.9682428239423,-1.81314770210696,24.764029696662));
#35008=CARTESIAN_POINT('Ctrl Pts',(-3.49590310398264,-3.96857692817898,
24.8434015867153));
#35009=CARTESIAN_POINT('Ctrl Pts',(-1.17196912594307,-5.15726959884261,
24.9227734767688));
#35010=CARTESIAN_POINT('Ctrl Pts',(1.43745393706658,-5.08966281065081,25.0021453668222));
#35011=CARTESIAN_POINT('Ctrl Pts',(3.69671640275713,-3.78222542756197,25.0815172568756));
#35012=CARTESIAN_POINT('Ctrl Pts',(4.87329911188321,-1.85225894830422,25.1502477494805));
#35013=CARTESIAN_POINT('Ctrl Pts',(5.07297546809779,-0.504207096881882,
25.192520945401));
#35014=CARTESIAN_POINT('Ctrl Pts',(5.07323119136609,7.2716719250257E-5,
25.2083368446371));
#35015=CARTESIAN_POINT('Origin',(0.,0.,-2.20833684463713));
#35016=CARTESIAN_POINT('',(5.07323420419449,-7.41988534934401E-5,23.2083368446371));
#35017=CARTESIAN_POINT('',(5.07316553675605,-5.48786176412603E-6,23.2916631553629));
#35018=CARTESIAN_POINT('',(5.0736,-1.85409460923845E-12,-2.20833684463713));
#35019=CARTESIAN_POINT('Ctrl Pts',(5.07316569050492,-5.48591970746248E-6,
23.2916631553629));
#35020=CARTESIAN_POINT('Ctrl Pts',(5.07314958741115,0.42768514602335,23.3050764665037));
#35021=CARTESIAN_POINT('Ctrl Pts',(4.91412543793041,1.69899265595715,23.344947074329));
#35022=CARTESIAN_POINT('Ctrl Pts',(3.86415592530766,3.6109888303426,23.4112749788386));
#35023=CARTESIAN_POINT('Ctrl Pts',(1.66640053022393,5.01936755177924,23.4906468688921));
#35024=CARTESIAN_POINT('Ctrl Pts',(-0.937286345425383,5.20503944789203,
23.5700187589454));
#35025=CARTESIAN_POINT('Ctrl Pts',(-3.31265234202061,4.12277525560054,23.6493906489989));
#35026=CARTESIAN_POINT('Ctrl Pts',(-4.88106356050821,2.03621213668325,23.7287625390522));
#35027=CARTESIAN_POINT('Ctrl Pts',(-5.26045849971908,-0.546367751667005,
23.8081344291057));
#35028=CARTESIAN_POINT('Ctrl Pts',(-4.35841739221935,-2.99585366506712,
23.887506319159));
#35029=CARTESIAN_POINT('Ctrl Pts',(-2.3946754551717,-4.71555625687105,23.9668782092125));
#35030=CARTESIAN_POINT('Ctrl Pts',(0.152404122233421,-5.28655978220554,
24.0462500992659));
#35031=CARTESIAN_POINT('Ctrl Pts',(2.66235839280233,-4.56976904619763,24.1256219893193));
#35032=CARTESIAN_POINT('Ctrl Pts',(4.52376805191542,-2.73979268554746,24.2049938793727));
#35033=CARTESIAN_POINT('Ctrl Pts',(5.05332835032277,-0.998334355631039,
24.2603409347206));
#35034=CARTESIAN_POINT('Ctrl Pts',(5.07399526625627,-0.0776027111923523,
24.289230693384));
#35035=CARTESIAN_POINT('Ctrl Pts',(5.07393893245752,-7.63518475176573E-5,
24.2916631553629));
#35036=CARTESIAN_POINT('Ctrl Pts',(5.07323420419449,-7.41988534933707E-5,
23.2083368446371));
#35037=CARTESIAN_POINT('Ctrl Pts',(5.07297208311489,0.506109773689648,23.2242124916405));
#35038=CARTESIAN_POINT('Ctrl Pts',(4.87223466883649,1.85606959653113,23.2665454353283));
#35039=CARTESIAN_POINT('Ctrl Pts',(3.69245444696201,3.78638634033052,23.3353356757007));
#35040=CARTESIAN_POINT('Ctrl Pts',(1.43172095156667,5.09127847004479,23.4147075657541));
#35041=CARTESIAN_POINT('Ctrl Pts',(-1.17777659548102,5.1559464348325,23.4940794558075));
#35042=CARTESIAN_POINT('Ctrl Pts',(-3.50037037246962,3.96463726004727,23.5734513458609));
#35043=CARTESIAN_POINT('Ctrl Pts',(-4.97028167379665,1.80755122457705,23.6528232359143));
#35044=CARTESIAN_POINT('Ctrl Pts',(-5.22944336137752,-0.789850288405212,
23.7321951259677));
#35045=CARTESIAN_POINT('Ctrl Pts',(-4.21472422106041,-3.19484601935549,
23.8115670160211));
#35046=CARTESIAN_POINT('Ctrl Pts',(-2.17330758975551,-4.82158433170509,
23.8909389060745));
#35047=CARTESIAN_POINT('Ctrl Pts',(0.397521959947206,-5.27379537322471,
23.9703107961279));
#35048=CARTESIAN_POINT('Ctrl Pts',(2.87151604007067,-4.4413215351868,24.0496826861813));
#35049=CARTESIAN_POINT('Ctrl Pts',(4.64534728528402,-2.52767212981305,24.129024702351));
#35050=CARTESIAN_POINT('Ctrl Pts',(5.07402451266825,-0.842236060605585,
24.1819094218363));
#35051=CARTESIAN_POINT('Ctrl Pts',(5.07403455984306,1.01136344364921E-6,
24.2083368446371));
#35052=CARTESIAN_POINT('Origin',(0.,0.,-2.20833684463713));
#35053=CARTESIAN_POINT('',(5.07368445537635,0.000127432987209741,22.2083368446371));
#35054=CARTESIAN_POINT('',(5.0739114897015,8.59482686052055E-5,22.2916631553629));
#35055=CARTESIAN_POINT('',(5.0736,-1.85409460923845E-12,-2.20833684463713));
#35056=CARTESIAN_POINT('Ctrl Pts',(5.0739114897015,8.59482686050433E-5,
22.2916631553629));
#35057=CARTESIAN_POINT('Ctrl Pts',(5.07398263122595,0.0893847065795861,
22.2944649429389));
#35058=CARTESIAN_POINT('Ctrl Pts',(5.04987059102411,1.02189374093949,22.3237240271994));
#35059=CARTESIAN_POINT('Ctrl Pts',(4.50458503707303,2.77121862106756,22.3794404081444));
#35060=CARTESIAN_POINT('Ctrl Pts',(2.63048120009391,4.58819259887664,22.4588122981978));
#35061=CARTESIAN_POINT('Ctrl Pts',(0.115597647321455,5.28749259670008,22.5381841882512));
#35062=CARTESIAN_POINT('Ctrl Pts',(-2.42744506809483,4.69877132337436,22.6175560783046));
#35063=CARTESIAN_POINT('Ctrl Pts',(-4.37916762715256,2.96543963879382,22.696927968358));
#35064=CARTESIAN_POINT('Ctrl Pts',(-5.26413459813381,0.509733484286287,
22.7762998584114));
#35065=CARTESIAN_POINT('Ctrl Pts',(-4.86677005798463,-2.07014265165558,
22.8556717484648));
#35066=CARTESIAN_POINT('Ctrl Pts',(-3.28387109087741,-4.14573660239302,
22.9350436385182));
#35067=CARTESIAN_POINT('Ctrl Pts',(-0.901028401772815,-5.21143830245831,
23.0144155285717));
#35068=CARTESIAN_POINT('Ctrl Pts',(1.70130281532621,-5.00764516247504,23.093787418625));
#35069=CARTESIAN_POINT('Ctrl Pts',(3.88920043041414,-3.58400074773866,23.1731593086785));
#35070=CARTESIAN_POINT('Ctrl Pts',(4.92006185002291,-1.67542824897262,23.239117887591));
#35071=CARTESIAN_POINT('Ctrl Pts',(5.07318135021192,-0.415919972782139,
23.2786191698192));
#35072=CARTESIAN_POINT('Ctrl Pts',(5.07316569050492,-5.48591970746248E-6,
23.2916631553629));
#35073=CARTESIAN_POINT('Ctrl Pts',(5.07368445537635,0.000127432987209863,
22.2083368446371));
#35074=CARTESIAN_POINT('Ctrl Pts',(5.07385799503573,0.167927931732477,22.2136009680757));
#35075=CARTESIAN_POINT('Ctrl Pts',(5.02468445773871,1.17898674996513,22.2453223881989));
#35076=CARTESIAN_POINT('Ctrl Pts',(4.37115162329097,2.97723307464397,22.3035011050064));
#35077=CARTESIAN_POINT('Ctrl Pts',(2.4147715124657,4.70529942618521,22.3828729950599));
#35078=CARTESIAN_POINT('Ctrl Pts',(-0.129853572474074,5.28716128664959,
22.4622448851132));
#35079=CARTESIAN_POINT('Ctrl Pts',(-2.64284027062663,4.58108446095525,22.5416167751666));
#35080=CARTESIAN_POINT('Ctrl Pts',(-4.51204028846786,2.7590644882843,22.62098866522));
#35081=CARTESIAN_POINT('Ctrl Pts',(-5.28211549991429,0.264943102456049,
22.7003605552734));
#35082=CARTESIAN_POINT('Ctrl Pts',(-4.76548000969985,-2.2937181486802,22.7797324453269));
#35083=CARTESIAN_POINT('Ctrl Pts',(-3.08798363825926,-4.29363457062517,
22.8591043353802));
#35084=CARTESIAN_POINT('Ctrl Pts',(-0.658261551986295,-5.24763120247219,
22.9384762254337));
#35085=CARTESIAN_POINT('Ctrl Pts',(1.93181173129385,-4.92331644248731,23.017848115487));
#35086=CARTESIAN_POINT('Ctrl Pts',(4.05129987868926,-3.39969271923279,23.0972200055405));
#35087=CARTESIAN_POINT('Ctrl Pts',(4.95736217363157,-1.51830523331034,23.1607162485905));
#35088=CARTESIAN_POINT('Ctrl Pts',(5.07340891666056,-0.3374627456306,23.197755194956));
#35089=CARTESIAN_POINT('Ctrl Pts',(5.07323420419449,-7.41988534933707E-5,
23.2083368446371));
#35090=CARTESIAN_POINT('Origin',(0.,0.,-2.20833684463713));
#35091=CARTESIAN_POINT('',(5.0647135783285,-0.000493560823505712,21.2083368446371));
#35092=CARTESIAN_POINT('',(5.07311795825563,-0.000541267147824199,21.2916631553629));
#35093=CARTESIAN_POINT('',(5.0736,-1.85409460923845E-12,-2.20833684463713));
#35094=CARTESIAN_POINT('Ctrl Pts',(5.07311795825563,-0.000541267147824084,
21.2916631553629));
#35095=CARTESIAN_POINT('Ctrl Pts',(5.07265472641037,0.594063927299599,21.3103107160587));
#35096=CARTESIAN_POINT('Ctrl Pts',(4.82066183061084,2.03342224951305,21.3554155734389));
#35097=CARTESIAN_POINT('Ctrl Pts',(3.48937383888172,3.97367066688458,21.4269777275036));
#35098=CARTESIAN_POINT('Ctrl Pts',(1.16402860508423,5.15930893371516,21.5063496175569));
#35099=CARTESIAN_POINT('Ctrl Pts',(-1.44552439996815,5.08729102078623,21.5857215076104));
#35100=CARTESIAN_POINT('Ctrl Pts',(-3.70260503654192,3.77647571272897,21.6650933976637));
#35101=CARTESIAN_POINT('Ctrl Pts',(-5.057922432142,1.54547807796832,21.7444652877172));
#35102=CARTESIAN_POINT('Ctrl Pts',(-5.18104412158608,-1.06186685398839,
21.8238371777705));
#35103=CARTESIAN_POINT('Ctrl Pts',(-4.04212630117128,-3.41061102326193,
21.903209067824));
#35104=CARTESIAN_POINT('Ctrl Pts',(-1.91852825506946,-4.92850206746972,
21.9825809578774));
#35105=CARTESIAN_POINT('Ctrl Pts',(0.672404619068471,-5.245839892308,22.0619528479308));
#35106=CARTESIAN_POINT('Ctrl Pts',(3.09954884704109,-4.28529268150223,22.1413247379842));
#35107=CARTESIAN_POINT('Ctrl Pts',(4.71262161876037,-2.35161833566565,22.2178948404616));
#35108=CARTESIAN_POINT('Ctrl Pts',(5.07331084138903,-0.753863997357442,
22.2680076462545));
#35109=CARTESIAN_POINT('Ctrl Pts',(5.0739114897015,8.59482686050433E-5,
22.2916631553629));
#35110=CARTESIAN_POINT('Ctrl Pts',(5.0647135783285,-0.000493560823505643,
21.2083368446371));
#35111=CARTESIAN_POINT('Ctrl Pts',(5.06741194864459,0.674127865172368,21.2294467411954));
#35112=CARTESIAN_POINT('Ctrl Pts',(4.7845254230904,2.19368980981962,21.2770139344383));
#35113=CARTESIAN_POINT('Ctrl Pts',(3.29092685490723,4.12830747359771,21.3510384243656));
#35114=CARTESIAN_POINT('Ctrl Pts',(0.929079443196039,5.20946188754723,21.430410314419));
#35115=CARTESIAN_POINT('Ctrl Pts',(-1.68303999757346,5.01382783115869,21.5097822044724));
#35116=CARTESIAN_POINT('Ctrl Pts',(-3.8722246926078,3.60110493868854,21.5891540945258));
#35117=CARTESIAN_POINT('Ctrl Pts',(-5.12503498129818,1.30888173016128,21.6685259845792));
#35118=CARTESIAN_POINT('Ctrl Pts',(-5.12574462250326,-1.300972874894,21.7478978746326));
#35119=CARTESIAN_POINT('Ctrl Pts',(-3.87976959979778,-3.59455409188016,
21.827269764686));
#35120=CARTESIAN_POINT('Ctrl Pts',(-1.68766624540451,-5.01217052435348,
21.9066416547394));
#35121=CARTESIAN_POINT('Ctrl Pts',(0.915005995631755,-5.2090130440819,21.9860135447928));
#35122=CARTESIAN_POINT('Ctrl Pts',(3.29507231119182,-4.13685632854986,22.0653854348462));
#35123=CARTESIAN_POINT('Ctrl Pts',(4.76770779675958,-2.19496036885575,22.139493201461));
#35124=CARTESIAN_POINT('Ctrl Pts',(5.07298579089609,-0.675431391209716,
22.1871436713913));
#35125=CARTESIAN_POINT('Ctrl Pts',(5.07368445537635,0.000127432987209863,
22.2083368446371));
#35126=CARTESIAN_POINT('Origin',(0.,0.,-2.20833684463713));
#35127=CARTESIAN_POINT('',(5.07022284182504,-0.00437131830465176,20.2083368446371));
#35128=CARTESIAN_POINT('',(5.07763086250027,0.00422747191343611,20.2916631553629));
#35129=CARTESIAN_POINT('',(5.0736,-1.85409460923845E-12,-2.20833684463713));
#35130=CARTESIAN_POINT('Ctrl Pts',(5.07763086250027,0.00422747191343598,
20.2916631553629));
#35131=CARTESIAN_POINT('Ctrl Pts',(5.07981016603818,0.259793667372929,20.2996991924939));
#35132=CARTESIAN_POINT('Ctrl Pts',(4.94610737387947,2.19579442888697,20.3606498229938));
#35133=CARTESIAN_POINT('Ctrl Pts',(2.45559119020176,5.46873373673919,20.4745150468627));
#35134=CARTESIAN_POINT('Ctrl Pts',(-3.26379011618977,5.03400372054189,20.6332588269695));
#35135=CARTESIAN_POINT('Ctrl Pts',(-5.99600976813329,-0.0197068834827358,
20.7920026070763));
#35136=CARTESIAN_POINT('Ctrl Pts',(-3.70230252414087,-4.19446206534972,
20.9242890904987));
#35137=CARTESIAN_POINT('Ctrl Pts',(-0.376480053418488,-5.26605971579228,
21.0301182772365));
#35138=CARTESIAN_POINT('Ctrl Pts',(2.18257651229242,-4.8205851862161,21.10949016729));
#35139=CARTESIAN_POINT('Ctrl Pts',(4.22530652207796,-3.18086119603153,21.1888620573433));
#35140=CARTESIAN_POINT('Ctrl Pts',(4.99434160286696,-1.34186431057878,21.249586386701));
#35141=CARTESIAN_POINT('Ctrl Pts',(5.07331196316984,-0.249566309185764,
21.2838534193742));
#35142=CARTESIAN_POINT('Ctrl Pts',(5.07311795825563,-0.000541267147824084,
21.2916631553629));
#35143=CARTESIAN_POINT('Ctrl Pts',(5.07022284182504,-0.00437131830465176,
20.2083368446371));
#35144=CARTESIAN_POINT('Ctrl Pts',(5.06064558604025,1.17531423721709,20.2452925143152));
#35145=CARTESIAN_POINT('Ctrl Pts',(4.06283412548092,4.05874270439873,20.3351627773622));
#35146=CARTESIAN_POINT('Ctrl Pts',(-0.73672307947618,5.95134306184733,20.4779476337782));
#35147=CARTESIAN_POINT('Ctrl Pts',(-5.3995463563661,2.60828838171381,20.6366914138849));
#35148=CARTESIAN_POINT('Ctrl Pts',(-5.1196790448508,-3.11863163173554,20.7954351939918));
#35149=CARTESIAN_POINT('Ctrl Pts',(-0.158509478954971,-5.99736559883163,
20.9541789740985));
#35150=CARTESIAN_POINT('Ctrl Pts',(4.27441519030586,-3.72585141387614,21.091812857647));
#35151=CARTESIAN_POINT('Ctrl Pts',(5.06064814629056,-1.01689503187705,21.1765321478265));
#35152=CARTESIAN_POINT('Ctrl Pts',(5.0647135783285,-0.000493560823505643,
21.2083368446371));
#35153=CARTESIAN_POINT('Origin',(0.,0.,-2.20833684463713));
#35154=CARTESIAN_POINT('',(5.08190747034449,-0.0016131106486481,19.2083368446371));
#35155=CARTESIAN_POINT('',(5.0654395261759,0.00158764291868628,19.2916631553629));
#35156=CARTESIAN_POINT('',(5.0736,-1.85409460923845E-12,-2.20833684463713));
#35157=CARTESIAN_POINT('Ctrl Pts',(5.0654395261759,0.00158764291868674,
19.2916631553629));
#35158=CARTESIAN_POINT('Ctrl Pts',(5.06734596007678,0.765537039397172,19.3155449656136));
#35159=CARTESIAN_POINT('Ctrl Pts',(4.5467586954857,3.21970245674355,19.3923413692333));
#35160=CARTESIAN_POINT('Ctrl Pts',(0.736723079475925,5.95134306184737,19.5220523662219));
#35161=CARTESIAN_POINT('Ctrl Pts',(-4.59927593805429,3.84720861430001,19.6807961463287));
#35162=CARTESIAN_POINT('Ctrl Pts',(-5.72720375155086,-1.77677009197966,
19.8395399264355));
#35163=CARTESIAN_POINT('Ctrl Pts',(-1.61419617037545,-5.77483540889735,
19.9982837065423));
#35164=CARTESIAN_POINT('Ctrl Pts',(3.69280075007907,-4.55444079317796,20.1489914495181));
#35165=CARTESIAN_POINT('Ctrl Pts',(5.0654601874783,-1.42302350869954,20.246784599125));
#35166=CARTESIAN_POINT('Ctrl Pts',(5.07763086250027,0.00422747191343598,
20.2916631553629));
#35167=CARTESIAN_POINT('Ctrl Pts',(5.08190747034449,-0.00161311064864815,
19.2083368446371));
#35168=CARTESIAN_POINT('Ctrl Pts',(5.08137262398886,1.67206424053112,19.2611382874349));
#35169=CARTESIAN_POINT('Ctrl Pts',(3.25971341308398,5.0343135906333,19.3668543236016));
#35170=CARTESIAN_POINT('Ctrl Pts',(-2.45559119020206,5.46873373673905,19.5254849531373));
#35171=CARTESIAN_POINT('Ctrl Pts',(-5.92771323046149,0.905806267444168,
19.6842287332441));
#35172=CARTESIAN_POINT('Ctrl Pts',(-3.97578039972873,-4.48936692070992,
19.8429725133509));
#35173=CARTESIAN_POINT('Ctrl Pts',(1.61419617037569,-5.77483540889728,20.0017162934577));
#35174=CARTESIAN_POINT('Ctrl Pts',(4.76969253787625,-2.70752266133374,20.1235044038864));
#35175=CARTESIAN_POINT('Ctrl Pts',(5.0743586806711,-0.513806323102652,20.1923779209462));
#35176=CARTESIAN_POINT('Ctrl Pts',(5.07022284182504,-0.00437131830465176,
20.2083368446371));
#35177=CARTESIAN_POINT('Origin',(0.,0.,-2.20833684463713));
#35178=CARTESIAN_POINT('',(5.07322996641872,-7.44046081432859E-5,18.2083368446371));
#35179=CARTESIAN_POINT('',(5.0733324096026,-5.65345686568016E-5,18.2916631553629));
#35180=CARTESIAN_POINT('',(5.0736,-1.85409460923845E-12,-2.20833684463713));
#35181=CARTESIAN_POINT('Ctrl Pts',(5.0733324096026,-5.65345686565077E-5,
18.2916631553629));
#35182=CARTESIAN_POINT('Ctrl Pts',(5.07342932055268,0.423040487316443,18.3049334420489));
#35183=CARTESIAN_POINT('Ctrl Pts',(4.9168904884294,1.68971643561363,18.3446610254193));
#35184=CARTESIAN_POINT('Ctrl Pts',(3.87222469260764,3.60110493868871,18.4108459054742));
#35185=CARTESIAN_POINT('Ctrl Pts',(1.68303999757325,5.01382783115876,18.4902177955276));
#35186=CARTESIAN_POINT('Ctrl Pts',(-0.929079443196312,5.2094618875472,18.569589685581));
#35187=CARTESIAN_POINT('Ctrl Pts',(-3.29092685490746,4.12830747359753,18.6489615756344));
#35188=CARTESIAN_POINT('Ctrl Pts',(-5.42625155540715,1.36247937795741,18.7547907623723));
#35189=CARTESIAN_POINT('Ctrl Pts',(-4.95432466322409,-3.37745298000962,
18.8870772457946));
#35190=CARTESIAN_POINT('Ctrl Pts',(0.158509478955228,-5.99736559883162,
19.0458210259014));
#35191=CARTESIAN_POINT('Ctrl Pts',(4.3733083201864,-3.5517155504766,19.1806829957575));
#35192=CARTESIAN_POINT('Ctrl Pts',(5.06312190111345,-0.927134966817506,
19.2626303722447));
#35193=CARTESIAN_POINT('Ctrl Pts',(5.0654395261759,0.00158764291868674,
19.2916631553629));
#35194=CARTESIAN_POINT('Ctrl Pts',(5.07322996641872,-7.44046081432165E-5,
18.2083368446371));
#35195=CARTESIAN_POINT('Ctrl Pts',(5.07298661447134,0.501546775803683,18.2240694671857));
#35196=CARTESIAN_POINT('Ctrl Pts',(4.87479289587003,1.8469289142109,18.2662593864187));
#35197=CARTESIAN_POINT('Ctrl Pts',(3.70260503654169,3.77647571272922,18.3349066023362));
#35198=CARTESIAN_POINT('Ctrl Pts',(1.44552439996779,5.08729102078633,18.4142784923897));
#35199=CARTESIAN_POINT('Ctrl Pts',(-1.16402860508455,5.15930893371508,18.4936503824431));
#35200=CARTESIAN_POINT('Ctrl Pts',(-3.48937383888192,3.97367066688439,18.5730222724965));
#35201=CARTESIAN_POINT('Ctrl Pts',(-4.96594823061187,1.82167865277138,18.6523941625499));
#35202=CARTESIAN_POINT('Ctrl Pts',(-5.23050112077116,-0.77713504302674,
18.7317660526033));
#35203=CARTESIAN_POINT('Ctrl Pts',(-4.22530652207786,-3.18086119603167,
18.8111379426567));
#35204=CARTESIAN_POINT('Ctrl Pts',(-2.18257651229225,-4.82058518621618,
18.8905098327101));
#35205=CARTESIAN_POINT('Ctrl Pts',(0.37648005341871,-5.26605971579227,18.9698817227635));
#35206=CARTESIAN_POINT('Ctrl Pts',(3.70230252414111,-4.19446206534953,19.0757109095013));
#35207=CARTESIAN_POINT('Ctrl Pts',(5.08048878136776,-1.68603810060634,19.1551959501259));
#35208=CARTESIAN_POINT('Ctrl Pts',(5.08190861649065,-0.00519970863047212,
19.2082236940659));
#35209=CARTESIAN_POINT('Ctrl Pts',(5.08190747034449,-0.00161311064864815,
19.2083368446371));
#35210=CARTESIAN_POINT('Origin',(0.,0.,-2.20833684463713));
#35211=CARTESIAN_POINT('',(5.07369825422177,0.000126003717071388,17.2083368446371));
#35212=CARTESIAN_POINT('',(5.07392231800261,8.23068815517256E-5,17.2916631553629));
#35213=CARTESIAN_POINT('',(5.0736,-1.85409460923845E-12,-2.20833684463713));
#35214=CARTESIAN_POINT('Ctrl Pts',(5.07392231800261,8.23068815519051E-5,
17.2916631553629));
#35215=CARTESIAN_POINT('Ctrl Pts',(5.07398762507078,0.0848220371273371,
17.2943219184842));
#35216=CARTESIAN_POINT('Ctrl Pts',(5.05121938853888,1.01276996498335,17.3234379782898));
#35217=CARTESIAN_POINT('Ctrl Pts',(4.51204028846775,2.7590644882845,17.3790113347799));
#35218=CARTESIAN_POINT('Ctrl Pts',(2.64284027062647,4.58108446095533,17.4583832248334));
#35219=CARTESIAN_POINT('Ctrl Pts',(0.129853572473924,5.28716128664959,17.5377551148867));
#35220=CARTESIAN_POINT('Ctrl Pts',(-2.41477151246584,4.70529942618515,17.6171270049402));
#35221=CARTESIAN_POINT('Ctrl Pts',(-4.37115162329109,2.9772330746438,17.6964988949936));
#35222=CARTESIAN_POINT('Ctrl Pts',(-5.2627514922539,0.523926824466488,17.775870785047));
#35223=CARTESIAN_POINT('Ctrl Pts',(-4.87231403886184,-2.05702097999283,
17.8552426751004));
#35224=CARTESIAN_POINT('Ctrl Pts',(-3.29507231119166,-4.13685632854999,
17.9346145651538));
#35225=CARTESIAN_POINT('Ctrl Pts',(-0.915005995631555,-5.20901304408194,
18.0139864552072));
#35226=CARTESIAN_POINT('Ctrl Pts',(1.68766624540468,-5.01217052435341,18.0933583452606));
#35227=CARTESIAN_POINT('Ctrl Pts',(3.8797695997979,-3.59455409188004,18.172730235314));
#35228=CARTESIAN_POINT('Ctrl Pts',(4.9174284825737,-1.68443961943593,18.2388318386815));
#35229=CARTESIAN_POINT('Ctrl Pts',(5.07323610680991,-0.420498442869185,
18.2784761453644));
#35230=CARTESIAN_POINT('Ctrl Pts',(5.0733324096026,-5.65345686565077E-5,
18.2916631553629));
#35231=CARTESIAN_POINT('Ctrl Pts',(5.07369825422177,0.000126003717071926,
17.2083368446371));
#35232=CARTESIAN_POINT('Ctrl Pts',(5.07386566986272,0.163365799600409,17.2134579436209));
#35233=CARTESIAN_POINT('Ctrl Pts',(5.02624395147431,1.16985927909857,17.2450363392892));
#35234=CARTESIAN_POINT('Ctrl Pts',(4.37916762715237,2.96543963879408,17.303072031642));
#35235=CARTESIAN_POINT('Ctrl Pts',(2.42744506809458,4.69877132337447,17.3824439216954));
#35236=CARTESIAN_POINT('Ctrl Pts',(-0.115597647321682,5.28749259670007,
17.4618158117488));
#35237=CARTESIAN_POINT('Ctrl Pts',(-2.63048120009413,4.58819259887652,17.5411877018022));
#35238=CARTESIAN_POINT('Ctrl Pts',(-4.5045850370732,2.7712186210673,17.6205595918556));
#35239=CARTESIAN_POINT('Ctrl Pts',(-5.28138253005218,0.27918271172893,17.699931481909));
#35240=CARTESIAN_POINT('Ctrl Pts',(-4.77164579536179,-2.28086298099153,
17.7793033719624));
#35241=CARTESIAN_POINT('Ctrl Pts',(-3.09954884704088,-4.28529268150238,
17.8586752620158));
#35242=CARTESIAN_POINT('Ctrl Pts',(-0.672404619068171,-5.24583989230806,
17.9380471520692));
#35243=CARTESIAN_POINT('Ctrl Pts',(1.91852825506979,-4.9285020674696,18.0174190421226));
#35244=CARTESIAN_POINT('Ctrl Pts',(4.04212630117149,-3.41061102326166,18.096790932176));
#35245=CARTESIAN_POINT('Ctrl Pts',(4.95529462550652,-1.52742091164643,18.1604301996809));
#35246=CARTESIAN_POINT('Ctrl Pts',(5.07339585550224,-0.342021443822988,
18.1976121705012));
#35247=CARTESIAN_POINT('Ctrl Pts',(5.07322996641872,-7.44046081432165E-5,
18.2083368446371));
#35248=CARTESIAN_POINT('Origin',(0.,0.,-2.20833684463713));
#35249=CARTESIAN_POINT('',(5.07366101292862,-0.000128884195875409,16.2083368446371));
#35250=CARTESIAN_POINT('',(5.07342183474754,-0.000122761774360241,16.2916631553629));
#35251=CARTESIAN_POINT('',(5.0736,-1.85409460923845E-12,-2.20833684463713));
#35252=CARTESIAN_POINT('Ctrl Pts',(5.07342183474754,-0.000122761774360089,
16.2916631553629));
#35253=CARTESIAN_POINT('Ctrl Pts',(5.07288953552851,0.589818979702204,16.3101676916039));
#35254=CARTESIAN_POINT('Ctrl Pts',(4.82300217163475,2.02368301235074,16.3551295245292));
#35255=CARTESIAN_POINT('Ctrl Pts',(3.50037037246945,3.9646372600474,16.4265486541391));
#35256=CARTESIAN_POINT('Ctrl Pts',(1.17777659548083,5.15594643483254,16.5059205441925));
#35257=CARTESIAN_POINT('Ctrl Pts',(-1.43172095156687,5.09127847004474,16.5852924342459));
#35258=CARTESIAN_POINT('Ctrl Pts',(-3.69245444696213,3.78638634033038,16.6646643242993));
#35259=CARTESIAN_POINT('Ctrl Pts',(-5.05371420635461,1.5591388772047,16.7440362143527));
#35260=CARTESIAN_POINT('Ctrl Pts',(-5.18390038229795,-1.04791136166686,
16.8234081044061));
#35261=CARTESIAN_POINT('Ctrl Pts',(-4.05129987868913,-3.39969271923294,
16.9027799944595));
#35262=CARTESIAN_POINT('Ctrl Pts',(-1.93181173129365,-4.9233164424874,16.9821518845129));
#35263=CARTESIAN_POINT('Ctrl Pts',(0.658261551986501,-5.24763120247215,
17.0615237745663));
#35264=CARTESIAN_POINT('Ctrl Pts',(3.08798363825942,-4.29363457062506,17.1408956646198));
#35265=CARTESIAN_POINT('Ctrl Pts',(4.70928800664519,-2.36071043051411,17.2176087915519));
#35266=CARTESIAN_POINT('Ctrl Pts',(5.0733377557896,-0.758421261304332,17.2678646217997));
#35267=CARTESIAN_POINT('Ctrl Pts',(5.07392231800261,8.23068815519051E-5,
17.2916631553629));
#35268=CARTESIAN_POINT('Ctrl Pts',(5.07366101292862,-0.000128884195875374,
16.2083368446371));
#35269=CARTESIAN_POINT('Ctrl Pts',(5.07297133880781,0.668223813333716,16.2293037167406));
#35270=CARTESIAN_POINT('Ctrl Pts',(4.77257120255655,2.18054683036438,16.2767278855287));
#35271=CARTESIAN_POINT('Ctrl Pts',(3.31265234202039,4.12277525560071,16.3506093510011));
#35272=CARTESIAN_POINT('Ctrl Pts',(0.937286345425132,5.20503944789207,16.4299812410546));
#35273=CARTESIAN_POINT('Ctrl Pts',(-1.66640053022416,5.01936755177917,16.509353131108));
#35274=CARTESIAN_POINT('Ctrl Pts',(-3.86415592530783,3.6109888303424,16.5887250211614));
#35275=CARTESIAN_POINT('Ctrl Pts',(-5.12061148999576,1.32298122241861,16.6680969112148));
#35276=CARTESIAN_POINT('Ctrl Pts',(-5.1296974302943,-1.28730168253218,16.7474688012682));
#35277=CARTESIAN_POINT('Ctrl Pts',(-3.88920043041393,-3.58400074773889,
16.8268406913216));
#35278=CARTESIAN_POINT('Ctrl Pts',(-1.70130281532588,-5.00764516247516,
16.906212581375));
#35279=CARTESIAN_POINT('Ctrl Pts',(0.90102840177319,-5.21143830245825,16.9855844714284));
#35280=CARTESIAN_POINT('Ctrl Pts',(3.28387109087768,-4.1457366023928,17.0649563614818));
#35281=CARTESIAN_POINT('Ctrl Pts',(4.76464092528408,-2.20406061763576,17.1392071525514));
#35282=CARTESIAN_POINT('Ctrl Pts',(5.07300074510805,-0.679985153784537,
17.1870006469365));
#35283=CARTESIAN_POINT('Ctrl Pts',(5.07369825422177,0.000126003717071926,
17.2083368446371));
#35284=CARTESIAN_POINT('Origin',(0.,0.,-2.20833684463713));
#35285=CARTESIAN_POINT('',(5.07324617544329,7.96922658102828E-5,15.2083368446371));
#35286=CARTESIAN_POINT('',(5.07342714732068,0.00012340910666319,15.2916631553629));
#35287=CARTESIAN_POINT('',(5.0736,-1.85409460923845E-12,-2.20833684463713));
#35288=CARTESIAN_POINT('Ctrl Pts',(5.07342714732068,0.000123409106663336,
15.2916631553629));
#35289=CARTESIAN_POINT('Ctrl Pts',(5.07365576358557,0.251759202071401,15.2995561680391));
#35290=CARTESIAN_POINT('Ctrl Pts',(4.99363067660841,1.34673145111339,15.3339064773998));
#35291=CARTESIAN_POINT('Ctrl Pts',(4.21831964333036,3.19009729224721,15.3947140834449));
#35292=CARTESIAN_POINT('Ctrl Pts',(2.17873636962922,4.81913365439941,15.4740859734983));
#35293=CARTESIAN_POINT('Ctrl Pts',(-0.391582261162836,5.27423972531144,
15.5534578635517));
#35294=CARTESIAN_POINT('Ctrl Pts',(-2.86651231988745,4.44455267346898,15.6328297536051));
#35295=CARTESIAN_POINT('Ctrl Pts',(-4.64316632240643,2.53218242822043,15.7122016436585));
#35296=CARTESIAN_POINT('Ctrl Pts',(-5.28875528625864,0.00297814834715876,
15.7915735337119));
#35297=CARTESIAN_POINT('Ctrl Pts',(-4.64601516884489,-2.52695160186966,
15.8709454237653));
#35298=CARTESIAN_POINT('Ctrl Pts',(-2.87151604007055,-4.44132153518687,
15.9503173138187));
#35299=CARTESIAN_POINT('Ctrl Pts',(-0.397521959947054,-5.27379537322474,
16.0296892038721));
#35300=CARTESIAN_POINT('Ctrl Pts',(2.1733075897557,-4.82158433170501,16.1090610939255));
#35301=CARTESIAN_POINT('Ctrl Pts',(4.21472422106055,-3.1948460193553,16.1884329839789));
#35302=CARTESIAN_POINT('Ctrl Pts',(4.99287463290549,-1.35054413899492,16.2493003377914));
#35303=CARTESIAN_POINT('Ctrl Pts',(5.07365060287866,-0.253664125066255,
16.2837103949194));
#35304=CARTESIAN_POINT('Ctrl Pts',(5.07342183474754,-0.000122761774360089,
16.2916631553629));
#35305=CARTESIAN_POINT('Ctrl Pts',(5.07324617544329,7.96922658102828E-5,
15.2083368446371));
#35306=CARTESIAN_POINT('Ctrl Pts',(5.07343036424897,0.330250553788653,15.2186921931759));
#35307=CARTESIAN_POINT('Ctrl Pts',(4.96059306642381,1.5038639780885,15.2555048383992));
#35308=CARTESIAN_POINT('Ctrl Pts',(4.06576497321036,3.38238030533612,15.3187747803069));
#35309=CARTESIAN_POINT('Ctrl Pts',(1.95279534724736,4.91503119817963,15.3981466703603));
#35310=CARTESIAN_POINT('Ctrl Pts',(-0.635870902865948,5.2503913703836,15.4775185604137));
#35311=CARTESIAN_POINT('Ctrl Pts',(-3.06964040851742,4.30676782630626,15.5568904504671));
#35312=CARTESIAN_POINT('Ctrl Pts',(-4.75565230518791,2.31402517260967,15.6362623405205));
#35313=CARTESIAN_POINT('Ctrl Pts',(-5.28319782677237,-0.24240889112691,
15.7156342305739));
#35314=CARTESIAN_POINT('Ctrl Pts',(-4.52376805191524,-2.73979268554778,
15.7950061206273));
#35315=CARTESIAN_POINT('Ctrl Pts',(-2.66235839280204,-4.56976904619777,
15.8743780106807));
#35316=CARTESIAN_POINT('Ctrl Pts',(-0.15240412223312,-5.28655978220556,
15.9537499007341));
#35317=CARTESIAN_POINT('Ctrl Pts',(2.39467545517194,-4.71555625687092,16.0331217907875));
#35318=CARTESIAN_POINT('Ctrl Pts',(4.35841739221953,-2.99585366506689,16.112493680841));
#35319=CARTESIAN_POINT('Ctrl Pts',(5.02217539318898,-1.19342375387563,16.1708986987908));
#35320=CARTESIAN_POINT('Ctrl Pts',(5.0738416122916,-0.175144979162809,16.2028464200562));
#35321=CARTESIAN_POINT('Ctrl Pts',(5.07366101292862,-0.000128884195875374,
16.2083368446371));
#35322=CARTESIAN_POINT('Origin',(0.,0.,-2.20833684463713));
#35323=CARTESIAN_POINT('',(5.07403332299931,-8.66482790312043E-6,14.2083368446371));
#35324=CARTESIAN_POINT('',(5.07391786048903,-8.38031740753252E-5,14.2916631553629));
#35325=CARTESIAN_POINT('',(5.0736,-1.85409460923845E-12,-2.20833684463713));
#35326=CARTESIAN_POINT('Ctrl Pts',(5.07391786048903,-8.38031740754523E-5,
14.2916631553629));
#35327=CARTESIAN_POINT('Ctrl Pts',(5.07332646114364,0.756517455027875,14.3154019411588));
#35328=CARTESIAN_POINT('Ctrl Pts',(4.7106825315255,2.35691208085668,14.3655980236392));
#35329=CARTESIAN_POINT('Ctrl Pts',(3.09281731455568,4.29015412381589,14.442251402804));
#35330=CARTESIAN_POINT('Ctrl Pts',(0.664171081076821,5.24688651700904,14.5216232928574));
#35331=CARTESIAN_POINT('Ctrl Pts',(-1.92626575763464,4.9254889684451,14.6009951829108));
#35332=CARTESIAN_POINT('Ctrl Pts',(-4.04746852150321,3.4042532095528,14.6803670729642));
#35333=CARTESIAN_POINT('Ctrl Pts',(-5.1827169124532,1.05374890400015,14.7597389630177));
#35334=CARTESIAN_POINT('Ctrl Pts',(-5.05546693527891,-1.55344630213332,
14.839110853071));
#35335=CARTESIAN_POINT('Ctrl Pts',(-3.69671640275692,-3.78222542756219,
14.9184827431245));
#35336=CARTESIAN_POINT('Ctrl Pts',(-1.43745393706629,-5.08966281065088,
14.9978546331779));
#35337=CARTESIAN_POINT('Ctrl Pts',(1.17196912594334,-5.15726959884254,15.0772265232312));
#35338=CARTESIAN_POINT('Ctrl Pts',(3.49590310398282,-3.96857692817882,15.1565984132847));
#35339=CARTESIAN_POINT('Ctrl Pts',(4.82182831793198,-2.02749096887971,15.2280772906619));
#35340=CARTESIAN_POINT('Ctrl Pts',(5.07288944423512,-0.591721367900843,
15.2730988713546));
#35341=CARTESIAN_POINT('Ctrl Pts',(5.07342714732068,0.000123409106663336,
15.2916631553629));
#35342=CARTESIAN_POINT('Ctrl Pts',(5.07403332299931,-8.66482790325162E-6,
14.2083368446371));
#35343=CARTESIAN_POINT('Ctrl Pts',(5.07395003551347,0.835016825572543,14.2345379662956));
#35344=CARTESIAN_POINT('Ctrl Pts',(4.65105118571099,2.51331333377907,14.2871963846386));
#35345=CARTESIAN_POINT('Ctrl Pts',(2.89043509646017,4.42903220810837,14.3663120996661));
#35346=CARTESIAN_POINT('Ctrl Pts',(0.420014577610126,5.27205169757513,14.4456839897195));
#35347=CARTESIAN_POINT('Ctrl Pts',(-2.15272056265924,4.83081106300113,14.5250558797729));
#35348=CARTESIAN_POINT('Ctrl Pts',(-4.201057738831,3.21279554629894,14.6044277698263));
#35349=CARTESIAN_POINT('Ctrl Pts',(-5.22602654870706,0.81215014592063,14.6837996598797));
#35350=CARTESIAN_POINT('Ctrl Pts',(-4.97794685893165,-1.78633323234006,
14.7631715499331));
#35351=CARTESIAN_POINT('Ctrl Pts',(-3.51725033281897,-3.94966978918425,
14.8425434399865));
#35352=CARTESIAN_POINT('Ctrl Pts',(-1.19975941093315,-5.15087552782897,
14.9219153300399));
#35353=CARTESIAN_POINT('Ctrl Pts',(1.40999024783357,-5.09733938916413,15.0012872200933));
#35354=CARTESIAN_POINT('Ctrl Pts',(3.67626940318851,-3.8021026580683,15.0806591101467));
#35355=CARTESIAN_POINT('Ctrl Pts',(4.86818118380815,-1.87050241988135,15.1496756516613));
#35356=CARTESIAN_POINT('Ctrl Pts',(5.07295977285751,-0.513316266501481,
15.1922348964914));
#35357=CARTESIAN_POINT('Ctrl Pts',(5.07324617544329,7.96922658102828E-5,
15.2083368446371));
#35358=CARTESIAN_POINT('Origin',(0.,0.,-2.20833684463713));
#35359=CARTESIAN_POINT('',(5.07322036085286,-6.69861637152269E-5,13.2083368446371));
#35360=CARTESIAN_POINT('',(5.07316540514723,3.01288341894208E-6,13.2916631553629));
#35361=CARTESIAN_POINT('',(5.0736,-1.85409460923845E-12,-2.20833684463713));
#35362=CARTESIAN_POINT('Ctrl Pts',(5.07316545149283,3.01256212205392E-6,
13.2916631553629));
#35363=CARTESIAN_POINT('Ctrl Pts',(5.07317410528241,0.418572877762161,13.3047904175941));
#35364=CARTESIAN_POINT('Ctrl Pts',(4.91873112752187,1.68074170142874,13.3443749765097));
#35365=CARTESIAN_POINT('Ctrl Pts',(3.8835697329937,3.59010131838716,13.4104168321098));
#35366=CARTESIAN_POINT('Ctrl Pts',(1.69344007832116,5.01030957610862,13.4897887221632));
#35367=CARTESIAN_POINT('Ctrl Pts',(-0.909207831064397,5.21001751122212,
13.5691606122166));
#35368=CARTESIAN_POINT('Ctrl Pts',(-3.29037472530003,4.14057671278008,13.64853250227));
#35369=CARTESIAN_POINT('Ctrl Pts',(-4.87001361957351,2.06250059211591,13.7279043923234));
#35370=CARTESIAN_POINT('Ctrl Pts',(-5.26332797571119,-0.517996107520081,
13.8072762823768));
#35371=CARTESIAN_POINT('Ctrl Pts',(-4.37450728714447,-2.97231010192914,
13.8866481724302));
#35372=CARTESIAN_POINT('Ctrl Pts',(-2.420066306237,-4.70257593460501,13.9660200624836));
#35373=CARTESIAN_POINT('Ctrl Pts',(0.123897470143854,-5.28730467858643,
14.045391952537));
#35374=CARTESIAN_POINT('Ctrl Pts',(2.63768009704007,-4.58405770611459,14.1247638425904));
#35375=CARTESIAN_POINT('Ctrl Pts',(4.50892969070322,-2.76414442307289,14.2041357326438));
#35376=CARTESIAN_POINT('Ctrl Pts',(5.05065740926092,-1.01658127603429,14.2597688369013));
#35377=CARTESIAN_POINT('Ctrl Pts',(5.07398558617533,-0.0867280307438605,
14.2889446444744));
#35378=CARTESIAN_POINT('Ctrl Pts',(5.07391786048903,-8.38031740754523E-5,
14.2916631553629));
#35379=CARTESIAN_POINT('Ctrl Pts',(5.07322036085286,-6.69861637153657E-5,
13.2083368446371));
#35380=CARTESIAN_POINT('Ctrl Pts',(5.07298878663719,0.497000397927876,13.2239264427309));
#35381=CARTESIAN_POINT('Ctrl Pts',(4.87730902789417,1.83782529464356,13.2659733375091));
#35382=CARTESIAN_POINT('Ctrl Pts',(3.71281646953824,3.76642207019282,13.3344775289718));
#35383=CARTESIAN_POINT('Ctrl Pts',(1.45915164597774,5.08348481077208,13.4138494190252));
#35384=CARTESIAN_POINT('Ctrl Pts',(-1.14995928876559,5.16222190355004,13.4932213090786));
#35385=CARTESIAN_POINT('Ctrl Pts',(-3.47894268615732,3.98345316700755,13.572593199132));
#35386=CARTESIAN_POINT('Ctrl Pts',(-4.96046334571011,1.83432405620607,13.6519650891854));
#35387=CARTESIAN_POINT('Ctrl Pts',(-5.23362611404733,-0.761642334479749,
13.7313369792388));
#35388=CARTESIAN_POINT('Ctrl Pts',(-4.23188914543755,-3.17207433835303,
13.8107088692922));
#35389=CARTESIAN_POINT('Ctrl Pts',(-2.19927334812693,-4.80979605467098,
13.8900807593456));
#35390=CARTESIAN_POINT('Ctrl Pts',(0.369080568778457,-5.27586209837409,
13.9694526493991));
#35391=CARTESIAN_POINT('Ctrl Pts',(2.84752727607539,-4.45673981283591,14.0488245394524));
#35392=CARTESIAN_POINT('Ctrl Pts',(4.63232264181505,-2.55196557371717,14.1281964295059));
#35393=CARTESIAN_POINT('Ctrl Pts',(5.07202231626624,-0.859526521495883,
14.1813671979007));
#35394=CARTESIAN_POINT('Ctrl Pts',(5.07403413732223,-0.00817292128436273,
14.2080806696111));
#35395=CARTESIAN_POINT('Ctrl Pts',(5.07403332299931,-8.66482790325162E-6,
14.2083368446371));
#35396=CARTESIAN_POINT('Origin',(0.,0.,-2.20833684463713));
#35397=CARTESIAN_POINT('',(5.07371259150425,0.000124614973235349,12.2083368446371));
#35398=CARTESIAN_POINT('',(5.07393295843892,7.85666071205126E-5,12.2916631553629));
#35399=CARTESIAN_POINT('',(5.0736,-1.85409460923845E-12,-2.20833684463713));
#35400=CARTESIAN_POINT('Ctrl Pts',(5.07393295843892,7.85666071204203E-5,
12.2916631553629));
#35401=CARTESIAN_POINT('Ctrl Pts',(5.07399255467328,0.080259357669063,12.2941788940293));
#35402=CARTESIAN_POINT('Ctrl Pts',(5.0525559141232,1.00364648464526,12.3231519293802));
#35403=CARTESIAN_POINT('Ctrl Pts',(4.51946174941847,2.74689039512926,12.3785822614155));
#35404=CARTESIAN_POINT('Ctrl Pts',(2.6551818185972,4.57394259446934,12.4579541514689));
#35405=CARTESIAN_POINT('Ctrl Pts',(0.144105473910954,5.28679250204684,12.5373260415223));
#35406=CARTESIAN_POINT('Ctrl Pts',(-2.40207464524796,4.7117914582425,12.6166979315757));
#35407=CARTESIAN_POINT('Ctrl Pts',(-4.36311469772651,2.98900844458373,12.6960698216291));
#35408=CARTESIAN_POINT('Ctrl Pts',(-5.26130966742946,0.538109589882336,
12.7754417116825));
#35409=CARTESIAN_POINT('Ctrl Pts',(-4.87786124785798,-2.043871569829,12.854813601736));
#35410=CARTESIAN_POINT('Ctrl Pts',(-3.30617662527107,-4.12797013916298,
12.9341854917893));
#35411=CARTESIAN_POINT('Ctrl Pts',(-0.929114694865931,-5.20650431970379,
13.0135573818428));
#35412=CARTESIAN_POINT('Ctrl Pts',(1.67427751864803,-5.01674557236658,13.0929292718962));
#35413=CARTESIAN_POINT('Ctrl Pts',(3.86981943456978,-3.60491870797887,13.1723011619496));
#35414=CARTESIAN_POINT('Ctrl Pts',(4.91547184132152,-1.69367935817457,13.2385457897718));
#35415=CARTESIAN_POINT('Ctrl Pts',(5.07315666403118,-0.425032354751582,
13.2783331209096));
#35416=CARTESIAN_POINT('Ctrl Pts',(5.07316545149283,3.01256212205392E-6,
13.2916631553629));
#35417=CARTESIAN_POINT('Ctrl Pts',(5.07371259150425,0.000124614973235296,
12.2083368446371));
#35418=CARTESIAN_POINT('Ctrl Pts',(5.07387461653381,0.158804080659856,12.2133149191661));
#35419=CARTESIAN_POINT('Ctrl Pts',(5.02779682862049,1.1607339041827,12.2447502903796));
#35420=CARTESIAN_POINT('Ctrl Pts',(4.38714636147788,2.95362288559007,12.3026429582776));
#35421=CARTESIAN_POINT('Ctrl Pts',(2.44010389315499,4.69220996311119,12.382014848331));
#35422=CARTESIAN_POINT('Ctrl Pts',(-0.101342482462103,5.28778507964898,
12.4613867383844));
#35423=CARTESIAN_POINT('Ctrl Pts',(-2.61810205366918,4.59526745509803,12.5407586284378));
#35424=CARTESIAN_POINT('Ctrl Pts',(-4.49709775967304,2.78335284993721,12.6201305184912));
#35425=CARTESIAN_POINT('Ctrl Pts',(-5.28061040557763,0.293419651378745,
12.6995024085446));
#35426=CARTESIAN_POINT('Ctrl Pts',(-4.7777780451164,-2.26798992478223,12.778874298598));
#35427=CARTESIAN_POINT('Ctrl Pts',(-3.11108952829712,-4.27692217537683,
12.8582461886514));
#35428=CARTESIAN_POINT('Ctrl Pts',(-0.686546488664521,-5.24400565085626,
12.9376180787048));
#35429=CARTESIAN_POINT('Ctrl Pts',(1.90523775596186,-4.93366095719673,13.0169899687582));
#35430=CARTESIAN_POINT('Ctrl Pts',(4.03291030040817,-3.42148737483739,13.0963618588116));
#35431=CARTESIAN_POINT('Ctrl Pts',(4.95323103438167,-1.53655914035534,13.1601441507712));
#35432=CARTESIAN_POINT('Ctrl Pts',(5.07338179405736,-0.346578710011678,
13.1974691460464));
#35433=CARTESIAN_POINT('Ctrl Pts',(5.07322036085286,-6.69861637153657E-5,
13.2083368446371));
#35434=CARTESIAN_POINT('Origin',(0.,0.,-2.20833684463713));
#35435=CARTESIAN_POINT('',(5.0736465461671,-0.000129729951178492,11.2083368446371));
#35436=CARTESIAN_POINT('',(5.07340926806867,-0.000121118768615341,11.2916631553629));
#35437=CARTESIAN_POINT('',(5.0736,-1.85409460923845E-12,-2.20833684463713));
#35438=CARTESIAN_POINT('Ctrl Pts',(5.07340926806867,-0.000121118768615022,
11.2916631553629));
#35439=CARTESIAN_POINT('Ctrl Pts',(5.07289012258619,0.585265031435054,11.310024667149));
#35440=CARTESIAN_POINT('Ctrl Pts',(4.82580215794652,2.01456720880964,11.3548434756196));
#35441=CARTESIAN_POINT('Ctrl Pts',(3.51104609249152,3.95518604919035,11.4261195807747));
#35442=CARTESIAN_POINT('Ctrl Pts',(1.19167245960881,5.152752477688,11.5054914708281));
#35443=CARTESIAN_POINT('Ctrl Pts',(-1.41798994671238,5.09511980804502,11.5848633608815));
#35444=CARTESIAN_POINT('Ctrl Pts',(-3.68223314068194,3.79632723101863,11.6642352509349));
#35445=CARTESIAN_POINT('Ctrl Pts',(-5.04949249206616,1.57275774354392,11.7436071409883));
#35446=CARTESIAN_POINT('Ctrl Pts',(-5.18670664924514,-1.03393204901786,
11.8229790310417));
#35447=CARTESIAN_POINT('Ctrl Pts',(-4.06045054724843,-3.38875828300867,
11.9023509210951));
#35448=CARTESIAN_POINT('Ctrl Pts',(-1.94507767959685,-4.91809050014781,
11.9817228111485));
#35449=CARTESIAN_POINT('Ctrl Pts',(0.644111805448097,-5.24938675745961,
12.0610947012019));
#35450=CARTESIAN_POINT('Ctrl Pts',(3.0763970804032,-4.30194401997477,12.1404665912553));
#35451=CARTESIAN_POINT('Ctrl Pts',(4.70593891054333,-2.36980219715329,12.2173227426423));
#35452=CARTESIAN_POINT('Ctrl Pts',(5.07336579829568,-0.762978855367823,
12.2677215973449));
#35453=CARTESIAN_POINT('Ctrl Pts',(5.07393295843892,7.85666071204203E-5,
12.2916631553629));
#35454=CARTESIAN_POINT('Ctrl Pts',(5.0736465461671,-0.000129729951178388,
11.2083368446371));
#35455=CARTESIAN_POINT('Ctrl Pts',(5.07296127147132,0.663669285094766,11.2291606922858));
#35456=CARTESIAN_POINT('Ctrl Pts',(4.77561643393883,2.17143981582611,11.276441836619));
#35457=CARTESIAN_POINT('Ctrl Pts',(3.32375507563458,4.11382954733217,11.3501802776367));
#35458=CARTESIAN_POINT('Ctrl Pts',(0.951315435152466,5.20249366075065,11.4295521676901));
#35459=CARTESIAN_POINT('Ctrl Pts',(-1.6528625396318,5.02384183393465,11.5089240577436));
#35460=CARTESIAN_POINT('Ctrl Pts',(-3.85440685831092,3.62139325645746,11.5882959477969));
#35461=CARTESIAN_POINT('Ctrl Pts',(-5.11702619789041,1.33678129752526,11.6676678378503));
#35462=CARTESIAN_POINT('Ctrl Pts',(-5.13314928200913,-1.27346762656892,
11.7470397279037));
#35463=CARTESIAN_POINT('Ctrl Pts',(-3.89884856306365,-3.57350265560368,
11.8264116179572));
#35464=CARTESIAN_POINT('Ctrl Pts',(-1.71479696411077,-5.00304034754732,
11.9057835080105));
#35465=CARTESIAN_POINT('Ctrl Pts',(0.886975379660772,-5.21384848487043,
11.985155398064));
#35466=CARTESIAN_POINT('Ctrl Pts',(3.27268248423369,-4.15457467193696,12.0645272881174));
#35467=CARTESIAN_POINT('Ctrl Pts',(4.76154396611873,-2.21316538967253,12.1389211036417));
#35468=CARTESIAN_POINT('Ctrl Pts',(5.0730134915642,-0.684540002865494,12.1868576224816));
#35469=CARTESIAN_POINT('Ctrl Pts',(5.07371259150425,0.000124614973235296,
12.2083368446371));
#35470=CARTESIAN_POINT('Origin',(0.,0.,-2.20833684463713));
#35471=CARTESIAN_POINT('',(5.07325419654647,8.30592867887003E-5,10.2083368446371));
#35472=CARTESIAN_POINT('',(5.07344000894767,0.000124864012350097,10.2916631553629));
#35473=CARTESIAN_POINT('',(5.0736,-1.85409460923845E-12,-2.20833684463713));
#35474=CARTESIAN_POINT('Ctrl Pts',(5.07344000894767,0.000124864012350061,
10.2916631553629));
#35475=CARTESIAN_POINT('Ctrl Pts',(5.07366802985413,0.247199120889535,10.2994131435843));
#35476=CARTESIAN_POINT('Ctrl Pts',(4.99543134296861,1.33760465491503,10.3336204284901));
#35477=CARTESIAN_POINT('Ctrl Pts',(4.22690463795744,3.1787133448809,10.3942850100804));
#35478=CARTESIAN_POINT('Ctrl Pts',(2.1917205673539,4.81324238969408,10.4736569001339));
#35479=CARTESIAN_POINT('Ctrl Pts',(-0.377361782165876,5.27527624230907,
10.5530287901872));
#35480=CARTESIAN_POINT('Ctrl Pts',(-2.85451963682615,4.45226447892349,10.6324006802407));
#35481=CARTESIAN_POINT('Ctrl Pts',(-4.63632282632763,2.54469094339242,10.711772570294));
#35482=CARTESIAN_POINT('Ctrl Pts',(-5.28872803766221,0.0172363266288179,
10.7911444603475));
#35483=CARTESIAN_POINT('Ctrl Pts',(-4.65281080542322,-2.5144170211496,10.8705163504009));
#35484=CARTESIAN_POINT('Ctrl Pts',(-2.88347915980519,-4.43356394814365,
10.9498882404543));
#35485=CARTESIAN_POINT('Ctrl Pts',(-0.411738373331464,-5.27270451089727,
11.0292601305077));
#35486=CARTESIAN_POINT('Ctrl Pts',(2.16030096951836,-4.82742592572977,11.1086320205611));
#35487=CARTESIAN_POINT('Ctrl Pts',(4.20609577793862,-3.20619707038057,11.1880039106145));
#35488=CARTESIAN_POINT('Ctrl Pts',(4.99105565025759,-1.3596709971465,11.2490142888818));
#35489=CARTESIAN_POINT('Ctrl Pts',(5.07363816480692,-0.25822406855438,11.2835673704646));
#35490=CARTESIAN_POINT('Ctrl Pts',(5.07340926806867,-0.000121118768615022,
11.2916631553629));
#35491=CARTESIAN_POINT('Ctrl Pts',(5.07325419654647,8.30592867889779E-5,
10.2083368446371));
#35492=CARTESIAN_POINT('Ctrl Pts',(5.07344390313192,0.32569224224827,10.2185491687211));
#35493=CARTESIAN_POINT('Ctrl Pts',(4.96261803044706,1.49473693663548,10.2552187894896));
#35494=CARTESIAN_POINT('Ctrl Pts',(4.07486890650351,3.37140693807807,10.3183457069425));
#35495=CARTESIAN_POINT('Ctrl Pts',(1.96603890048266,4.90974870936374,10.3977175969959));
#35496=CARTESIAN_POINT('Ctrl Pts',(-0.621713829942471,5.25208656259283,
10.4770894870493));
#35497=CARTESIAN_POINT('Ctrl Pts',(-3.05801844753381,4.31502775447074,10.5564613771027));
#35498=CARTESIAN_POINT('Ctrl Pts',(-4.74939654011498,2.32683773651149,10.6358332671561));
#35499=CARTESIAN_POINT('Ctrl Pts',(-5.28383214813503,-0.228164803694007,
10.7152051572095));
#35500=CARTESIAN_POINT('Ctrl Pts',(-4.53113794043347,-2.72758690275384,
10.7945770472629));
#35501=CARTESIAN_POINT('Ctrl Pts',(-2.67466855994604,-4.56257486971405,
10.8739489373163));
#35502=CARTESIAN_POINT('Ctrl Pts',(-0.166655838534166,-5.2861296975001,
10.9533208273697));
#35503=CARTESIAN_POINT('Ctrl Pts',(2.38195387625819,-4.72199503162473,11.0326927174231));
#35504=CARTESIAN_POINT('Ctrl Pts',(4.3503248991595,-3.00759282800428,11.1120646074765));
#35505=CARTESIAN_POINT('Ctrl Pts',(5.02057706818124,-1.20254945990408,11.1706126498812));
#35506=CARTESIAN_POINT('Ctrl Pts',(5.07383193265951,-0.17970643375256,11.2027033956014));
#35507=CARTESIAN_POINT('Ctrl Pts',(5.0736465461671,-0.000129729951178388,
11.2083368446371));
#35508=CARTESIAN_POINT('Origin',(0.,0.,-2.20833684463713));
#35509=CARTESIAN_POINT('',(5.07403156349013,-1.34850231131101E-5,9.20833684463708));
#35510=CARTESIAN_POINT('',(5.07390676572803,-8.73588085612467E-5,9.29166315536294));
#35511=CARTESIAN_POINT('',(5.0736,-1.85409460923845E-12,-2.20833684463713));
#35512=CARTESIAN_POINT('Ctrl Pts',(5.07390676572803,-8.73588085611478E-5,
9.29166315536294));
#35513=CARTESIAN_POINT('Ctrl Pts',(5.07329990983557,0.75196019632477,9.31525891670402));
#35514=CARTESIAN_POINT('Ctrl Pts',(4.71401054212216,2.34781906214645,9.36531197472956));
#35515=CARTESIAN_POINT('Ctrl Pts',(3.10437209115777,4.28180047024037,9.44182232943961));
#35516=CARTESIAN_POINT('Ctrl Pts',(0.67831398067512,5.24507688131743,9.52119421949299));
#35517=CARTESIAN_POINT('Ctrl Pts',(-1.91297991407746,4.93066417388633,9.6005661095464));
#35518=CARTESIAN_POINT('Ctrl Pts',(-4.03827613607002,3.41515258753654,9.6799379995998));
#35519=CARTESIAN_POINT('Ctrl Pts',(-5.1798572298885,1.06771739017486,9.75930988965322));
#35520=CARTESIAN_POINT('Ctrl Pts',(-5.05963656792565,-1.53981140008104,
9.8386817797066));
#35521=CARTESIAN_POINT('Ctrl Pts',(-3.70689963733171,-3.77224554159189,
9.91805366976003));
#35522=CARTESIAN_POINT('Ctrl Pts',(-1.45117016016697,-5.08576901889487,
9.99742555981341));
#35523=CARTESIAN_POINT('Ctrl Pts',(1.1580611559038,-5.16041042035386,10.0767974498668));
#35524=CARTESIAN_POINT('Ctrl Pts',(3.48519133772131,-3.97798726578937,10.1561693399202));
#35525=CARTESIAN_POINT('Ctrl Pts',(4.81900834166099,-2.03660616436304,10.2277912417523));
#35526=CARTESIAN_POINT('Ctrl Pts',(5.07288960070042,-0.596275311661321,
10.2729558468998));
#35527=CARTESIAN_POINT('Ctrl Pts',(5.07344000894767,0.000124864012350061,
10.2916631553629));
#35528=CARTESIAN_POINT('Ctrl Pts',(5.07403156349013,-1.34850231132098E-5,
9.20833684463708));
#35529=CARTESIAN_POINT('Ctrl Pts',(5.07390455498411,0.830454679150979,9.2343949418408));
#35530=CARTESIAN_POINT('Ctrl Pts',(4.65463656321598,2.50423700786744,9.28691033572898));
#35531=CARTESIAN_POINT('Ctrl Pts',(2.90236501609723,4.42122366100663,9.36588302630163));
#35532=CARTESIAN_POINT('Ctrl Pts',(0.434226208411351,5.27090020273944,9.44525491635504));
#35533=CARTESIAN_POINT('Ctrl Pts',(-2.13968914250016,4.83659712202464,9.52462680640844));
#35534=CARTESIAN_POINT('Ctrl Pts',(-4.1923809544202,3.22410968801074,9.60399869646184));
#35535=CARTESIAN_POINT('Ctrl Pts',(-5.22381804552131,0.826236270443201,
9.68337058651526));
#35536=CARTESIAN_POINT('Ctrl Pts',(-4.98274462345855,-1.77290647376134,
9.76274247656865));
#35537=CARTESIAN_POINT('Ctrl Pts',(-3.52788564023945,-3.94017312521954,
9.84211436662205));
#35538=CARTESIAN_POINT('Ctrl Pts',(-1.21364152390043,-5.14762232479954,
9.92148625667546));
#35539=CARTESIAN_POINT('Ctrl Pts',(1.39624298131078,-5.10112212012714,10.0008581467289));
#35540=CARTESIAN_POINT('Ctrl Pts',(3.66600578680612,-3.81199985813406,10.0802300367823));
#35541=CARTESIAN_POINT('Ctrl Pts',(4.86560152926764,-1.87962374426628,10.1493896027517));
#35542=CARTESIAN_POINT('Ctrl Pts',(5.07295242603298,-0.517870759272535,
10.1920918720366));
#35543=CARTESIAN_POINT('Ctrl Pts',(5.07325419654647,8.30592867889779E-5,
10.2083368446371));
#35544=CARTESIAN_POINT('Origin',(0.,0.,-2.20833684463713));
#35545=CARTESIAN_POINT('',(5.07321399251666,-6.32753131005193E-5,8.20833684463707));
#35546=CARTESIAN_POINT('',(5.07316567838514,7.26391603613751E-6,8.29166315536292));
#35547=CARTESIAN_POINT('',(5.0736,-1.85409460923845E-12,-2.20833684463713));
#35548=CARTESIAN_POINT('Ctrl Pts',(5.07316594763625,7.25941288019782E-6,
8.29166315536292));
#35549=CARTESIAN_POINT('Ctrl Pts',(5.07318657601694,0.414016596607197,8.30464739313926));
#35550=CARTESIAN_POINT('Ctrl Pts',(4.92101378278626,1.67161602862595,8.34408892760008));
#35551=CARTESIAN_POINT('Ctrl Pts',(3.89323433265495,3.57961838445758,8.40998775874535));
#35552=CARTESIAN_POINT('Ctrl Pts',(1.70694143925982,5.00572594837628,8.48935964879875));
#35553=CARTESIAN_POINT('Ctrl Pts',(-0.895158610488236,5.21244975125697,
8.56873153885215));
#35554=CARTESIAN_POINT('Ctrl Pts',(-3.27920000412133,4.14943233229326,8.64810342890557));
#35555=CARTESIAN_POINT('Ctrl Pts',(-4.86443553513654,2.0756223817956,8.72747531895896));
#35556=CARTESIAN_POINT('Ctrl Pts',(-5.26470533703792,-0.503804586595236,
8.80684720901237));
#35557=CARTESIAN_POINT('Ctrl Pts',(-4.38250457206448,-2.96050587284403,
8.88621909906576));
#35558=CARTESIAN_POINT('Ctrl Pts',(-2.43273539384546,-4.69603448143659,
8.96559098911917));
#35559=CARTESIAN_POINT('Ctrl Pts',(0.109642741545844,-5.28761948484726,
9.04496287917257));
#35560=CARTESIAN_POINT('Ctrl Pts',(2.62531214778668,-4.59115208569632,9.12433476922599));
#35561=CARTESIAN_POINT('Ctrl Pts',(4.50146132585655,-2.77629020081255,9.20370665927937));
#35562=CARTESIAN_POINT('Ctrl Pts',(5.04930321710503,-1.02570491769659,9.25948278799171));
#35563=CARTESIAN_POINT('Ctrl Pts',(5.07398036113186,-0.0912906316256552,
9.28880162001956));
#35564=CARTESIAN_POINT('Ctrl Pts',(5.07390676572803,-8.73588085611478E-5,
9.29166315536294));
#35565=CARTESIAN_POINT('Ctrl Pts',(5.07321399251666,-6.32753131006233E-5,
8.20833684463707));
#35566=CARTESIAN_POINT('Ctrl Pts',(5.07299759473682,0.492445607247212,8.22378341827604));
#35567=CARTESIAN_POINT('Ctrl Pts',(4.87982559067105,1.82870276667211,8.26568728859948));
#35568=CARTESIAN_POINT('Ctrl Pts',(3.72295704063487,3.75639883677136,8.33404845560738));
#35569=CARTESIAN_POINT('Ctrl Pts',(1.47285113468463,5.07953254565499,8.41342034566079));
#35570=CARTESIAN_POINT('Ctrl Pts',(-1.1360380475741,5.16530336977162,8.49279223571419));
#35571=CARTESIAN_POINT('Ctrl Pts',(-3.46819087602133,3.99281772621695,8.57216412576759));
#35572=CARTESIAN_POINT('Ctrl Pts',(-4.95550008378004,1.84769052250801,8.651536015821));
#35573=CARTESIAN_POINT('Ctrl Pts',(-5.23566043994335,-0.74753000269027,
8.7309079058744));
#35574=CARTESIAN_POINT('Ctrl Pts',(-4.24042550187429,-3.16065387386283,
8.81027979592781));
#35575=CARTESIAN_POINT('Ctrl Pts',(-2.21223229757129,-4.8038494573511,8.88965168598121));
#35576=CARTESIAN_POINT('Ctrl Pts',(0.354855797726969,-5.27683794616905,
8.96902357603462));
#35577=CARTESIAN_POINT('Ctrl Pts',(2.83550180615889,-4.46440039138287,9.04839546608801));
#35578=CARTESIAN_POINT('Ctrl Pts',(4.6254258508873,-2.56444478303851,9.12776735614143));
#35579=CARTESIAN_POINT('Ctrl Pts',(5.0708816691802,-0.868647987514843,9.18108114899111));
#35580=CARTESIAN_POINT('Ctrl Pts',(5.07403350920893,-0.0127359204844534,
9.20793764515633));
#35581=CARTESIAN_POINT('Ctrl Pts',(5.07403156349013,-1.34850231132098E-5,
9.20833684463708));
#35582=CARTESIAN_POINT('Origin',(0.,0.,-2.20833684463713));
#35583=CARTESIAN_POINT('',(5.0737268532953,0.000123079057421927,7.20833684463709));
#35584=CARTESIAN_POINT('',(5.07394313380083,7.47405269748897E-5,7.29166315536293));
#35585=CARTESIAN_POINT('',(5.0736,-1.85409460923845E-12,-2.20833684463713));
#35586=CARTESIAN_POINT('Ctrl Pts',(5.07394313380082,7.47405269749084E-5,
7.29166315536293));
#35587=CARTESIAN_POINT('Ctrl Pts',(5.07399715749136,0.0756966636928046,
7.29403586957452));
#35588=CARTESIAN_POINT('Ctrl Pts',(5.05387993962774,0.994523136339973,7.32286588047058));
#35589=CARTESIAN_POINT('Ctrl Pts',(4.52685078861501,2.73469619609302,7.37815318805109));
#35590=CARTESIAN_POINT('Ctrl Pts',(2.66750326347436,4.56676775046241,7.45752507810451));
#35591=CARTESIAN_POINT('Ctrl Pts',(0.158357847769689,5.28638478918814,7.5368969681579));
#35592=CARTESIAN_POINT('Ctrl Pts',(-2.38936318913255,4.71825019448189,7.61626885821132));
#35593=CARTESIAN_POINT('Ctrl Pts',(-4.3550406419278,3.0007602960695,7.69564074826471));
#35594=CARTESIAN_POINT('Ctrl Pts',(-5.25983983406839,0.552291831604834,
7.77501263831812));
#35595=CARTESIAN_POINT('Ctrl Pts',(-4.88335368508791,-2.03071370056153,
7.85438452837152));
#35596=CARTESIAN_POINT('Ctrl Pts',(-3.31729338754006,-4.11904187017964,
7.93375641842492));
#35597=CARTESIAN_POINT('Ctrl Pts',(-0.943147763491834,-5.20398055756651,
8.01312830847834));
#35598=CARTESIAN_POINT('Ctrl Pts',(1.66074656812082,-5.02124109994579,8.09250019853171));
#35599=CARTESIAN_POINT('Ctrl Pts',(3.86008671173945,-3.61533842470695,8.17187208858515));
#35600=CARTESIAN_POINT('Ctrl Pts',(4.91315662948087,-1.70280471015196,8.23825974086219));
#35601=CARTESIAN_POINT('Ctrl Pts',(5.07314454265331,-0.429588399925582,
8.27819009645479));
#35602=CARTESIAN_POINT('Ctrl Pts',(5.07316594763625,7.25941288019782E-6,
8.29166315536292));
#35603=CARTESIAN_POINT('Ctrl Pts',(5.0737268532953,0.000123079057421736,
7.20833684463709));
#35604=CARTESIAN_POINT('Ctrl Pts',(5.07388334783635,0.154242294956097,7.2131718947113));
#35605=CARTESIAN_POINT('Ctrl Pts',(5.02933704432274,1.15160862859258,7.24446424146999));
#35606=CARTESIAN_POINT('Ctrl Pts',(4.39509322077433,2.9417846501764,7.30221388491313));
#35607=CARTESIAN_POINT('Ctrl Pts',(2.45274496186498,4.68561452739722,7.38158577496654));
#35608=CARTESIAN_POINT('Ctrl Pts',(-0.0870865406957981,5.28803907717593,
7.46095766501995));
#35609=CARTESIAN_POINT('Ctrl Pts',(-2.60570395470586,4.60230901263053,7.54032955507335));
#35610=CARTESIAN_POINT('Ctrl Pts',(-4.48957765297745,2.79546665964655,7.61970144512676));
#35611=CARTESIAN_POINT('Ctrl Pts',(-5.27980017249532,0.307654816033177,
7.69907333518014));
#35612=CARTESIAN_POINT('Ctrl Pts',(-4.78387505663278,-2.25510105978351,
7.77844522523357));
#35613=CARTESIAN_POINT('Ctrl Pts',(-3.12260856590233,-4.26851930901846,
7.85781711528695));
#35614=CARTESIAN_POINT('Ctrl Pts',(-0.70068154029489,-5.24213570278374,
7.93718900534038));
#35615=CARTESIAN_POINT('Ctrl Pts',(1.8919299575961,-4.93877944262147,8.01656089539376));
#35616=CARTESIAN_POINT('Ctrl Pts',(4.02367150553262,-3.43234744203947,8.09593278544719));
#35617=CARTESIAN_POINT('Ctrl Pts',(4.95114565728143,-1.54568603506211,8.15985810186161));
#35618=CARTESIAN_POINT('Ctrl Pts',(5.07336824653293,-0.351136531432447,
8.19732612159157));
#35619=CARTESIAN_POINT('Ctrl Pts',(5.07321399251666,-6.32753131006233E-5,
8.20833684463707));
#35620=CARTESIAN_POINT('Origin',(0.,0.,-2.20833684463713));
#35621=CARTESIAN_POINT('',(5.07363207848188,-0.00013042437206158,6.20833684463708));
#35622=CARTESIAN_POINT('',(5.07339692231655,-0.000119345805453296,6.29166315536293));
#35623=CARTESIAN_POINT('',(5.0736,-1.85409460923845E-12,-2.20833684463713));
#35624=CARTESIAN_POINT('Ctrl Pts',(5.07339692231655,-0.000119345805453183,
6.29166315536293));
#35625=CARTESIAN_POINT('Ctrl Pts',(5.07289122007049,0.580711075066297,6.30988164269423));
#35626=CARTESIAN_POINT('Ctrl Pts',(4.82858806615863,2.00545098816607,6.35455742671001));
#35627=CARTESIAN_POINT('Ctrl Pts',(3.52169629398765,3.94570609146495,6.42569050741027));
#35628=CARTESIAN_POINT('Ctrl Pts',(1.20555966211655,5.14952106980711,6.50506239746365));
#35629=CARTESIAN_POINT('Ctrl Pts',(-1.40424863498509,5.09892411381582,6.58443428751707));
#35630=CARTESIAN_POINT('Ctrl Pts',(-3.67198507285601,3.80624052997609,6.66380617757046));
#35631=CARTESIAN_POINT('Ctrl Pts',(-5.04523407478029,1.58636517800468,6.74317806762388));
#35632=CARTESIAN_POINT('Ctrl Pts',(-5.1894752235243,-1.01994521996889,6.82254995767727));
#35633=CARTESIAN_POINT('Ctrl Pts',(-4.06957169452636,-3.37779921996849,
6.90192184773068));
#35634=CARTESIAN_POINT('Ctrl Pts',(-1.95832950858598,-4.91282880661553,
6.98129373778407));
#35635=CARTESIAN_POINT('Ctrl Pts',(0.629957410957137,-5.25110417033315,
7.06066562783749));
#35636=CARTESIAN_POINT('Ctrl Pts',(3.06478809957816,-4.31022218127953,7.14003751789089));
#35637=CARTESIAN_POINT('Ctrl Pts',(4.70257511155161,-2.37889312808664,7.2170366937327));
#35638=CARTESIAN_POINT('Ctrl Pts',(5.07339475843234,-0.767536645770191,
7.26757857289005));
#35639=CARTESIAN_POINT('Ctrl Pts',(5.07394313380082,7.47405269749084E-5,
7.29166315536293));
#35640=CARTESIAN_POINT('Ctrl Pts',(5.07363207848188,-0.000130424372061667,
6.20833684463708));
#35641=CARTESIAN_POINT('Ctrl Pts',(5.07295192244443,0.659114832324929,6.22901766783102));
#35642=CARTESIAN_POINT('Ctrl Pts',(4.77864726944019,2.16233220285461,6.27615578770943));
#35643=CARTESIAN_POINT('Ctrl Pts',(3.33483365177601,4.10485393921541,6.34975120427228));
#35644=CARTESIAN_POINT('Ctrl Pts',(0.96533761058682,5.19991006123149,6.42912309432572));
#35645=CARTESIAN_POINT('Ctrl Pts',(-1.63931253580277,5.02827960213728,6.50849498437909));
#35646=CARTESIAN_POINT('Ctrl Pts',(-3.84462977702757,3.63177136187054,6.58786687443252));
#35647=CARTESIAN_POINT('Ctrl Pts',(-5.11340371451209,1.35057165664169,6.6672387644859));
#35648=CARTESIAN_POINT('Ctrl Pts',(-5.13656382546863,-1.25962431470543,
6.74661065453933));
#35649=CARTESIAN_POINT('Ctrl Pts',(-3.90846835813217,-3.56297859112141,
6.82598254459271));
#35650=CARTESIAN_POINT('Ctrl Pts',(-1.72827865000271,-4.99839916925957,
6.90535443464612));
#35651=CARTESIAN_POINT('Ctrl Pts',(0.872915911787522,-5.21622077353501,
6.98472632469953));
#35652=CARTESIAN_POINT('Ctrl Pts',(3.26147008963291,-4.16338254328616,7.06409821475292));
#35653=CARTESIAN_POINT('Ctrl Pts',(4.7584325270959,-2.22226951355623,7.13863505473211));
#35654=CARTESIAN_POINT('Ctrl Pts',(5.07302701285767,-0.689094952273734,
7.18671459802684));
#35655=CARTESIAN_POINT('Ctrl Pts',(5.0737268532953,0.000123079057421736,
7.20833684463709));
#35656=CARTESIAN_POINT('Origin',(0.,0.,-2.20833684463713));
#35657=CARTESIAN_POINT('',(5.07326256235615,8.6340948239616E-5,5.20833684463708));
#35658=CARTESIAN_POINT('',(5.07345306532775,0.000126183674940957,5.29166315536293));
#35659=CARTESIAN_POINT('',(5.0736,-1.85409460923845E-12,-2.20833684463713));
#35660=CARTESIAN_POINT('Ctrl Pts',(5.07345306532775,0.000126183674940827,
5.29166315536293));
#35661=CARTESIAN_POINT('Ctrl Pts',(5.07368016839978,0.24263894378533,5.29927011912949));
#35662=CARTESIAN_POINT('Ctrl Pts',(4.99721910617995,1.32847790639321,5.33333437958052));
#35663=CARTESIAN_POINT('Ctrl Pts',(4.23545891089922,3.1673062942182,5.39385593671601));
#35664=CARTESIAN_POINT('Ctrl Pts',(2.20468883537238,4.80731614172549,5.47322782676942));
#35665=CARTESIAN_POINT('Ctrl Pts',(-0.363138560455233,5.27627441792221,
5.55259971682281));
#35666=CARTESIAN_POINT('Ctrl Pts',(-2.84250620674952,4.45994392474844,5.63197160687622));
#35667=CARTESIAN_POINT('Ctrl Pts',(-4.62944563286038,2.55718096342436,5.71134349692963));
#35668=CARTESIAN_POINT('Ctrl Pts',(-5.28866234991055,0.0314943796341776,
5.79071538698302));
#35669=CARTESIAN_POINT('Ctrl Pts',(-4.65957262477808,-2.50186416532327,
5.87008727703643));
#35670=CARTESIAN_POINT('Ctrl Pts',(-2.89542132203872,-4.42577413739037,
5.94945916708984));
#35671=CARTESIAN_POINT('Ctrl Pts',(-0.425951794157121,-5.27157532587407,
6.02883105714324));
#35672=CARTESIAN_POINT('Ctrl Pts',(2.14727864795285,-4.8332324334089,6.10820294719664));
#35673=CARTESIAN_POINT('Ctrl Pts',(4.19743676434218,-3.21752481834385,6.18757483725004));
#35674=CARTESIAN_POINT('Ctrl Pts',(4.98922373212554,-1.36879789494917,6.24872823997214));
#35675=CARTESIAN_POINT('Ctrl Pts',(5.0736256122357,-0.262783913782733,6.28342434600977));
#35676=CARTESIAN_POINT('Ctrl Pts',(5.07339692231655,-0.000119345805453183,
6.29166315536293));
#35677=CARTESIAN_POINT('Ctrl Pts',(5.07326256235615,8.63409482398936E-5,
5.20833684463708));
#35678=CARTESIAN_POINT('Ctrl Pts',(5.07345742030602,0.321133824030879,5.21840614426627));
#35679=CARTESIAN_POINT('Ctrl Pts',(4.96462985132702,1.48560987617541,5.25493274057992));
#35680=CARTESIAN_POINT('Ctrl Pts',(4.08394322312664,3.36040906700182,5.31791663357805));
#35681=CARTESIAN_POINT('Ctrl Pts',(1.979268164295,4.90443053586431,5.39728852363145));
#35682=CARTESIAN_POINT('Ctrl Pts',(-0.607552238323124,5.25374358196311,
5.47666041368485));
#35683=CARTESIAN_POINT('Ctrl Pts',(-3.04637426047979,4.32325632045987,5.55603230373826));
#35684=CARTESIAN_POINT('Ctrl Pts',(-4.74310625581864,2.33963338865815,5.63540419379165));
#35685=CARTESIAN_POINT('Ctrl Pts',(-5.28442806592769,-0.213919057930008,
5.71477608384507));
#35686=CARTESIAN_POINT('Ctrl Pts',(-4.53847489605989,-2.71536129550824,
5.79414797389846));
#35687=CARTESIAN_POINT('Ctrl Pts',(-2.68695928725567,-4.55534753185094,
5.87351986395187));
#35688=CARTESIAN_POINT('Ctrl Pts',(-0.180906343559476,-5.28566119252549,
5.95289175400528));
#35689=CARTESIAN_POINT('Ctrl Pts',(2.36921498499841,-4.72839948631341,6.03226364405867));
#35690=CARTESIAN_POINT('Ctrl Pts',(4.3422007873791,-3.01931013137013,6.1116355341121));
#35691=CARTESIAN_POINT('Ctrl Pts',(5.01896602830084,-1.21167525394927,6.17032660097155));
#35692=CARTESIAN_POINT('Ctrl Pts',(5.07382205657331,-0.184267811620037,
6.20256037114655));
#35693=CARTESIAN_POINT('Ctrl Pts',(5.07363207848188,-0.000130424372061667,
6.20833684463708));
#35694=CARTESIAN_POINT('Origin',(0.,0.,-2.20833684463713));
#35695=CARTESIAN_POINT('',(5.07402907570203,-1.82827833135855E-5,4.20833684463708));
#35696=CARTESIAN_POINT('',(5.07389532565035,-9.07960786141478E-5,4.29166315536292));
#35697=CARTESIAN_POINT('',(5.0736,-1.85409460923845E-12,-2.20833684463713));
#35698=CARTESIAN_POINT('Ctrl Pts',(5.07389532565035,-9.07960786142303E-5,
4.29166315536292));
#35699=CARTESIAN_POINT('Ctrl Pts',(5.07327433146367,0.747403143972462,4.3151158922492));
#35700=CARTESIAN_POINT('Ctrl Pts',(4.7173237838915,2.33872520323751,4.36502592581995));
#35701=CARTESIAN_POINT('Ctrl Pts',(3.11590430478523,4.27341569598967,4.44139325607517));
#35702=CARTESIAN_POINT('Ctrl Pts',(0.692451950200399,5.24322912373411,4.52076514612856));
#35703=CARTESIAN_POINT('Ctrl Pts',(-1.89968016673685,4.93580354262775,4.60013703618198));
#35704=CARTESIAN_POINT('Ctrl Pts',(-4.02905439992773,3.42602714375309,4.67950892623537));
#35705=CARTESIAN_POINT('Ctrl Pts',(-5.17695989945686,1.08167811604265,4.75888081628878));
#35706=CARTESIAN_POINT('Ctrl Pts',(-5.06376942648468,-1.5261653064819,4.83825270634218));
#35707=CARTESIAN_POINT('Ctrl Pts',(-3.71705592968434,-3.76223823845706,
4.91762459639559));
#35708=CARTESIAN_POINT('Ctrl Pts',(-1.46487583597662,-5.08183826311717,
4.996996486449));
#35709=CARTESIAN_POINT('Ctrl Pts',(1.14414476892732,-5.16351373534013,5.07636837650239));
#35710=CARTESIAN_POINT('Ctrl Pts',(3.47445424064207,-3.98736869087803,5.15574026655581));
#35711=CARTESIAN_POINT('Ctrl Pts',(4.81617424358115,-2.04572091909076,5.22750519284264));
#35712=CARTESIAN_POINT('Ctrl Pts',(5.07289029565433,-0.600829257314202,
5.27281282244502));
#35713=CARTESIAN_POINT('Ctrl Pts',(5.07345306532775,0.000126183674940827,
5.29166315536293));
#35714=CARTESIAN_POINT('Ctrl Pts',(5.07402907570203,-1.82827833134858E-5,
4.20833684463708));
#35715=CARTESIAN_POINT('Ctrl Pts',(5.07386028856637,0.825892891192897,4.23425191738599));
#35716=CARTESIAN_POINT('Ctrl Pts',(4.65820682968666,2.49515959185088,4.28662428681936));
#35717=CARTESIAN_POINT('Ctrl Pts',(2.91427384097298,4.41338297988409,4.36545395293721));
#35718=CARTESIAN_POINT('Ctrl Pts',(0.44843468320075,5.26971039832481,4.44482584299061));
#35719=CARTESIAN_POINT('Ctrl Pts',(-2.12664217080585,4.84234802803972,4.52419773304401));
#35720=CARTESIAN_POINT('Ctrl Pts',(-4.18367369924674,3.23540039647972,4.60356962309741));
#35721=CARTESIAN_POINT('Ctrl Pts',(-5.22157157495578,0.840316389774564,
4.68294151315082));
#35722=CARTESIAN_POINT('Ctrl Pts',(-4.98750617275825,-1.75946682947089,
4.76231340320422));
#35723=CARTESIAN_POINT('Ctrl Pts',(-3.53849530653447,-3.93064782357102,
4.84168529325762));
#35724=CARTESIAN_POINT('Ctrl Pts',(-1.22751481596538,-5.14433170819062,
4.92105718331103));
#35725=CARTESIAN_POINT('Ctrl Pts',(1.3824855667149,-5.10486777548008,5.00042907336443));
#35726=CARTESIAN_POINT('Ctrl Pts',(3.65571552542333,-3.82186935209575,5.07980096341784));
#35727=CARTESIAN_POINT('Ctrl Pts',(4.86300805809873,-1.88874478353847,5.14910355384205));
#35728=CARTESIAN_POINT('Ctrl Pts',(5.07294542694196,-0.522425194224716,
5.1919488475818));
#35729=CARTESIAN_POINT('Ctrl Pts',(5.07326256235615,8.63409482398936E-5,
5.20833684463708));
#35730=CARTESIAN_POINT('Origin',(0.,0.,-2.20833684463713));
#35731=CARTESIAN_POINT('',(5.0732079990561,-5.95000919163813E-5,3.20833684463708));
#35732=CARTESIAN_POINT('',(5.07316685382493,1.14989646604178E-5,3.29166315536292));
#35733=CARTESIAN_POINT('',(5.0736,-1.85409460923845E-12,-2.20833684463713));
#35734=CARTESIAN_POINT('Ctrl Pts',(5.07316685382493,1.14989646600797E-5,
3.29166315536292));
#35735=CARTESIAN_POINT('Ctrl Pts',(5.07319917633903,0.409460216043812,3.30450436868445));
#35736=CARTESIAN_POINT('Ctrl Pts',(4.923282999623,1.66249023374937,3.34380287869045));
#35737=CARTESIAN_POINT('Ctrl Pts',(3.90287063578958,3.56910943340232,3.40955868538091));
#35738=CARTESIAN_POINT('Ctrl Pts',(1.7204303939291,5.00110593838552,3.48893057543432));
#35739=CARTESIAN_POINT('Ctrl Pts',(-0.881102883784432,5.21484410653825,
3.56830246548772));
#35740=CARTESIAN_POINT('Ctrl Pts',(-3.26800144929621,4.15825779319991,3.64767435554113));
#35741=CARTESIAN_POINT('Ctrl Pts',(-4.85882209535798,2.08872908558557,3.72704624559453));
#35742=CARTESIAN_POINT('Ctrl Pts',(-5.2660444338108,-0.489609403954008,
3.80641813564793));
#35743=CARTESIAN_POINT('Ctrl Pts',(-4.39047000437897,-2.94868012642242,
3.88579002570134));
#35744=CARTESIAN_POINT('Ctrl Pts',(-2.44538680002092,-4.68945889688708,
3.96516191575474));
#35745=CARTESIAN_POINT('Ctrl Pts',(0.0953872160503347,-5.28789586001125,
4.04453380580815));
#35746=CARTESIAN_POINT('Ctrl Pts',(2.61292511742776,-4.59821309619564,4.12390569586154));
#35747=CARTESIAN_POINT('Ctrl Pts',(4.49396024381142,-2.78841580011883,4.20327758591496));
#35748=CARTESIAN_POINT('Ctrl Pts',(5.04793652990732,-1.03482867897542,4.25919673908208));
#35749=CARTESIAN_POINT('Ctrl Pts',(5.07397488200138,-0.0958531905725829,
4.28865859556473));
#35750=CARTESIAN_POINT('Ctrl Pts',(5.07389532565035,-9.07960786142303E-5,
4.29166315536292));
#35751=CARTESIAN_POINT('Ctrl Pts',(5.0732079990561,-5.95000919163813E-5,
3.20833684463708));
#35752=CARTESIAN_POINT('Ctrl Pts',(5.07300669336618,0.487890744857983,3.22364039382123));
#35753=CARTESIAN_POINT('Ctrl Pts',(4.88232843229471,1.81957999791209,3.26540123968986));
#35754=CARTESIAN_POINT('Ctrl Pts',(3.73307055280206,3.74634830136122,3.33361938224296));
#35755=CARTESIAN_POINT('Ctrl Pts',(1.48653991852054,5.07554336184363,3.41299127229636));
#35756=CARTESIAN_POINT('Ctrl Pts',(-1.12210854951228,5.16834729390561,3.49236316234976));
#35757=CARTESIAN_POINT('Ctrl Pts',(-3.45741385862906,4.00215326511488,3.57173505240317));
#35758=CARTESIAN_POINT('Ctrl Pts',(-4.95050080463958,1.86104355955814,3.65110694245657));
#35759=CARTESIAN_POINT('Ctrl Pts',(-5.23765671238755,-0.733412237756895,
3.73047883250997));
#35760=CARTESIAN_POINT('Ctrl Pts',(-4.24893103835441,-3.14921043733482,
3.80985072256337));
#35761=CARTESIAN_POINT('Ctrl Pts',(-2.22517516822744,-4.79786794503704,
3.88922261261678));
#35762=CARTESIAN_POINT('Ctrl Pts',(0.340628447538026,-5.2777754412288,3.96859450267018));
#35763=CARTESIAN_POINT('Ctrl Pts',(2.82345572745151,-4.472028522095,4.04796639272359));
#35764=CARTESIAN_POINT('Ctrl Pts',(4.61849544177105,-2.57690535364612,4.12733828277699));
#35765=CARTESIAN_POINT('Ctrl Pts',(5.06972869559084,-0.877769583505955,
4.18079510008149));
#35766=CARTESIAN_POINT('Ctrl Pts',(5.07403260725396,-0.0172989136932101,
4.20779462070152));
#35767=CARTESIAN_POINT('Ctrl Pts',(5.07402907570203,-1.82827833134858E-5,
4.20833684463708));
#35768=CARTESIAN_POINT('Origin',(0.,0.,-2.20833684463713));
#35769=CARTESIAN_POINT('',(5.07374102492394,0.00012139426775859,2.20833684463708));
#35770=CARTESIAN_POINT('',(5.07395289332891,7.08096438841769E-5,2.29166315536292));
#35771=CARTESIAN_POINT('',(5.0736,-1.85409460923845E-12,-2.20833684463713));
#35772=CARTESIAN_POINT('Ctrl Pts',(5.07395289332891,7.08096438841854E-5,
2.29166315536292));
#35773=CARTESIAN_POINT('Ctrl Pts',(5.07400149993288,0.0711339346777274,
2.2938928451197));
#35774=CARTESIAN_POINT('Ctrl Pts',(5.05519150559033,0.985399910949532,2.32257983156095));
#35775=CARTESIAN_POINT('Ctrl Pts',(4.53420692607935,2.72248212093367,2.37772411468667));
#35776=CARTESIAN_POINT('Ctrl Pts',(2.67980532059554,4.5595597146017,2.45709600474007));
#35777=CARTESIAN_POINT('Ctrl Pts',(0.172609070663326,5.28593865420646,2.53646789479348));
#35778=CARTESIAN_POINT('Ctrl Pts',(-2.37663436681889,4.72467463787357,2.61583978484688));
#35779=CARTESIAN_POINT('Ctrl Pts',(-4.34693493313492,3.01249033764445,2.69521167490029));
#35780=CARTESIAN_POINT('Ctrl Pts',(-5.25833177151656,0.56647005919948,2.77458356495369));
#35781=CARTESIAN_POINT('Ctrl Pts',(-4.88881062947673,-2.01754107180632,
2.85395545500709));
#35782=CARTESIAN_POINT('Ctrl Pts',(-3.32838603929513,-4.11008366347149,
2.93332734506049));
#35783=CARTESIAN_POINT('Ctrl Pts',(-0.957173977198773,-5.20141897223089,
3.0126992351139));
#35784=CARTESIAN_POINT('Ctrl Pts',(1.64720354707453,-5.02570013250045,3.0920711251673));
#35785=CARTESIAN_POINT('Ctrl Pts',(3.85032593330369,-3.62573186469146,3.1714430152207));
#35786=CARTESIAN_POINT('Ctrl Pts',(4.91082792455161,-1.71192991859137,3.23797369195258));
#35787=CARTESIAN_POINT('Ctrl Pts',(5.07313258089171,-0.434144349474542,
3.27804707199999));
#35788=CARTESIAN_POINT('Ctrl Pts',(5.07316685382493,1.14989646600797E-5,
3.29166315536292));
#35789=CARTESIAN_POINT('Ctrl Pts',(5.07374102492394,0.000121394267758555,
2.20833684463708));
#35790=CARTESIAN_POINT('Ctrl Pts',(5.07389186228029,0.149680441629337,2.21302887025649));
#35791=CARTESIAN_POINT('Ctrl Pts',(5.03086461164817,1.14248345247706,2.24417819256036));
#35792=CARTESIAN_POINT('Ctrl Pts',(4.40300813596794,2.92992503348825,2.3017848115487));
#35793=CARTESIAN_POINT('Ctrl Pts',(2.46536820371062,4.67898503603904,2.38115670160211));
#35794=CARTESIAN_POINT('Ctrl Pts',(-0.0728299659737919,5.28825464055465,
2.46052859165552));
#35795=CARTESIAN_POINT('Ctrl Pts',(-2.59328691715172,4.60931711999155,2.53990048170891));
#35796=CARTESIAN_POINT('Ctrl Pts',(-4.4820249154556,2.80756015154502,2.61927237176233));
#35797=CARTESIAN_POINT('Ctrl Pts',(-5.27895156514789,0.321887744613165,
2.69864426181572));
#35798=CARTESIAN_POINT('Ctrl Pts',(-4.7899372983315,-2.2421958044211,2.77801615186913));
#35799=CARTESIAN_POINT('Ctrl Pts',(-3.13410490798781,-4.26008541851404,
2.85738804192253));
#35800=CARTESIAN_POINT('Ctrl Pts',(-0.714811499281904,-5.2402276541964,
2.93675993197593));
#35801=CARTESIAN_POINT('Ctrl Pts',(1.8786084084407,-4.94386203236353,3.01613182202934));
#35802=CARTESIAN_POINT('Ctrl Pts',(4.01440346609632,-3.44318256249998,3.09550371208274));
#35803=CARTESIAN_POINT('Ctrl Pts',(4.9490470546202,-1.55481288423713,3.15957205295199));
#35804=CARTESIAN_POINT('Ctrl Pts',(5.07335471749433,-0.355694245953322,
3.19718309713677));
#35805=CARTESIAN_POINT('Ctrl Pts',(5.0732079990561,-5.95000919163813E-5,
3.20833684463708));
#35806=CARTESIAN_POINT('Origin',(0.,0.,-2.20833684463713));
#35807=CARTESIAN_POINT('',(5.07361762168166,-0.000130982038957922,1.20833684463708));
#35808=CARTESIAN_POINT('',(5.07338480805012,-0.000117445791330803,1.29166315536292));
#35809=CARTESIAN_POINT('',(5.0736,-1.85409460923845E-12,-2.20833684463713));
#35810=CARTESIAN_POINT('Ctrl Pts',(5.07338480805012,-0.000117445791331001,
1.29166315536292));
#35811=CARTESIAN_POINT('Ctrl Pts',(5.07289281667254,0.576157106237108,1.30973861823942));
#35812=CARTESIAN_POINT('Ctrl Pts',(4.83135991405541,1.99633436079896,1.35427137780039));
#35813=CARTESIAN_POINT('Ctrl Pts',(3.53232089954478,3.93619745533352,1.42526143404583));
#35814=CARTESIAN_POINT('Ctrl Pts',(1.21943810235538,5.14625223481536,1.50463332409923));
#35815=CARTESIAN_POINT('Ctrl Pts',(-1.39049711694202,5.10269135980955,1.58400521415263));
#35816=CARTESIAN_POINT('Ctrl Pts',(-3.66171031660135,3.81612616476449,1.66337710420604));
#35817=CARTESIAN_POINT('Ctrl Pts',(-5.04093898807,1.59996108251987,1.74274899425944));
#35818=CARTESIAN_POINT('Ctrl Pts',(-5.19220608004013,-1.00595097780601,
1.82212088431284));
#35819=CARTESIAN_POINT('Ctrl Pts',(-4.07866326363067,-3.3668156066614,1.90149277436625));
#35820=CARTESIAN_POINT('Ctrl Pts',(-1.97156710418735,-4.90753140600723,
1.98086466441965));
#35821=CARTESIAN_POINT('Ctrl Pts',(0.61579843785608,-5.25278341751101,2.06023655447306));
#35822=CARTESIAN_POINT('Ctrl Pts',(3.0531568434793,-4.31846901533485,2.13960844452646));
#35823=CARTESIAN_POINT('Ctrl Pts',(4.69919647653223,-2.38798317189229,2.21675064482308));
#35824=CARTESIAN_POINT('Ctrl Pts',(5.07342473837308,-0.772094669942323,
2.26743554843524));
#35825=CARTESIAN_POINT('Ctrl Pts',(5.07395289332891,7.08096438841854E-5,
2.29166315536292));
#35826=CARTESIAN_POINT('Ctrl Pts',(5.07361762168166,-0.000130982038957766,
1.20833684463708));
#35827=CARTESIAN_POINT('Ctrl Pts',(5.07294327622754,0.654560436527497,1.2288746433762));
#35828=CARTESIAN_POINT('Ctrl Pts',(4.78166373276894,2.15322402421039,1.2758697387998));
#35829=CARTESIAN_POINT('Ctrl Pts',(3.34588798700519,4.09584848370755,1.34932213090786));
#35830=CARTESIAN_POINT('Ctrl Pts',(0.979352771366438,5.19728867487042,1.42869402096127));
#35831=CARTESIAN_POINT('Ctrl Pts',(-1.6257506180571,5.03268082057239,1.50806591101467));
#35832=CARTESIAN_POINT('Ctrl Pts',(-3.83482475204895,3.64212307300266,1.58743780106807));
#35833=CARTESIAN_POINT('Ctrl Pts',(-5.10974406648874,1.36435219862418,1.66680969112148));
#35834=CARTESIAN_POINT('Ctrl Pts',(-5.13994103560183,-1.2457718471981,1.74618158117488));
#35835=CARTESIAN_POINT('Ctrl Pts',(-3.91805974601548,-3.55242863073578,
1.82555347122828));
#35836=CARTESIAN_POINT('Ctrl Pts',(-1.74174777450957,-4.99372166181597,
1.90492536128169));
#35837=CARTESIAN_POINT('Ctrl Pts',(0.858850099431454,-5.21855515011689,
1.98429725133509));
#35838=CARTESIAN_POINT('Ctrl Pts',(3.25023399025869,-4.17216015459491,2.0636691413885));
#35839=CARTESIAN_POINT('Ctrl Pts',(4.75530658628425,-2.2313729735679,2.13834900582249));
#35840=CARTESIAN_POINT('Ctrl Pts',(5.0730413237258,-0.693650010686127,2.18657157357202));
#35841=CARTESIAN_POINT('Ctrl Pts',(5.07374102492394,0.000121394267758555,
2.20833684463708));
#35842=CARTESIAN_POINT('Origin',(0.,0.,-2.20833684463713));
#35843=CARTESIAN_POINT('',(5.07327550687406,0.000108476183186546,0.208336844637077));
#35844=CARTESIAN_POINT('',(5.07346622253939,0.000127574377019038,0.291663155362924));
#35845=CARTESIAN_POINT('',(5.0736,-1.85409460923845E-12,-2.20833684463713));
#35846=CARTESIAN_POINT('',(1.3130361863565,-4.90075024188322,0.));
#35847=CARTESIAN_POINT('Ctrl Pts',(1.3130361863565,-4.90075024188322,0.));
#35848=CARTESIAN_POINT('Ctrl Pts',(2.12771778283771,-4.68247622999897,0.0264572966844678));
#35849=CARTESIAN_POINT('Ctrl Pts',(3.64531650851188,-3.8320815322798,0.0793718900534037));
#35850=CARTESIAN_POINT('Ctrl Pts',(4.86042636846397,-1.89775322538081,0.148817504932429));
#35851=CARTESIAN_POINT('Ctrl Pts',(5.07294944175775,-0.526932428119567,
0.191805823126987));
#35852=CARTESIAN_POINT('Ctrl Pts',(5.07327550687406,0.000108476183186372,
0.208336844637077));
#35853=CARTESIAN_POINT('',(-1.31317395760259,-4.90115117757553,2.08166817117217E-16));
#35854=CARTESIAN_POINT('Origin',(0.,0.,0.));
#35855=CARTESIAN_POINT('Ctrl Pts',(-1.31317395760259,-4.90115117757553,
2.32154790183459E-16));
#35856=CARTESIAN_POINT('Ctrl Pts',(-0.533836595431888,-5.10962665469163,
0.025313101045988));
#35857=CARTESIAN_POINT('Ctrl Pts',(1.16384881260007,-5.14969078544564,0.0770834987764434));
#35858=CARTESIAN_POINT('Ctrl Pts',(3.46369715057722,-3.99673439595713,0.155311193191368));
#35859=CARTESIAN_POINT('Ctrl Pts',(4.8133239766203,-2.05483010796368,0.22721914393302));
#35860=CARTESIAN_POINT('Ctrl Pts',(5.0728909576883,-0.605381739016801,0.272669797990206));
#35861=CARTESIAN_POINT('Ctrl Pts',(5.07346622253938,0.000127574377019116,
0.291663155362924));
#35862=CARTESIAN_POINT('Origin',(4.45462538595717E-16,-1.65775395963113E-16,
40.));
#35863=CARTESIAN_POINT('Ctrl Pts',(3.43378788736169,2.9358415841302,40.));
#35864=CARTESIAN_POINT('Ctrl Pts',(3.52814292550769,2.83820823955091,40.));
#35865=CARTESIAN_POINT('Ctrl Pts',(3.61787392647867,2.73637499985595,40.));
#35866=CARTESIAN_POINT('Ctrl Pts',(3.7028436241849,2.63075402506017,40.));
#35867=CARTESIAN_POINT('Ctrl Pts',(3.78889648523297,2.52378663182211,40.));
#35868=CARTESIAN_POINT('Ctrl Pts',(3.87006637156126,2.41293377092847,40.));
#35869=CARTESIAN_POINT('Ctrl Pts',(3.94617716449749,2.2985820569619,40.));
#35870=CARTESIAN_POINT('Ctrl Pts',(3.98452054291682,2.24097352507873,40.));
#35871=CARTESIAN_POINT('Ctrl Pts',(4.02157936104048,2.18247639180456,40.));
#35872=CARTESIAN_POINT('Ctrl Pts',(4.0573273224032,2.12313686354418,40.));
#35873=CARTESIAN_POINT('Ctrl Pts',(4.07057108419318,2.10115299237913,40.));
#35874=CARTESIAN_POINT('Ctrl Pts',(4.08363549665298,2.07905229886435,40.));
#35875=CARTESIAN_POINT('Ctrl Pts',(4.09651028112638,2.05685278711327,40.));
#35876=CARTESIAN_POINT('Ctrl Pts',(4.16636767341313,1.93640028523473,40.));
#35877=CARTESIAN_POINT('Ctrl Pts',(4.23070798356748,1.81293936852798,40.));
#35878=CARTESIAN_POINT('Ctrl Pts',(4.28936081037521,1.68687424953695,40.));
#35879=CARTESIAN_POINT('Ctrl Pts',(4.34350578332916,1.57049806053275,40.));
#35880=CARTESIAN_POINT('Ctrl Pts',(4.39280381894615,1.45190174917925,40.));
#35881=CARTESIAN_POINT('Ctrl Pts',(4.4370895395389,1.33137973638483,40.));
#35882=CARTESIAN_POINT('Ctrl Pts',(4.45048806014006,1.29491613932226,40.));
#35883=CARTESIAN_POINT('Ctrl Pts',(4.46342755329992,1.25827614359673,40.));
#35884=CARTESIAN_POINT('Ctrl Pts',(4.47590283035858,1.22146759434429,40.));
#35885=CARTESIAN_POINT('Ctrl Pts',(4.48543045669819,1.19335614625929,40.));
#35886=CARTESIAN_POINT('Ctrl Pts',(4.49468731429383,1.16514638329788,40.));
#35887=CARTESIAN_POINT('Ctrl Pts',(4.50367097326761,1.13684175481395,40.));
#35888=CARTESIAN_POINT('Ctrl Pts',(4.50984234488601,1.11739774192287,40.));
#35889=CARTESIAN_POINT('Ctrl Pts',(4.51588427541961,1.09791040265649,40.));
#35890=CARTESIAN_POINT('Ctrl Pts',(4.52179265714445,1.0783924896528,40.));
#35891=CARTESIAN_POINT('Ctrl Pts',(4.53324480098953,1.04056115821829,40.));
#35892=CARTESIAN_POINT('Ctrl Pts',(4.54419899621228,1.00260320591424,40.));
#35893=CARTESIAN_POINT('Ctrl Pts',(4.5546518960517,0.964527761093808,40.));
#35894=CARTESIAN_POINT('Ctrl Pts',(4.59117593379611,0.831486307992675,40.));
#35895=CARTESIAN_POINT('Ctrl Pts',(4.62158314424656,0.697012525339414,40.));
#35896=CARTESIAN_POINT('Ctrl Pts',(4.64596931935994,0.561539349137144,40.));
#35897=CARTESIAN_POINT('Ctrl Pts',(4.67073918176772,0.42393466456182,40.));
#35898=CARTESIAN_POINT('Ctrl Pts',(4.68929722659476,0.28529820513645,40.));
#35899=CARTESIAN_POINT('Ctrl Pts',(4.70169535323682,0.146060437529888,40.));
#35900=CARTESIAN_POINT('Ctrl Pts',(4.71417778478848,0.00587587951314419,
40.));
#35901=CARTESIAN_POINT('Ctrl Pts',(4.7204163646451,-0.134918963378981,40.));
#35902=CARTESIAN_POINT('Ctrl Pts',(4.72041312729179,-0.275897046739804,
40.));
#35903=CARTESIAN_POINT('Ctrl Pts',(4.72041101510801,-0.367877004659711,
40.));
#35904=CARTESIAN_POINT('Ctrl Pts',(4.71775084452937,-0.459935190334389,
40.));
#35905=CARTESIAN_POINT('Ctrl Pts',(4.71242122767243,-0.55195336772424,40.));
#35906=CARTESIAN_POINT('Ctrl Pts',(4.71074982773409,-0.580810822236322,
40.));
#35907=CARTESIAN_POINT('Ctrl Pts',(4.70881582061262,-0.609664336690085,
40.));
#35908=CARTESIAN_POINT('Ctrl Pts',(4.70661866095158,-0.638510242454293,
40.));
#35909=CARTESIAN_POINT('Ctrl Pts',(4.70521659891363,-0.65691752988966,40.));
#35910=CARTESIAN_POINT('Ctrl Pts',(4.70370712995809,-0.675324500804579,
40.));
#35911=CARTESIAN_POINT('Ctrl Pts',(4.70209092940465,-0.693720810758238,
40.));
#35912=CARTESIAN_POINT('Ctrl Pts',(4.68953110086222,-0.836682337618008,
40.));
#35913=CARTESIAN_POINT('Ctrl Pts',(4.67055276432277,-0.978761795279802,
40.));
#35914=CARTESIAN_POINT('Ctrl Pts',(4.64522498551854,-1.11951304986637,40.));
#35915=CARTESIAN_POINT('Ctrl Pts',(4.63006091029742,-1.20378268237205,40.));
#35916=CARTESIAN_POINT('Ctrl Pts',(4.61261985737539,-1.28757653832611,40.));
#35917=CARTESIAN_POINT('Ctrl Pts',(4.59290787692688,-1.37080047994428,40.));
#35918=CARTESIAN_POINT('Ctrl Pts',(4.56017758990635,-1.5089876856012,40.));
#35919=CARTESIAN_POINT('Ctrl Pts',(4.52118921321033,-1.64560413309505,40.));
#35920=CARTESIAN_POINT('Ctrl Pts',(4.47619425969956,-1.78030079004358,40.));
#35921=CARTESIAN_POINT('Ctrl Pts',(4.43085717885509,-1.91602163758472,40.));
#35922=CARTESIAN_POINT('Ctrl Pts',(4.3794215892058,-2.04979410792511,40.));
#35923=CARTESIAN_POINT('Ctrl Pts',(4.32209322112883,-2.18124988516394,40.));
#35924=CARTESIAN_POINT('Ctrl Pts',(4.29589299313303,-2.24132784395735,40.));
#35925=CARTESIAN_POINT('Ctrl Pts',(4.26846127047772,-2.30092169976294,40.));
#35926=CARTESIAN_POINT('Ctrl Pts',(4.23981435864377,-2.35999488119432,40.));
#35927=CARTESIAN_POINT('Ctrl Pts',(4.22808815540088,-2.38417564230685,40.));
#35928=CARTESIAN_POINT('Ctrl Pts',(4.21615831686625,-2.40826914901153,40.));
#35929=CARTESIAN_POINT('Ctrl Pts',(4.20402586547368,-2.43227283763382,40.));
#35930=CARTESIAN_POINT('Ctrl Pts',(4.19226175293326,-2.45554777896271,40.));
#35931=CARTESIAN_POINT('Ctrl Pts',(4.18030467857245,-2.47874278381504,40.));
#35932=CARTESIAN_POINT('Ctrl Pts',(4.16817016036066,-2.50182817485463,40.));
#35933=CARTESIAN_POINT('Ctrl Pts',(4.10062993280007,-2.63032050861895,40.));
#35934=CARTESIAN_POINT('Ctrl Pts',(4.02752679248241,-2.75556160907446,40.));
#35935=CARTESIAN_POINT('Ctrl Pts',(3.94914189359867,-2.87720021634157,40.));
#35936=CARTESIAN_POINT('Ctrl Pts',(3.87013649228652,-2.99980172656921,40.));
#35937=CARTESIAN_POINT('Ctrl Pts',(3.78576510402317,-3.11874421706065,40.));
#35938=CARTESIAN_POINT('Ctrl Pts',(3.69626453833047,-3.23365468399741,40.));
#35939=CARTESIAN_POINT('Ctrl Pts',(3.6256051940776,-3.3243747613366,40.));
#35940=CARTESIAN_POINT('Ctrl Pts',(3.55174784325694,-3.41258159925288,40.));
#35941=CARTESIAN_POINT('Ctrl Pts',(3.4747885470066,-3.49808125449705,40.));
#35942=CARTESIAN_POINT('Ctrl Pts',(3.37754842452615,-3.60611234824477,40.));
#35943=CARTESIAN_POINT('Ctrl Pts',(3.27535698426899,-3.70982288325437,40.));
#35944=CARTESIAN_POINT('Ctrl Pts',(3.16857103825032,-3.80899091582305,40.));
#35945=CARTESIAN_POINT('Ctrl Pts',(3.13709749914945,-3.83821919039451,40.));
#35946=CARTESIAN_POINT('Ctrl Pts',(3.10522459675968,-3.86705262006651,40.));
#35947=CARTESIAN_POINT('Ctrl Pts',(3.07296088810501,-3.89548488187744,40.));
#35948=CARTESIAN_POINT('Ctrl Pts',(3.05413623645007,-3.91207402945752,40.));
#35949=CARTESIAN_POINT('Ctrl Pts',(3.03517853882814,-3.92852660249152,40.));
#35950=CARTESIAN_POINT('Ctrl Pts',(3.01608945850777,-3.94484129509693,40.));
#35951=CARTESIAN_POINT('Ctrl Pts',(3.00324987792049,-3.95581478396849,40.));
#35952=CARTESIAN_POINT('Ctrl Pts',(2.99035184084321,-3.96672500977969,40.));
#35953=CARTESIAN_POINT('Ctrl Pts',(2.97740348730282,-3.97756535219416,40.));
#35954=CARTESIAN_POINT('Ctrl Pts',(2.86172546572695,-4.07441082060052,40.));
#35955=CARTESIAN_POINT('Ctrl Pts',(2.74187291014631,-4.16582105105552,40.));
#35956=CARTESIAN_POINT('Ctrl Pts',(2.61830752500134,-4.25161650299712,40.));
#35957=CARTESIAN_POINT('Ctrl Pts',(2.49666368456262,-4.33607776416752,40.));
#35958=CARTESIAN_POINT('Ctrl Pts',(2.37142082394795,-4.41509790443455,40.));
#35959=CARTESIAN_POINT('Ctrl Pts',(2.24297630552737,-4.4884725438774,40.));
#35960=CARTESIAN_POINT('Ctrl Pts',(2.11148832986889,-4.56358577505025,40.));
#35961=CARTESIAN_POINT('Ctrl Pts',(1.97664462468232,-4.63278348201276,40.));
#35962=CARTESIAN_POINT('Ctrl Pts',(1.83883549494666,-4.69580305762063,40.));
#35963=CARTESIAN_POINT('Ctrl Pts',(1.701026365211,-4.7588226332285,40.));
#35964=CARTESIAN_POINT('Ctrl Pts',(1.56025109502399,-4.81566463443687,40.));
#35965=CARTESIAN_POINT('Ctrl Pts',(1.41687422066896,-4.86601447289837,40.));
#35966=CARTESIAN_POINT('Ctrl Pts',(1.38245545626202,-4.8781013539643,40.));
#35967=CARTESIAN_POINT('Ctrl Pts',(1.34788667776073,-4.88981384734562,40.));
#35968=CARTESIAN_POINT('Ctrl Pts',(1.31317395760249,-4.90115117757556,40.));
#35969=CARTESIAN_POINT('Ctrl Pts',(-1.31303618635638,-4.90075024188325,
40.));
#35970=CARTESIAN_POINT('Ctrl Pts',(-1.45437915259461,-4.85452838596849,
40.));
#35971=CARTESIAN_POINT('Ctrl Pts',(-1.59345673045457,-4.80203124199391,
40.));
#35972=CARTESIAN_POINT('Ctrl Pts',(-1.72991111250498,-4.74351762389719,
40.));
#35973=CARTESIAN_POINT('Ctrl Pts',(-1.86679415923463,-4.68482018816886,
40.));
#35974=CARTESIAN_POINT('Ctrl Pts',(-2.001038164382,-4.62006797676633,40.));
#35975=CARTESIAN_POINT('Ctrl Pts',(-2.1322557155067,-4.54947707893507,40.));
#35976=CARTESIAN_POINT('Ctrl Pts',(-2.19315308373731,-4.5167162183481,40.));
#35977=CARTESIAN_POINT('Ctrl Pts',(-2.25339817251141,-4.48269720490963,
40.));
#35978=CARTESIAN_POINT('Ctrl Pts',(-2.31294973629581,-4.44743875160342,
40.));
#35979=CARTESIAN_POINT('Ctrl Pts',(-2.33562884151057,-4.43401122558351,
40.));
#35980=CARTESIAN_POINT('Ctrl Pts',(-2.35820900730168,-4.42040290103079,
40.));
#35981=CARTESIAN_POINT('Ctrl Pts',(-2.38068262652232,-4.40661797963936,
40.));
#35982=CARTESIAN_POINT('Ctrl Pts',(-2.50650561756839,-4.32944037759069,
40.));
#35983=CARTESIAN_POINT('Ctrl Pts',(-2.62877991395688,-4.24686153480494,
40.));
#35984=CARTESIAN_POINT('Ctrl Pts',(-2.74713717330506,-4.15910670751388,
40.));
#35985=CARTESIAN_POINT('Ctrl Pts',(-2.86467013316358,-4.07196304898213,
40.));
#35986=CARTESIAN_POINT('Ctrl Pts',(-2.97834099898066,-3.97971476207056,
40.));
#35987=CARTESIAN_POINT('Ctrl Pts',(-3.08775357309594,-3.88254556003572,
40.));
#35988=CARTESIAN_POINT('Ctrl Pts',(-3.14513584653695,-3.8315844180802,40.));
#35989=CARTESIAN_POINT('Ctrl Pts',(-3.2013462077245,-3.77926917964798,40.));
#35990=CARTESIAN_POINT('Ctrl Pts',(-3.25632275100474,-3.72562292402786,
40.));
#35991=CARTESIAN_POINT('Ctrl Pts',(-3.27574922848208,-3.70666651617886,
40.));
#35992=CARTESIAN_POINT('Ctrl Pts',(-3.29502416873062,-3.6875411953518,40.));
#35993=CARTESIAN_POINT('Ctrl Pts',(-3.31412620910246,-3.66826697432299,
40.));
#35994=CARTESIAN_POINT('Ctrl Pts',(-3.34404060290358,-3.63808294021764,
40.));
#35995=CARTESIAN_POINT('Ctrl Pts',(-3.37353997543889,-3.60752519082335,
40.));
#35996=CARTESIAN_POINT('Ctrl Pts',(-3.40261591802411,-3.57659932769541,
40.));
#35997=CARTESIAN_POINT('Ctrl Pts',(-3.50164274205642,-3.47127204562902,
40.));
#35998=CARTESIAN_POINT('Ctrl Pts',(-3.59576101414824,-3.36167756876611,
40.));
#35999=CARTESIAN_POINT('Ctrl Pts',(-3.68480291336662,-3.24822038520781,
40.));
#36000=CARTESIAN_POINT('Ctrl Pts',(-3.77450749603108,-3.13391881043548,
40.));
#36001=CARTESIAN_POINT('Ctrl Pts',(-3.85906025603562,-3.01569612122462,
40.));
#36002=CARTESIAN_POINT('Ctrl Pts',(-3.93824649098464,-2.893935566612,40.));
#36003=CARTESIAN_POINT('Ctrl Pts',(-4.01670520549023,-2.7732936823433,40.));
#36004=CARTESIAN_POINT('Ctrl Pts',(-4.08989581732523,-2.64917791019356,
40.));
#36005=CARTESIAN_POINT('Ctrl Pts',(-4.15756259897637,-2.52194215997081,
40.));
#36006=CARTESIAN_POINT('Ctrl Pts',(-4.20177691057784,-2.43880474793609,
40.));
#36007=CARTESIAN_POINT('Ctrl Pts',(-4.24363187369716,-2.35433490941293,
40.));
#36008=CARTESIAN_POINT('Ctrl Pts',(-4.2830443332661,-2.26862918510464,40.));
#36009=CARTESIAN_POINT('Ctrl Pts',(-4.30136127527663,-2.22879744663171,
40.));
#36010=CARTESIAN_POINT('Ctrl Pts',(-4.31915051766851,-2.18869875186795,
40.));
#36011=CARTESIAN_POINT('Ctrl Pts',(-4.33640298127534,-2.14834275431588,
40.));
#36012=CARTESIAN_POINT('Ctrl Pts',(-4.3436590160159,-2.13136984384344,40.));
#36013=CARTESIAN_POINT('Ctrl Pts',(-4.35081962128211,-2.11435240712678,
40.));
#36014=CARTESIAN_POINT('Ctrl Pts',(-4.35787943356684,-2.09730289812436,
40.));
#36015=CARTESIAN_POINT('Ctrl Pts',(-4.41262610226673,-1.96508920982698,
40.));
#36016=CARTESIAN_POINT('Ctrl Pts',(-4.46139597719794,-1.83076168016892,
40.));
#36017=CARTESIAN_POINT('Ctrl Pts',(-4.50399603348697,-1.69468832090704,
40.));
#36018=CARTESIAN_POINT('Ctrl Pts',(-4.527154798591,-1.62071445235899,40.));
#36019=CARTESIAN_POINT('Ctrl Pts',(-4.54848933959424,-1.54622425456777,
40.));
#36020=CARTESIAN_POINT('Ctrl Pts',(-4.56796247846724,-1.47127487515815,
40.));
#36021=CARTESIAN_POINT('Ctrl Pts',(-4.60386684913915,-1.33308398988268,
40.));
#36022=CARTESIAN_POINT('Ctrl Pts',(-4.633446346586,-1.19333212031901,40.));
#36023=CARTESIAN_POINT('Ctrl Pts',(-4.65669710227076,-1.05245525970538,
40.));
#36024=CARTESIAN_POINT('Ctrl Pts',(-4.67988218362711,-0.911976321350021,
40.));
#36025=CARTESIAN_POINT('Ctrl Pts',(-4.6967741641367,-0.770377936579903,
40.));
#36026=CARTESIAN_POINT('Ctrl Pts',(-4.70731777033656,-0.628096038990404,
40.));
#36027=CARTESIAN_POINT('Ctrl Pts',(-4.71196239382317,-0.565418637090442,
40.));
#36028=CARTESIAN_POINT('Ctrl Pts',(-4.71537442348699,-0.502608716141042,
40.));
#36029=CARTESIAN_POINT('Ctrl Pts',(-4.71754599609844,-0.439704378705418,
40.));
#36030=CARTESIAN_POINT('Ctrl Pts',(-4.71847271903558,-0.412859827415833,
40.));
#36031=CARTESIAN_POINT('Ctrl Pts',(-4.71917350957111,-0.385998089715844,
40.));
#36032=CARTESIAN_POINT('Ctrl Pts',(-4.71964765055488,-0.359122168611144,
40.));
#36033=CARTESIAN_POINT('Ctrl Pts',(-4.72007766112019,-0.334747709487924,
40.));
#36034=CARTESIAN_POINT('Ctrl Pts',(-4.72032117948226,-0.310357499793734,
40.));
#36035=CARTESIAN_POINT('Ctrl Pts',(-4.72037779701569,-0.28598141917232,
40.));
#36036=CARTESIAN_POINT('Ctrl Pts',(-4.72070503729545,-0.145091575346323,
40.));
#36037=CARTESIAN_POINT('Ctrl Pts',(-4.71479792201471,-0.00450394063596596,
40.));
#36038=CARTESIAN_POINT('Ctrl Pts',(-4.7026779767235,0.135364936808135,40.));
#36039=CARTESIAN_POINT('Ctrl Pts',(-4.6906385436001,0.274304672555548,40.));
#36040=CARTESIAN_POINT('Ctrl Pts',(-4.67246842821977,0.412535934949348,
40.));
#36041=CARTESIAN_POINT('Ctrl Pts',(-4.64813815685378,0.549644620304502,
40.));
#36042=CARTESIAN_POINT('Ctrl Pts',(-4.62922788638654,0.656209906177027,
40.));
#36043=CARTESIAN_POINT('Ctrl Pts',(-4.60659531784607,0.762097046731738,
40.));
#36044=CARTESIAN_POINT('Ctrl Pts',(-4.58020591978812,0.867104757427845,
40.));
#36045=CARTESIAN_POINT('Ctrl Pts',(-4.54608550784896,1.00287543085781,40.));
#36046=CARTESIAN_POINT('Ctrl Pts',(-4.5056856677851,1.13717725960422,40.));
#36047=CARTESIAN_POINT('Ctrl Pts',(-4.45916773762384,1.26960241773677,40.));
#36048=CARTESIAN_POINT('Ctrl Pts',(-4.44595800567878,1.30720729043101,40.));
#36049=CARTESIAN_POINT('Ctrl Pts',(-4.43225465907289,1.34466063579127,40.));
#36050=CARTESIAN_POINT('Ctrl Pts',(-4.41806080497834,1.381952618119,40.));
#36051=CARTESIAN_POINT('Ctrl Pts',(-4.41034395548629,1.40222735202608,40.));
#36052=CARTESIAN_POINT('Ctrl Pts',(-4.40248211604979,1.42245438558641,40.));
#36053=CARTESIAN_POINT('Ctrl Pts',(-4.39447575604619,1.44263210700853,40.));
#36054=CARTESIAN_POINT('Ctrl Pts',(-4.38774337392406,1.45959913458491,40.));
#36055=CARTESIAN_POINT('Ctrl Pts',(-4.38091020364865,1.47652766568619,40.));
#36056=CARTESIAN_POINT('Ctrl Pts',(-4.37398035764513,1.49340802308437,40.));
#36057=CARTESIAN_POINT('Ctrl Pts',(-4.32139777601335,1.62149352028206,40.));
#36058=CARTESIAN_POINT('Ctrl Pts',(-4.26319329324451,1.74695839038908,40.));
#36059=CARTESIAN_POINT('Ctrl Pts',(-4.19959993118347,1.86944841739778,40.));
#36060=CARTESIAN_POINT('Ctrl Pts',(-4.13606105752427,1.99183349185173,40.));
#36061=CARTESIAN_POINT('Ctrl Pts',(-4.06714208355231,2.1112494937512,40.));
#36062=CARTESIAN_POINT('Ctrl Pts',(-3.99303011697524,2.22731770598438,40.));
#36063=CARTESIAN_POINT('Ctrl Pts',(-3.9202059518248,2.34136906700981,40.));
#36064=CARTESIAN_POINT('Ctrl Pts',(-3.84236718991447,2.45218850722107,40.));
#36065=CARTESIAN_POINT('Ctrl Pts',(-3.75965485123955,2.55938335127685,40.));
#36066=CARTESIAN_POINT('Ctrl Pts',(-3.67819754057762,2.66495168429094,40.));
#36067=CARTESIAN_POINT('Ctrl Pts',(-3.59201299654429,2.76700506575445,40.));
#36068=CARTESIAN_POINT('Ctrl Pts',(-3.50120707213067,2.86512829543056,40.));
#36069=CARTESIAN_POINT('Ctrl Pts',(-3.47910751146495,2.88900867857677,40.));
#36070=CARTESIAN_POINT('Ctrl Pts',(-3.45673410716774,2.91265607078183,40.));
#36071=CARTESIAN_POINT('Ctrl Pts',(-3.43409108914464,2.93606647242288,40.));
#36072=CARTESIAN_POINT('Origin',(0.,0.,-2.20833684463713));
#36073=CARTESIAN_POINT('Ctrl Pts',(5.07346622253938,0.000127574377019116,
0.291663155362924));
#36074=CARTESIAN_POINT('Ctrl Pts',(5.07369228799229,0.238078384188188,0.299127094674674));
#36075=CARTESIAN_POINT('Ctrl Pts',(4.99899491470862,1.31934885093053,0.333048330670892));
#36076=CARTESIAN_POINT('Ctrl Pts',(4.24398161873799,3.15587819282154,0.393426863351577));
#36077=CARTESIAN_POINT('Ctrl Pts',(2.21764149317933,4.80135391043019,0.472798753404982));
#36078=CARTESIAN_POINT('Ctrl Pts',(-0.348912918530393,5.27723479734493,
0.552170643458385));
#36079=CARTESIAN_POINT('Ctrl Pts',(-2.83047200092439,4.46759066254957,0.631542533511789));
#36080=CARTESIAN_POINT('Ctrl Pts',(-4.62253485344812,2.56965255248809,0.710914423565193));
#36081=CARTESIAN_POINT('Ctrl Pts',(-5.28855819093304,0.045752121671659,
0.790286313618596));
#36082=CARTESIAN_POINT('Ctrl Pts',(-4.66630059499956,-2.48929308216644,
0.869658203672));
#36083=CARTESIAN_POINT('Ctrl Pts',(-2.90734243084918,-4.4179521825598,0.949030093725403));
#36084=CARTESIAN_POINT('Ctrl Pts',(-0.440162123945536,-5.27040781417518,
1.02840198377881));
#36085=CARTESIAN_POINT('Ctrl Pts',(2.1342407222512,-4.83900381899044,1.10777387383221));
#36086=CARTESIAN_POINT('Ctrl Pts',(4.18874724188064,-3.228829177505,1.18714576388562));
#36087=CARTESIAN_POINT('Ctrl Pts',(4.9873788651986,-1.37792482956251,1.24844219106252));
#36088=CARTESIAN_POINT('Ctrl Pts',(5.07361295102991,-0.267343660459586,
1.28328132155495));
#36089=CARTESIAN_POINT('Ctrl Pts',(5.07338480805012,-0.000117445791331001,
1.29166315536292));
#36090=CARTESIAN_POINT('Ctrl Pts',(5.07327550687406,0.000108476183186372,
0.208336844637077));
#36091=CARTESIAN_POINT('Ctrl Pts',(5.07347129707779,0.316577306682802,0.218263119811455));
#36092=CARTESIAN_POINT('Ctrl Pts',(4.96661393653962,1.47641857544861,0.254646691670301));
#36093=CARTESIAN_POINT('Ctrl Pts',(4.09299916691648,3.34943642687043,0.317487560213614));
#36094=CARTESIAN_POINT('Ctrl Pts',(1.99247705733062,4.89905044646781,0.396859450267019));
#36095=CARTESIAN_POINT('Ctrl Pts',(-0.593383061700938,5.2553763257097,0.476231340320422));
#36096=CARTESIAN_POINT('Ctrl Pts',(-3.03470961035893,4.33144609848054,0.555603230373826));
#36097=CARTESIAN_POINT('Ctrl Pts',(-4.73678060915323,2.35241593705463,0.634975120427228));
#36098=CARTESIAN_POINT('Ctrl Pts',(-5.28498604656423,-0.199673823356779,
0.714347010480634));
#36099=CARTESIAN_POINT('Ctrl Pts',(-4.5457786161601,-2.703114858517,0.793718900534037));
#36100=CARTESIAN_POINT('Ctrl Pts',(-2.69923061743508,-4.5480876646044,0.87309079058744));
#36101=CARTESIAN_POINT('Ctrl Pts',(-0.195155463808127,-5.28515396379925,
0.952462680640845));
#36102=CARTESIAN_POINT('Ctrl Pts',(2.35645883694709,-4.73476973691702,1.03183457069425));
#36103=CARTESIAN_POINT('Ctrl Pts',(4.33404513553918,-3.03100540392648,1.11120646074765));
#36104=CARTESIAN_POINT('Ctrl Pts',(5.01734225874463,-1.22080114526538,1.17004055206193));
#36105=CARTESIAN_POINT('Ctrl Pts',(5.0738119846015,-0.188829126190742,1.20241734669174));
#36106=CARTESIAN_POINT('Ctrl Pts',(5.07361762168166,-0.000130982038957766,
1.20833684463708));
#36107=CARTESIAN_POINT('Ctrl Pts',(-3.43378788736187,2.93584158412999,-1.38777878078145E-15));
#36108=CARTESIAN_POINT('Ctrl Pts',(-3.92183073605352,2.36502208507736,0.0264572966844665));
#36109=CARTESIAN_POINT('Ctrl Pts',(-4.60729903172261,0.975909964327098,
0.0793718900534022));
#36110=CARTESIAN_POINT('Ctrl Pts',(-4.51258247789853,-1.34695556252418,
0.158743780106806));
#36111=CARTESIAN_POINT('Ctrl Pts',(-3.3188765366808,-3.34104229843846,0.23811567016021));
#36112=CARTESIAN_POINT('Ctrl Pts',(-1.31656588610641,-4.52159485055713,
0.317487560213613));
#36113=CARTESIAN_POINT('Ctrl Pts',(1.00638734295355,-4.60052063353559,0.396859450267017));
#36114=CARTESIAN_POINT('Ctrl Pts',(3.08422378627015,-3.55886290155616,0.476231340320421));
#36115=CARTESIAN_POINT('Ctrl Pts',(4.41073058968579,-1.65022475069956,0.555603230373823));
#36116=CARTESIAN_POINT('Ctrl Pts',(4.66280353786907,0.660378394082181,0.634975120427229));
#36117=CARTESIAN_POINT('Ctrl Pts',(3.77902238214553,2.81012864743368,0.71434701048063));
#36118=CARTESIAN_POINT('Ctrl Pts',(1.9746826426622,4.27533046137772,0.793718900534036));
#36119=CARTESIAN_POINT('Ctrl Pts',(-0.310686955552407,4.69907511544172,
0.873090790587439));
#36120=CARTESIAN_POINT('Ctrl Pts',(-2.52037308462949,3.97813341921581,0.952462680640842));
#36121=CARTESIAN_POINT('Ctrl Pts',(-4.11610234038262,2.28812831500376,1.03183457069425));
#36122=CARTESIAN_POINT('Ctrl Pts',(-4.70915794841686,0.0407396420060994,
1.11120646074765));
#36123=CARTESIAN_POINT('Ctrl Pts',(-4.15507322474362,-2.21657281259016,
1.19057835080105));
#36124=CARTESIAN_POINT('Ctrl Pts',(-2.58882179654858,-3.93393319787912,
1.26995024085446));
#36125=CARTESIAN_POINT('Ctrl Pts',(-0.391939142907391,-4.69299607822649,
1.34932213090786));
#36126=CARTESIAN_POINT('Ctrl Pts',(1.90041903637464,-4.30885554699701,1.42869402096126));
#36127=CARTESIAN_POINT('Ctrl Pts',(3.72983933538439,-2.87508731801348,1.50806591101467));
#36128=CARTESIAN_POINT('Ctrl Pts',(4.65067903319439,-0.740954194967835,
1.58743780106807));
#36129=CARTESIAN_POINT('Ctrl Pts',(4.43862360995218,1.57367373662795,1.66680969112148));
#36130=CARTESIAN_POINT('Ctrl Pts',(3.1453293014661,3.50495822568453,1.74618158117488));
#36131=CARTESIAN_POINT('Ctrl Pts',(1.08583973646247,4.58244265094549,1.82555347122828));
#36132=CARTESIAN_POINT('Ctrl Pts',(-1.2381579844814,4.54365418850119,1.90492536128169));
#36133=CARTESIAN_POINT('Ctrl Pts',(-3.26054316123182,3.39804162347539,1.98429725133509));
#36134=CARTESIAN_POINT('Ctrl Pts',(-4.48866724088482,1.42467364012815,2.0636691413885));
#36135=CARTESIAN_POINT('Ctrl Pts',(-4.62336191621359,-0.895741688344198,
2.1430410314419));
#36136=CARTESIAN_POINT('Ctrl Pts',(-3.63181586235956,-2.99795632430514,
2.2224129214953));
#36137=CARTESIAN_POINT('Ctrl Pts',(-1.75556750333933,-4.36987543548745,
2.30178481154871));
#36138=CARTESIAN_POINT('Ctrl Pts',(0.548333213620371,-4.67730256316232,
2.38115670160211));
#36139=CARTESIAN_POINT('Ctrl Pts',(2.71866117345249,-3.84534913947276,2.46052859165552));
#36140=CARTESIAN_POINT('Ctrl Pts',(4.22672928908848,-2.07667717694978,2.53990048170891));
#36141=CARTESIAN_POINT('Ctrl Pts',(4.7051755056078,0.19786874923449,2.61927237176232));
#36142=CARTESIAN_POINT('Ctrl Pts',(4.03745138369107,2.42421428607854,2.69864426181572));
#36143=CARTESIAN_POINT('Ctrl Pts',(2.38621304145389,4.06002658874208,2.77801615186912));
#36144=CARTESIAN_POINT('Ctrl Pts',(0.153698484111727,4.70682540110399,2.85738804192253));
#36145=CARTESIAN_POINT('Ctrl Pts',(-2.11625668375435,4.20705196413855,2.93675993197593));
#36146=CARTESIAN_POINT('Ctrl Pts',(-3.87069640771252,2.68244998086038,3.01613182202934));
#36147=CARTESIAN_POINT('Ctrl Pts',(-4.68224305439313,0.504409119747013,
3.09550371208274));
#36148=CARTESIAN_POINT('Ctrl Pts',(-4.35320565699276,-1.79650468644612,
3.17487560213615));
#36149=CARTESIAN_POINT('Ctrl Pts',(-2.96373699720624,-3.65979392751662,
3.25424749218954));
#36150=CARTESIAN_POINT('Ctrl Pts',(-0.852308565020845,-4.63156546866054,
3.33361938224295));
#36151=CARTESIAN_POINT('Ctrl Pts',(1.46674034705061,-4.47509791343502,3.41299127229636));
#36152=CARTESIAN_POINT('Ctrl Pts',(3.42849455715522,-3.22850641195795,3.49236316234976));
#36153=CARTESIAN_POINT('Ctrl Pts',(4.55507508198081,-1.19545789470566,3.57173505240317));
#36154=CARTESIAN_POINT('Ctrl Pts',(4.57204939932356,1.12880151959577,3.65110694245656));
#36155=CARTESIAN_POINT('Ctrl Pts',(3.47528260305076,3.17808738228345,3.73047883250997));
#36156=CARTESIAN_POINT('Ctrl Pts',(1.53194465708238,4.45319819322398,3.80985072256337));
#36157=CARTESIAN_POINT('Ctrl Pts',(-0.784571616449287,4.64351978128216,
3.88922261261678));
#36158=CARTESIAN_POINT('Ctrl Pts',(-2.90996798083373,3.70269022887672,3.96859450267018));
#36159=CARTESIAN_POINT('Ctrl Pts',(-4.32650258619195,1.85989353248269,4.04796639272359));
#36160=CARTESIAN_POINT('Ctrl Pts',(-4.68911073810485,-0.4359691116196,4.12733828277699));
#36161=CARTESIAN_POINT('Ctrl Pts',(-3.90946189338598,-2.62563064513263,
4.2067101728304));
#36162=CARTESIAN_POINT('Ctrl Pts',(-2.17747678488539,-4.17569436522619,
4.28608206288379));
#36163=CARTESIAN_POINT('Ctrl Pts',(0.0849368486501527,-4.70856818069336,
4.3654539529372));
#36164=CARTESIAN_POINT('Ctrl Pts',(2.32666005385904,-4.09444520958252,4.4448258429906));
#36165=CARTESIAN_POINT('Ctrl Pts',(4.00161401992256,-2.48292444831813,4.52419773304401));
#36166=CARTESIAN_POINT('Ctrl Pts',(4.70178366815532,-0.266568787303479,
4.60356962309741));
#36167=CARTESIAN_POINT('Ctrl Pts',(4.25660922204708,2.0147224402583,4.68294151315081));
#36168=CARTESIAN_POINT('Ctrl Pts',(2.77453419129287,3.80523174088563,4.76231340320422));
#36169=CARTESIAN_POINT('Ctrl Pts',(0.616588772866969,4.6687950121708,4.84168529325762));
#36170=CARTESIAN_POINT('Ctrl Pts',(-1.69155630583321,4.39505015269366,4.92105718331103));
#36171=CARTESIAN_POINT('Ctrl Pts',(-3.5876420126288,3.05068080429882,5.00042907336443));
#36172=CARTESIAN_POINT('Ctrl Pts',(-4.60978606625892,0.96317236454425,5.07980096341783));
#36173=CARTESIAN_POINT('Ctrl Pts',(-4.50899643773674,-1.35896273126747,
5.15917285347124));
#36174=CARTESIAN_POINT('Ctrl Pts',(-3.30982525747623,-3.3500575137554,5.23854474352463));
#36175=CARTESIAN_POINT('Ctrl Pts',(-1.30438797066844,-4.52508570111905,
5.31791663357805));
#36176=CARTESIAN_POINT('Ctrl Pts',(1.01879533858038,-4.5978130277974,5.39728852363144));
#36177=CARTESIAN_POINT('Ctrl Pts',(3.09380235841625,-3.55052327799082,5.47666041368486));
#36178=CARTESIAN_POINT('Ctrl Pts',(4.41516597175728,-1.63833391661564,5.55603230373825));
#36179=CARTESIAN_POINT('Ctrl Pts',(4.66100492718236,0.672949960456484,5.63540419379167));
#36180=CARTESIAN_POINT('Ctrl Pts',(3.77143339930522,2.82030471671088,5.71477608384506));
#36181=CARTESIAN_POINT('Ctrl Pts',(1.96314904328358,4.28063948661312,5.79414797389847));
#36182=CARTESIAN_POINT('Ctrl Pts',(-0.323354074325263,4.69821995261119,
5.87351986395187));
#36183=CARTESIAN_POINT('Ctrl Pts',(-2.53108885516056,3.97132443748664,5.95289175400528));
#36184=CARTESIAN_POINT('Ctrl Pts',(-4.1222559933489,2.2770230797679,6.03226364405868));
#36185=CARTESIAN_POINT('Ctrl Pts',(-4.70925069601632,0.0280439399227974,
6.11163553411208));
#36186=CARTESIAN_POINT('Ctrl Pts',(-4.14908235288379,-2.22776664161329,
6.19100742416549));
#36187=CARTESIAN_POINT('Ctrl Pts',(-2.57820673242676,-3.94089820033021,
6.27037931421889));
#36188=CARTESIAN_POINT('Ctrl Pts',(-0.37928565871439,-4.6940356804769,6.34975120427229));
#36189=CARTESIAN_POINT('Ctrl Pts',(1.91202856192625,-4.30371645893114,6.42912309432569));
#36190=CARTESIAN_POINT('Ctrl Pts',(3.73757685708508,-2.86502143410457,6.5084949843791));
#36191=CARTESIAN_POINT('Ctrl Pts',(4.65265970284404,-0.728413529547492,
6.58786687443251));
#36192=CARTESIAN_POINT('Ctrl Pts',(4.43436494347775,1.58563429849135,6.6672387644859));
#36193=CARTESIAN_POINT('Ctrl Pts',(3.13586869918061,3.51342512115968,6.74661065453932));
#36194=CARTESIAN_POINT('Ctrl Pts',(1.07348178089069,4.58535336114812,6.8259825445927));
#36195=CARTESIAN_POINT('Ctrl Pts',(-1.25040292311256,4.54029967186839,6.90535443464612));
#36196=CARTESIAN_POINT('Ctrl Pts',(-3.26969224276554,3.38923903230437,6.98472632469952));
#36197=CARTESIAN_POINT('Ctrl Pts',(-4.49249176942184,1.41256726642436,7.06409821475293));
#36198=CARTESIAN_POINT('Ctrl Pts',(-4.62093024500886,-0.908202758892002,
7.14347010480633));
#36199=CARTESIAN_POINT('Ctrl Pts',(-3.62372034116731,-3.00773660241498,
7.22284199485974));
#36200=CARTESIAN_POINT('Ctrl Pts',(-1.74378018318635,-4.37459246710173,
7.30221388491313));
#36201=CARTESIAN_POINT('Ctrl Pts',(0.560940967626854,-4.67580728979868,
7.38158577496654));
#36202=CARTESIAN_POINT('Ctrl Pts',(2.72901814034792,-3.83800580642455,7.46095766501994));
#36203=CARTESIAN_POINT('Ctrl Pts',(4.23231253465944,-2.06527460388716,7.54032955507336));
#36204=CARTESIAN_POINT('Ctrl Pts',(4.70462496359279,0.210552920749357,7.61970144512673));
#36205=CARTESIAN_POINT('Ctrl Pts',(4.03090116490568,2.4350902199423,7.69907333518017));
#36206=CARTESIAN_POINT('Ctrl Pts',(2.37525876469593,4.06644493153808,7.77844522523354));
#36207=CARTESIAN_POINT('Ctrl Pts',(0.141008586952364,4.70722265873438,7.85781711528697));
#36208=CARTESIAN_POINT('Ctrl Pts',(-2.1275909704556,4.2013313655236,7.93718900534037));
#36209=CARTESIAN_POINT('Ctrl Pts',(-3.87791407680332,2.67200505116051,8.01656089539376));
#36210=CARTESIAN_POINT('Ctrl Pts',(-4.68358589765895,0.491784220717585,
8.09593278544718));
#36211=CARTESIAN_POINT('Ctrl Pts',(-4.3483465607864,-1.80823415734624,8.17530467550056));
#36212=CARTESIAN_POINT('Ctrl Pts',(-2.95385962660815,-3.66777069713892,
8.25467656555399));
#36213=CARTESIAN_POINT('Ctrl Pts',(-0.839819025645543,-4.63384641358131,
8.33404845560737));
#36214=CARTESIAN_POINT('Ctrl Pts',(1.47879963105641,-4.47112740052035,8.41342034566079));
#36215=CARTESIAN_POINT('Ctrl Pts',(3.43718597090052,-3.21925164936531,8.49279223571418));
#36216=CARTESIAN_POINT('Ctrl Pts',(4.55828141631537,-1.1831733221175,8.57216412576761));
#36217=CARTESIAN_POINT('Ctrl Pts',(4.56898959830056,1.1411234074884,8.65153601582098));
#36218=CARTESIAN_POINT('Ctrl Pts',(3.46670202742665,3.18744500086393,8.73090790587441));
#36219=CARTESIAN_POINT('Ctrl Pts',(1.51993351608642,4.45731204731885,8.8102797959278));
#36220=CARTESIAN_POINT('Ctrl Pts',(-0.797087435456723,4.64138774513978,
8.88965168598121));
#36221=CARTESIAN_POINT('Ctrl Pts',(-2.91993965204571,3.69483166178214,8.96902357603462));
#36222=CARTESIAN_POINT('Ctrl Pts',(-4.33150103257314,1.84822276398555,9.04839546608801));
#36223=CARTESIAN_POINT('Ctrl Pts',(-4.68791834918067,-0.448609108146216,
9.12776735614143));
#36224=CARTESIAN_POINT('Ctrl Pts',(-3.90236913245906,-2.63616079451299,
9.20713924619481));
#36225=CARTESIAN_POINT('Ctrl Pts',(-2.16621143281798,-4.18154954637933,
9.28651113624823));
#36226=CARTESIAN_POINT('Ctrl Pts',(0.0976305770298679,-4.70832208445062,
9.36588302630162));
#36227=CARTESIAN_POINT('Ctrl Pts',(2.33768999441487,-4.08815778444389,9.44525491635505));
#36228=CARTESIAN_POINT('Ctrl Pts',(4.00829330354943,-2.47212729713041,9.52462680640842));
#36229=CARTESIAN_POINT('Ctrl Pts',(4.70248523614611,-0.253892072196923,
9.60399869646185));
#36230=CARTESIAN_POINT('Ctrl Pts',(4.25116217399211,2.02619069954319,9.68337058651524));
#36231=CARTESIAN_POINT('Ctrl Pts',(2.76426541604147,3.81269790177162,9.76274247656865));
#36232=CARTESIAN_POINT('Ctrl Pts',(0.603999721340871,4.67044033439211,9.84211436662206));
#36233=CARTESIAN_POINT('Ctrl Pts',(-1.70339896854767,4.39047383939904,9.92148625667545));
#36234=CARTESIAN_POINT('Ctrl Pts',(-3.59585344010767,3.04099763527736,10.0008581467289));
#36235=CARTESIAN_POINT('Ctrl Pts',(-4.61236597294403,0.95074113833618,10.0802300367823));
#36236=CARTESIAN_POINT('Ctrl Pts',(-4.5053163640701,-1.37111379547384,10.1596019268357));
#36237=CARTESIAN_POINT('Ctrl Pts',(-3.30078166125737,-3.35896844361534,
10.2389738168891));
#36238=CARTESIAN_POINT('Ctrl Pts',(-1.29218385191862,-4.5285858138427,10.3183457069425));
#36239=CARTESIAN_POINT('Ctrl Pts',(1.03118708354706,-4.59504970367267,10.3977175969959));
#36240=CARTESIAN_POINT('Ctrl Pts',(3.1033631279546,-3.54216965665798,10.4770894870493));
#36241=CARTESIAN_POINT('Ctrl Pts',(4.41956678357015,-1.62642492174092,10.5564613771027));
#36242=CARTESIAN_POINT('Ctrl Pts',(4.65917375325315,0.68551332408169,10.6358332671561));
#36243=CARTESIAN_POINT('Ctrl Pts',(3.76381630954987,2.83046204151602,10.7152051572095));
#36244=CARTESIAN_POINT('Ctrl Pts',(1.95160154390631,4.28591647075852,10.7945770472629));
#36245=CARTESIAN_POINT('Ctrl Pts',(-0.336019038036085,4.69733113443942,
10.8739489373163));
#36246=CARTESIAN_POINT('Ctrl Pts',(-2.54178612607839,3.96448633113698,10.9533208273697));
#36247=CARTESIAN_POINT('Ctrl Pts',(-4.12837973995617,2.26590143281123,11.0326927174231));
#36248=CARTESIAN_POINT('Ctrl Pts',(-4.70930918719419,0.0153479609404256,
11.1120646074765));
#36249=CARTESIAN_POINT('Ctrl Pts',(-4.14306134031078,-2.23894424024334,
11.1914364975299));
#36250=CARTESIAN_POINT('Ctrl Pts',(-2.5675729214384,-3.94783458032284,11.2708083875833));
#36251=CARTESIAN_POINT('Ctrl Pts',(-0.366629422129896,-4.69504115501934,
11.3501802776367));
#36252=CARTESIAN_POINT('Ctrl Pts',(1.92362419288899,-4.29854609665044,11.4295521676901));
#36253=CARTESIAN_POINT('Ctrl Pts',(3.74528721239005,-2.85493472380791,11.5089240577435));
#36254=CARTESIAN_POINT('Ctrl Pts',(4.65460655700554,-0.715867571536574,
11.5882959477969));
#36255=CARTESIAN_POINT('Ctrl Pts',(4.43007404713131,1.59758333661508,11.6676678378504));
#36256=CARTESIAN_POINT('Ctrl Pts',(3.12638530517848,3.52186648015801,11.7470397279037));
#36257=CARTESIAN_POINT('Ctrl Pts',(1.06111602302068,4.5882307446537,11.8264116179572));
#36258=CARTESIAN_POINT('Ctrl Pts',(-1.26263877360451,4.53691215562823,11.9057835080105));
#36259=CARTESIAN_POINT('Ctrl Pts',(-3.27881755978316,3.38041180777642,11.985155398064));
#36260=CARTESIAN_POINT('Ctrl Pts',(-4.49628364593817,1.40045062596491,12.0645272881173));
#36261=CARTESIAN_POINT('Ctrl Pts',(-4.6184649882977,-0.920657228486762,
12.1438991781708));
#36262=CARTESIAN_POINT('Ctrl Pts',(-3.61559848230676,-3.01749501991928,
12.2232710682242));
#36263=CARTESIAN_POINT('Ctrl Pts',(-1.7319801890174,-4.37927770361138,12.3026429582776));
#36264=CARTESIAN_POINT('Ctrl Pts',(0.573544644643477,-4.67427803207056,
12.382014848331));
#36265=CARTESIAN_POINT('Ctrl Pts',(2.73935527238874,-3.83063457825627,12.4613867383844));
#36266=CARTESIAN_POINT('Ctrl Pts',(4.23786501924016,-2.05385702014458,12.5407586284378));
#36267=CARTESIAN_POINT('Ctrl Pts',(4.7040402277598,0.22323556193892,12.6201305184912));
#36268=CARTESIAN_POINT('Ctrl Pts',(4.02432164901358,2.44594845525766,12.6995024085446));
#36269=CARTESIAN_POINT('Ctrl Pts',(2.3642872242525,4.0728337188907,12.778874298598));
#36270=CARTESIAN_POINT('Ctrl Pts',(0.12831766492455,4.70758570366646,12.8582461886514));
#36271=CARTESIAN_POINT('Ctrl Pts',(-2.13890979355269,4.19558023109331,12.9376180787048));
#36272=CARTESIAN_POINT('Ctrl Pts',(-3.88510356071705,2.66154070098513,13.0169899687582));
#36273=CARTESIAN_POINT('Ctrl Pts',(-4.68489470002156,0.479155747337376,
13.0963618588116));
#36274=CARTESIAN_POINT('Ctrl Pts',(-4.34345586023936,-1.81995048576848,
13.175733748865));
#36275=CARTESIAN_POINT('Ctrl Pts',(-2.94396078697933,-3.67572080893321,
13.2551056389184));
#36276=CARTESIAN_POINT('Ctrl Pts',(-0.827323382357809,-4.63609367911183,
13.3344775289718));
#36277=CARTESIAN_POINT('Ctrl Pts',(1.49084816695683,-4.4671243908781,13.4138494190252));
#36278=CARTESIAN_POINT('Ctrl Pts',(3.44585240273723,-3.2099734888386,13.4932213090786));
#36279=CARTESIAN_POINT('Ctrl Pts',(4.56145462047577,-1.17088015007382,13.572593199132));
#36280=CARTESIAN_POINT('Ctrl Pts',(4.56589658927495,1.15343700154968,13.6519650891854));
#36281=CARTESIAN_POINT('Ctrl Pts',(3.45809625536746,3.19677945268519,13.7313369792388));
#36282=CARTESIAN_POINT('Ctrl Pts',(1.50791132801865,4.4613935050979,13.8107088692922));
#36283=CARTESIAN_POINT('Ctrl Pts',(-0.809597461130395,4.63922197479575,
13.8900807593457));
#36284=CARTESIAN_POINT('Ctrl Pts',(-2.92989010076163,3.68694624017703,13.969452649399));
#36285=CARTESIAN_POINT('Ctrl Pts',(-4.33646799704908,1.83653856236827,14.0488245394525));
#36286=CARTESIAN_POINT('Ctrl Pts',(-4.68669188786449,-0.461245844124263,
14.1281964295058));
#36287=CARTESIAN_POINT('Ctrl Pts',(-3.8952480086126,-2.64667178393849,14.2075683195593));
#36288=CARTESIAN_POINT('Ctrl Pts',(-2.15493033644793,-4.1873743354939,14.2869402096127));
#36289=CARTESIAN_POINT('Ctrl Pts',(0.110323595818042,-4.70804176751889,
14.3663120996661));
#36290=CARTESIAN_POINT('Ctrl Pts',(2.34870294433987,-4.08184064604999,14.4456839897195));
#36291=CARTESIAN_POINT('Ctrl Pts',(4.01494345438633,-2.46131217820434,14.5250558797729));
#36292=CARTESIAN_POINT('Ctrl Pts',(4.70315262587088,-0.241213511770193,
14.6044277698263));
#36293=CARTESIAN_POINT('Ctrl Pts',(4.24568422794502,2.03764423221413,14.6837996598797));
#36294=CARTESIAN_POINT('Ctrl Pts',(2.7539765497544,3.82013635148006,14.7631715499331));
#36295=CARTESIAN_POINT('Ctrl Pts',(0.591406279867313,4.67205171125386,14.8425434399865));
#36296=CARTESIAN_POINT('Ctrl Pts',(-1.71522925073988,4.38586561557727,14.9219153300399));
#36297=CARTESIAN_POINT('Ctrl Pts',(-3.60403873246238,3.0312923638949,15.0012872200933));
#36298=CARTESIAN_POINT('Ctrl Pts',(-4.61491235636145,0.938303002019602,
15.0806591101467));
#36299=CARTESIAN_POINT('Ctrl Pts',(-4.50160354518612,-1.38325489424921,
15.1600310002001));
#36300=CARTESIAN_POINT('Ctrl Pts',(-3.29171407453388,-3.36785496006171,
15.2394028902535));
#36301=CARTESIAN_POINT('Ctrl Pts',(-1.27997034141067,-4.53205301222367,
15.3187747803069));
#36302=CARTESIAN_POINT('Ctrl Pts',(1.04357133371383,-4.59225298213712,15.3981466703603));
#36303=CARTESIAN_POINT('Ctrl Pts',(3.11290134185163,-3.53379029038156,15.4775185604137));
#36304=CARTESIAN_POINT('Ctrl Pts',(4.42393547340459,-1.6145041058012,15.5568904504671));
#36305=CARTESIAN_POINT('Ctrl Pts',(4.65730871585136,0.69807170530811,15.6362623405205));
#36306=CARTESIAN_POINT('Ctrl Pts',(3.75617186389461,2.84059879415993,15.7156342305739));
#36307=CARTESIAN_POINT('Ctrl Pts',(1.94003986003872,4.2911623043131,15.7950061206273));
#36308=CARTESIAN_POINT('Ctrl Pts',(-0.348681559517582,4.69640817546235,
15.8743780106807));
#36309=CARTESIAN_POINT('Ctrl Pts',(-2.55246492296822,3.95761941039193,15.9537499007341));
#36310=CARTESIAN_POINT('Ctrl Pts',(-4.13447348097045,2.25476331699244,16.0331217907876));
#36311=CARTESIAN_POINT('Ctrl Pts',(-4.70933345050753,0.00265187040668795,
16.1124936808409));
#36312=CARTESIAN_POINT('Ctrl Pts',(-4.13701021543854,-2.25010556593871,
16.1918655708943));
#36313=CARTESIAN_POINT('Ctrl Pts',(-2.55692044899651,-3.95474226694862,
16.2712374609477));
#36314=CARTESIAN_POINT('Ctrl Pts',(-0.353970520843347,-4.69601250539775,
16.3506093510012));
#36315=CARTESIAN_POINT('Ctrl Pts',(1.93520584271894,-4.29334449198998,16.4299812410546));
#36316=CARTESIAN_POINT('Ctrl Pts',(3.75297034643966,-2.8448272634702,16.509353131108));
#36317=CARTESIAN_POINT('Ctrl Pts',(4.65651958094123,-0.703316410525392,
16.5887250211614));
#36318=CARTESIAN_POINT('Ctrl Pts',(4.42575095234045,1.60952076333056,16.6680969112148));
#36319=CARTESIAN_POINT('Ctrl Pts',(3.11687918839165,3.53028224171774,16.7474688012682));
#36320=CARTESIAN_POINT('Ctrl Pts',(1.04874255247428,4.59107478042509,16.8268406913216));
#36321=CARTESIAN_POINT('Ctrl Pts',(-1.27486544641699,4.53349166431028,16.906212581375));
#36322=CARTESIAN_POINT('Ctrl Pts',(-3.28791904717816,3.37156001439364,16.9855844714284));
#36323=CARTESIAN_POINT('Ctrl Pts',(-4.50004284053898,1.38832380607291,17.0649563614818));
#36324=CARTESIAN_POINT('Ctrl Pts',(-4.61596616842608,-0.933105005158158,
17.1443282515352));
#36325=CARTESIAN_POINT('Ctrl Pts',(-3.60745033643721,-3.02723150865552,
17.2237001415886));
#36326=CARTESIAN_POINT('Ctrl Pts',(-1.72016762240852,-4.3839311057331,17.303072031642));
#36327=CARTESIAN_POINT('Ctrl Pts',(0.586144182924747,-4.67271481097615,
17.3824439216954));
#36328=CARTESIAN_POINT('Ctrl Pts',(2.74967243806105,-3.82323548987727,17.4618158117488));
#36329=CARTESIAN_POINT('Ctrl Pts',(4.24338680893684,-2.04242454395285,17.5411877018022));
#36330=CARTESIAN_POINT('Ctrl Pts',(4.70342110133588,0.235916647177909,17.6205595918556));
#36331=CARTESIAN_POINT('Ctrl Pts',(4.01771326340766,2.45678878743836,17.699931481909));
#36332=CARTESIAN_POINT('Ctrl Pts',(2.35329778315649,4.07919314165109,17.7793033719624));
#36333=CARTESIAN_POINT('Ctrl Pts',(0.115627163561191,4.70791408521782,17.8586752620158));
#36334=CARTESIAN_POINT('Ctrl Pts',(-2.15021562607272,4.18979944864554,17.9380471520692));
#36335=CARTESIAN_POINT('Ctrl Pts',(-3.89225998228542,2.6510554089743,18.0174190421226));
#36336=CARTESIAN_POINT('Ctrl Pts',(-4.68617856238767,0.466526807638264,
18.096790932176));
#36337=CARTESIAN_POINT('Ctrl Pts',(-4.33851638857381,-1.83165928184378,
18.1761628222294));
#36338=CARTESIAN_POINT('Ctrl Pts',(-2.93407303174987,-3.68363345125881,
18.2555347122828));
#36339=CARTESIAN_POINT('Ctrl Pts',(-0.814760394348088,-4.63832755437977,
18.3349066023362));
#36340=CARTESIAN_POINT('Ctrl Pts',(1.50277006074129,-4.46305057284721,18.4142784923896));
#36341=CARTESIAN_POINT('Ctrl Pts',(3.45471245456617,-3.20074439226408,18.493650382443));
#36342=CARTESIAN_POINT('Ctrl Pts',(4.56418179760217,-1.15844177813615,18.5730222724965));
#36343=CARTESIAN_POINT('Ctrl Pts',(4.56354990278295,1.16548416044567,18.6523941625499));
#36344=CARTESIAN_POINT('Ctrl Pts',(3.44799414715945,3.20657754587687,18.7317660526033));
#36345=CARTESIAN_POINT('Ctrl Pts',(1.49865065220682,4.46452630956668,18.8111379426567));
#36346=CARTESIAN_POINT('Ctrl Pts',(-0.827291992766502,4.63872722375952,
18.8905098327101));
#36347=CARTESIAN_POINT('Ctrl Pts',(-2.93038174053102,3.67602118591242,18.9698817227635));
#36348=CARTESIAN_POINT('Ctrl Pts',(-4.8317659974063,1.21320979378885,19.0757109095013));
#36349=CARTESIAN_POINT('Ctrl Pts',(-4.41154214902252,-3.00742829557681,
19.2079973929237));
#36350=CARTESIAN_POINT('Ctrl Pts',(0.14114360583215,-5.34031031892966,19.3667411730305));
#36351=CARTESIAN_POINT('Ctrl Pts',(4.55878074835922,-2.77696271962162,19.5254849531373));
#36352=CARTESIAN_POINT('Ctrl Pts',(4.80798654830346,2.32253130646654,19.6842287332441));
#36353=CARTESIAN_POINT('Ctrl Pts',(0.656009676029318,5.29932988758691,19.8429725133509));
#36354=CARTESIAN_POINT('Ctrl Pts',(-4.09539160933947,3.42571876325565,20.0017162934577));
#36355=CARTESIAN_POINT('Ctrl Pts',(-5.09974667860472,-1.58211192901314,
20.1604600735645));
#36356=CARTESIAN_POINT('Ctrl Pts',(-1.43734916996091,-5.14215993940121,
20.3192038536714));
#36357=CARTESIAN_POINT('Ctrl Pts',(3.54020456892056,-3.99752392897281,20.4779476337781));
#36358=CARTESIAN_POINT('Ctrl Pts',(5.27828887711237,0.806568563691912,20.636691413885));
#36359=CARTESIAN_POINT('Ctrl Pts',(2.1865632094635,4.86959394496087,20.7954351939918));
#36360=CARTESIAN_POINT('Ctrl Pts',(-2.90621803008048,4.48249178265495,20.9541789740986));
#36361=CARTESIAN_POINT('Ctrl Pts',(-5.339103029404,-0.0175478502156508,
21.1129227542054));
#36362=CARTESIAN_POINT('Ctrl Pts',(-3.29668819545046,-3.73492805813105,
21.2452092376277));
#36363=CARTESIAN_POINT('Ctrl Pts',(-0.335233909123966,-4.68912434583344,
21.3510384243656));
#36364=CARTESIAN_POINT('Ctrl Pts',(1.9434592869775,-4.29245481019942,21.430410314419));
#36365=CARTESIAN_POINT('Ctrl Pts',(3.76239327895729,-2.83237457985877,21.5097822044724));
#36366=CARTESIAN_POINT('Ctrl Pts',(4.65746145505442,-0.691994213306775,
21.5891540945258));
#36367=CARTESIAN_POINT('Ctrl Pts',(4.42189226956134,1.62210042840564,21.6685259845792));
#36368=CARTESIAN_POINT('Ctrl Pts',(3.10708740551244,3.53832597274477,21.7478978746326));
#36369=CARTESIAN_POINT('Ctrl Pts',(1.03650075501011,4.59406889295405,21.827269764686));
#36370=CARTESIAN_POINT('Ctrl Pts',(-1.28715662605568,4.52994106929143,21.9066416547395));
#36371=CARTESIAN_POINT('Ctrl Pts',(-3.29695756540469,3.36273516855513,21.9860135447928));
#36372=CARTESIAN_POINT('Ctrl Pts',(-4.5037900244027,1.37615964733944,22.0653854348462));
#36373=CARTESIAN_POINT('Ctrl Pts',(-4.61342283197247,-0.945531571193242,
22.1447573248996));
#36374=CARTESIAN_POINT('Ctrl Pts',(-3.59928179145312,-3.03695363259649,
22.224129214953));
#36375=CARTESIAN_POINT('Ctrl Pts',(-1.70833944819064,-4.388548607559,22.3035011050065));
#36376=CARTESIAN_POINT('Ctrl Pts',(0.598737773532913,-4.67111975194625,
22.3828729950598));
#36377=CARTESIAN_POINT('Ctrl Pts',(2.75997059360609,-3.81580751573965,22.4622448851133));
#36378=CARTESIAN_POINT('Ctrl Pts',(4.24887708766878,-2.03097775393672,22.5416167751666));
#36379=CARTESIAN_POINT('Ctrl Pts',(4.7027684336848,0.248596203073706,22.6209886652201));
#36380=CARTESIAN_POINT('Ctrl Pts',(4.01107478934813,2.46761134605171,22.7003605552734));
#36381=CARTESIAN_POINT('Ctrl Pts',(2.34229273922348,4.08552253105782,22.7797324453269));
#36382=CARTESIAN_POINT('Ctrl Pts',(0.10293307930986,4.70820909782832,22.8591043353802));
#36383=CARTESIAN_POINT('Ctrl Pts',(-2.16150070095897,4.18398654725925,22.9384762254337));
#36384=CARTESIAN_POINT('Ctrl Pts',(-3.89939777427635,2.64055403030605,23.017848115487));
#36385=CARTESIAN_POINT('Ctrl Pts',(-4.6874101388992,0.453888451717589,23.0972200055405));
#36386=CARTESIAN_POINT('Ctrl Pts',(-4.33357979136315,-1.84334337837373,
23.1765918955938));
#36387=CARTESIAN_POINT('Ctrl Pts',(-2.92409898707257,-3.69154082613157,
23.2559637856473));
#36388=CARTESIAN_POINT('Ctrl Pts',(-0.802314148160901,-4.64048710795707,
23.3353356757007));
#36389=CARTESIAN_POINT('Ctrl Pts',(1.51491264465863,-4.45902099747155,23.4147075657541));
#36390=CARTESIAN_POINT('Ctrl Pts',(3.46311006868958,-3.19134724418486,23.4940794558075));
#36391=CARTESIAN_POINT('Ctrl Pts',(4.56770154637975,-1.14626836492011,23.5734513458609));
#36392=CARTESIAN_POINT('Ctrl Pts',(4.55961103731633,1.17803895017003,23.6528232359143));
#36393=CARTESIAN_POINT('Ctrl Pts',(3.44080937235073,3.21537858488653,23.7321951259677));
#36394=CARTESIAN_POINT('Ctrl Pts',(1.48383416024502,4.46945911326291,23.8115670160211));
#36395=CARTESIAN_POINT('Ctrl Pts',(-0.834599768812189,4.6347892947245,23.8909389060745));
#36396=CARTESIAN_POINT('Ctrl Pts',(-2.94972704158065,3.67109506287238,23.9703107961279));
#36397=CARTESIAN_POINT('Ctrl Pts',(-4.34630733610966,1.81313019956259,24.0496826861813));
#36398=CARTESIAN_POINT('Ctrl Pts',(-4.68413678396127,-0.486509167079313,
24.1290545762347));
#36399=CARTESIAN_POINT('Ctrl Pts',(-3.8809208793951,-2.66763597748286,24.2084264662881));
#36400=CARTESIAN_POINT('Ctrl Pts',(-2.13232123888401,-4.19893256848769,
24.2877983563416));
#36401=CARTESIAN_POINT('Ctrl Pts',(0.13570713560786,-4.70737847998643,24.3671702463949));
#36402=CARTESIAN_POINT('Ctrl Pts',(2.37067755224746,-4.06911741336709,24.4465421364484));
#36403=CARTESIAN_POINT('Ctrl Pts',(4.02815616456577,-2.43962835168955,24.5259140265017));
#36404=CARTESIAN_POINT('Ctrl Pts',(4.70438485136804,-0.215851223566548,
24.6052859165551));
#36405=CARTESIAN_POINT('Ctrl Pts',(4.23463580135646,2.06050678483885,24.6846578066085));
#36406=CARTESIAN_POINT('Ctrl Pts',(2.73333884334173,3.83492990131186,24.7640296966619));
#36407=CARTESIAN_POINT('Ctrl Pts',(0.566206593231879,4.6751725822987,24.8434015867153));
#36408=CARTESIAN_POINT('Ctrl Pts',(-1.73885232971224,4.3765535705565,24.9227734767688));
#36409=CARTESIAN_POINT('Ctrl Pts',(-3.62033067402275,3.0118157963638,25.0021453668221));
#36410=CARTESIAN_POINT('Ctrl Pts',(-4.61990447960738,0.913406360718075,
25.0815172568756));
#36411=CARTESIAN_POINT('Ctrl Pts',(-4.49407977994478,-1.40750684260792,
25.1608891469289));
#36412=CARTESIAN_POINT('Ctrl Pts',(-3.27350719336448,-3.38555449453819,
25.2402610369824));
#36413=CARTESIAN_POINT('Ctrl Pts',(-1.25551550026584,-4.53888856539668,
25.3196329270357));
#36414=CARTESIAN_POINT('Ctrl Pts',(1.06831698966113,-4.58655942838399,25.3990048170892));
#36415=CARTESIAN_POINT('Ctrl Pts',(3.1319098255862,-3.51695456679402,25.4783767071426));
#36416=CARTESIAN_POINT('Ctrl Pts',(4.43257636036326,-1.59062735737991,25.557748597196));
#36417=CARTESIAN_POINT('Ctrl Pts',(4.65347710509718,0.723173155497971,25.6371204872493));
#36418=CARTESIAN_POINT('Ctrl Pts',(3.74080112732632,2.86081028841317,25.7164923773028));
#36419=CARTESIAN_POINT('Ctrl Pts',(1.91687427506164,4.30156036736711,25.7958642673562));
#36420=CARTESIAN_POINT('Ctrl Pts',(-0.373998907678805,4.69445986217281,
25.8752361574096));
#36421=CARTESIAN_POINT('Ctrl Pts',(-2.57376678434128,3.9437993255639,25.954608047463));
#36422=CARTESIAN_POINT('Ctrl Pts',(-4.14657076927436,2.23243800269932,26.0339799375164));
#36423=CARTESIAN_POINT('Ctrl Pts',(-4.70927929309089,-0.0227402762051125,
26.1133518275698));
#36424=CARTESIAN_POINT('Ctrl Pts',(-4.1248178049234,-2.27237907416072,26.1927237176232));
#36425=CARTESIAN_POINT('Ctrl Pts',(-2.53555982960589,-3.96847135947655,
26.2720956076766));
#36426=CARTESIAN_POINT('Ctrl Pts',(-0.328645092162861,-4.69785280568621,
26.35146749773));
#36427=CARTESIAN_POINT('Ctrl Pts',(1.95832686228742,-4.28284770695154,26.4308393877834));
#36428=CARTESIAN_POINT('Ctrl Pts',(3.76825472776749,-2.8245503867261,26.5102112778369));
#36429=CARTESIAN_POINT('Ctrl Pts',(4.66024408245379,-0.67819884433039,26.5895831678902));
#36430=CARTESIAN_POINT('Ctrl Pts',(4.41700829392964,1.63336043537654,26.6689550579436));
#36431=CARTESIAN_POINT('Ctrl Pts',(3.09779906188623,3.54703672840772,26.748326947997));
#36432=CARTESIAN_POINT('Ctrl Pts',(1.0239728352293,4.59666272563139,26.8276988380504));
#36433=CARTESIAN_POINT('Ctrl Pts',(-1.29929090756406,4.52655185743165,26.9070707281039));
#36434=CARTESIAN_POINT('Ctrl Pts',(-3.30605026120649,3.35378297611415,26.9864426181572));
#36435=CARTESIAN_POINT('Ctrl Pts',(-4.50746308903716,1.36403998528792,27.0658145082107));
#36436=CARTESIAN_POINT('Ctrl Pts',(-4.61086788547865,-0.957980126703151,
27.1451863982641));
#36437=CARTESIAN_POINT('Ctrl Pts',(-3.59107547100053,-3.04663840028233,
27.2245582883174));
#36438=CARTESIAN_POINT('Ctrl Pts',(-1.69650502049742,-4.39314230317249,
27.3039301783709));
#36439=CARTESIAN_POINT('Ctrl Pts',(0.611330297848721,-4.66948646506538,
27.3833020684242));
#36440=CARTESIAN_POINT('Ctrl Pts',(2.77024690879558,-3.80835405980132,27.4626739584777));
#36441=CARTESIAN_POINT('Ctrl Pts',(4.25433750459734,-2.01951503521836,27.542045848531));
#36442=CARTESIAN_POINT('Ctrl Pts',(4.70208090109553,0.261273381823074,27.6214177385845));
#36443=CARTESIAN_POINT('Ctrl Pts',(4.00440779796637,2.47841618137125,27.7007896286379));
#36444=CARTESIAN_POINT('Ctrl Pts',(2.33126981885889,4.09182228501852,27.7801615186913));
#36445=CARTESIAN_POINT('Ctrl Pts',(0.0902396720556605,4.70846953713028,
27.8595334087446));
#36446=CARTESIAN_POINT('Ctrl Pts',(-2.17277265911822,4.17814403201768,27.9389052987981));
#36447=CARTESIAN_POINT('Ctrl Pts',(-3.90650237988159,2.63003188887054,28.0182771888515));
#36448=CARTESIAN_POINT('Ctrl Pts',(-4.68861676780222,0.441249799071397,
28.0976490789049));
#36449=CARTESIAN_POINT('Ctrl Pts',(-4.32859448916339,-1.85501976509172,
28.1770209689583));
#36450=CARTESIAN_POINT('Ctrl Pts',(-2.91413617414575,-3.69941062049508,
28.2563928590117));
#36451=CARTESIAN_POINT('Ctrl Pts',(-0.78980073743719,-4.64263323725236,
28.3357647490651));
#36452=CARTESIAN_POINT('Ctrl Pts',(1.52692841071678,-4.4549206737093,28.4151366391185));
#36453=CARTESIAN_POINT('Ctrl Pts',(3.47170117781886,-3.18199929485031,28.494508529172));
#36454=CARTESIAN_POINT('Ctrl Pts',(4.57077522248444,-1.13394993100173,28.5738804192253));
#36455=CARTESIAN_POINT('Ctrl Pts',(4.55641854019218,1.19032712608322,28.6532523092787));
#36456=CARTESIAN_POINT('Ctrl Pts',(3.43212838697049,3.22464312999871,28.7326241993321));
#36457=CARTESIAN_POINT('Ctrl Pts',(1.47177935557015,4.47344320507303,28.8119960893855));
#36458=CARTESIAN_POINT('Ctrl Pts',(-0.84709186911874,4.63252241719017,28.891367979439));
#36459=CARTESIAN_POINT('Ctrl Pts',(-2.95961338949639,3.66312942239424,28.9707398694923));
#36460=CARTESIAN_POINT('Ctrl Pts',(-4.35117963918583,1.80140620850249,29.0501117595457));
#36461=CARTESIAN_POINT('Ctrl Pts',(-4.68280815994235,-0.499135570435458,
29.1294836495992));
#36462=CARTESIAN_POINT('Ctrl Pts',(-3.87371497815696,-2.67808902923317,
29.2088555396525));
#36463=CARTESIAN_POINT('Ctrl Pts',(-2.12099340201518,-4.2046659283592,29.288227429706));
#36464=CARTESIAN_POINT('Ctrl Pts',(0.148397472118242,-4.70699551420707,
29.3675993197594));
#36465=CARTESIAN_POINT('Ctrl Pts',(2.38163905051584,-4.06271141155196,29.4469712098127));
#36466=CARTESIAN_POINT('Ctrl Pts',(4.03471862787643,-2.428759801702,29.5263430998662));
#36467=CARTESIAN_POINT('Ctrl Pts',(4.70494967818454,-0.203167680126035,
29.6057149899196));
#36468=CARTESIAN_POINT('Ctrl Pts',(4.22906540111636,2.07191563862461,29.685086879973));
#36469=CARTESIAN_POINT('Ctrl Pts',(2.72299015321369,3.84228489391376,29.7644587700264));
#36470=CARTESIAN_POINT('Ctrl Pts',(0.553600531224683,4.67668205379885,29.8438306600798));
#36471=CARTESIAN_POINT('Ctrl Pts',(-1.75064495479666,4.37184981703873,29.9232025501332));
#36472=CARTESIAN_POINT('Ctrl Pts',(-3.62843720481647,3.00204464177339,30.0025744401866));
#36473=CARTESIAN_POINT('Ctrl Pts',(-4.62235018315249,0.900948036685143,
30.08194633024));
#36474=CARTESIAN_POINT('Ctrl Pts',(-4.49026888827113,-1.41961751592495,
30.1613182202934));
#36475=CARTESIAN_POINT('Ctrl Pts',(-3.26436803124854,-3.39436738392576,
30.2406901103467));
#36476=CARTESIAN_POINT('Ctrl Pts',(-1.24327434736992,-4.54225687050705,
30.3200620004003));
#36477=CARTESIAN_POINT('Ctrl Pts',(1.08067821558697,-4.58366263754788,30.3994338904535));
#36478=CARTESIAN_POINT('Ctrl Pts',(3.14137995726753,-3.50849833184719,30.4788057805071));
#36479=CARTESIAN_POINT('Ctrl Pts',(4.4368484946843,-1.57867159843783,30.5581776705604));
#36480=CARTESIAN_POINT('Ctrl Pts',(4.65151055959353,0.735716042020659,30.6375495606138));
#36481=CARTESIAN_POINT('Ctrl Pts',(3.73307494812974,2.87088488312276,30.7169214506672));
#36482=CARTESIAN_POINT('Ctrl Pts',(1.90527054232277,4.30671252129204,30.7962933407206));
#36483=CARTESIAN_POINT('Ctrl Pts',(-0.386653550349159,4.69343452202104,
30.875665230774));
#36484=CARTESIAN_POINT('Ctrl Pts',(-2.58438969399916,3.93684626192686,30.9550371208274));
#36485=CARTESIAN_POINT('Ctrl Pts',(-4.15257422864054,2.2212509664887,31.0344090108808));
#36486=CARTESIAN_POINT('Ctrl Pts',(-4.70920087275226,-0.0354361477304668,
31.1137809009342));
#36487=CARTESIAN_POINT('Ctrl Pts',(-4.11867660790086,-2.28349109479913,
31.1931527909877));
#36488=CARTESIAN_POINT('Ctrl Pts',(-2.52485183790083,-3.97529266559651,
31.272524681041));
#36489=CARTESIAN_POINT('Ctrl Pts',(-0.315978748852904,-4.69872174221564,
31.3518965710945));
#36490=CARTESIAN_POINT('Ctrl Pts',(1.9698660640085,-4.27755260287519,31.4312684611479));
#36491=CARTESIAN_POINT('Ctrl Pts',(3.77585586390199,-2.81438111767642,31.5106403512012));
#36492=CARTESIAN_POINT('Ctrl Pts',(4.66205553306415,-0.665632621738598,
31.5900122412547));
#36493=CARTESIAN_POINT('Ctrl Pts',(4.41258879365675,1.64526250750188,31.669384131308));
#36494=CARTESIAN_POINT('Ctrl Pts',(3.08822519121424,3.55537533164171,31.7487560213615));
#36495=CARTESIAN_POINT('Ctrl Pts',(1.01157676786242,4.59940659468345,31.8281279114149));
#36496=CARTESIAN_POINT('Ctrl Pts',(-1.31148951705349,4.52303259187412,31.9074998014683));
#36497=CARTESIAN_POINT('Ctrl Pts',(-3.31507985854797,3.34485786124704,31.9868716915217));
#36498=CARTESIAN_POINT('Ctrl Pts',(-4.51112408430495,1.35188315933753,32.066243581575));
#36499=CARTESIAN_POINT('Ctrl Pts',(-4.60826846832906,-0.970407287843986,
32.1456154716285));
#36500=CARTESIAN_POINT('Ctrl Pts',(-3.58284885369746,-3.05630866766684,
32.2249873616819));
#36501=CARTESIAN_POINT('Ctrl Pts',(-1.68465518880656,-4.39770002107054,
32.3043592517353));
#36502=CARTESIAN_POINT('Ctrl Pts',(0.623916751156621,-4.66782138348531,
32.3837311417887));
#36503=CARTESIAN_POINT('Ctrl Pts',(2.7805039515543,-3.80087178893047,32.4631030318421));
#36504=CARTESIAN_POINT('Ctrl Pts',(4.25976654389448,-2.00803823967918,32.5424749218955));
#36505=CARTESIAN_POINT('Ctrl Pts',(4.7013594349753,0.273948980040725,32.6218468119489));
#36506=CARTESIAN_POINT('Ctrl Pts',(3.99771157397872,2.4892028345985,32.7012187020023));
#36507=CARTESIAN_POINT('Ctrl Pts',(2.32023002234538,4.09809238840509,32.7805905920557));
#36508=CARTESIAN_POINT('Ctrl Pts',(0.0775455730107522,4.70869570736983,
32.8599624821091));
#36509=CARTESIAN_POINT('Ctrl Pts',(-2.18402880626508,4.17227117454043,32.9393343721625));
#36510=CARTESIAN_POINT('Ctrl Pts',(-3.91357860260051,2.61949061875855,33.018706262216));
#36511=CARTESIAN_POINT('Ctrl Pts',(-4.68978931390171,0.42860794639128,33.0980781522693));
#36512=CARTESIAN_POINT('Ctrl Pts',(-4.32357772900909,-1.86668267300931,
33.1774500423228));
#36513=CARTESIAN_POINT('Ctrl Pts',(-2.90415217940683,-3.70725352509686,
33.2568219323761));
#36514=CARTESIAN_POINT('Ctrl Pts',(-0.777281587132916,-4.64474562433732,
33.3361938224295));
#36515=CARTESIAN_POINT('Ctrl Pts',(1.53893307928302,-4.45078797045929,33.4155657124829));
#36516=CARTESIAN_POINT('Ctrl Pts',(3.4802670539562,-3.17262821862943,33.4949376025364));
#36517=CARTESIAN_POINT('Ctrl Pts',(4.57381567772608,-1.12162325523486,33.5743094925897));
#36518=CARTESIAN_POINT('Ctrl Pts',(4.55319292637118,1.20260665046394,33.6536813826432));
#36519=CARTESIAN_POINT('Ctrl Pts',(3.42342245647383,3.23388423803441,33.7330532726965));
#36520=CARTESIAN_POINT('Ctrl Pts',(1.45971385379651,4.47739478330101,33.81242516275));
#36521=CARTESIAN_POINT('Ctrl Pts',(-0.859577812643769,4.63022186990074,
33.8917970528033));
#36522=CARTESIAN_POINT('Ctrl Pts',(-2.96947822656726,3.65513715781495,33.9711689428568));
#36523=CARTESIAN_POINT('Ctrl Pts',(-4.35602031732756,1.78966912459429,34.0505408329101));
#36524=CARTESIAN_POINT('Ctrl Pts',(-4.6814455006743,-0.511758346012144,
34.1299127229636));
#36525=CARTESIAN_POINT('Ctrl Pts',(-3.86648092226059,-2.68852261628789,
34.209284613017));
#36526=CARTESIAN_POINT('Ctrl Pts',(-2.1096501494946,-4.21036872817975,34.2886565030704));
#36527=CARTESIAN_POINT('Ctrl Pts',(0.161086730056863,-4.70657833738016,
34.3680283931238));
#36528=CARTESIAN_POINT('Ctrl Pts',(2.39258323872595,-4.05627588142921,34.4474002831772));
#36529=CARTESIAN_POINT('Ctrl Pts',(4.04125176633455,-2.41787359917646,34.5267721732306));
#36530=CARTESIAN_POINT('Ctrl Pts',(4.7054803088231,-0.190482660036747,34.606144063284));
#36531=CARTESIAN_POINT('Ctrl Pts',(4.22346426348634,2.08330943346165,34.6855159533374));
#36532=CARTESIAN_POINT('Ctrl Pts',(2.71262167204393,3.84961196029602,34.7648878433908));
#36533=CARTESIAN_POINT('Ctrl Pts',(0.540990445577805,4.67815753457386,34.8442597334442));
#36534=CARTESIAN_POINT('Ctrl Pts',(-1.76242485596904,4.36711428835555,34.9236316234976));
#36535=CARTESIAN_POINT('Ctrl Pts',(-3.63651736366306,2.99225166793732,35.0030035135511));
#36536=CARTESIAN_POINT('Ctrl Pts',(-4.62476229086341,0.888483164446288,
35.0823754036044));
#36537=CARTESIAN_POINT('Ctrl Pts',(-4.48642536074711,-1.43171787127975,
35.1617472936579));
#36538=CARTESIAN_POINT('Ctrl Pts',(-3.25520514328689,-3.40315560261577,
35.2411191837112));
#36539=CARTESIAN_POINT('Ctrl Pts',(-1.2310241581964,-4.54559216191174,35.3204910737646));
#36540=CARTESIAN_POINT('Ctrl Pts',(1.09303158700498,-4.58073253206361,35.399862963818));
#36541=CARTESIAN_POINT('Ctrl Pts',(3.15082725699632,-3.50001659668431,35.4792348538714));
#36542=CARTESIAN_POINT('Ctrl Pts',(4.44108838142123,-1.56670436550804,35.5586067439248));
#36543=CARTESIAN_POINT('Ctrl Pts',(4.64951020631433,0.748253581264717,35.6379786339782));
#36544=CARTESIAN_POINT('Ctrl Pts',(3.72532163646553,2.8809386118726,35.7173505240316));
#36545=CARTESIAN_POINT('Ctrl Pts',(1.89365296183327,4.31183337347777,35.7967224140851));
#36546=CARTESIAN_POINT('Ctrl Pts',(-0.399305382771815,4.69237506938502,
35.8760943041384));
#36547=CARTESIAN_POINT('Ctrl Pts',(-2.59499381998119,3.92986458478612,35.9554661941919));
#36548=CARTESIAN_POINT('Ctrl Pts',(-4.1585475065645,2.210047785941,36.0348380842453));
#36549=CARTESIAN_POINT('Ctrl Pts',(-4.70908822533747,-0.0481317617014899,
36.1142099742986));
#36550=CARTESIAN_POINT('Ctrl Pts',(-4.11250547580826,-2.29458651873135,
36.1935818643521));
#36551=CARTESIAN_POINT('Ctrl Pts',(-2.51412549524861,-3.98208507877941,
36.2729537544055));
#36552=CARTESIAN_POINT('Ctrl Pts',(-0.303310108968769,-4.6995565278326,
36.3523256444589));
#36553=CARTESIAN_POINT('Ctrl Pts',(1.98139094849032,-4.27222640899768,36.4316975345123));
#36554=CARTESIAN_POINT('Ctrl Pts',(3.7834295566316,-2.80419139334371,36.5110694245656));
#36555=CARTESIAN_POINT('Ctrl Pts',(4.66383309925673,-0.653061561243602,
36.5904413146191));
#36556=CARTESIAN_POINT('Ctrl Pts',(4.4081372221224,1.65715262164824,36.6698132046725));
#36557=CARTESIAN_POINT('Ctrl Pts',(3.07862887492527,3.56368809395169,36.7491850947259));
#36558=CARTESIAN_POINT('Ctrl Pts',(0.999173348225765,4.60211703465827,36.8285569847793));
#36559=CARTESIAN_POINT('Ctrl Pts',(-1.3236785944688,4.51948045233538,36.9079288748327));
#36560=CARTESIAN_POINT('Ctrl Pts',(-3.32408536146365,3.33590843552393,36.9873007648862));
#36561=CARTESIAN_POINT('Ctrl Pts',(-4.51475229214413,1.33971650772689,37.0666726549395));
#36562=CARTESIAN_POINT('Ctrl Pts',(-4.60563555769299,-0.982827395940232,
37.146044544993));
#36563=CARTESIAN_POINT('Ctrl Pts',(-3.57459619578919,-3.06595672140786,
37.2254164350463));
#36564=CARTESIAN_POINT('Ctrl Pts',(-1.67279311282567,-4.40222577592056,
37.3047883250997));
#36565=CARTESIAN_POINT('Ctrl Pts',(0.636498669757439,-4.6661223755806,37.3841602151531));
#36566=CARTESIAN_POINT('Ctrl Pts',(2.79074078525356,-3.79336189283575,37.4635321052066));
#36567=CARTESIAN_POINT('Ctrl Pts',(4.26516462266191,-1.9965468494605,37.5429039952599));
#36568=CARTESIAN_POINT('Ctrl Pts',(4.70060379877145,0.286622587162363,37.6222758853134));
#36569=CARTESIAN_POINT('Ctrl Pts',(3.99098629411051,2.49997139597979,37.7016477753667));
#36570=CARTESIAN_POINT('Ctrl Pts',(2.3091733621022,4.10433270633122,37.7810196654202));
#36571=CARTESIAN_POINT('Ctrl Pts',(0.0648509103550771,4.70888765420329,
37.8603915554735));
#36572=CARTESIAN_POINT('Ctrl Pts',(-2.19526907961097,4.16636799246395,37.9397634455269));
#36573=CARTESIAN_POINT('Ctrl Pts',(-3.92062638092667,2.60893030984724,38.0191353355804));
#36574=CARTESIAN_POINT('Ctrl Pts',(-4.69092777401319,0.415962978544177,
38.0985072256337));
#36575=CARTESIAN_POINT('Ctrl Pts',(-4.31852954453265,-1.87833201365752,
38.1778791156872));
#36576=CARTESIAN_POINT('Ctrl Pts',(-2.89414707692572,-3.71506948486711,
38.2572510057405));
#36577=CARTESIAN_POINT('Ctrl Pts',(-0.764756787430149,-4.64682425288566,
38.336622895794));
#36578=CARTESIAN_POINT('Ctrl Pts',(1.55092656265596,-4.44662291817819,38.4159947858474));
#36579=CARTESIAN_POINT('Ctrl Pts',(3.48880763512333,-3.16323408359078,38.4953666759007));
#36580=CARTESIAN_POINT('Ctrl Pts',(4.57682288978048,-1.10928842689192,38.5747385659542));
#36581=CARTESIAN_POINT('Ctrl Pts',(4.5499342195639,1.21487743324952,38.6541104560075));
#36582=CARTESIAN_POINT('Ctrl Pts',(3.41469164371823,3.24310184347568,38.733482346061));
#36583=CARTESIAN_POINT('Ctrl Pts',(1.44763774336306,4.48131381605587,38.8128542361143));
#36584=CARTESIAN_POINT('Ctrl Pts',(-0.872057510020701,4.62788767559439,
38.8922261261678));
#36585=CARTESIAN_POINT('Ctrl Pts',(-2.9793214784951,3.6471183158447,38.9715980162212));
#36586=CARTESIAN_POINT('Ctrl Pts',(-4.36082934025308,1.77791905463904,39.0509699062746));
#36587=CARTESIAN_POINT('Ctrl Pts',(-4.68004880681061,-0.524377442655287,
39.130341796328));
#36588=CARTESIAN_POINT('Ctrl Pts',(-3.85921878174905,-2.6989365861694,39.2097136863814));
#36589=CARTESIAN_POINT('Ctrl Pts',(-2.09829153079023,-4.21604107122303,
39.2890855764348));
#36590=CARTESIAN_POINT('Ctrl Pts',(0.173774754931348,-4.70612667927191,
39.3684574664882));
#36591=CARTESIAN_POINT('Ctrl Pts',(2.40351015490339,-4.04981138575493,39.4478293565416));
#36592=CARTESIAN_POINT('Ctrl Pts',(4.04775531046155,-2.40696884895629,39.527201246595));
#36593=CARTESIAN_POINT('Ctrl Pts',(4.70597715859854,-0.177798095133498,
39.6065731366484));
#36594=CARTESIAN_POINT('Ctrl Pts',(4.21783163769349,2.0946915601602,39.6859450267019));
#36595=CARTESIAN_POINT('Ctrl Pts',(2.70223496968604,3.85690448821556,39.7653169167552));
#36596=CARTESIAN_POINT('Ctrl Pts',(0.528373605920714,4.67961139929736,39.8446888068086));
#36597=CARTESIAN_POINT('Ctrl Pts',(-1.77418661813221,4.36232362711485,39.9240606968621));
#36598=CARTESIAN_POINT('Ctrl Pts',(-3.6445811625546,2.98248116081159,40.0034325869154));
#36599=CARTESIAN_POINT('Ctrl Pts',(-4.62712170766669,0.875927969712799,
40.0828044769689));
#36600=CARTESIAN_POINT('Ctrl Pts',(-4.48258575488106,-1.44364637546354,
40.1621763670223));
#36601=CARTESIAN_POINT('Ctrl Pts',(-3.24594541476057,-3.41224896374515,
40.2415482570757));
#36602=CARTESIAN_POINT('Ctrl Pts',(-1.89461073269764,-4.16947670058303,
40.2944628504446));
#36603=CARTESIAN_POINT('Ctrl Pts',(-1.16918346556913,-4.36383719750631,
40.3209201471291));
#36604=CARTESIAN_POINT('Ctrl Pts',(-3.57461543774205,3.05624720968391,-0.106973382376353));
#36605=CARTESIAN_POINT('Ctrl Pts',(-4.08267404777841,2.46201708819397,-0.0805160856918847));
#36606=CARTESIAN_POINT('Ctrl Pts',(-4.79625497710715,1.01593427979912,-0.027601492322949));
#36607=CARTESIAN_POINT('Ctrl Pts',(-4.69765387924802,-1.40219731261579,
0.051770397730455));
#36608=CARTESIAN_POINT('Ctrl Pts',(-3.45499130789169,-3.47806613859392,
0.131142287783858));
#36609=CARTESIAN_POINT('Ctrl Pts',(-1.37056128557091,-4.70703587006775,
0.210514177837262));
#36610=CARTESIAN_POINT('Ctrl Pts',(1.04766160592227,-4.78919858119765,0.289886067890666));
#36611=CARTESIAN_POINT('Ctrl Pts',(3.21071490770584,-3.70482006635648,0.36925795794407));
#36612=CARTESIAN_POINT('Ctrl Pts',(4.59162481050196,-1.71790426872487,0.448629847997472));
#36613=CARTESIAN_POINT('Ctrl Pts',(4.85403585089543,0.687462033087635,0.528001738050878));
#36614=CARTESIAN_POINT('Ctrl Pts',(3.93400879434301,2.92537849589629,0.607373628104279));
#36615=CARTESIAN_POINT('Ctrl Pts',(2.05566892616791,4.45067161106188,0.686745518157684));
#36616=CARTESIAN_POINT('Ctrl Pts',(-0.323428943211738,4.89179500940945,
0.766117408211087));
#36617=CARTESIAN_POINT('Ctrl Pts',(-2.62373939006112,4.1412858336604,0.845489298264492));
#36618=CARTESIAN_POINT('Ctrl Pts',(-4.28491317807112,2.38196972749854,0.924861188317894));
#36619=CARTESIAN_POINT('Ctrl Pts',(-4.90229136258891,0.042410468561284,
1.0042330783713));
#36620=CARTESIAN_POINT('Ctrl Pts',(-4.32548234816227,-2.30747956911558,
1.0836049684247));
#36621=CARTESIAN_POINT('Ctrl Pts',(-2.69499534131545,-4.09527285943935,
1.16297685847811));
#36622=CARTESIAN_POINT('Ctrl Pts',(-0.408013469920106,-4.88546665687605,
1.24234874853151));
#36623=CARTESIAN_POINT('Ctrl Pts',(1.97835959833349,-4.48557163766149,1.32172063858491));
#36624=CARTESIAN_POINT('Ctrl Pts',(3.8828086375498,-2.99300127117732,1.40109252863832));
#36625=CARTESIAN_POINT('Ctrl Pts',(4.84141409235741,-0.771342433159628,
1.48046441869172));
#36626=CARTESIAN_POINT('Ctrl Pts',(4.62066178777609,1.63821372124453,1.55983630874512));
#36627=CARTESIAN_POINT('Ctrl Pts',(3.27432650082566,3.64870463556752,1.63920819879853));
#36628=CARTESIAN_POINT('Ctrl Pts',(1.13037252509344,4.77037917890212,1.71858008885193));
#36629=CARTESIAN_POINT('Ctrl Pts',(-1.2889376953016,4.72999991227064,1.79795197890533));
#36630=CARTESIAN_POINT('Ctrl Pts',(-3.394265546355,3.53740313723842,1.87732386895874));
#36631=CARTESIAN_POINT('Ctrl Pts',(-4.67275782327988,1.48310278759205,1.95669575901214));
#36632=CARTESIAN_POINT('Ctrl Pts',(-4.81297663748911,-0.9324781181648,2.03606764906555));
#36633=CARTESIAN_POINT('Ctrl Pts',(-3.78076499611659,-3.12090941842389,
2.11543953911895));
#36634=CARTESIAN_POINT('Ctrl Pts',(-1.82756737028867,-4.54909409232738,
2.19481142917235));
#36635=CARTESIAN_POINT('Ctrl Pts',(0.57082162169894,-4.86912951461188,2.27418331922576));
#36636=CARTESIAN_POINT('Ctrl Pts',(2.8301597301281,-4.00305576476012,2.35355520927916));
#36637=CARTESIAN_POINT('Ctrl Pts',(4.40007719275289,-2.16184649123289,2.43292709933256));
#36638=CARTESIAN_POINT('Ctrl Pts',(4.89814559062742,0.205983802396055,2.51229898938597));
#36639=CARTESIAN_POINT('Ctrl Pts',(4.20303656448716,2.52363689769692,2.59167087943937));
#36640=CARTESIAN_POINT('Ctrl Pts',(2.48407713450111,4.22653763069529,2.67104276949277));
#36641=CARTESIAN_POINT('Ctrl Pts',(0.160002012962259,4.89986315213815,2.75041465954618));
#36642=CARTESIAN_POINT('Ctrl Pts',(-2.20304924477586,4.37959285538356,2.82978654959959));
#36643=CARTESIAN_POINT('Ctrl Pts',(-4.02944258285332,2.79246343312173,2.90915843965298));
#36644=CARTESIAN_POINT('Ctrl Pts',(-4.8742726267676,0.525096099564501,2.9885303297064));
#36645=CARTESIAN_POINT('Ctrl Pts',(-4.53174064782075,-1.87018348156618,
3.06790221975979));
#36646=CARTESIAN_POINT('Ctrl Pts',(-3.08528667790254,-3.80989050616825,
3.1472741098132));
#36647=CARTESIAN_POINT('Ctrl Pts',(-0.887263702413488,-4.82151663651732,
3.2266459998666));
#36648=CARTESIAN_POINT('Ctrl Pts',(1.52689474705858,-4.65863198645683,3.30601788992001));
#36649=CARTESIAN_POINT('Ctrl Pts',(3.56910501587138,-3.36091489620245,3.38538977997341));
#36650=CARTESIAN_POINT('Ctrl Pts',(4.74188920289787,-1.24448637649211,3.46476167002681));
#36651=CARTESIAN_POINT('Ctrl Pts',(4.75955967609216,1.17509626990786,3.54413356008022));
#36652=CARTESIAN_POINT('Ctrl Pts',(3.61781194729703,3.30842806598974,3.62350545013362));
#36653=CARTESIAN_POINT('Ctrl Pts',(1.59477323603129,4.63583410827783,3.70287734018703));
#36654=CARTESIAN_POINT('Ctrl Pts',(-0.816748705561003,4.83396122303419,
3.78224923024042));
#36655=CARTESIAN_POINT('Ctrl Pts',(-3.02931247032122,3.85454608365112,3.86162112029383));
#36656=CARTESIAN_POINT('Ctrl Pts',(-4.50394242258063,1.93617205018365,3.94099301034724));
#36657=CARTESIAN_POINT('Ctrl Pts',(-4.88142197000684,-0.453849209064403,
4.02036490040064));
#36658=CARTESIAN_POINT('Ctrl Pts',(-4.06979793038364,-2.73331380556256,
4.09973679045404));
#36659=CARTESIAN_POINT('Ctrl Pts',(-2.2667801232639,-4.34694920911316,4.17910868050745));
#36660=CARTESIAN_POINT('Ctrl Pts',(0.0884203044502142,-4.90167740713265,
4.25848057056085));
#36661=CARTESIAN_POINT('Ctrl Pts',(2.42208174171528,-4.26236783845356,4.33785246061425));
#36662=CARTESIAN_POINT('Ctrl Pts',(4.16572942788551,-2.58475489891836,4.41722435066765));
#36663=CARTESIAN_POINT('Ctrl Pts',(4.89461464610853,-0.277501387264568,
4.49659624072106));
#36664=CARTESIAN_POINT('Ctrl Pts',(4.43118257058524,2.09735084808797,4.57596813077446));
#36665=CARTESIAN_POINT('Ctrl Pts',(2.88832422912366,3.96129305925364,4.65534002082787));
#36666=CARTESIAN_POINT('Ctrl Pts',(0.641876498644775,4.86027304935857,4.73471191088126));
#36667=CARTESIAN_POINT('Ctrl Pts',(-1.76093092613442,4.57530128267169,4.81408380093468));
#36668=CARTESIAN_POINT('Ctrl Pts',(-3.73477947506178,3.17579625078358,4.89345569098808));
#36669=CARTESIAN_POINT('Ctrl Pts',(-4.79884401065823,1.00267428171038,4.97282758104148));
#36670=CARTESIAN_POINT('Ctrl Pts',(-4.6939207673194,-1.41469692300561,5.05219947109488));
#36671=CARTESIAN_POINT('Ctrl Pts',(-3.44556881487893,-3.48745108865595,
5.13157136114829));
#36672=CARTESIAN_POINT('Ctrl Pts',(-1.35788392577118,-4.71066988845176,
5.21094325120169));
#36673=CARTESIAN_POINT('Ctrl Pts',(1.06057848202937,-4.78637993031164,5.2903151412551));
#36674=CARTESIAN_POINT('Ctrl Pts',(3.22068631915819,-3.69613841561989,5.3696870313085));
#36675=CARTESIAN_POINT('Ctrl Pts',(4.59624209780833,-1.70552576414673,5.44905892136191));
#36676=CARTESIAN_POINT('Ctrl Pts',(4.85216347504167,0.700549188355308,5.52843081141531));
#36677=CARTESIAN_POINT('Ctrl Pts',(3.92610856983656,2.93597190921332,5.60780270146871));
#36678=CARTESIAN_POINT('Ctrl Pts',(2.04366230731317,4.45619837165057,5.68717459152211));
#36679=CARTESIAN_POINT('Ctrl Pts',(-0.336615569701915,4.89090477438153,
5.76654648157553));
#36680=CARTESIAN_POINT('Ctrl Pts',(-2.63489463902355,4.13419759990724,5.84591837162891));
#36681=CARTESIAN_POINT('Ctrl Pts',(-4.29131920651939,2.37040904098672,5.92529026168234));
#36682=CARTESIAN_POINT('Ctrl Pts',(-4.90238791398106,0.0291940864932555,
6.00466215173572));
#36683=CARTESIAN_POINT('Ctrl Pts',(-4.31924577684855,-2.31913248284995,
6.08403404178914));
#36684=CARTESIAN_POINT('Ctrl Pts',(-2.68394492896408,-4.1025235126836,6.16340593184253));
#36685=CARTESIAN_POINT('Ctrl Pts',(-0.394841037195299,-4.88654889560929,
6.24277782189594));
#36686=CARTESIAN_POINT('Ctrl Pts',(1.99044525726845,-4.48022178375707,6.32214971194934));
#36687=CARTESIAN_POINT('Ctrl Pts',(3.89086349283745,-2.98252256218433,6.40152160200274));
#36688=CARTESIAN_POINT('Ctrl Pts',(4.84347599383151,-0.758287446165202,
6.48089349205615));
#36689=CARTESIAN_POINT('Ctrl Pts',(4.61622846358046,1.65066481329898,6.56026538210956));
#36690=CARTESIAN_POINT('Ctrl Pts',(3.26447789744962,3.65751877792811,6.63963727216296));
#36691=CARTESIAN_POINT('Ctrl Pts',(1.11750774129931,4.77340926403445,6.71900916221636));
#36692=CARTESIAN_POINT('Ctrl Pts',(-1.30168482707007,4.7265078191842,6.79838105226977));
#36693=CARTESIAN_POINT('Ctrl Pts',(-3.4037898527957,3.52823953152828,6.87775294232317));
#36694=CARTESIAN_POINT('Ctrl Pts',(-4.67673920454132,1.4704999036178,6.95712483237657));
#36695=CARTESIAN_POINT('Ctrl Pts',(-4.81044523784733,-0.945450245917632,
7.03649672242998));
#36696=CARTESIAN_POINT('Ctrl Pts',(-3.77233745895366,-3.13109080826615,
7.11586861248337));
#36697=CARTESIAN_POINT('Ctrl Pts',(-1.81529662498623,-4.554004580273,7.19524050253679));
#36698=CARTESIAN_POINT('Ctrl Pts',(0.583946448736947,-4.8675729166435,7.27461239259018));
#36699=CARTESIAN_POINT('Ctrl Pts',(2.84094146009133,-3.99541126470955,7.3539842826436));
#36700=CARTESIAN_POINT('Ctrl Pts',(4.40588942008474,-2.14997627238517,7.433356172697));
#36701=CARTESIAN_POINT('Ctrl Pts',(4.8975724696163,0.219188181000477,7.51272806275039));
#36702=CARTESIAN_POINT('Ctrl Pts',(4.19621770614212,2.53495887865921,7.59209995280381));
#36703=CARTESIAN_POINT('Ctrl Pts',(2.47267359762208,4.23321920451286,7.6714718428572));
#36704=CARTESIAN_POINT('Ctrl Pts',(0.14679167389147,4.90027670221897,7.75084373291062));
#36705=CARTESIAN_POINT('Ctrl Pts',(-2.21484837668125,4.37363764184302,7.83021562296401));
#36706=CARTESIAN_POINT('Ctrl Pts',(-4.03695626517815,2.78159013279685,7.90958751301742));
#36707=CARTESIAN_POINT('Ctrl Pts',(-4.87567054312876,0.511953424346666,
7.98895940307082));
#36708=CARTESIAN_POINT('Ctrl Pts',(-4.52668226888691,-1.88239400508467,
8.06833129312423));
#36709=CARTESIAN_POINT('Ctrl Pts',(-3.07500421358545,-3.81819442148583,
8.14770318317762));
#36710=CARTESIAN_POINT('Ctrl Pts',(-0.874261938260974,-4.82389112824304,
8.22707507323104));
#36711=CARTESIAN_POINT('Ctrl Pts',(1.53944861007788,-4.65449863366217,8.30644696328443));
#36712=CARTESIAN_POINT('Ctrl Pts',(3.5781528845135,-3.35128057447919,8.38581885333784));
#36713=CARTESIAN_POINT('Ctrl Pts',(4.74522703638871,-1.23169798528678,8.46519074339124));
#36714=CARTESIAN_POINT('Ctrl Pts',(4.75637438558149,1.18792350680425,8.54456263344465));
#36715=CARTESIAN_POINT('Ctrl Pts',(3.60887946250276,3.31816946206181,8.62393452349805));
#36716=CARTESIAN_POINT('Ctrl Pts',(1.58226949047756,4.64011668100466,8.70330641355145));
#36717=CARTESIAN_POINT('Ctrl Pts',(-0.829777827133893,4.83174174717884,
8.78267830360486));
#36718=CARTESIAN_POINT('Ctrl Pts',(-3.03969310273758,3.84636521861918,8.86205019365827));
#36719=CARTESIAN_POINT('Ctrl Pts',(-4.50914586676094,1.9240226365889,8.94142208371166));
#36720=CARTESIAN_POINT('Ctrl Pts',(-4.88018067846642,-0.467007600962554,
9.02079397376508));
#36721=CARTESIAN_POINT('Ctrl Pts',(-4.0624142789942,-2.74427582062334,9.10016586381847));
#36722=CARTESIAN_POINT('Ctrl Pts',(-2.25505275316047,-4.35304452473175,
9.17953775387187));
#36723=CARTESIAN_POINT('Ctrl Pts',(0.101634631868527,-4.90142121791617,
9.25890964392528));
#36724=CARTESIAN_POINT('Ctrl Pts',(2.4335640455388,-4.25582255152803,9.33828153397868));
#36725=CARTESIAN_POINT('Ctrl Pts',(4.17268264431847,-2.57351493169112,9.41765342403209));
#36726=CARTESIAN_POINT('Ctrl Pts',(4.89534498701854,-0.264304770872935,
9.49702531408549));
#36727=CARTESIAN_POINT('Ctrl Pts',(4.42551212654324,2.10928944710123,9.57639720413889));
#36728=CARTESIAN_POINT('Ctrl Pts',(2.8776343077469,3.96906542459454,9.65576909419229));
#36729=CARTESIAN_POINT('Ctrl Pts',(0.628771141118955,4.86198585003388,9.73514098424571));
#36730=CARTESIAN_POINT('Ctrl Pts',(-1.77325928372426,4.57053728422814,9.81451287429909));
#36731=CARTESIAN_POINT('Ctrl Pts',(-3.74332767209512,3.16571595269709,9.89388476435253));
#36732=CARTESIAN_POINT('Ctrl Pts',(-4.80152972525885,0.989733222282404,
9.97325665440589));
#36733=CARTESIAN_POINT('Ctrl Pts',(-4.69008976535528,-1.42734633034291,
10.0526285444593));
#36734=CARTESIAN_POINT('Ctrl Pts',(-3.43615431994881,-3.49672747627419,
10.1320004345127));
#36735=CARTESIAN_POINT('Ctrl Pts',(-1.34517928800141,-4.71431354886008,
10.2113723245661));
#36736=CARTESIAN_POINT('Ctrl Pts',(1.07347844099931,-4.78350327589974,10.2907442146195));
#36737=CARTESIAN_POINT('Ctrl Pts',(3.23063919787684,-3.68744219303511,10.3701161046729));
#36738=CARTESIAN_POINT('Ctrl Pts',(4.60082339705013,-1.69312835396196,10.4494879947263));
#36739=CARTESIAN_POINT('Ctrl Pts',(4.85025720045185,0.713627804460256,10.5288598847798));
#36740=CARTESIAN_POINT('Ctrl Pts',(3.91817908568572,2.94654580930431,10.6082317748331));
#36741=CARTESIAN_POINT('Ctrl Pts',(2.03164121838884,4.46169177707037,10.6876036648866));
#36742=CARTESIAN_POINT('Ctrl Pts',(-0.349799952746016,4.8899795037293,10.7669755549399));
#36743=CARTESIAN_POINT('Ctrl Pts',(-2.64603062966098,4.12707904706582,10.8463474449934));
#36744=CARTESIAN_POINT('Ctrl Pts',(-4.29769410207999,2.35883126967163,10.9257193350467));
#36745=CARTESIAN_POINT('Ctrl Pts',(-4.90244880401686,0.0159774161698882,
11.0050912251002));
#36746=CARTESIAN_POINT('Ctrl Pts',(-4.31297782868159,-2.33076850054543,
11.0844631151536));
#36747=CARTESIAN_POINT('Ctrl Pts',(-2.672875000894,-4.10974436959645,11.163835005207));
#36748=CARTESIAN_POINT('Ctrl Pts',(-0.381665739197088,-4.88759560697865,
11.2432068952604));
#36749=CARTESIAN_POINT('Ctrl Pts',(2.00251645176545,-4.47483937301022,11.3225787853138));
#36750=CARTESIAN_POINT('Ctrl Pts',(3.89889006757291,-2.97202217266546,11.4019506753672));
#36751=CARTESIAN_POINT('Ctrl Pts',(4.84550269296641,-0.745226949518873,
11.4813225654206));
#36752=CARTESIAN_POINT('Ctrl Pts',(4.61176158769154,1.66310390899864,11.560694455474));
#36753=CARTESIAN_POINT('Ctrl Pts',(3.25460556761616,3.66630633650213,11.6400663455274));
#36754=CARTESIAN_POINT('Ctrl Pts',(1.10463483521672,4.77640465566513,11.7194382355808));
#36755=CARTESIAN_POINT('Ctrl Pts',(-1.3144224979738,4.72298137310049,11.7988101256342));
#36756=CARTESIAN_POINT('Ctrl Pts',(-3.41328942008276,3.51905028219049,11.8781820156876));
#36757=CARTESIAN_POINT('Ctrl Pts',(-4.6806865946475,1.45788633182458,11.957553905741));
#36758=CARTESIAN_POINT('Ctrl Pts',(-4.80787887528018,-0.95841550199713,
12.0369257957944));
#36759=CARTESIAN_POINT('Ctrl Pts',(-3.76388250395398,-3.14124944094907,
12.1162976858478));
#36760=CARTESIAN_POINT('Ctrl Pts',(-1.80301268587722,-4.55888196912352,
12.1956695759012));
#36761=CARTESIAN_POINT('Ctrl Pts',(0.59706703157835,-4.86598094053357,12.2750414659546));
#36762=CARTESIAN_POINT('Ctrl Pts',(2.8517025417269,-3.98773772549578,12.354413356008));
#36763=CARTESIAN_POINT('Ctrl Pts',(4.41166962484727,-2.13809042723494,12.4337852460614));
#36764=CARTESIAN_POINT('Ctrl Pts',(4.89696375241996,0.232390966517433,12.5131571361148));
#36765=CARTESIAN_POINT('Ctrl Pts',(4.18936834914853,2.54626243521486,12.5925290261683));
#36766=CARTESIAN_POINT('Ctrl Pts',(2.46125208903407,4.23987001075024,12.6719009162216));
#36767=CARTESIAN_POINT('Ctrl Pts',(0.133580267920011,4.90065463645993,12.751272806275));
#36768=CARTESIAN_POINT('Ctrl Pts',(-2.22663141078444,4.36765064014303,12.8306446963284));
#36769=CARTESIAN_POINT('Ctrl Pts',(-4.04444060638688,2.770696615518,12.9100165863818));
#36770=CARTESIAN_POINT('Ctrl Pts',(-4.87703302249085,0.498807028185692,
12.9893884764353));
#36771=CARTESIAN_POINT('Ctrl Pts',(-4.52159098944558,-1.89459084712199,
13.0687603664886));
#36772=CARTESIAN_POINT('Ctrl Pts',(-3.06469939974324,-3.82647058567648,
13.1481322565421));
#36773=CARTESIAN_POINT('Ctrl Pts',(-0.861253819860521,-4.82623055930914,
13.2275041465954));
#36774=CARTESIAN_POINT('Ctrl Pts',(1.55199128418723,-4.65033145137426,13.3068760366489));
#36775=CARTESIAN_POINT('Ctrl Pts',(3.58717474668141,-3.34162189521869,13.3862479267023));
#36776=CARTESIAN_POINT('Ctrl Pts',(4.74853038096063,-1.21890064194246,13.4656198167557));
#36777=CARTESIAN_POINT('Ctrl Pts',(4.75315452513156,1.20074210972015,13.5449917068091));
#36778=CARTESIAN_POINT('Ctrl Pts',(3.59992074790953,3.32788674125251,13.6243635968625));
#36779=CARTESIAN_POINT('Ctrl Pts',(1.56975424478615,4.64436552876813,13.7037354869159));
#36780=CARTESIAN_POINT('Ctrl Pts',(-0.842800917775063,4.82948715360455,
13.7831073769693));
#36781=CARTESIAN_POINT('Ctrl Pts',(-3.05005164227443,3.83815639771137,13.8624792670227));
#36782=CARTESIAN_POINT('Ctrl Pts',(-4.51431653789056,1.91185923895083,13.9418511570761));
#36783=CARTESIAN_POINT('Ctrl Pts',(-4.87890391714672,-0.480162598589543,
14.0212230471295));
#36784=CARTESIAN_POINT('Ctrl Pts',(-4.05500110145656,-2.75521788993537,
14.1005949371829));
#36785=CARTESIAN_POINT('Ctrl Pts',(-2.24330899304429,-4.35910820186428,
14.1799668272363));
#36786=CARTESIAN_POINT('Ctrl Pts',(0.114848220593315,-4.90112940454139,
14.2593387172897));
#36787=CARTESIAN_POINT('Ctrl Pts',(2.4450286619066,-4.2492463327382,14.3387106073431));
#36788=CARTESIAN_POINT('Ctrl Pts',(4.17960553315863,-2.56225625982719,14.4180824973965));
#36789=CARTESIAN_POINT('Ctrl Pts',(4.89603974793314,-0.2511062334803,14.4974543874499));
#36790=CARTESIAN_POINT('Ctrl Pts',(4.41980951731128,2.12121271552818,14.5768262775033));
#36791=CARTESIAN_POINT('Ctrl Pts',(2.86692347135483,3.97680894225867,14.6561981675567));
#36792=CARTESIAN_POINT('Ctrl Pts',(0.615661213603817,4.86366331317225,14.7355700576101));
#36793=CARTESIAN_POINT('Ctrl Pts',(-1.78557475303814,4.56574006653321,14.8149419476636));
#36794=CARTESIAN_POINT('Ctrl Pts',(-3.75184866214265,3.15561264578087,14.8943138377169));
#36795=CARTESIAN_POINT('Ctrl Pts',(-4.80418054172537,0.976784969346447,
14.9736857277704));
#36796=CARTESIAN_POINT('Ctrl Pts',(-4.68622467521704,-1.43998536354391,
15.0530576178237));
#36797=CARTESIAN_POINT('Ctrl Pts',(-3.42671485060823,-3.50597844922854,
15.1324295078772));
#36798=CARTESIAN_POINT('Ctrl Pts',(-1.33246487329588,-4.71792294503274,
15.2118013979305));
#36799=CARTESIAN_POINT('Ctrl Pts',(1.08637059779033,-4.78059185437226,15.291173287984));
#36800=CARTESIAN_POINT('Ctrl Pts',(3.24056859589536,-3.67871916964732,15.3705451780373));
#36801=CARTESIAN_POINT('Ctrl Pts',(4.60537125691718,-1.68071863790306,15.4499170680908));
#36802=CARTESIAN_POINT('Ctrl Pts',(4.84831567357043,0.726701233826767,15.5292889581442));
#36803=CARTESIAN_POINT('Ctrl Pts',(3.91022112370653,2.95709829352236,15.6086608481976));
#36804=CARTESIAN_POINT('Ctrl Pts',(2.01960536323555,4.46715275434186,15.688032738251));
#36805=CARTESIAN_POINT('Ctrl Pts',(-0.362981793399331,4.88901869207872,
15.7674046283044));
#36806=CARTESIAN_POINT('Ctrl Pts',(-2.65714738860797,4.11993049808428,15.8467765183578));
#36807=CARTESIAN_POINT('Ctrl Pts',(-4.3040377614491,2.34723635406844,15.9261484084112));
#36808=CARTESIAN_POINT('Ctrl Pts',(-4.90247406242457,0.00276062972017743,
16.0055202984646));
#36809=CARTESIAN_POINT('Ctrl Pts',(-4.30667853324066,-2.34238757791569,
16.084892188518));
#36810=CARTESIAN_POINT('Ctrl Pts',(-2.66178564602119,-4.11693535636137,
16.1642640785714));
#36811=CARTESIAN_POINT('Ctrl Pts',(-0.368487667211246,-4.88860679467341,
16.2436359686248));
#36812=CARTESIAN_POINT('Ctrl Pts',(2.01457309173119,-4.46942443856166,16.3230078586782));
#36813=CARTESIAN_POINT('Ctrl Pts',(3.90688830464663,-2.96150018209857,16.4023797487316));
#36814=CARTESIAN_POINT('Ctrl Pts',(4.84749417442,-0.732161036485258,16.481751638785));
#36815=CARTESIAN_POINT('Ctrl Pts',(4.60726119282582,1.67553091707946,16.5611235288384));
#36816=CARTESIAN_POINT('Ctrl Pts',(3.24470958308425,3.67506724782763,16.6404954188918));
#36817=CARTESIAN_POINT('Ctrl Pts',(1.09175390014313,4.77936533189424,16.7198673089452));
#36818=CARTESIAN_POINT('Ctrl Pts',(-1.32715061480029,4.7194205995551,16.7992391989986));
#36819=CARTESIAN_POINT('Ctrl Pts',(-3.42276418043948,3.50983545637255,16.878611089052));
#36820=CARTESIAN_POINT('Ctrl Pts',(-4.68459996247752,1.44526216311684,16.9579829791054));
#36821=CARTESIAN_POINT('Ctrl Pts',(-4.80527757305004,-0.971373790661056,
17.0373548691589));
#36822=CARTESIAN_POINT('Ctrl Pts',(-3.75540018385452,-3.15138524551466,
17.1167267592122));
#36823=CARTESIAN_POINT('Ctrl Pts',(-1.79071565870356,-4.56372621798453,
17.1960986492656));
#36824=CARTESIAN_POINT('Ctrl Pts',(0.610183305945333,-4.86435360814148,
17.275470539319));
#36825=CARTESIAN_POINT('Ctrl Pts',(2.86244283812717,-3.98003518345987,17.3548424293725));
#36826=CARTESIAN_POINT('Ctrl Pts',(4.41741787585788,-2.1261890788619,17.4342143194258));
#36827=CARTESIAN_POINT('Ctrl Pts',(4.89631923419534,0.245592132270697,17.5135862094793));
#36828=CARTESIAN_POINT('Ctrl Pts',(4.1824889384277,2.55754735438707,17.5929580995327));
#36829=CARTESIAN_POINT('Ctrl Pts',(2.44981194564648,4.24649024808584,17.6723299895861));
#36830=CARTESIAN_POINT('Ctrl Pts',(0.120369299865439,4.90099648569508,17.7517018796395));
#36831=CARTESIAN_POINT('Ctrl Pts',(-2.2384009215371,4.36163277449207,17.8310737696929));
#36832=CARTESIAN_POINT('Ctrl Pts',(-4.0518905292873,2.75978129753081,17.9104456597463));
#36833=CARTESIAN_POINT('Ctrl Pts',(-4.87836953900975,0.485660146581001,
17.9898175497997));
#36834=CARTESIAN_POINT('Ctrl Pts',(-4.51644893866981,-1.90677984789346,
18.0691894398531));
#36835=CARTESIAN_POINT('Ctrl Pts',(-3.05440612489714,-3.83470774368921,
18.1485613299065));
#36836=CARTESIAN_POINT('Ctrl Pts',(-0.848175594775907,-4.82855605094715,
18.2279332199599));
#36837=CARTESIAN_POINT('Ctrl Pts',(1.56440212229575,-4.64609055668262,18.3073051100133));
#36838=CARTESIAN_POINT('Ctrl Pts',(3.59639816964341,-3.33201429213606,18.3866770000667));
#36839=CARTESIAN_POINT('Ctrl Pts',(4.75136940590255,-1.20595214372204,18.4660488901201));
#36840=CARTESIAN_POINT('Ctrl Pts',(4.75071159562135,1.21328335035095,18.5454207801735));
#36841=CARTESIAN_POINT('Ctrl Pts',(3.58940432897552,3.33808667681415,18.6247926702269));
#36842=CARTESIAN_POINT('Ctrl Pts',(1.56011376732896,4.64762681676405,18.7041645602803));
#36843=CARTESIAN_POINT('Ctrl Pts',(-0.861221142909775,4.82897211168874,
18.7835364503337));
#36844=CARTESIAN_POINT('Ctrl Pts',(-3.05056344532316,3.82678328180746,18.8629083403871));
#36845=CARTESIAN_POINT('Ctrl Pts',(-5.02992785007326,1.26296632184503,18.968737527125));
#36846=CARTESIAN_POINT('Ctrl Pts',(-4.59246965375637,-3.13076985705441,
19.1010240105473));
#36847=CARTESIAN_POINT('Ctrl Pts',(0.146932230206506,-5.55932874556365,
19.2597677906541));
#36848=CARTESIAN_POINT('Ctrl Pts',(4.74574684718979,-2.89085235699285,19.418511570761));
#36849=CARTESIAN_POINT('Ctrl Pts',(5.00517315099097,2.41778366488237,19.5772553508677));
#36850=CARTESIAN_POINT('Ctrl Pts',(0.682914143844855,5.5166676123404,19.7359991309746));
#36851=CARTESIAN_POINT('Ctrl Pts',(-4.26335305224441,3.56621538027044,19.8947429110814));
#36852=CARTESIAN_POINT('Ctrl Pts',(-5.30889903625343,-1.64699798333531,
20.0534866911882));
#36853=CARTESIAN_POINT('Ctrl Pts',(-1.49629817009909,-5.35305176256659,
20.212230471295));
#36854=CARTESIAN_POINT('Ctrl Pts',(3.68539651252336,-4.16147159288513,20.3709742514018));
#36855=CARTESIAN_POINT('Ctrl Pts',(5.49476366156206,0.839647798276105,20.5297180315086));
#36856=CARTESIAN_POINT('Ctrl Pts',(2.27623920304293,5.06930720888698,20.6884618116154));
#36857=CARTESIAN_POINT('Ctrl Pts',(-3.02540872545025,4.66632909528393,20.8472055917223));
#36858=CARTESIAN_POINT('Ctrl Pts',(-5.55807194231375,-0.0182675279713449,
21.005949371829));
#36859=CARTESIAN_POINT('Ctrl Pts',(-3.4318929716806,-3.88810606053727,21.1382358552514));
#36860=CARTESIAN_POINT('Ctrl Pts',(-0.348982623888803,-4.88143613581972,
21.2440650419892));
#36861=CARTESIAN_POINT('Ctrl Pts',(2.02316502874914,-4.46849826887164,21.3234369320426));
#36862=CARTESIAN_POINT('Ctrl Pts',(3.91669769333085,-2.94853678524969,21.4028088220961));
#36863=CARTESIAN_POINT('Ctrl Pts',(4.84847467696001,-0.720374489880037,
21.4821807121494));
#36864=CARTESIAN_POINT('Ctrl Pts',(4.60324425657816,1.68862650319429,21.5615526022029));
#36865=CARTESIAN_POINT('Ctrl Pts',(3.23451621663553,3.68344087079137,21.6409244922562));
#36866=CARTESIAN_POINT('Ctrl Pts',(1.07901003836815,4.78248223987442,21.7202963823097));
#36867=CARTESIAN_POINT('Ctrl Pts',(-1.33994588402651,4.71572438645636,21.7996682723631));
#36868=CARTESIAN_POINT('Ctrl Pts',(-3.4321733891171,3.50064868327975,21.8790401624164));
#36869=CARTESIAN_POINT('Ctrl Pts',(-4.68850082698247,1.43259912421573,21.9584120524699));
#36870=CARTESIAN_POINT('Ctrl Pts',(-4.80262992851033,-0.984309998791622,
22.0377839425233));
#36871=CARTESIAN_POINT('Ctrl Pts',(-3.74689662802585,-3.16150609615164,
22.1171558325767));
#36872=CARTESIAN_POINT('Ctrl Pts',(-1.77840238381691,-4.56853309419591,
22.1965277226301));
#36873=CARTESIAN_POINT('Ctrl Pts',(0.62329338871143,-4.86269313206684,22.2758996126835));
#36874=CARTESIAN_POINT('Ctrl Pts',(2.87316334475109,-3.97230257099384,22.3552715027369));
#36875=CARTESIAN_POINT('Ctrl Pts',(4.4231333235665,-2.11427282962158,22.4346433927903));
#36876=CARTESIAN_POINT('Ctrl Pts',(4.89563979914059,0.258791705958885,22.5140152828437));
#36877=CARTESIAN_POINT('Ctrl Pts',(4.17557820525643,2.56881377105699,22.5933871728971));
#36878=CARTESIAN_POINT('Ctrl Pts',(2.43835555951363,4.25307922033076,22.6727590629505));
#36879=CARTESIAN_POINT('Ctrl Pts',(0.107154601980389,4.90130359745224,22.7521309530039));
#36880=CARTESIAN_POINT('Ctrl Pts',(-2.25014882333759,4.35558147263095,22.8315028430573));
#36881=CARTESIAN_POINT('Ctrl Pts',(-4.05932105856842,2.74884923313531,22.9108747331107));
#36882=CARTESIAN_POINT('Ctrl Pts',(-4.87965162531074,0.472503462573818,
22.9902466231641));
#36883=CARTESIAN_POINT('Ctrl Pts',(-4.51130988023697,-1.91894313613435,
23.0696185132175));
#36884=CARTESIAN_POINT('Ctrl Pts',(-3.04402302167418,-3.84293941821872,
23.1489904032709));
#36885=CARTESIAN_POINT('Ctrl Pts',(-0.835218899364871,-4.83080417279082,
23.2283622933243));
#36886=CARTESIAN_POINT('Ctrl Pts',(1.57704270154782,-4.64189571913938,23.3077341833777));
#36887=CARTESIAN_POINT('Ctrl Pts',(3.60514018926443,-3.32223174536946,23.3871060734312));
#36888=CARTESIAN_POINT('Ctrl Pts',(4.75503350768461,-1.19327947079072,23.4664779634845));
#36889=CARTESIAN_POINT('Ctrl Pts',(4.74661118820946,1.22635304091963,23.545849853538));
#36890=CARTESIAN_POINT('Ctrl Pts',(3.58192489000304,3.34724866670522,23.6252217435913));
#36891=CARTESIAN_POINT('Ctrl Pts',(1.54468961690465,4.65276192610169,23.7045936336447));
#36892=CARTESIAN_POINT('Ctrl Pts',(-0.868828627683255,4.82487267911367,
23.7839655236982));
#36893=CARTESIAN_POINT('Ctrl Pts',(-3.0707021417273,3.8216551271151,23.8633374137516));
#36894=CARTESIAN_POINT('Ctrl Pts',(-4.52455941090918,1.88749084526948,23.9427093038049));
#36895=CARTESIAN_POINT('Ctrl Pts',(-4.8762440225472,-0.506462028608541,
24.0220811938584));
#36896=CARTESIAN_POINT('Ctrl Pts',(-4.04008638366986,-2.77704187334428,
24.1014530839117));
#36897=CARTESIAN_POINT('Ctrl Pts',(-2.21977264431323,-4.37114046461548,
24.1808249739652));
#36898=CARTESIAN_POINT('Ctrl Pts',(0.141272797816377,-4.90043891405946,
24.2601968640185));
#36899=CARTESIAN_POINT('Ctrl Pts',(2.46790449909909,-4.23600129097727,24.339568754072));
#36900=CARTESIAN_POINT('Ctrl Pts',(4.19336012701565,-2.53968312964219,24.4189406441254));
#36901=CARTESIAN_POINT('Ctrl Pts',(4.89732250983615,-0.224703779419903,
24.4983125341788));
#36902=CARTESIAN_POINT('Ctrl Pts',(4.40830796930024,2.14501291409586,24.5776844242322));
#36903=CARTESIAN_POINT('Ctrl Pts',(2.84543936506689,3.99220920964338,24.6570563142856));
#36904=CARTESIAN_POINT('Ctrl Pts',(0.589428029776467,4.86691217832701,24.736428204339));
#36905=CARTESIAN_POINT('Ctrl Pts',(-1.8101666688907,4.5560461130975,24.8158000943924));
#36906=CARTESIAN_POINT('Ctrl Pts',(-3.76880877375201,3.13533729935451,24.8951719844458));
#36907=CARTESIAN_POINT('Ctrl Pts',(-4.80937740344408,0.950867259440163,
24.9745438744992));
#36908=CARTESIAN_POINT('Ctrl Pts',(-4.67839234303351,-1.46523194016486,
25.0539157645526));
#36909=CARTESIAN_POINT('Ctrl Pts',(-3.40776126330575,-3.52440388238162,
25.133287654606));
#36910=CARTESIAN_POINT('Ctrl Pts',(-1.30700708278832,-4.72503883998586,
25.2126595446594));
#36911=CARTESIAN_POINT('Ctrl Pts',(1.11213113008524,-4.77466479486562,25.2920314347128));
#36912=CARTESIAN_POINT('Ctrl Pts',(3.26035666133054,-3.66119297425736,25.3714033247662));
#36913=CARTESIAN_POINT('Ctrl Pts',(4.61436652655277,-1.65586264903317,25.4507752148196));
#36914=CARTESIAN_POINT('Ctrl Pts',(4.84432691963378,0.752832152305638,25.530147104873));
#36915=CARTESIAN_POINT('Ctrl Pts',(3.89421999782782,2.97813870770851,25.6095189949265));
#36916=CARTESIAN_POINT('Ctrl Pts',(1.99548970426076,4.47797726591181,25.6888908849798));
#36917=CARTESIAN_POINT('Ctrl Pts',(-0.389337464322654,4.88699047397359,
25.7682627750333));
#36918=CARTESIAN_POINT('Ctrl Pts',(-2.67932288838098,4.10554361974534,25.8476346650867));
#36919=CARTESIAN_POINT('Ctrl Pts',(-4.31663118741032,2.32399542721376,25.92700655514));
#36920=CARTESIAN_POINT('Ctrl Pts',(-4.90241768388754,-0.0236729073104641,
26.0063784451935));
#36921=CARTESIAN_POINT('Ctrl Pts',(-4.29398608388724,-2.36557457401295,
26.0857503352468));
#36922=CARTESIAN_POINT('Ctrl Pts',(-2.63954897842897,-4.13122751059639,
26.1651222253003));
#36923=CARTESIAN_POINT('Ctrl Pts',(-0.342123584367958,-4.89052256991551,
26.2444941153537));
#36924=CARTESIAN_POINT('Ctrl Pts',(2.03864235756733,-4.45849715619131,26.323866005407));
#36925=CARTESIAN_POINT('Ctrl Pts',(3.92279953365755,-2.94039170393502,26.4032378954605));
#36926=CARTESIAN_POINT('Ctrl Pts',(4.85137142631832,-0.706013341046749,
26.4826097855139));
#36927=CARTESIAN_POINT('Ctrl Pts',(4.59815997785643,1.70034830898648,26.5619816755673));
#36928=CARTESIAN_POINT('Ctrl Pts',(3.22484693664317,3.69250887460774,26.6413535656207));
#36929=CARTESIAN_POINT('Ctrl Pts',(1.06596831974129,4.78518245160429,26.7207254556741));
#36930=CARTESIAN_POINT('Ctrl Pts',(-1.3525778203687,4.71219617521178,26.8000973457275));
#36931=CARTESIAN_POINT('Ctrl Pts',(-3.44163899731715,3.49132934080697,26.8794692357809));
#36932=CARTESIAN_POINT('Ctrl Pts',(-4.69232453245783,1.419982406908,26.9588411258343));
#36933=CARTESIAN_POINT('Ctrl Pts',(-4.79997019777595,-0.997269098236029,
27.0382130158877));
#36934=CARTESIAN_POINT('Ctrl Pts',(-3.73835374746968,-3.17158805846741,
27.1175849059411));
#36935=CARTESIAN_POINT('Ctrl Pts',(-1.7660825989855,-4.57331518784726,27.1969567959945));
#36936=CARTESIAN_POINT('Ctrl Pts',(0.636402361454069,-4.860992860329,27.2763286860479));
#36937=CARTESIAN_POINT('Ctrl Pts',(2.88386111529617,-3.96454343165977,27.3557005761013));
#36938=CARTESIAN_POINT('Ctrl Pts',(4.42881768477039,-2.10233999840624,27.4350724661547));
#36939=CARTESIAN_POINT('Ctrl Pts',(4.89492406925623,0.271988805008393,27.5144443562081));
#36940=CARTESIAN_POINT('Ctrl Pts',(4.16863778520187,2.58006173756,27.5938162462615));
#36941=CARTESIAN_POINT('Ctrl Pts',(2.42688056379555,4.25963734171175,27.673188136315));
#36942=CARTESIAN_POINT('Ctrl Pts',(0.0939406088576867,4.90157471796985,
27.7525600263683));
#36943=CARTESIAN_POINT('Ctrl Pts',(-2.2618830704639,4.34949934238213,27.8319319164218));
#36944=CARTESIAN_POINT('Ctrl Pts',(-4.06671704041374,2.73789555444364,27.9113038064751));
#36945=CARTESIAN_POINT('Ctrl Pts',(-4.88090774084432,0.45934646967172,27.9906756965286));
#36946=CARTESIAN_POINT('Ctrl Pts',(-4.50612011931125,-1.93109839836612,
28.0700475865819));
#36947=CARTESIAN_POINT('Ctrl Pts',(-3.03365161084166,-3.85113197097576,
28.1494194766353));
#36948=CARTESIAN_POINT('Ctrl Pts',(-0.822192284844965,-4.83303831979172,
28.2287913666888));
#36949=CARTESIAN_POINT('Ctrl Pts',(1.5895512618482,-4.63762723165528,28.3081632567421));
#36950=CARTESIAN_POINT('Ctrl Pts',(3.61408363956719,-3.31250041510136,28.3875351467956));
#36951=CARTESIAN_POINT('Ctrl Pts',(4.75823324232603,-1.18045582952402,28.4669070368489));
#36952=CARTESIAN_POINT('Ctrl Pts',(4.7432877594249,1.23914518323065,28.5462789269024));
#36953=CARTESIAN_POINT('Ctrl Pts',(3.57288787741725,3.35689317215169,28.6256508169558));
#36954=CARTESIAN_POINT('Ctrl Pts',(1.53214041692396,4.65690941469359,28.7050227070092));
#36955=CARTESIAN_POINT('Ctrl Pts',(-0.881833057796704,4.82251283171032,
28.7843945970626));
#36956=CARTESIAN_POINT('Ctrl Pts',(-3.08099395154251,3.81336279737351,28.863766487116));
#36957=CARTESIAN_POINT('Ctrl Pts',(-4.52963153835698,1.87528602633188,28.9431383771694));
#36958=CARTESIAN_POINT('Ctrl Pts',(-4.87486090859702,-0.519606269848997,
29.0225102672228));
#36959=CARTESIAN_POINT('Ctrl Pts',(-4.03258495182442,-2.78792362882362,
29.1018821572762));
#36960=CARTESIAN_POINT('Ctrl Pts',(-2.20798022676276,-4.37710896278109,
29.1812540473296));
#36961=CARTESIAN_POINT('Ctrl Pts',(0.154483594256982,-4.90004024197141,
29.260625937383));
#36962=CARTESIAN_POINT('Ctrl Pts',(2.47931555365931,-4.22933256427261,29.3399978274364));
#36963=CARTESIAN_POINT('Ctrl Pts',(4.20019173206215,-2.52836883538588,29.4193697174898));
#36964=CARTESIAN_POINT('Ctrl Pts',(4.89791050150138,-0.211500054648609,
29.4987416075432));
#36965=CARTESIAN_POINT('Ctrl Pts',(4.40250911411586,2.15688967125365,29.5781134975966));
#36966=CARTESIAN_POINT('Ctrl Pts',(2.83466625132033,3.9998658474328,29.65748538765));
#36967=CARTESIAN_POINT('Ctrl Pts',(0.576304964130538,4.86848355673019,29.7368572777034));
#36968=CARTESIAN_POINT('Ctrl Pts',(-1.82244293669206,4.55114944781371,29.8162291677568));
#36969=CARTESIAN_POINT('Ctrl Pts',(-3.77724777204552,3.12516540720823,29.8956010578102));
#36970=CARTESIAN_POINT('Ctrl Pts',(-4.81192341092482,0.937897990843109,
29.9749729478637));
#36971=CARTESIAN_POINT('Ctrl Pts',(-4.67442515791461,-1.47783930008941,
30.0543448379171));
#36972=CARTESIAN_POINT('Ctrl Pts',(-3.39824728310101,-3.5335782086619,30.1337167279704));
#36973=CARTESIAN_POINT('Ctrl Pts',(-1.29426389201682,-4.7285452870471,30.2130886180239));
#36974=CARTESIAN_POINT('Ctrl Pts',(1.12499931835819,-4.77164919996508,30.2924605080772));
#36975=CARTESIAN_POINT('Ctrl Pts',(3.27021518492489,-3.65238992963792,30.3718323981307));
#36976=CARTESIAN_POINT('Ctrl Pts',(4.61881387094242,-1.64341655687892,30.451204288184));
#36977=CARTESIAN_POINT('Ctrl Pts',(4.84227972156944,0.765889451494932,30.5305761782375));
#36978=CARTESIAN_POINT('Ctrl Pts',(3.88617695022651,2.98862648475217,30.6099480682908));
#36979=CARTESIAN_POINT('Ctrl Pts',(1.98341007571514,4.48334072153628,30.6893199583443));
#36980=CARTESIAN_POINT('Ctrl Pts',(-0.40251110303664,4.8859230822605,30.7686918483976));
#36981=CARTESIAN_POINT('Ctrl Pts',(-2.69038146803192,4.09830539495341,30.8480637384511));
#36982=CARTESIAN_POINT('Ctrl Pts',(-4.322880862473,2.3123495848808,30.9274356285044));
#36983=CARTESIAN_POINT('Ctrl Pts',(-4.90233604735018,-0.0368894657697565,
31.0068075185579));
#36984=CARTESIAN_POINT('Ctrl Pts',(-4.28759302222965,-2.3771423242123,31.0861794086113));
#36985=CARTESIAN_POINT('Ctrl Pts',(-2.62840182732014,-4.13832857419201,
31.1655512986647));
#36986=CARTESIAN_POINT('Ctrl Pts',(-0.328937765144189,-4.89142714353344,
31.2449231887181));
#36987=CARTESIAN_POINT('Ctrl Pts',(2.05065480852948,-4.45298488770047,31.3242950787715));
#36988=CARTESIAN_POINT('Ctrl Pts',(3.93071240989281,-2.9298053697385,31.4036669688249));
#36989=CARTESIAN_POINT('Ctrl Pts',(4.85325716869055,-0.692931748722414,
31.4830388588783));
#36990=CARTESIAN_POINT('Ctrl Pts',(4.59355922369783,1.712738512504,31.5624107489317));
#36991=CARTESIAN_POINT('Ctrl Pts',(3.21488041948321,3.70118946316684,31.6417826389851));
#36992=CARTESIAN_POINT('Ctrl Pts',(1.05306386109957,4.78803885304619,31.7211545290385));
#36993=CARTESIAN_POINT('Ctrl Pts',(-1.36527672293062,4.70853257646772,31.8005264190919));
#36994=CARTESIAN_POINT('Ctrl Pts',(-3.45103891924366,3.48203818642175,31.8798983091454));
#36995=CARTESIAN_POINT('Ctrl Pts',(-4.69613567357401,1.40732700152429,31.9592701991987));
#36996=CARTESIAN_POINT('Ctrl Pts',(-4.79726417254176,-1.010205925879,32.0386420892522));
#36997=CARTESIAN_POINT('Ctrl Pts',(-3.72978973764247,-3.1816549257911,32.1180139793055));
#36998=CARTESIAN_POINT('Ctrl Pts',(-1.75374677840301,-4.57805982825421,
32.197385869359));
#36999=CARTESIAN_POINT('Ctrl Pts',(0.649505014202782,-4.85925948991811,
32.2767577594123));
#37000=CARTESIAN_POINT('Ctrl Pts',(2.89453882300369,-3.95675429562642,32.3561296494657));
#37001=CARTESIAN_POINT('Ctrl Pts',(4.43446938147393,-2.09039251304725,32.4355015395192));
#37002=CARTESIAN_POINT('Ctrl Pts',(4.89417301414864,0.285184258704931,32.5148734295725));
#37003=CARTESIAN_POINT('Ctrl Pts',(4.16166693364494,2.59129077628124,32.594245319626));
#37004=CARTESIAN_POINT('Ctrl Pts',(2.41538799979881,4.26616459648027,32.6736172096793));
#37005=CARTESIAN_POINT('Ctrl Pts',(0.0807258955723594,4.90181016397187,
32.7529890997328));
#37006=CARTESIAN_POINT('Ctrl Pts',(-2.2736008581318,4.34338562549266,32.8323609897862));
#37007=CARTESIAN_POINT('Ctrl Pts',(-4.07408347532516,2.72692196256443,32.9117328798396));
#37008=CARTESIAN_POINT('Ctrl Pts',(-4.88212837576012,0.446186145494932,
32.991104769893));
#37009=CARTESIAN_POINT('Ctrl Pts',(-4.5008976102678,-1.94323962900084,33.0704766599464));
#37010=CARTESIAN_POINT('Ctrl Pts',(-3.02325814948215,-3.85929653115999,
33.1498485499998));
#37011=CARTESIAN_POINT('Ctrl Pts',(-0.809159695351077,-4.83523734073656,
33.2292204400532));
#37012=CARTESIAN_POINT('Ctrl Pts',(1.60204826952296,-4.63332503672604,33.3085923301066));
#37013=CARTESIAN_POINT('Ctrl Pts',(3.6230008220149,-3.30274500946005,33.3879642201599));
#37014=CARTESIAN_POINT('Ctrl Pts',(4.76139839364027,-1.16762360839165,33.4673361102135));
#37015=CARTESIAN_POINT('Ctrl Pts',(4.73992985575147,1.25192831918992,33.5467080002668));
#37016=CARTESIAN_POINT('Ctrl Pts',(3.56382489665835,3.36651327931318,33.6260798903203));
#37017=CARTESIAN_POINT('Ctrl Pts',(1.51958008113186,4.66102305624645,33.7054517803736));
#37018=CARTESIAN_POINT('Ctrl Pts',(-0.894831078624851,4.82011793367764,
33.784823670427));
#37019=CARTESIAN_POINT('Ctrl Pts',(-3.09126336830355,3.80504275161507,33.8641955604804));
#37020=CARTESIAN_POINT('Ctrl Pts',(-4.53467074385896,1.86306757757831,33.9435674505338));
#37021=CARTESIAN_POINT('Ctrl Pts',(-4.87344236353374,-0.532746734526401,
34.0229393405872));
#37022=CARTESIAN_POINT('Ctrl Pts',(-4.02505421063338,-2.79878512131536,
34.1023112306406));
#37023=CARTESIAN_POINT('Ctrl Pts',(-2.19617176132914,-4.38304564755766,
34.181683120694));
#37024=CARTESIAN_POINT('Ctrl Pts',(0.167693267891119,-4.89960595576193,
34.2610550107475));
#37025=CARTESIAN_POINT('Ctrl Pts',(2.4907085882359,-4.22263309823643,34.3404269008008));
#37026=CARTESIAN_POINT('Ctrl Pts',(4.20699280957637,-2.51703616462034,34.4197987908543));
#37027=CARTESIAN_POINT('Ctrl Pts',(4.89846289452463,-0.198294792667773,
34.4991706809077));
#37028=CARTESIAN_POINT('Ctrl Pts',(4.39667826093041,2.16875075186054,34.578542570961));
#37029=CARTESIAN_POINT('Ctrl Pts',(2.82387253485585,4.00749341368399,34.6579144610145));
#37030=CARTESIAN_POINT('Ctrl Pts',(0.563177709826186,4.87001955037029,34.7372863510678));
#37031=CARTESIAN_POINT('Ctrl Pts',(-1.83470595874441,4.54621970419178,34.8166582411213));
#37032=CARTESIAN_POINT('Ctrl Pts',(-3.78565931681763,3.11497080095877,34.8960301311746));
#37033=CARTESIAN_POINT('Ctrl Pts',(-4.81443444472882,0.924921905483118,
34.9754020212281));
#37034=CARTESIAN_POINT('Ctrl Pts',(-4.67042399847396,-1.49043591888832,
35.0547739112815));
#37035=CARTESIAN_POINT('Ctrl Pts',(-3.38870860399896,-3.5427268524425,35.1341458013349));
#37036=CARTESIAN_POINT('Ctrl Pts',(-1.28151129436916,-4.73201736643453,
35.2135176913883));
#37037=CARTESIAN_POINT('Ctrl Pts',(1.13785932999185,-4.76859892410594,35.2928895814417));
#37038=CARTESIAN_POINT('Ctrl Pts',(3.28004994017574,-3.64356033897983,35.3722614714951));
#37039=CARTESIAN_POINT('Ctrl Pts',(4.62322764520025,-1.63095852016229,35.4516333615485));
#37040=CARTESIAN_POINT('Ctrl Pts',(4.84019732919482,0.77894118410138,35.5310052516019));
#37041=CARTESIAN_POINT('Ctrl Pts',(3.87810565739256,2.99909254007502,35.6103771416553));
#37042=CARTESIAN_POINT('Ctrl Pts',(1.97131603149074,4.48867159166511,35.6897490317087));
#37043=CARTESIAN_POINT('Ctrl Pts',(-0.415681816248198,4.88482017903162,
35.7691209217621));
#37044=CARTESIAN_POINT('Ctrl Pts',(-2.70142049364518,4.09103738315207,35.8484928118155));
#37045=CARTESIAN_POINT('Ctrl Pts',(-4.32909911828301,2.30068693609431,35.9278647018689));
#37046=CARTESIAN_POINT('Ctrl Pts',(-4.90221878000546,-0.0501057561118174,
36.0072365919223));
#37047=CARTESIAN_POINT('Ctrl Pts',(-4.28116879779583,-2.38869279703632,
36.0866084819757));
#37048=CARTESIAN_POINT('Ctrl Pts',(-2.61723557264952,-4.14539955988464,
36.1659803720291));
#37049=CARTESIAN_POINT('Ctrl Pts',(-0.315749555158452,-4.89229616563135,
36.2453522620825));
#37050=CARTESIAN_POINT('Ctrl Pts',(2.06265235506943,-4.44744025434409,36.3247241521359));
#37051=CARTESIAN_POINT('Ctrl Pts',(3.93859671720591,-2.9191977413407,36.4040960421893));
#37052=CARTESIAN_POINT('Ctrl Pts',(4.85510763696701,-0.679845120081316,
36.4834679322428));
#37053=CARTESIAN_POINT('Ctrl Pts',(4.58892508296144,1.72511626761826,36.5628398222961));
#37054=CARTESIAN_POINT('Ctrl Pts',(3.20489053615983,3.70984315100612,36.6422117123496));
#37055=CARTESIAN_POINT('Ctrl Pts',(1.04015174865454,4.7908604544074,36.721583602403));
#37056=CARTESIAN_POINT('Ctrl Pts',(-1.37796570248609,4.70483475550478,36.8009554924563));
#37057=CARTESIAN_POINT('Ctrl Pts',(-3.46041375857649,3.47272172413633,36.8803273825098));
#37058=CARTESIAN_POINT('Ctrl Pts',(-4.69991268257361,1.39466136750738,36.9596992725631));
#37059=CARTESIAN_POINT('Ctrl Pts',(-4.79452328017606,-1.02313541121578,
37.0390711626166));
#37060=CARTESIAN_POINT('Ctrl Pts',(-3.72119861922486,-3.19169866843862,
37.11844305267));
#37061=CARTESIAN_POINT('Ctrl Pts',(-1.74139821136397,-4.5827711947349,37.1978149427234));
#37062=CARTESIAN_POINT('Ctrl Pts',(0.66260294626563,-4.85749080178586,37.2771868327768));
#37063=CARTESIAN_POINT('Ctrl Pts',(2.90519549283168,-3.94893640139516,37.3565587228302));
#37064=CARTESIAN_POINT('Ctrl Pts',(4.44008884788513,-2.07842983444732,37.4359306128835));
#37065=CARTESIAN_POINT('Ctrl Pts',(4.8933863875636,0.298377639646022,37.515302502937));
#37066=CARTESIAN_POINT('Ctrl Pts',(4.15466583455884,2.60250098116825,37.5946743929904));
#37067=CARTESIAN_POINT('Ctrl Pts',(2.40387788045201,4.272660844218,37.6740462830438));
#37068=CARTESIAN_POINT('Ctrl Pts',(0.0675105955612736,4.90200998298708,
37.7534181730972));
#37069=CARTESIAN_POINT('Ctrl Pts',(-2.28530212097756,4.33724034032229,37.8327900631506));
#37070=CARTESIAN_POINT('Ctrl Pts',(-4.08142029927378,2.71592855106086,37.9121619532041));
#37071=CARTESIAN_POINT('Ctrl Pts',(-4.883313526743,0.433022578390986,37.9915338432574));
#37072=CARTESIAN_POINT('Ctrl Pts',(-4.49564238811839,-1.95536673594121,
38.0709057333108));
#37073=CARTESIAN_POINT('Ctrl Pts',(-3.01284271470332,-3.86743304144309,
38.1502776233642));
#37074=CARTESIAN_POINT('Ctrl Pts',(-0.796121224763853,-4.8374012186294,
38.2296495134176));
#37075=CARTESIAN_POINT('Ctrl Pts',(1.61453363327388,-4.62898916605744,38.309021403471));
#37076=CARTESIAN_POINT('Ctrl Pts',(3.63189167208741,-3.29296559930574,38.3883932935244));
#37077=CARTESIAN_POINT('Ctrl Pts',(4.76452893838759,-1.15478290032729,38.4677651835778));
#37078=CARTESIAN_POINT('Ctrl Pts',(4.73653750187218,1.26470235504111,38.5471370736312));
#37079=CARTESIAN_POINT('Ctrl Pts',(3.55473601316178,3.37610891998471,38.6265089636846));
#37080=CARTESIAN_POINT('Ctrl Pts',(1.50700870159436,4.66510281756139,38.705880853738));
#37081=CARTESIAN_POINT('Ctrl Pts',(-0.907822597135966,4.81768800868639,
38.7852527437914));
#37082=CARTESIAN_POINT('Ctrl Pts',(-3.10151031466514,3.79669503846564,38.8646246338448));
#37083=CARTESIAN_POINT('Ctrl Pts',(-4.53967699589137,1.85083561019,38.9439965238982));
#37084=CARTESIAN_POINT('Ctrl Pts',(-4.87198838803768,-0.545883369388725,
39.0233684139517));
#37085=CARTESIAN_POINT('Ctrl Pts',(-4.01749423301241,-2.80962619208844,
39.102740304005));
#37086=CARTESIAN_POINT('Ctrl Pts',(-2.18434729950916,-4.38895062645438,
39.1821121940585));
#37087=CARTESIAN_POINT('Ctrl Pts',(0.180901657890313,-4.89913577411435,
39.2614840841118));
#37088=CARTESIAN_POINT('Ctrl Pts',(2.50208364241399,-4.21590347870473,39.3408559741653));
#37089=CARTESIAN_POINT('Ctrl Pts',(4.21376307902776,-2.50568418547649,39.4202278642187));
#37090=CARTESIAN_POINT('Ctrl Pts',(4.89898012125377,-0.185090004541199,
39.4995997542721));
#37091=CARTESIAN_POINT('Ctrl Pts',(4.39081462818005,2.18059968579169,39.5789716443255));
#37092=CARTESIAN_POINT('Ctrl Pts',(2.81305984991034,4.01508502497055,39.6583435343788));
#37093=CARTESIAN_POINT('Ctrl Pts',(0.55004342451412,4.87153304143481,39.7377154244323));
#37094=CARTESIAN_POINT('Ctrl Pts',(-1.84695009786503,4.54123256689917,39.8170873144857));
#37095=CARTESIAN_POINT('Ctrl Pts',(-3.79405383067523,3.10479958283119,39.8964592045391));
#37096=CARTESIAN_POINT('Ctrl Pts',(-4.8168906266497,0.911851793294956,39.9758310945925));
#37097=CARTESIAN_POINT('Ctrl Pts',(-4.66642692152748,-1.50285363850387,
40.0552029846459));
#37098=CARTESIAN_POINT('Ctrl Pts',(-3.37906911267765,-3.55219315325672,
40.1345748746994));
#37099=CARTESIAN_POINT('Ctrl Pts',(-1.9723130827443,-4.34047654372169,40.1874894680682));
#37100=CARTESIAN_POINT('Ctrl Pts',(-1.21713437249821,-4.54280821229862,
40.2139467647527));
#37101=CARTESIAN_POINT('Ctrl Pts',(-3.71544298812222,3.17665283523783,-0.213946764752703));
#37102=CARTESIAN_POINT('Ctrl Pts',(-4.2435173595033,2.55901209131059,-0.187489468068236));
#37103=CARTESIAN_POINT('Ctrl Pts',(-4.98521092249169,1.05595859527115,-0.1345748746993));
#37104=CARTESIAN_POINT('Ctrl Pts',(-4.8827252805975,-1.45743906270739,-0.0552029846458962));
#37105=CARTESIAN_POINT('Ctrl Pts',(-3.59110607910258,-3.61508997874938,
0.0241689054075074));
#37106=CARTESIAN_POINT('Ctrl Pts',(-1.42455668503541,-4.89247688957836,
0.103540795460911));
#37107=CARTESIAN_POINT('Ctrl Pts',(1.08893586889099,-4.9778765288597,0.182912685514315));
#37108=CARTESIAN_POINT('Ctrl Pts',(3.33720602914152,-3.85077723115681,0.262284575567719));
#37109=CARTESIAN_POINT('Ctrl Pts',(4.77251903131815,-1.78558378675016,0.341656465621122));
#37110=CARTESIAN_POINT('Ctrl Pts',(5.04526816392178,0.714545672093079,0.421028355674526));
#37111=CARTESIAN_POINT('Ctrl Pts',(4.0889952065405,3.04062834435892,0.500400245727928));
#37112=CARTESIAN_POINT('Ctrl Pts',(2.13665520967362,4.62601276074604,0.579772135781332));
#37113=CARTESIAN_POINT('Ctrl Pts',(-0.336170930871067,5.08451490337719,
0.659144025834737));
#37114=CARTESIAN_POINT('Ctrl Pts',(-2.72710569549275,4.30443824810499,0.738515915888139));
#37115=CARTESIAN_POINT('Ctrl Pts',(-4.45372401575963,2.47581113999331,0.817887805941545));
#37116=CARTESIAN_POINT('Ctrl Pts',(-5.09542477676098,0.0440812951164733,
0.897259695994947));
#37117=CARTESIAN_POINT('Ctrl Pts',(-4.49589147158092,-2.39838632564101,
0.976631586048351));
#37118=CARTESIAN_POINT('Ctrl Pts',(-2.80116888608231,-4.25661252099957,
1.05600347610176));
#37119=CARTESIAN_POINT('Ctrl Pts',(-0.424087796932823,-5.07793723552562,
1.13537536615516));
#37120=CARTESIAN_POINT('Ctrl Pts',(2.05630016029234,-4.66228772832596,1.21474725620856));
#37121=CARTESIAN_POINT('Ctrl Pts',(4.03577793971522,-3.11091522434116,1.29411914626197));
#37122=CARTESIAN_POINT('Ctrl Pts',(5.03214915152042,-0.801730671351417,
1.37349103631537));
#37123=CARTESIAN_POINT('Ctrl Pts',(4.80269996559999,1.70275370586111,1.45286292636877));
#37124=CARTESIAN_POINT('Ctrl Pts',(3.40332370018522,3.79245104545052,1.53223481642218));
#37125=CARTESIAN_POINT('Ctrl Pts',(1.17490531372441,4.95831570685873,1.61160670647558));
#37126=CARTESIAN_POINT('Ctrl Pts',(-1.33971740612181,4.9163456360401,1.69097859652898));
#37127=CARTESIAN_POINT('Ctrl Pts',(-3.52798793147818,3.67676465100145,1.77035048658239));
#37128=CARTESIAN_POINT('Ctrl Pts',(-4.85684840567494,1.54153193505596,1.84972237663579));
#37129=CARTESIAN_POINT('Ctrl Pts',(-5.00259135876462,-0.969214547985408,
1.9290942666892));
#37130=CARTESIAN_POINT('Ctrl Pts',(-3.92971412987363,-3.24386251254264,
2.0084661567426));
#37131=CARTESIAN_POINT('Ctrl Pts',(-1.89956723723801,-4.72831274916731,
2.087838046796));
#37132=CARTESIAN_POINT('Ctrl Pts',(0.593310029777512,-5.06095646606144,
2.16720993684941));
#37133=CARTESIAN_POINT('Ctrl Pts',(2.94165828680369,-4.16076239004749,2.24658182690281));
#37134=CARTESIAN_POINT('Ctrl Pts',(4.57342509641733,-2.24701580551599,2.32595371695621));
#37135=CARTESIAN_POINT('Ctrl Pts',(5.09111567564703,0.214098855557618,2.40532560700962));
#37136=CARTESIAN_POINT('Ctrl Pts',(4.36862174528326,2.62305950931529,2.48469749706302));
#37137=CARTESIAN_POINT('Ctrl Pts',(2.58194122754832,4.39304867264849,2.56406938711643));
#37138=CARTESIAN_POINT('Ctrl Pts',(0.166305541812792,5.09290090317231,2.64344127716983));
#37139=CARTESIAN_POINT('Ctrl Pts',(-2.28984180579737,4.55213374662856,2.72281316722323));
#37140=CARTESIAN_POINT('Ctrl Pts',(-4.18818875799412,2.90247688538309,2.80218505727664));
#37141=CARTESIAN_POINT('Ctrl Pts',(-5.06630219914209,0.545783079381991,
2.88155694733003));
#37142=CARTESIAN_POINT('Ctrl Pts',(-4.71027563864874,-1.94386227668626,
2.96092883738345));
#37143=CARTESIAN_POINT('Ctrl Pts',(-3.20683635859883,-3.95998708481986,
3.04030072743684));
#37144=CARTESIAN_POINT('Ctrl Pts',(-0.922218839806132,-5.01146780437411,
3.11967261749025));
#37145=CARTESIAN_POINT('Ctrl Pts',(1.58704914706656,-4.84216605947864,3.19904450754365));
#37146=CARTESIAN_POINT('Ctrl Pts',(3.70971547458753,-3.49332338044696,3.27841639759706));
#37147=CARTESIAN_POINT('Ctrl Pts',(4.92870332381492,-1.29351485827855,3.35778828765046));
#37148=CARTESIAN_POINT('Ctrl Pts',(4.94706995286075,1.22139102021994,3.43716017770387));
#37149=CARTESIAN_POINT('Ctrl Pts',(3.76034129154331,3.43876874969603,3.51653206775727));
#37150=CARTESIAN_POINT('Ctrl Pts',(1.65760181498019,4.81847002333168,3.59590395781068));
#37151=CARTESIAN_POINT('Ctrl Pts',(-0.848925794672718,5.02440266478622,
3.67527584786407));
#37152=CARTESIAN_POINT('Ctrl Pts',(-3.14865695980872,4.00640193842551,3.75464773791748));
#37153=CARTESIAN_POINT('Ctrl Pts',(-4.68138225896931,2.01245056788461,3.83401962797088));
#37154=CARTESIAN_POINT('Ctrl Pts',(-5.07373320190881,-0.471729306509208,
3.91339151802429));
#37155=CARTESIAN_POINT('Ctrl Pts',(-4.23013396738131,-2.84099696599249,
3.99276340807769));
#37156=CARTESIAN_POINT('Ctrl Pts',(-2.3560834616424,-4.51820405300012,4.0721352981311));
#37157=CARTESIAN_POINT('Ctrl Pts',(0.0919037602502722,-5.09478663357196,
4.1515071881845));
#37158=CARTESIAN_POINT('Ctrl Pts',(2.51750342957152,-4.43029046732459,4.2308790782379));
#37159=CARTESIAN_POINT('Ctrl Pts',(4.32984483584847,-2.6865853495186,4.3102509682913));
#37160=CARTESIAN_POINT('Ctrl Pts',(5.08744562406172,-0.288433987225658,
4.38962285834471));
#37161=CARTESIAN_POINT('Ctrl Pts',(4.60575591912341,2.17997925591765,4.46899474839811));
#37162=CARTESIAN_POINT('Ctrl Pts',(3.00211426695445,4.11735437762165,4.54836663845152));
#37163=CARTESIAN_POINT('Ctrl Pts',(0.667164224422586,5.05175108654635,4.62773852850492));
#37164=CARTESIAN_POINT('Ctrl Pts',(-1.83030554643563,4.75555241264972,4.70711041855833));
#37165=CARTESIAN_POINT('Ctrl Pts',(-3.88191693749475,3.30091169726834,4.78648230861172));
#37166=CARTESIAN_POINT('Ctrl Pts',(-4.98790195505755,1.04217619887652,4.86585419866514));
#37167=CARTESIAN_POINT('Ctrl Pts',(-4.87884509690204,-1.47043111474375,
4.94522608871853));
#37168=CARTESIAN_POINT('Ctrl Pts',(-3.58131237228163,-3.62484466355651,
5.02459797877194));
#37169=CARTESIAN_POINT('Ctrl Pts',(-1.4113798808739,-4.89625407578446,5.10396986882534));
#37170=CARTESIAN_POINT('Ctrl Pts',(1.10236162547835,-4.97494683282589,5.18334175887874));
#37171=CARTESIAN_POINT('Ctrl Pts',(3.34757027990012,-3.84175355324895,5.26271364893216));
#37172=CARTESIAN_POINT('Ctrl Pts',(4.77731822385938,-1.77271761167783,5.34208553898555));
#37173=CARTESIAN_POINT('Ctrl Pts',(5.04332202290099,0.728148416254135,5.42145742903896));
#37174=CARTESIAN_POINT('Ctrl Pts',(4.0807837403679,3.05163910171577,5.50082931909235));
#37175=CARTESIAN_POINT('Ctrl Pts',(2.12417557134277,4.63175725668802,5.58020120914577));
#37176=CARTESIAN_POINT('Ctrl Pts',(-0.349877065078572,5.08358959615188,
5.65957309919917));
#37177=CARTESIAN_POINT('Ctrl Pts',(-2.73870042288654,4.29707076232783,5.73894498925257));
#37178=CARTESIAN_POINT('Ctrl Pts',(-4.46038241968988,2.46379500220554,5.81831687930597));
#37179=CARTESIAN_POINT('Ctrl Pts',(-5.09552513194581,0.0303442330637155,
5.89768876935938));
#37180=CARTESIAN_POINT('Ctrl Pts',(-4.48940920081331,-2.41049832408661,
5.97706065941278));
#37181=CARTESIAN_POINT('Ctrl Pts',(-2.78968312550141,-4.26414882503699,
6.05643254946618));
#37182=CARTESIAN_POINT('Ctrl Pts',(-0.410396415676208,-5.07906211074168,
6.13580443951959));
#37183=CARTESIAN_POINT('Ctrl Pts',(2.06886195261065,-4.65672710858298,6.21517632957299));
#37184=CARTESIAN_POINT('Ctrl Pts',(4.04415012858982,-3.10002369026409,6.2945482196264));
#37185=CARTESIAN_POINT('Ctrl Pts',(5.03429228481897,-0.788161362782912,
6.37392010967979));
#37186=CARTESIAN_POINT('Ctrl Pts',(4.79809198368318,1.7156953281066,6.45329199973321));
#37187=CARTESIAN_POINT('Ctrl Pts',(3.39308709571864,3.80161243469653,6.5326638897866));
#37188=CARTESIAN_POINT('Ctrl Pts',(1.16153370170793,4.96146516692078,6.61203577984001));
#37189=CARTESIAN_POINT('Ctrl Pts',(-1.35296673102758,4.91271596650001,6.69140766989341));
#37190=CARTESIAN_POINT('Ctrl Pts',(-3.53788746282585,3.66724003075218,6.77077955994682));
#37191=CARTESIAN_POINT('Ctrl Pts',(-4.8609866396608,1.52843254081124,6.85015145000022));
#37192=CARTESIAN_POINT('Ctrl Pts',(-4.99996023068582,-0.982697732943262,
6.92952334005363));
#37193=CARTESIAN_POINT('Ctrl Pts',(-3.92095457674001,-3.25444501411732,
7.00889523010702));
#37194=CARTESIAN_POINT('Ctrl Pts',(-1.8868130667861,-4.73341669344426,7.08826712016043));
#37195=CARTESIAN_POINT('Ctrl Pts',(0.606951929847044,-5.05933854348832,
7.16763901021384));
#37196=CARTESIAN_POINT('Ctrl Pts',(2.95286477983474,-4.15281672299454,7.24701090026724));
#37197=CARTESIAN_POINT('Ctrl Pts',(4.57946630551004,-2.23467794088318,7.32638279032065));
#37198=CARTESIAN_POINT('Ctrl Pts',(5.0905199756398,0.227823441251604,7.40575468037404));
#37199=CARTESIAN_POINT('Ctrl Pts',(4.36153424737857,2.63482753737611,7.48512657042746));
#37200=CARTESIAN_POINT('Ctrl Pts',(2.57008843054822,4.39999347748764,7.56449846048085));
#37201=CARTESIAN_POINT('Ctrl Pts',(0.152574760830579,5.09333074570355,7.64387035053426));
#37202=CARTESIAN_POINT('Ctrl Pts',(-2.3021057829069,4.54594391816246,7.72324224058766));
#37203=CARTESIAN_POINT('Ctrl Pts',(-4.19599845355297,2.89117521443317,7.80261413064106));
#37204=CARTESIAN_POINT('Ctrl Pts',(-5.06775518859857,0.532122627975753,
7.88198602069447));
#37205=CARTESIAN_POINT('Ctrl Pts',(-4.70501797698741,-1.95655385282311,
7.96135791074787));
#37206=CARTESIAN_POINT('Ctrl Pts',(-3.19614880056275,-3.96861814583273,
8.04072980080128));
#37207=CARTESIAN_POINT('Ctrl Pts',(-0.908704850876407,-5.01393584290478,
8.12010169085468));
#37208=CARTESIAN_POINT('Ctrl Pts',(1.60009758909935,-4.83786986680398,8.19947358090808));
#37209=CARTESIAN_POINT('Ctrl Pts',(3.71911979812647,-3.48330949959307,8.27884547096148));
#37210=CARTESIAN_POINT('Ctrl Pts',(4.93217265646204,-1.28022264845606,8.3582173610149));
#37211=CARTESIAN_POINT('Ctrl Pts',(4.94375917286243,1.23472360612009,8.43758925106829));
#37212=CARTESIAN_POINT('Ctrl Pts',(3.75105689757885,3.4488939232597,8.5169611411217));
#37213=CARTESIAN_POINT('Ctrl Pts',(1.64460546486869,4.82292131469047,8.5963330311751));
#37214=CARTESIAN_POINT('Ctrl Pts',(-0.862468218811062,5.02209574921791,
8.67570492122851));
#37215=CARTESIAN_POINT('Ctrl Pts',(-3.15944655342946,3.99789877545622,8.75507681128191));
#37216=CARTESIAN_POINT('Ctrl Pts',(-4.68679070094874,1.99982250919225,8.83444870133531));
#37217=CARTESIAN_POINT('Ctrl Pts',(-5.07244300775217,-0.485406093778898,
8.91382059138872));
#37218=CARTESIAN_POINT('Ctrl Pts',(-4.22245942552934,-2.85239084673368,
8.99319248144211));
#37219=CARTESIAN_POINT('Ctrl Pts',(-2.34389407350296,-4.52453950308418,
9.07256437149552));
#37220=CARTESIAN_POINT('Ctrl Pts',(0.105638686707185,-5.09452035138171,
9.15193626154893));
#37221=CARTESIAN_POINT('Ctrl Pts',(2.52943809666274,-4.42348731861218,9.23130815160232));
#37222=CARTESIAN_POINT('Ctrl Pts',(4.33707198508751,-2.67490256625183,9.31068004165574));
#37223=CARTESIAN_POINT('Ctrl Pts',(5.08820473789098,-0.274717469548947,
9.39005193170913));
#37224=CARTESIAN_POINT('Ctrl Pts',(4.59986207909436,2.19238819465928,9.46942382176255));
#37225=CARTESIAN_POINT('Ctrl Pts',(2.99100319945234,4.12543294741746,9.54879571181595));
#37226=CARTESIAN_POINT('Ctrl Pts',(0.653542560897033,5.05353136567566,9.62816760186935));
#37227=CARTESIAN_POINT('Ctrl Pts',(-1.84311959890086,4.75060072905723,9.70753949192275));
#37228=CARTESIAN_POINT('Ctrl Pts',(-3.89080190408257,3.29043427011681,9.78691138197615));
#37229=CARTESIAN_POINT('Ctrl Pts',(-4.99069347757367,1.02872530622863,9.86628327202957));
#37230=CARTESIAN_POINT('Ctrl Pts',(-4.87486316664046,-1.48357886521197,
9.94565516208295));
#37231=CARTESIAN_POINT('Ctrl Pts',(-3.57152697864026,-3.63448650893304,
10.0250270521364));
#37232=CARTESIAN_POINT('Ctrl Pts',(-1.39817472408419,-4.90004128387748,
10.1043989421898));
#37233=CARTESIAN_POINT('Ctrl Pts',(1.11576979845155,-4.9719568481268,10.1837708322432));
#37234=CARTESIAN_POINT('Ctrl Pts',(3.35791526779908,-3.83271472941224,10.2631427222966));
#37235=CARTESIAN_POINT('Ctrl Pts',(4.7820800105301,-1.75983178618299,10.34251461235));
#37236=CARTESIAN_POINT('Ctrl Pts',(5.04134064765054,0.741742284838825,10.4218865024034));
#37237=CARTESIAN_POINT('Ctrl Pts',(4.07254186182158,3.0626295770926,10.5012583924568));
#37238=CARTESIAN_POINT('Ctrl Pts',(2.11168089287137,4.63746708338223,10.5806302825102));
#37239=CARTESIAN_POINT('Ctrl Pts',(-0.363580867455945,5.08262787301918,
10.6600021725636));
#37240=CARTESIAN_POINT('Ctrl Pts',(-2.75027513324356,4.28967176299466,10.739374062617));
#37241=CARTESIAN_POINT('Ctrl Pts',(-4.46700846420381,2.45176110653202,10.8187459526704));
#37242=CARTESIAN_POINT('Ctrl Pts',(-5.09558842083953,0.0166068713993523,
10.8981178427238));
#37243=CARTESIAN_POINT('Ctrl Pts',(-4.48289431705241,-2.42259276084751,
10.9774897327772));
#37244=CARTESIAN_POINT('Ctrl Pts',(-2.77817708034959,-4.27165415887005,
11.0568616228306));
#37245=CARTESIAN_POINT('Ctrl Pts',(-0.396702056264276,-5.08015005893795,
11.136233512884));
#37246=CARTESIAN_POINT('Ctrl Pts',(2.0814087106419,-4.65113264937,11.2156054029374));
#37247=CARTESIAN_POINT('Ctrl Pts',(4.05249292275577,-3.08910962152302,11.2949772929908));
#37248=CARTESIAN_POINT('Ctrl Pts',(5.03639882892726,-0.774586327501172,
11.3743491830442));
#37249=CARTESIAN_POINT('Ctrl Pts',(4.79344912825178,1.7286244813822,11.4537210730976));
#37250=CARTESIAN_POINT('Ctrl Pts',(3.38282583005384,3.81074619284624,11.533092963151));
#37251=CARTESIAN_POINT('Ctrl Pts',(1.14815364741277,4.96457856667656,11.6124648532044));
#37252=CARTESIAN_POINT('Ctrl Pts',(-1.36620622234309,4.90905059057276,11.6918367432579));
#37253=CARTESIAN_POINT('Ctrl Pts',(-3.54776128038234,3.65768875660455,11.7712086333112));
#37254=CARTESIAN_POINT('Ctrl Pts',(-4.86508954335683,1.51532203768426,11.8505805233647));
#37255=CARTESIAN_POINT('Ctrl Pts',(-4.99729276226266,-0.9961737755075,11.9299524134181));
#37256=CARTESIAN_POINT('Ctrl Pts',(-3.91216652560121,-3.26500386197887,
12.0093243034715));
#37257=CARTESIAN_POINT('Ctrl Pts',(-1.87404518273703,-4.73848623463566,
12.0886961935249));
#37258=CARTESIAN_POINT('Ctrl Pts',(0.620589418513222,-5.05768384899659,
12.1680680835782));
#37259=CARTESIAN_POINT('Ctrl Pts',(2.96404981106505,-4.14484087273527,12.2474399736317));
#37260=CARTESIAN_POINT('Ctrl Pts',(4.58547423045439,-2.2223238343253,12.3268118636851));
#37261=CARTESIAN_POINT('Ctrl Pts',(5.08988727708011,0.241546371095948,12.4061837537385));
#37262=CARTESIAN_POINT('Ctrl Pts',(4.3544150492835,2.64657641517207,12.4855556437919));
#37263=CARTESIAN_POINT('Ctrl Pts',(2.55821695381563,4.40690630260979,12.5649275338453));
#37264=CARTESIAN_POINT('Ctrl Pts',(0.138842870915485,5.09372356925339,12.6442994238987));
#37265=CARTESIAN_POINT('Ctrl Pts',(-2.3143530280162,4.53972104919276,12.7236713139521));
#37266=CARTESIAN_POINT('Ctrl Pts',(-4.20377765205669,2.87985253005087,12.8030432040055));
#37267=CARTESIAN_POINT('Ctrl Pts',(-5.06917134496016,0.518458309034014,
12.8824150940589));
#37268=CARTESIAN_POINT('Ctrl Pts',(-4.69972611865178,-1.9692312084755,12.9617869841123));
#37269=CARTESIAN_POINT('Ctrl Pts',(-3.18543801250715,-3.97722036241972,
13.0411588741657));
#37270=CARTESIAN_POINT('Ctrl Pts',(-0.895184257363228,-5.01636743950647,
13.1205307642191));
#37271=CARTESIAN_POINT('Ctrl Pts',(1.61313440141763,-4.83353851187042,13.1999026542725));
#37272=CARTESIAN_POINT('Ctrl Pts',(3.72849709062559,-3.47327030159879,13.2792745443259));
#37273=CARTESIAN_POINT('Ctrl Pts',(4.93560614144549,-1.26692113381109,13.3586464343793));
#37274=CARTESIAN_POINT('Ctrl Pts',(4.94041246098816,1.24804721789062,13.4380183244327));
#37275=CARTESIAN_POINT('Ctrl Pts',(3.74174524045162,3.45899402981983,13.5173902144861));
#37276=CARTESIAN_POINT('Ctrl Pts',(1.63159716155366,4.82733755243838,13.5967621045395));
#37277=CARTESIAN_POINT('Ctrl Pts',(-0.87600437441973,5.01975233241333,13.6761339945929));
#37278=CARTESIAN_POINT('Ctrl Pts',(-3.17021318378723,3.98936655524573,13.7555058846463));
#37279=CARTESIAN_POINT('Ctrl Pts',(-4.69216507873203,1.98717991553337,13.8348777746998));
#37280=CARTESIAN_POINT('Ctrl Pts',(-5.07111594642896,-0.499079353054812,
13.9142496647532));
#37281=CARTESIAN_POINT('Ctrl Pts',(-4.21475419430051,-2.86376399593225,
13.9936215548066));
#37282=CARTESIAN_POINT('Ctrl Pts',(-2.33168764964064,-4.53084206823465,
14.07299344486));
#37283=CARTESIAN_POINT('Ctrl Pts',(0.119372845368581,-5.09421704156391,
14.1523653349133));
#37284=CARTESIAN_POINT('Ctrl Pts',(2.54135437947334,-4.4166520194264,14.2317372249668));
#37285=CARTESIAN_POINT('Ctrl Pts',(4.34426761193091,-2.66320034145004,14.3111091150202));
#37286=CARTESIAN_POINT('Ctrl Pts',(5.08892686999541,-0.260998955190403,
14.3904810050736));
#37287=CARTESIAN_POINT('Ctrl Pts',(4.59393480667753,2.20478119884224,14.469852895127));
#37288=CARTESIAN_POINT('Ctrl Pts',(2.97987039295526,4.13348153303728,14.5492247851804));
#37289=CARTESIAN_POINT('Ctrl Pts',(0.639916147340316,5.05527491509065,14.6285966752338));
#37290=CARTESIAN_POINT('Ctrl Pts',(-1.85592025533638,4.74561451748915,14.7079685652872));
#37291=CARTESIAN_POINT('Ctrl Pts',(-3.89965859182293,3.27993292766684,14.7873404553406));
#37292=CARTESIAN_POINT('Ctrl Pts',(-4.99344872708928,1.01526693667329,14.866712345394));
#37293=CARTESIAN_POINT('Ctrl Pts',(-4.87084580524798,-1.49671583283861,
14.9460842354474));
#37294=CARTESIAN_POINT('Ctrl Pts',(-3.56171562668257,-3.64410193839537,
15.0254561255008));
#37295=CARTESIAN_POINT('Ctrl Pts',(-1.38495940518108,-4.90379287784181,
15.1048280155542));
#37296=CARTESIAN_POINT('Ctrl Pts',(1.12916986186683,-4.9689307266074,15.1841999056076));
#37297=CARTESIAN_POINT('Ctrl Pts',(3.36823584993909,-3.82364804891307,15.263571795661));
#37298=CARTESIAN_POINT('Ctrl Pts',(4.78680704042976,-1.74693317000493,15.3429436857144));
#37299=CARTESIAN_POINT('Ctrl Pts',(5.0393226312895,0.755330762345426,15.4223155757678));
#37300=CARTESIAN_POINT('Ctrl Pts',(4.06427038351844,3.07359779288479,15.5016874658212));
#37301=CARTESIAN_POINT('Ctrl Pts',(2.09917086643239,4.64314320437064,15.5810593558746));
#37302=CARTESIAN_POINT('Ctrl Pts',(-0.377282027281083,5.08162920869508,
15.660431245928));
#37303=CARTESIAN_POINT('Ctrl Pts',(-2.76182985424771,4.28224158577663,15.7398031359814));
#37304=CARTESIAN_POINT('Ctrl Pts',(-4.47360204192776,2.43970939114443,15.8191750260348));
#37305=CARTESIAN_POINT('Ctrl Pts',(-5.09561467434161,0.00286938903366673,
15.8985469160882));
#37306=CARTESIAN_POINT('Ctrl Pts',(-4.47634685104277,-2.43466958989267,
15.9779188061416));
#37307=CARTESIAN_POINT('Ctrl Pts',(-2.76665084304587,-4.27912844577413,
16.0572906961951));
#37308=CARTESIAN_POINT('Ctrl Pts',(-0.383004813579153,-5.08120108394907,
16.1366625862484));
#37309=CARTESIAN_POINT('Ctrl Pts',(2.09394034074345,-4.64550438513334,16.2160344763019));
#37310=CARTESIAN_POINT('Ctrl Pts',(4.06080626285358,-3.07817310072693,16.2954063663552));
#37311=CARTESIAN_POINT('Ctrl Pts',(5.03846876789878,-0.761005662445124,
16.3747782564087));
#37312=CARTESIAN_POINT('Ctrl Pts',(4.7887714333112,1.74154107082836,16.4541501464621));
#37313=CARTESIAN_POINT('Ctrl Pts',(3.37253997777685,3.81985225393751,16.5335220365155));
#37314=CARTESIAN_POINT('Ctrl Pts',(1.13476524781198,4.96765588336339,16.6128939265689));
#37315=CARTESIAN_POINT('Ctrl Pts',(-1.37943578318358,4.90534953479992,16.6922658166222));
#37316=CARTESIAN_POINT('Ctrl Pts',(-3.5576093137008,3.64811089835147,16.7716377066757));
#37317=CARTESIAN_POINT('Ctrl Pts',(-4.86915708441607,1.50220052016076,16.851009596729));
#37318=CARTESIAN_POINT('Ctrl Pts',(-4.99458897767399,-1.00964257616395,
16.9303814867825));
#37319=CARTESIAN_POINT('Ctrl Pts',(-3.90335003127183,-3.2755389823738,17.0097533768359));
#37320=CARTESIAN_POINT('Ctrl Pts',(-1.8612636949986,-4.74352133023597,17.0891252668893));
#37321=CARTESIAN_POINT('Ctrl Pts',(0.634222428965914,-5.05599240530682,
17.1684971569427));
#37322=CARTESIAN_POINT('Ctrl Pts',(2.9752132381933,-4.13683487704247,17.2478690469961));
#37323=CARTESIAN_POINT('Ctrl Pts',(4.59144894277892,-2.20995361377096,17.3272409370495));
#37324=CARTESIAN_POINT('Ctrl Pts',(5.08921736705481,0.255267617363485,17.4066128271029));
#37325=CARTESIAN_POINT('Ctrl Pts',(4.34726461344772,2.65830592133578,17.4859847171563));
#37326=CARTESIAN_POINT('Ctrl Pts',(2.54632610813648,4.41378735452059,17.5653566072097));
#37327=CARTESIAN_POINT('Ctrl Pts',(0.125111436169681,5.09407888617233,17.6447284972631));
#37328=CARTESIAN_POINT('Ctrl Pts',(-2.32658621700147,4.53346610033861,17.7241003873165));
#37329=CARTESIAN_POINT('Ctrl Pts',(-4.21152107628919,2.8685071860873,17.8034722773699));
#37330=CARTESIAN_POINT('Ctrl Pts',(-5.07056051563183,0.504793485523745,
17.8828441674233));
#37331=CARTESIAN_POINT('Ctrl Pts',(-4.69438148876582,-1.98190041394314,
17.9622160574767));
#37332=CARTESIAN_POINT('Ctrl Pts',(-3.1747392180444,-3.9857820361196,18.0415879475301));
#37333=CARTESIAN_POINT('Ctrl Pts',(-0.881590795203727,-5.01878454751455,
18.1209598375835));
#37334=CARTESIAN_POINT('Ctrl Pts',(1.62603418385021,-4.82913054051801,18.2003317276369));
#37335=CARTESIAN_POINT('Ctrl Pts',(3.73808388472066,-3.46328419200805,18.2797036176903));
#37336=CARTESIAN_POINT('Ctrl Pts',(4.93855701420293,-1.25346250930793,18.3590755077438));
#37337=CARTESIAN_POINT('Ctrl Pts',(4.93787328845974,1.26108254025623,18.4384473977971));
#37338=CARTESIAN_POINT('Ctrl Pts',(3.73081451079157,3.46959580775143,18.5178192878506));
#37339=CARTESIAN_POINT('Ctrl Pts',(1.62157688245111,4.83072732396141,18.597191177904));
#37340=CARTESIAN_POINT('Ctrl Pts',(-0.895150293053049,5.01921699961797,
18.6765630679574));
#37341=CARTESIAN_POINT('Ctrl Pts',(-3.17074515011531,3.97754537770249,18.7559349580108));
#37342=CARTESIAN_POINT('Ctrl Pts',(-5.22808970274021,1.31272284990122,18.8617641447486));
#37343=CARTESIAN_POINT('Ctrl Pts',(-4.77339715849023,-3.25411141853201,
18.994050628171));
#37344=CARTESIAN_POINT('Ctrl Pts',(0.152720854580862,-5.77834717219764,
19.1527944082778));
#37345=CARTESIAN_POINT('Ctrl Pts',(4.93271294602037,-3.00474199436408,19.3115381883846));
#37346=CARTESIAN_POINT('Ctrl Pts',(5.20235975367847,2.51303602329821,19.4702819684914));
#37347=CARTESIAN_POINT('Ctrl Pts',(0.709818611660393,5.73400533709388,19.6290257485982));
#37348=CARTESIAN_POINT('Ctrl Pts',(-4.43131449514935,3.70671199728522,19.787769528705));
#37349=CARTESIAN_POINT('Ctrl Pts',(-5.51805139390214,-1.71188403765749,
19.9465133088118));
#37350=CARTESIAN_POINT('Ctrl Pts',(-1.55524717023727,-5.56394358573197,
20.1052570889187));
#37351=CARTESIAN_POINT('Ctrl Pts',(3.83058845612614,-4.32541925679744,20.2640008690254));
#37352=CARTESIAN_POINT('Ctrl Pts',(5.71123844601177,0.87272703286029,20.4227446491323));
#37353=CARTESIAN_POINT('Ctrl Pts',(2.36591519662234,5.26902047281308,20.581488429239));
#37354=CARTESIAN_POINT('Ctrl Pts',(-3.14459942082001,4.85016640791291,20.7402322093459));
#37355=CARTESIAN_POINT('Ctrl Pts',(-5.77704085522352,-0.0189872057270379,
20.8989759894526));
#37356=CARTESIAN_POINT('Ctrl Pts',(-3.56709774791074,-4.0412840629435,21.031262472875));
#37357=CARTESIAN_POINT('Ctrl Pts',(-0.362731338653644,-5.07374792580599,
21.1370916596129));
#37358=CARTESIAN_POINT('Ctrl Pts',(2.10287077052077,-4.64454172754387,21.2164635496663));
#37359=CARTESIAN_POINT('Ctrl Pts',(4.07100210770441,-3.06469899064061,21.2958354397197));
#37360=CARTESIAN_POINT('Ctrl Pts',(5.03948789886561,-0.748754766453301,
21.3752073297731));
#37361=CARTESIAN_POINT('Ctrl Pts',(4.78459624359497,1.75515257798294,21.4545792198265));
#37362=CARTESIAN_POINT('Ctrl Pts',(3.36194502775863,3.82855576883798,21.5339511098799));
#37363=CARTESIAN_POINT('Ctrl Pts',(1.12151932172619,4.97089558679479,21.6133229999333));
#37364=CARTESIAN_POINT('Ctrl Pts',(-1.39273514199732,4.9015077036213,21.6926948899867));
#37365=CARTESIAN_POINT('Ctrl Pts',(-3.56738921282951,3.63856219800436,21.7720667800401));
#37366=CARTESIAN_POINT('Ctrl Pts',(-4.87321162956223,1.48903860109202,21.8514386700935));
#37367=CARTESIAN_POINT('Ctrl Pts',(-4.99183702504821,-1.02308842639,21.9308105601469));
#37368=CARTESIAN_POINT('Ctrl Pts',(-3.89451146459856,-3.28605855970678,
22.0101824502003));
#37369=CARTESIAN_POINT('Ctrl Pts',(-1.84846531944319,-4.74851758083281,
22.0895543402537));
#37370=CARTESIAN_POINT('Ctrl Pts',(0.647849003889951,-5.05426651218743,
22.1689262303072));
#37371=CARTESIAN_POINT('Ctrl Pts',(2.98635609589609,-4.12879762624803,22.2482981203605));
#37372=CARTESIAN_POINT('Ctrl Pts',(4.59738955946421,-2.19756790530644,22.3276700104139));
#37373=CARTESIAN_POINT('Ctrl Pts',(5.08851116459638,0.268987208844064,22.4070419004674));
#37374=CARTESIAN_POINT('Ctrl Pts',(4.34008162116472,2.67001619606227,22.4864137905207));
#37375=CARTESIAN_POINT('Ctrl Pts',(2.53441837980377,4.4206359096037,22.5657856805742));
#37376=CARTESIAN_POINT('Ctrl Pts',(0.11137612465092,5.09439809707615,22.6451575706275));
#37377=CARTESIAN_POINT('Ctrl Pts',(-2.3387969457162,4.52717639800266,22.724529460681));
#37378=CARTESIAN_POINT('Ctrl Pts',(-4.2192443428605,2.85714443596456,22.8039013507343));
#37379=CARTESIAN_POINT('Ctrl Pts',(-5.07189311172227,0.491118473430054,
22.8832732407878));
#37380=CARTESIAN_POINT('Ctrl Pts',(-4.6890399691108,-1.99454289389497,22.9626451308412));
#37381=CARTESIAN_POINT('Ctrl Pts',(-3.1639470562758,-3.99433801030587,23.0420170208946));
#37382=CARTESIAN_POINT('Ctrl Pts',(-0.868123650568842,-5.02112123762457,
23.121388910948));
#37383=CARTESIAN_POINT('Ctrl Pts',(1.63917275843702,-4.82477044080721,23.2007608010014));
#37384=CARTESIAN_POINT('Ctrl Pts',(3.74717030983928,-3.45311624655406,23.2801326910548));
#37385=CARTESIAN_POINT('Ctrl Pts',(4.94236546898948,-1.24029057666132,23.3595045811082));
#37386=CARTESIAN_POINT('Ctrl Pts',(4.93361133910258,1.27466713166923,23.4388764711616));
#37387=CARTESIAN_POINT('Ctrl Pts',(3.72304040765536,3.47911874852391,23.518248361215));
#37388=CARTESIAN_POINT('Ctrl Pts',(1.60554507356429,4.83606473894047,23.5976202512684));
#37389=CARTESIAN_POINT('Ctrl Pts',(-0.903057486554317,5.01495606350285,
23.6769921413218));
#37390=CARTESIAN_POINT('Ctrl Pts',(-3.19167724187396,3.97221519135782,23.7563640313752));
#37391=CARTESIAN_POINT('Ctrl Pts',(-4.70281148570869,1.96185149097637,23.8357359214286));
#37392=CARTESIAN_POINT('Ctrl Pts',(-5.06835126113314,-0.526414890137771,
23.915107811482));
#37393=CARTESIAN_POINT('Ctrl Pts',(-4.1992518879446,-2.88644776920571,23.9944797015354));
#37394=CARTESIAN_POINT('Ctrl Pts',(-2.30722404974247,-4.54334836074326,
24.0738515915888));
#37395=CARTESIAN_POINT('Ctrl Pts',(0.1468384600249,-5.09349934813251,24.1532234816422));
#37396=CARTESIAN_POINT('Ctrl Pts',(2.56513144595071,-4.40288516858744,24.2325953716957));
#37397=CARTESIAN_POINT('Ctrl Pts',(4.35856408946553,-2.63973790759483,24.311967261749));
#37398=CARTESIAN_POINT('Ctrl Pts',(5.09026016830426,-0.23355633527326,24.3913391518024));
#37399=CARTESIAN_POINT('Ctrl Pts',(4.58198013724401,2.22951904335289,24.4707110418559));
#37400=CARTESIAN_POINT('Ctrl Pts',(2.95753988679205,4.1494885179749,24.5500829319092));
#37401=CARTESIAN_POINT('Ctrl Pts',(0.612649466321058,5.05865177435533,24.6294548219626));
#37402=CARTESIAN_POINT('Ctrl Pts',(-1.88148100806917,4.73553865563851,24.7088267120161));
#37403=CARTESIAN_POINT('Ctrl Pts',(-3.91728687348126,3.25885880234522,24.7881986020694));
#37404=CARTESIAN_POINT('Ctrl Pts',(-4.99885032728078,0.988328158162253,
24.8675704921229));
#37405=CARTESIAN_POINT('Ctrl Pts',(-4.86270490612224,-1.5229570377218,24.9469423821763));
#37406=CARTESIAN_POINT('Ctrl Pts',(-3.54201533324704,-3.66325327022505,
25.0263142722297));
#37407=CARTESIAN_POINT('Ctrl Pts',(-1.3584986653108,-4.91118911457504,25.1056861622831));
#37408=CARTESIAN_POINT('Ctrl Pts',(1.15594527050936,-4.96277016134726,25.1850580523365));
#37409=CARTESIAN_POINT('Ctrl Pts',(3.38880349707489,-3.80543138172069,25.2644299423899));
#37410=CARTESIAN_POINT('Ctrl Pts',(4.79615669274227,-1.72109794068643,25.3438018324433));
#37411=CARTESIAN_POINT('Ctrl Pts',(5.0351767341704,0.782491149113306,25.4231737224967));
#37412=CARTESIAN_POINT('Ctrl Pts',(4.04763886832931,3.09546712700384,25.5025456125501));
#37413=CARTESIAN_POINT('Ctrl Pts',(2.07410513345989,4.65439416445651,25.5819175026035));
#37414=CARTESIAN_POINT('Ctrl Pts',(-0.404676020966502,5.07952108577436,
25.6612893926569));
#37415=CARTESIAN_POINT('Ctrl Pts',(-2.78487899242069,4.26728791392678,25.7406612827102));
#37416=CARTESIAN_POINT('Ctrl Pts',(-4.48669160554627,2.41555285172821,25.8200331727637));
#37417=CARTESIAN_POINT('Ctrl Pts',(-5.09555607468418,-0.0246055384158182,
25.8994050628171));
#37418=CARTESIAN_POINT('Ctrl Pts',(-4.46315436285108,-2.45877007386518,
25.9787769528705));
#37419=CARTESIAN_POINT('Ctrl Pts',(-2.74353812725205,-4.29398366171623,
26.0581488429239));
#37420=CARTESIAN_POINT('Ctrl Pts',(-0.355602076573053,-5.0831923341448,
26.1375207329773));
#37421=CARTESIAN_POINT('Ctrl Pts',(2.11895785284724,-4.63414660543109,26.2168926230307));
#37422=CARTESIAN_POINT('Ctrl Pts',(4.07734433954763,-3.05623302114393,26.2962645130841));
#37423=CARTESIAN_POINT('Ctrl Pts',(5.04249877018284,-0.733827837763115,
26.3756364031375));
#37424=CARTESIAN_POINT('Ctrl Pts',(4.77931166178323,1.76733618259643,26.4550082931909));
#37425=CARTESIAN_POINT('Ctrl Pts',(3.3518948114001,3.83798102080776,26.5343801832444));
#37426=CARTESIAN_POINT('Ctrl Pts',(1.10796380425329,4.97370217757719,26.6137520732977));
#37427=CARTESIAN_POINT('Ctrl Pts',(-1.40586473317334,4.89784049299189,26.6931239633511));
#37428=CARTESIAN_POINT('Ctrl Pts',(-3.57722773342779,3.62887570549981,26.7724958534045));
#37429=CARTESIAN_POINT('Ctrl Pts',(-4.87718597587851,1.47592482852807,26.851867743458));
#37430=CARTESIAN_POINT('Ctrl Pts',(-4.98907251007324,-1.0365580697689,26.9312396335114));
#37431=CARTESIAN_POINT('Ctrl Pts',(-3.88563202393884,-3.29653771665249,
27.0106115235647));
#37432=CARTESIAN_POINT('Ctrl Pts',(-1.83566017747357,-4.75348807252204,
27.0899834136182));
#37433=CARTESIAN_POINT('Ctrl Pts',(0.661474425059423,-5.05249925559262,
27.1693553036715));
#37434=CARTESIAN_POINT('Ctrl Pts',(2.99747532179674,-4.12073280351822,27.248727193725));
#37435=CARTESIAN_POINT('Ctrl Pts',(4.60329786494346,-2.18516496159412,27.3280990837784));
#37436=CARTESIAN_POINT('Ctrl Pts',(5.08776723741692,0.282704228193704,27.4074709738318));
#37437=CARTESIAN_POINT('Ctrl Pts',(4.33286777243738,2.68170729374875,27.4868428638852));
#37438=CARTESIAN_POINT('Ctrl Pts',(2.5224913087322,4.42745239840498,27.5662147539386));
#37439=CARTESIAN_POINT('Ctrl Pts',(0.0976415456597213,5.09467989880942,
27.6455866439919));
#37440=CARTESIAN_POINT('Ctrl Pts',(-2.35099348180958,4.52085465274658,27.7249585340454));
#37441=CARTESIAN_POINT('Ctrl Pts',(-4.22693170094588,2.84575922001675,27.8043304240988));
#37442=CARTESIAN_POINT('Ctrl Pts',(-5.07319871388641,0.477443140272041,
27.8837023141522));
#37443=CARTESIAN_POINT('Ctrl Pts',(-4.68364574945911,-2.00717703164051,
27.9630742042056));
#37444=CARTESIAN_POINT('Ctrl Pts',(-3.15316704753758,-4.00285332145644,
28.042446094259));
#37445=CARTESIAN_POINT('Ctrl Pts',(-0.854583832252744,-5.02344340233109,
28.1218179843124));
#37446=CARTESIAN_POINT('Ctrl Pts',(1.65217411297962,-4.82033378960126,28.2011898743658));
#37447=CARTESIAN_POINT('Ctrl Pts',(3.75646610131553,-3.44300153535241,28.2805617644192));
#37448=CARTESIAN_POINT('Ctrl Pts',(4.94569126216762,-1.22696172804632,28.3599336544726));
#37449=CARTESIAN_POINT('Ctrl Pts',(4.93015697865761,1.28796324037807,28.439305544526));
#37450=CARTESIAN_POINT('Ctrl Pts',(3.71364736786401,3.48914321430466,28.5186774345794));
#37451=CARTESIAN_POINT('Ctrl Pts',(1.59250147827778,4.84037562431415,28.5980493246328));
#37452=CARTESIAN_POINT('Ctrl Pts',(-0.916574246474672,5.01250324623047,
28.6774212146862));
#37453=CARTESIAN_POINT('Ctrl Pts',(-3.20237451358863,3.96359617235279,28.7567931047396));
#37454=CARTESIAN_POINT('Ctrl Pts',(-4.70808343752814,1.94916584416126,28.836164994793));
#37455=CARTESIAN_POINT('Ctrl Pts',(-5.0669136572517,-0.540076969262536,
28.9155368848465));
#37456=CARTESIAN_POINT('Ctrl Pts',(-4.19145492549188,-2.89775822841407,
28.9949087748998));
#37457=CARTESIAN_POINT('Ctrl Pts',(-2.29496705151034,-4.54955199720298,
29.0742806649532));
#37458=CARTESIAN_POINT('Ctrl Pts',(0.160569716395729,-5.09308496973575,
29.1536525550067));
#37459=CARTESIAN_POINT('Ctrl Pts',(2.57699205680278,-4.39595371699326,29.23302444506));
#37460=CARTESIAN_POINT('Ctrl Pts',(4.36566483624787,-2.62797786906977,29.3123963351135));
#37461=CARTESIAN_POINT('Ctrl Pts',(5.09087132481821,-0.219832429171176,
29.3917682251668));
#37462=CARTESIAN_POINT('Ctrl Pts',(4.57595282711536,2.24186370388268,29.4711401152203));
#37463=CARTESIAN_POINT('Ctrl Pts',(2.94634234942697,4.15744680095185,29.5505120052737));
#37464=CARTESIAN_POINT('Ctrl Pts',(0.599009397036387,5.06028505966152,29.6298838953271));
#37465=CARTESIAN_POINT('Ctrl Pts',(-1.89424091858745,4.73044907858869,29.7092557853805));
#37466=CARTESIAN_POINT('Ctrl Pts',(-3.92605833927458,3.24828617264307,29.7886276754339));
#37467=CARTESIAN_POINT('Ctrl Pts',(-5.00149663869715,0.974847945001076,
29.8679995654873));
#37468=CARTESIAN_POINT('Ctrl Pts',(-4.85858142755809,-1.53606108425386,
29.9473714555407));
#37469=CARTESIAN_POINT('Ctrl Pts',(-3.53212653495348,-3.67278903339805,
30.026743345594));
#37470=CARTESIAN_POINT('Ctrl Pts',(-1.34525343666372,-4.91483370358714,
30.1061152356475));
#37471=CARTESIAN_POINT('Ctrl Pts',(1.16932042112941,-4.95963576238229,30.1854871257009));
#37472=CARTESIAN_POINT('Ctrl Pts',(3.39905041258226,-3.79628152742866,30.2648590157543));
#37473=CARTESIAN_POINT('Ctrl Pts',(4.80077924720052,-1.70816151532001,30.3442309058077));
#37474=CARTESIAN_POINT('Ctrl Pts',(5.03304888354535,0.796062860969203,30.4236027958611));
#37475=CARTESIAN_POINT('Ctrl Pts',(4.03927895232327,3.10636808638158,30.5029746859145));
#37476=CARTESIAN_POINT('Ctrl Pts',(2.06154960910751,4.65996892178051,30.5823465759679));
#37477=CARTESIAN_POINT('Ctrl Pts',(-0.418368655724119,5.07841164249995,
30.6617184660213));
#37478=CARTESIAN_POINT('Ctrl Pts',(-2.79637324206467,4.25976452797996,30.7410903560747));
#37479=CARTESIAN_POINT('Ctrl Pts',(-4.49318749630546,2.4034482032729,30.8204622461281));
#37480=CARTESIAN_POINT('Ctrl Pts',(-5.09547122194811,-0.0383427838090456,
30.8998341361815));
#37481=CARTESIAN_POINT('Ctrl Pts',(-4.45650943655845,-2.47079355362547,
30.9792060262349));
#37482=CARTESIAN_POINT('Ctrl Pts',(-2.73195181673944,-4.3013644827875,31.0585779162883));
#37483=CARTESIAN_POINT('Ctrl Pts',(-0.341896781435476,-5.08413254485124,
31.1379498063417));
#37484=CARTESIAN_POINT('Ctrl Pts',(2.13144355305047,-4.62841717252575,31.2173216963952));
#37485=CARTESIAN_POINT('Ctrl Pts',(4.08556895588362,-3.04522962180058,31.2966935864485));
#37486=CARTESIAN_POINT('Ctrl Pts',(5.04445880431697,-0.720230875706232,
31.376065476502));
#37487=CARTESIAN_POINT('Ctrl Pts',(4.77452965373889,1.78021451750611,31.4554373665553));
#37488=CARTESIAN_POINT('Ctrl Pts',(3.34153564775218,3.84700359469197,31.5348092566088));
#37489=CARTESIAN_POINT('Ctrl Pts',(1.09455095433672,4.97667111140894,31.6141811466621));
#37490=CARTESIAN_POINT('Ctrl Pts',(-1.41906392880775,4.89403256106132,31.6935530367156));
#37491=CARTESIAN_POINT('Ctrl Pts',(-3.58699797993935,3.61921851159646,31.772924926769));
#37492=CARTESIAN_POINT('Ctrl Pts',(-4.88114726284307,1.46277084371106,31.8522968168224));
#37493=CARTESIAN_POINT('Ctrl Pts',(-4.98625987675445,-1.05000456391402,
31.9316687068758));
#37494=CARTESIAN_POINT('Ctrl Pts',(-3.87673062158748,-3.30700118391536,
32.0110405969292));
#37495=CARTESIAN_POINT('Ctrl Pts',(-1.82283836799946,-4.75841963543788,
32.0904124869826));
#37496=CARTESIAN_POINT('Ctrl Pts',(0.675093277248947,-5.0506975963509,32.169784377036));
#37497=CARTESIAN_POINT('Ctrl Pts',(3.00857369445308,-4.11263680232238,32.2491562670894));
#37498=CARTESIAN_POINT('Ctrl Pts',(4.60917221905339,-2.17274678641531,32.3285281571428));
#37499=CARTESIAN_POINT('Ctrl Pts',(5.08698659332197,0.296419537369132,32.4079000471962));
#37500=CARTESIAN_POINT('Ctrl Pts',(4.32562229331115,2.69337871796399,32.4872719372496));
#37501=CARTESIAN_POINT('Ctrl Pts',(2.51054597725224,4.43423680455544,32.566643827303));
#37502=CARTESIAN_POINT('Ctrl Pts',(0.0839062181339619,5.09492462057391,
32.6460157173564));
#37503=CARTESIAN_POINT('Ctrl Pts',(-2.3631729099985,4.51450007644488,32.7253876074099));
#37504=CARTESIAN_POINT('Ctrl Pts',(-4.23458834804982,2.8343533063703,32.8047594974632));
#37505=CARTESIAN_POINT('Ctrl Pts',(-5.07446743761851,0.463764344598583,
32.8841313875167));
#37506=CARTESIAN_POINT('Ctrl Pts',(-4.67821749152652,-2.01979658499237,
32.96350327757));
#37507=CARTESIAN_POINT('Ctrl Pts',(-3.14236411955747,-4.01133953722311,
33.0428751676235));
#37508=CARTESIAN_POINT('Ctrl Pts',(-0.841037803569241,-5.02572905713579,
33.1222470576768));
#37509=CARTESIAN_POINT('Ctrl Pts',(1.6651634597629,-4.81586210299279,33.2016189477303));
#37510=CARTESIAN_POINT('Ctrl Pts',(3.76573459007359,-3.43286180029067,33.2809908377836));
#37511=CARTESIAN_POINT('Ctrl Pts',(4.94898110955447,-1.21362396154845,33.3603627278371));
#37512=CARTESIAN_POINT('Ctrl Pts',(4.92666678513176,1.3012499879159,33.4397346178904));
#37513=CARTESIAN_POINT('Ctrl Pts',(3.70422733684289,3.49914232059194,33.5191065079439));
#37514=CARTESIAN_POINT('Ctrl Pts',(1.5794463084672,4.8446513291919,33.5984783979973));
#37515=CARTESIAN_POINT('Ctrl Pts',(-0.930084344605925,5.01001399745455,
33.6778502880506));
#37516=CARTESIAN_POINT('Ctrl Pts',(-3.21304851003985,3.95494834541518,33.7572221781041));
#37517=CARTESIAN_POINT('Ctrl Pts',(-4.71332117039034,1.93646603056234,33.8365940681574));
#37518=CARTESIAN_POINT('Ctrl Pts',(-5.06543922639319,-0.553735123040657,
33.9159659582109));
#37519=CARTESIAN_POINT('Ctrl Pts',(-4.18362749900617,-2.90904762634284,
33.9953378482642));
#37520=CARTESIAN_POINT('Ctrl Pts',(-2.28269337316369,-4.55572256693558,
34.0747097383177));
#37521=CARTESIAN_POINT('Ctrl Pts',(0.174299805725373,-5.0926335741437,34.154081628371));
#37522=CARTESIAN_POINT('Ctrl Pts',(2.58883393774586,-4.38899031504365,34.2334535184245));
#37523=CARTESIAN_POINT('Ctrl Pts',(4.37273385281817,-2.61619873006421,34.3128254084779));
#37524=CARTESIAN_POINT('Ctrl Pts',(5.09144548022617,-0.206106925298799,
34.3921972985313));
#37525=CARTESIAN_POINT('Ctrl Pts',(4.56989225837449,2.25419207025942,34.4715691885847));
#37526=CARTESIAN_POINT('Ctrl Pts',(2.93512339766776,4.16537486707196,34.5509410786381));
#37527=CARTESIAN_POINT('Ctrl Pts',(0.585364974074578,5.06188156616671,34.6303129686915));
#37528=CARTESIAN_POINT('Ctrl Pts',(-1.9069870615198,4.72532512002801,34.7096848587449));
#37529=CARTESIAN_POINT('Ctrl Pts',(-3.93480126997218,3.23768993398022,34.7890567487983));
#37530=CARTESIAN_POINT('Ctrl Pts',(-5.00410659859424,0.961360646519953,
34.8684286388517));
#37531=CARTESIAN_POINT('Ctrl Pts',(-4.85442263620079,-1.54915396649689,
34.9478005289051));
#37532=CARTESIAN_POINT('Ctrl Pts',(-3.52221206471105,-3.68229810226921,
35.0271724189585));
#37533=CARTESIAN_POINT('Ctrl Pts',(-1.33199843054191,-4.91844257095733,
35.1065443090119));
#37534=CARTESIAN_POINT('Ctrl Pts',(1.1826870729787,-4.95646531614826,35.1859161990653));
#37535=CARTESIAN_POINT('Ctrl Pts',(3.40927262335516,-3.78710408127537,35.2652880891187));
#37536=CARTESIAN_POINT('Ctrl Pts',(4.80536690897926,-1.69521267481654,35.3446599791721));
#37537=CARTESIAN_POINT('Ctrl Pts',(5.03088445207529,0.809628786938043,35.4240318692255));
#37538=CARTESIAN_POINT('Ctrl Pts',(4.0308896783196,3.11724646827744,35.503403759279));
#37539=CARTESIAN_POINT('Ctrl Pts',(2.04897910114821,4.66550980985245,35.5827756493324));
#37540=CARTESIAN_POINT('Ctrl Pts',(-0.432058249724576,5.0772652886782,35.6621475393857));
#37541=CARTESIAN_POINT('Ctrl Pts',(-2.80784716730917,4.25221018151802,35.7415194294392));
#37542=CARTESIAN_POINT('Ctrl Pts',(-4.49965073000152,2.39132608624762,35.8208913194925));
#37543=CARTESIAN_POINT('Ctrl Pts',(-5.09534933467344,-0.052079750522149,
35.9002632095459));
#37544=CARTESIAN_POINT('Ctrl Pts',(-4.4498321197834,-2.48279907534128,35.9796350995994));
#37545=CARTESIAN_POINT('Ctrl Pts',(-2.72034565005043,-4.30871404098988,
36.0590069896527));
#37546=CARTESIAN_POINT('Ctrl Pts',(-0.328189001348134,-5.08503580343008,
36.1383788797062));
#37547=CARTESIAN_POINT('Ctrl Pts',(2.14391376164854,-4.62265409969052,36.2177507697596));
#37548=CARTESIAN_POINT('Ctrl Pts',(4.0937638777802,-3.03420408933768,36.2971226598129));
#37549=CARTESIAN_POINT('Ctrl Pts',(5.0463821746773,-0.706628678919033,36.3764945498664));
#37550=CARTESIAN_POINT('Ctrl Pts',(4.76971294380048,1.79307991358828,36.4558664399198));
#37551=CARTESIAN_POINT('Ctrl Pts',(3.33115219739438,3.85599820806056,36.5352383299732));
#37552=CARTESIAN_POINT('Ctrl Pts',(1.08113014908331,4.97960387415652,36.6146102200266));
#37553=CARTESIAN_POINT('Ctrl Pts',(-1.4322528105034,4.89018905867418,36.69398211008));
#37554=CARTESIAN_POINT('Ctrl Pts',(-3.59674215568932,3.60953501274872,36.7733540001334));
#37555=CARTESIAN_POINT('Ctrl Pts',(-4.88507307300309,1.44960622728788,36.8527258901868));
#37556=CARTESIAN_POINT('Ctrl Pts',(-4.98341100265913,-1.06344342649134,
36.9320977802402));
#37557=CARTESIAN_POINT('Ctrl Pts',(-3.86780104266052,-3.31744061546937,
37.0114696702936));
#37558=CARTESIAN_POINT('Ctrl Pts',(-1.81000330990226,-4.76331661354924,
37.090841560347));
#37559=CARTESIAN_POINT('Ctrl Pts',(0.688707222773825,-5.04885922799112,
37.1702134504005));
#37560=CARTESIAN_POINT('Ctrl Pts',(3.0196502004098,-4.10451090995456,37.2495853404537));
#37561=CARTESIAN_POINT('Ctrl Pts',(4.61501307310836,-2.16031281943414,37.3289572305073));
#37562=CARTESIAN_POINT('Ctrl Pts',(5.08616897635574,0.310132692129688,37.4083291205606));
#37563=CARTESIAN_POINT('Ctrl Pts',(4.31834537500717,2.70503056635669,37.4877010106141));
#37564=CARTESIAN_POINT('Ctrl Pts',(2.49858239880182,4.44098898210481,37.5670729006674));
#37565=CARTESIAN_POINT('Ctrl Pts',(0.0701702807674692,5.09513231177087,
37.6464447907209));
#37566=CARTESIAN_POINT('Ctrl Pts',(-2.37533516234416,4.50811268818063,37.7258166807742));
#37567=CARTESIAN_POINT('Ctrl Pts',(-4.2422142176209,2.82292679227449,37.8051885708277));
#37568=CARTESIAN_POINT('Ctrl Pts',(-5.07569927947281,0.450082178237795,
37.884560460881));
#37569=CARTESIAN_POINT('Ctrl Pts',(-4.67275523170413,-2.03240145822491,
37.9639323509345));
#37570=CARTESIAN_POINT('Ctrl Pts',(-3.13153835248091,-4.01979659801907,
38.0433042409878));
#37571=CARTESIAN_POINT('Ctrl Pts',(-0.827485662097561,-5.02797818437316,
38.1226761310413));
#37572=CARTESIAN_POINT('Ctrl Pts',(1.6781407038918,-4.81135541393667,38.2020480210947));
#37573=CARTESIAN_POINT('Ctrl Pts',(3.77497570905148,-3.42269711502072,38.281419911148));
#37574=CARTESIAN_POINT('Ctrl Pts',(4.95223498699472,-1.20027737376265,38.3607918012015));
#37575=CARTESIAN_POINT('Ctrl Pts',(4.92314078418044,1.31452727683269,38.4401636912548));
#37576=CARTESIAN_POINT('Ctrl Pts',(3.69478038260533,3.50911599649374,38.5195355813083));
#37577=CARTESIAN_POINT('Ctrl Pts',(1.56637965982565,4.8488918190669,38.5989074713616));
#37578=CARTESIAN_POINT('Ctrl Pts',(-0.943587684251231,5.00748834177839,
38.6782793614151));
#37579=CARTESIAN_POINT('Ctrl Pts',(-3.22369915083517,3.94627176108658,38.7576512514684));
#37580=CARTESIAN_POINT('Ctrl Pts',(-4.71852465152966,1.92375216574096,38.8370231415219));
#37581=CARTESIAN_POINT('Ctrl Pts',(-5.06392796926474,-0.567389296122155,
38.9163950315753));
#37582=CARTESIAN_POINT('Ctrl Pts',(-4.17576968427578,-2.92031579800749,
38.9957669216287));
#37583=CARTESIAN_POINT('Ctrl Pts',(-2.27040306822808,-4.56186018168572,
39.0751388116821));
#37584=CARTESIAN_POINT('Ctrl Pts',(0.188028560849278,-5.0921448689568,39.1545107017355));
#37585=CARTESIAN_POINT('Ctrl Pts',(2.60065712992459,-4.38199557165452,39.2338825917889));
#37586=CARTESIAN_POINT('Ctrl Pts',(4.37977084759398,-2.60439952199669,39.3132544818424));
#37587=CARTESIAN_POINT('Ctrl Pts',(5.091983083909,-0.192381913948899,39.3926263718957));
#37588=CARTESIAN_POINT('Ctrl Pts',(4.56379761866661,2.26650781142318,39.4719982619492));
#37589=CARTESIAN_POINT('Ctrl Pts',(2.92388473013463,4.17326556172555,39.5513701520025));
#37590=CARTESIAN_POINT('Ctrl Pts',(0.571713243107522,5.06345468357226,39.6307420420559));
#37591=CARTESIAN_POINT('Ctrl Pts',(-1.91971357759784,4.72014150668349,39.7101139321093));
#37592=CARTESIAN_POINT('Ctrl Pts',(-3.94352649879586,3.22711800485078,39.7894858221628));
#37593=CARTESIAN_POINT('Ctrl Pts',(-5.00665954563271,0.947775616877117,
39.8688577122161));
#37594=CARTESIAN_POINT('Ctrl Pts',(-4.85026808817391,-1.56206090154421,
39.9482296022695));
#37595=CARTESIAN_POINT('Ctrl Pts',(-3.51219281059473,-3.69213734276829,
40.027601492323));
#37596=CARTESIAN_POINT('Ctrl Pts',(-2.05001543279097,-4.51147638686035,
40.0805160856919));
#37597=CARTESIAN_POINT('Ctrl Pts',(-1.2650852794273,-4.72177922709094,40.1069733823764));
#37598=CARTESIAN_POINT('Ctrl Pts',(-3.8562705385024,3.29705846079174,-0.320920147129055));
#37599=CARTESIAN_POINT('Ctrl Pts',(-4.40436067122819,2.6560070944272,-0.294462850444587));
#37600=CARTESIAN_POINT('Ctrl Pts',(-5.17416686787623,1.09598291074317,-0.241548257075651));
#37601=CARTESIAN_POINT('Ctrl Pts',(-5.06779668194698,-1.512680812799,-0.162176367022247));
#37602=CARTESIAN_POINT('Ctrl Pts',(-3.72722085031348,-3.75211381890485,
-0.0828044769688437));
#37603=CARTESIAN_POINT('Ctrl Pts',(-1.47855208449991,-5.07791790908896,
-0.00343258691543986));
#37604=CARTESIAN_POINT('Ctrl Pts',(1.1302101318597,-5.16655447652177,0.0759393031379633));
#37605=CARTESIAN_POINT('Ctrl Pts',(3.46369715057722,-3.99673439595713,0.155311193191368));
#37606=CARTESIAN_POINT('Ctrl Pts',(4.95341325213432,-1.85326330477546,0.23468308324477));
#37607=CARTESIAN_POINT('Ctrl Pts',(5.23650047694814,0.741629311098527,0.314054973298175));
#37608=CARTESIAN_POINT('Ctrl Pts',(4.24398161873799,3.15587819282154,0.393426863351577));
#37609=CARTESIAN_POINT('Ctrl Pts',(2.21764149317933,4.80135391043019,0.472798753404982));
#37610=CARTESIAN_POINT('Ctrl Pts',(-0.348912918530393,5.27723479734493,
0.552170643458385));
#37611=CARTESIAN_POINT('Ctrl Pts',(-2.83047200092439,4.46759066254957,0.631542533511789));
#37612=CARTESIAN_POINT('Ctrl Pts',(-4.62253485344812,2.56965255248809,0.710914423565193));
#37613=CARTESIAN_POINT('Ctrl Pts',(-5.28855819093304,0.045752121671659,
0.790286313618596));
#37614=CARTESIAN_POINT('Ctrl Pts',(-4.66630059499956,-2.48929308216644,
0.869658203672));
#37615=CARTESIAN_POINT('Ctrl Pts',(-2.90734243084918,-4.4179521825598,0.949030093725403));
#37616=CARTESIAN_POINT('Ctrl Pts',(-0.440162123945536,-5.27040781417518,
1.02840198377881));
#37617=CARTESIAN_POINT('Ctrl Pts',(2.1342407222512,-4.83900381899044,1.10777387383221));
#37618=CARTESIAN_POINT('Ctrl Pts',(4.18874724188064,-3.228829177505,1.18714576388562));
#37619=CARTESIAN_POINT('Ctrl Pts',(5.22288421068343,-0.832118909543204,
1.26651765393902));
#37620=CARTESIAN_POINT('Ctrl Pts',(4.98473814342391,1.76729369047769,1.34588954399242));
#37621=CARTESIAN_POINT('Ctrl Pts',(3.53232089954478,3.93619745533352,1.42526143404583));
#37622=CARTESIAN_POINT('Ctrl Pts',(1.21943810235538,5.14625223481536,1.50463332409923));
#37623=CARTESIAN_POINT('Ctrl Pts',(-1.39049711694202,5.10269135980955,1.58400521415263));
#37624=CARTESIAN_POINT('Ctrl Pts',(-3.66171031660135,3.81612616476449,1.66337710420604));
#37625=CARTESIAN_POINT('Ctrl Pts',(-5.04093898807,1.59996108251987,1.74274899425944));
#37626=CARTESIAN_POINT('Ctrl Pts',(-5.19220608004013,-1.00595097780601,
1.82212088431284));
#37627=CARTESIAN_POINT('Ctrl Pts',(-4.07866326363067,-3.3668156066614,1.90149277436625));
#37628=CARTESIAN_POINT('Ctrl Pts',(-1.97156710418735,-4.90753140600723,
1.98086466441965));
#37629=CARTESIAN_POINT('Ctrl Pts',(0.61579843785608,-5.25278341751101,2.06023655447306));
#37630=CARTESIAN_POINT('Ctrl Pts',(3.0531568434793,-4.31846901533485,2.13960844452646));
#37631=CARTESIAN_POINT('Ctrl Pts',(4.74677300008174,-2.3321851197991,2.21898033457986));
#37632=CARTESIAN_POINT('Ctrl Pts',(5.28408576066664,0.222213908719184,2.29835222463327));
#37633=CARTESIAN_POINT('Ctrl Pts',(4.53420692607935,2.72248212093367,2.37772411468667));
#37634=CARTESIAN_POINT('Ctrl Pts',(2.67980532059554,4.5595597146017,2.45709600474007));
#37635=CARTESIAN_POINT('Ctrl Pts',(0.172609070663326,5.28593865420646,2.53646789479348));
#37636=CARTESIAN_POINT('Ctrl Pts',(-2.37663436681889,4.72467463787357,2.61583978484688));
#37637=CARTESIAN_POINT('Ctrl Pts',(-4.34693493313492,3.01249033764445,2.69521167490029));
#37638=CARTESIAN_POINT('Ctrl Pts',(-5.25833177151656,0.56647005919948,2.77458356495369));
#37639=CARTESIAN_POINT('Ctrl Pts',(-4.88881062947673,-2.01754107180632,
2.85395545500709));
#37640=CARTESIAN_POINT('Ctrl Pts',(-3.32838603929513,-4.11008366347149,
2.93332734506049));
#37641=CARTESIAN_POINT('Ctrl Pts',(-0.957173977198773,-5.20141897223089,
3.0126992351139));
#37642=CARTESIAN_POINT('Ctrl Pts',(1.64720354707453,-5.02570013250045,3.0920711251673));
#37643=CARTESIAN_POINT('Ctrl Pts',(3.85032593330369,-3.62573186469146,3.1714430152207));
#37644=CARTESIAN_POINT('Ctrl Pts',(5.11551744473197,-1.342543340065,3.25081490527411));
#37645=CARTESIAN_POINT('Ctrl Pts',(5.13458022962935,1.26768577053204,3.33018679532751));
#37646=CARTESIAN_POINT('Ctrl Pts',(3.90287063578958,3.56910943340232,3.40955868538091));
#37647=CARTESIAN_POINT('Ctrl Pts',(1.7204303939291,5.00110593838552,3.48893057543432));
#37648=CARTESIAN_POINT('Ctrl Pts',(-0.881102883784432,5.21484410653825,
3.56830246548772));
#37649=CARTESIAN_POINT('Ctrl Pts',(-3.26800144929621,4.15825779319991,3.64767435554113));
#37650=CARTESIAN_POINT('Ctrl Pts',(-4.85882209535798,2.08872908558557,3.72704624559453));
#37651=CARTESIAN_POINT('Ctrl Pts',(-5.2660444338108,-0.489609403954008,
3.80641813564793));
#37652=CARTESIAN_POINT('Ctrl Pts',(-4.39047000437897,-2.94868012642242,
3.88579002570134));
#37653=CARTESIAN_POINT('Ctrl Pts',(-2.44538680002092,-4.68945889688708,
3.96516191575474));
#37654=CARTESIAN_POINT('Ctrl Pts',(0.0953872160503347,-5.28789586001125,
4.04453380580815));
#37655=CARTESIAN_POINT('Ctrl Pts',(2.61292511742776,-4.59821309619564,4.12390569586154));
#37656=CARTESIAN_POINT('Ctrl Pts',(4.49396024381142,-2.78841580011883,4.20327758591496));
#37657=CARTESIAN_POINT('Ctrl Pts',(5.28027660201492,-0.299366587186749,
4.28264947596836));
#37658=CARTESIAN_POINT('Ctrl Pts',(4.78032926766157,2.26260766374733,4.36202136602176));
#37659=CARTESIAN_POINT('Ctrl Pts',(3.11590430478523,4.27341569598967,4.44139325607517));
#37660=CARTESIAN_POINT('Ctrl Pts',(0.692451950200399,5.24322912373411,4.52076514612856));
#37661=CARTESIAN_POINT('Ctrl Pts',(-1.89968016673685,4.93580354262775,4.60013703618198));
#37662=CARTESIAN_POINT('Ctrl Pts',(-4.02905439992773,3.42602714375309,4.67950892623537));
#37663=CARTESIAN_POINT('Ctrl Pts',(-5.17695989945686,1.08167811604265,4.75888081628878));
#37664=CARTESIAN_POINT('Ctrl Pts',(-5.06376942648468,-1.5261653064819,4.83825270634218));
#37665=CARTESIAN_POINT('Ctrl Pts',(-3.71705592968434,-3.76223823845706,
4.91762459639559));
#37666=CARTESIAN_POINT('Ctrl Pts',(-1.46487583597662,-5.08183826311717,
4.996996486449));
#37667=CARTESIAN_POINT('Ctrl Pts',(1.14414476892732,-5.16351373534013,5.07636837650239));
#37668=CARTESIAN_POINT('Ctrl Pts',(3.47445424064207,-3.98736869087803,5.15574026655581));
#37669=CARTESIAN_POINT('Ctrl Pts',(4.95839434991041,-1.83990945920892,5.2351121566092));
#37670=CARTESIAN_POINT('Ctrl Pts',(5.23448057076031,0.75574764415296,5.31448404666261));
#37671=CARTESIAN_POINT('Ctrl Pts',(4.23545891089922,3.1673062942182,5.39385593671601));
#37672=CARTESIAN_POINT('Ctrl Pts',(2.20468883537238,4.80731614172549,5.47322782676942));
#37673=CARTESIAN_POINT('Ctrl Pts',(-0.363138560455233,5.27627441792221,
5.55259971682281));
#37674=CARTESIAN_POINT('Ctrl Pts',(-2.84250620674952,4.45994392474844,5.63197160687622));
#37675=CARTESIAN_POINT('Ctrl Pts',(-4.62944563286038,2.55718096342436,5.71134349692963));
#37676=CARTESIAN_POINT('Ctrl Pts',(-5.28866234991055,0.0314943796341776,
5.79071538698302));
#37677=CARTESIAN_POINT('Ctrl Pts',(-4.65957262477808,-2.50186416532327,
5.87008727703643));
#37678=CARTESIAN_POINT('Ctrl Pts',(-2.89542132203872,-4.42577413739037,
5.94945916708984));
#37679=CARTESIAN_POINT('Ctrl Pts',(-0.425951794157121,-5.27157532587407,
6.02883105714324));
#37680=CARTESIAN_POINT('Ctrl Pts',(2.14727864795285,-4.8332324334089,6.10820294719664));
#37681=CARTESIAN_POINT('Ctrl Pts',(4.19743676434218,-3.21752481834385,6.18757483725004));
#37682=CARTESIAN_POINT('Ctrl Pts',(5.22510857580644,-0.81803527940062,6.26694672730345));
#37683=CARTESIAN_POINT('Ctrl Pts',(4.97995550378589,1.78072584291422,6.34631861735685));
#37684=CARTESIAN_POINT('Ctrl Pts',(3.52169629398765,3.94570609146495,6.42569050741027));
#37685=CARTESIAN_POINT('Ctrl Pts',(1.20555966211655,5.14952106980711,6.50506239746365));
#37686=CARTESIAN_POINT('Ctrl Pts',(-1.40424863498509,5.09892411381582,6.58443428751707));
#37687=CARTESIAN_POINT('Ctrl Pts',(-3.67198507285601,3.80624052997609,6.66380617757046));
#37688=CARTESIAN_POINT('Ctrl Pts',(-5.04523407478029,1.58636517800468,6.74317806762388));
#37689=CARTESIAN_POINT('Ctrl Pts',(-5.1894752235243,-1.01994521996889,6.82254995767727));
#37690=CARTESIAN_POINT('Ctrl Pts',(-4.06957169452636,-3.37779921996849,
6.90192184773068));
#37691=CARTESIAN_POINT('Ctrl Pts',(-1.95832950858598,-4.91282880661553,
6.98129373778407));
#37692=CARTESIAN_POINT('Ctrl Pts',(0.629957410957137,-5.25110417033315,
7.06066562783749));
#37693=CARTESIAN_POINT('Ctrl Pts',(3.06478809957816,-4.31022218127953,7.14003751789089));
#37694=CARTESIAN_POINT('Ctrl Pts',(4.75304319093534,-2.31937960938119,7.21940940794429));
#37695=CARTESIAN_POINT('Ctrl Pts',(5.28346748166331,0.236458701502723,7.2987812979977));
#37696=CARTESIAN_POINT('Ctrl Pts',(4.52685078861501,2.73469619609302,7.37815318805109));
#37697=CARTESIAN_POINT('Ctrl Pts',(2.66750326347436,4.56676775046241,7.45752507810451));
#37698=CARTESIAN_POINT('Ctrl Pts',(0.158357847769689,5.28638478918814,7.5368969681579));
#37699=CARTESIAN_POINT('Ctrl Pts',(-2.38936318913255,4.71825019448189,7.61626885821132));
#37700=CARTESIAN_POINT('Ctrl Pts',(-4.3550406419278,3.0007602960695,7.69564074826471));
#37701=CARTESIAN_POINT('Ctrl Pts',(-5.25983983406839,0.552291831604834,
7.77501263831812));
#37702=CARTESIAN_POINT('Ctrl Pts',(-4.88335368508791,-2.03071370056153,
7.85438452837152));
#37703=CARTESIAN_POINT('Ctrl Pts',(-3.31729338754006,-4.11904187017964,
7.93375641842492));
#37704=CARTESIAN_POINT('Ctrl Pts',(-0.943147763491834,-5.20398055756651,
8.01312830847834));
#37705=CARTESIAN_POINT('Ctrl Pts',(1.66074656812082,-5.02124109994579,8.09250019853171));
#37706=CARTESIAN_POINT('Ctrl Pts',(3.86008671173945,-3.61533842470695,8.17187208858515));
#37707=CARTESIAN_POINT('Ctrl Pts',(5.11911827653537,-1.32874731162534,8.25124397863853));
#37708=CARTESIAN_POINT('Ctrl Pts',(5.13114396014337,1.28152370543593,8.33061586869195));
#37709=CARTESIAN_POINT('Ctrl Pts',(3.89323433265495,3.57961838445758,8.40998775874535));
#37710=CARTESIAN_POINT('Ctrl Pts',(1.70694143925982,5.00572594837628,8.48935964879875));
#37711=CARTESIAN_POINT('Ctrl Pts',(-0.895158610488236,5.21244975125697,
8.56873153885215));
#37712=CARTESIAN_POINT('Ctrl Pts',(-3.27920000412133,4.14943233229326,8.64810342890557));
#37713=CARTESIAN_POINT('Ctrl Pts',(-4.86443553513654,2.0756223817956,8.72747531895896));
#37714=CARTESIAN_POINT('Ctrl Pts',(-5.26470533703792,-0.503804586595236,
8.80684720901237));
#37715=CARTESIAN_POINT('Ctrl Pts',(-4.38250457206448,-2.96050587284403,
8.88621909906576));
#37716=CARTESIAN_POINT('Ctrl Pts',(-2.43273539384546,-4.69603448143659,
8.96559098911917));
#37717=CARTESIAN_POINT('Ctrl Pts',(0.109642741545844,-5.28761948484726,
9.04496287917257));
#37718=CARTESIAN_POINT('Ctrl Pts',(2.62531214778668,-4.59115208569632,9.12433476922599));
#37719=CARTESIAN_POINT('Ctrl Pts',(4.50146132585655,-2.77629020081255,9.20370665927937));
#37720=CARTESIAN_POINT('Ctrl Pts',(5.28106448876342,-0.285130168224959,
9.28307854933281));
#37721=CARTESIAN_POINT('Ctrl Pts',(4.77421203164548,2.27548694221733,9.36245043938617));
#37722=CARTESIAN_POINT('Ctrl Pts',(3.10437209115777,4.28180047024037,9.44182232943961));
#37723=CARTESIAN_POINT('Ctrl Pts',(0.67831398067512,5.24507688131743,9.52119421949299));
#37724=CARTESIAN_POINT('Ctrl Pts',(-1.91297991407746,4.93066417388633,9.6005661095464));
#37725=CARTESIAN_POINT('Ctrl Pts',(-4.03827613607002,3.41515258753654,9.6799379995998));
#37726=CARTESIAN_POINT('Ctrl Pts',(-5.1798572298885,1.06771739017486,9.75930988965322));
#37727=CARTESIAN_POINT('Ctrl Pts',(-5.05963656792565,-1.53981140008104,
9.8386817797066));
#37728=CARTESIAN_POINT('Ctrl Pts',(-3.70689963733171,-3.77224554159189,
9.91805366976003));
#37729=CARTESIAN_POINT('Ctrl Pts',(-1.45117016016697,-5.08576901889487,
9.99742555981341));
#37730=CARTESIAN_POINT('Ctrl Pts',(1.1580611559038,-5.16041042035386,10.0767974498668));
#37731=CARTESIAN_POINT('Ctrl Pts',(3.48519133772131,-3.97798726578937,10.1561693399202));
#37732=CARTESIAN_POINT('Ctrl Pts',(4.96333662401008,-1.82653521840402,10.2355412299736));
#37733=CARTESIAN_POINT('Ctrl Pts',(5.23242409484924,0.769856765217389,10.314913120027));
#37734=CARTESIAN_POINT('Ctrl Pts',(4.22690463795744,3.1787133448809,10.3942850100804));
#37735=CARTESIAN_POINT('Ctrl Pts',(2.1917205673539,4.81324238969408,10.4736569001339));
#37736=CARTESIAN_POINT('Ctrl Pts',(-0.377361782165876,5.27527624230907,
10.5530287901872));
#37737=CARTESIAN_POINT('Ctrl Pts',(-2.85451963682615,4.45226447892349,10.6324006802407));
#37738=CARTESIAN_POINT('Ctrl Pts',(-4.63632282632763,2.54469094339242,10.711772570294));
#37739=CARTESIAN_POINT('Ctrl Pts',(-5.28872803766221,0.0172363266288179,
10.7911444603475));
#37740=CARTESIAN_POINT('Ctrl Pts',(-4.65281080542322,-2.5144170211496,10.8705163504009));
#37741=CARTESIAN_POINT('Ctrl Pts',(-2.88347915980519,-4.43356394814365,
10.9498882404543));
#37742=CARTESIAN_POINT('Ctrl Pts',(-0.411738373331464,-5.27270451089727,
11.0292601305077));
#37743=CARTESIAN_POINT('Ctrl Pts',(2.16030096951836,-4.82742592572977,11.1086320205611));
#37744=CARTESIAN_POINT('Ctrl Pts',(4.20609577793862,-3.20619707038057,11.1880039106145));
#37745=CARTESIAN_POINT('Ctrl Pts',(5.22729496488813,-0.803945705483474,
11.2673758006679));
#37746=CARTESIAN_POINT('Ctrl Pts',(4.975136668812,1.79414505376576,11.3467476907213));
#37747=CARTESIAN_POINT('Ctrl Pts',(3.51104609249152,3.95518604919035,11.4261195807747));
#37748=CARTESIAN_POINT('Ctrl Pts',(1.19167245960881,5.152752477688,11.5054914708281));
#37749=CARTESIAN_POINT('Ctrl Pts',(-1.41798994671238,5.09511980804502,11.5848633608815));
#37750=CARTESIAN_POINT('Ctrl Pts',(-3.68223314068194,3.79632723101863,11.6642352509349));
#37751=CARTESIAN_POINT('Ctrl Pts',(-5.04949249206616,1.57275774354392,11.7436071409883));
#37752=CARTESIAN_POINT('Ctrl Pts',(-5.18670664924514,-1.03393204901786,
11.8229790310417));
#37753=CARTESIAN_POINT('Ctrl Pts',(-4.06045054724843,-3.38875828300867,
11.9023509210951));
#37754=CARTESIAN_POINT('Ctrl Pts',(-1.94507767959685,-4.91809050014781,
11.9817228111485));
#37755=CARTESIAN_POINT('Ctrl Pts',(0.644111805448097,-5.24938675745961,
12.0610947012019));
#37756=CARTESIAN_POINT('Ctrl Pts',(3.0763970804032,-4.30194401997477,12.1404665912553));
#37757=CARTESIAN_POINT('Ctrl Pts',(4.7592788360615,-2.30655724141565,12.2198384813087));
#37758=CARTESIAN_POINT('Ctrl Pts',(5.28281080174027,0.250701775674464,12.2992103713621));
#37759=CARTESIAN_POINT('Ctrl Pts',(4.51946174941847,2.74689039512926,12.3785822614155));
#37760=CARTESIAN_POINT('Ctrl Pts',(2.6551818185972,4.57394259446934,12.4579541514689));
#37761=CARTESIAN_POINT('Ctrl Pts',(0.144105473910954,5.28679250204684,12.5373260415223));
#37762=CARTESIAN_POINT('Ctrl Pts',(-2.40207464524796,4.7117914582425,12.6166979315757));
#37763=CARTESIAN_POINT('Ctrl Pts',(-4.36311469772651,2.98900844458373,12.6960698216291));
#37764=CARTESIAN_POINT('Ctrl Pts',(-5.26130966742946,0.538109589882336,
12.7754417116825));
#37765=CARTESIAN_POINT('Ctrl Pts',(-4.87786124785798,-2.043871569829,12.854813601736));
#37766=CARTESIAN_POINT('Ctrl Pts',(-3.30617662527107,-4.12797013916298,
12.9341854917893));
#37767=CARTESIAN_POINT('Ctrl Pts',(-0.929114694865931,-5.20650431970379,
13.0135573818428));
#37768=CARTESIAN_POINT('Ctrl Pts',(1.67427751864803,-5.01674557236658,13.0929292718962));
#37769=CARTESIAN_POINT('Ctrl Pts',(3.86981943456978,-3.60491870797887,13.1723011619496));
#37770=CARTESIAN_POINT('Ctrl Pts',(5.12268190193035,-1.31494162567972,13.251673052003));
#37771=CARTESIAN_POINT('Ctrl Pts',(5.12767039684476,1.29535232606109,13.3310449420564));
#37772=CARTESIAN_POINT('Ctrl Pts',(3.8835697329937,3.59010131838716,13.4104168321098));
#37773=CARTESIAN_POINT('Ctrl Pts',(1.69344007832116,5.01030957610862,13.4897887221632));
#37774=CARTESIAN_POINT('Ctrl Pts',(-0.909207831064397,5.21001751122212,
13.5691606122166));
#37775=CARTESIAN_POINT('Ctrl Pts',(-3.29037472530003,4.14057671278008,13.64853250227));
#37776=CARTESIAN_POINT('Ctrl Pts',(-4.87001361957351,2.06250059211591,13.7279043923234));
#37777=CARTESIAN_POINT('Ctrl Pts',(-5.26332797571119,-0.517996107520081,
13.8072762823768));
#37778=CARTESIAN_POINT('Ctrl Pts',(-4.37450728714447,-2.97231010192914,
13.8866481724302));
#37779=CARTESIAN_POINT('Ctrl Pts',(-2.420066306237,-4.70257593460501,13.9660200624836));
#37780=CARTESIAN_POINT('Ctrl Pts',(0.123897470143854,-5.28730467858643,
14.045391952537));
#37781=CARTESIAN_POINT('Ctrl Pts',(2.63768009704007,-4.58405770611459,14.1247638425904));
#37782=CARTESIAN_POINT('Ctrl Pts',(4.50892969070322,-2.76414442307289,14.2041357326438));
#37783=CARTESIAN_POINT('Ctrl Pts',(5.28181399205766,-0.270891676900501,
14.2835076226972));
#37784=CARTESIAN_POINT('Ctrl Pts',(4.7680600960438,2.28834968215629,14.3628795127506));
#37785=CARTESIAN_POINT('Ctrl Pts',(3.09281731455568,4.29015412381589,14.442251402804));
#37786=CARTESIAN_POINT('Ctrl Pts',(0.664171081076821,5.24688651700904,14.5216232928574));
#37787=CARTESIAN_POINT('Ctrl Pts',(-1.92626575763464,4.9254889684451,14.6009951829108));
#37788=CARTESIAN_POINT('Ctrl Pts',(-4.04746852150321,3.4042532095528,14.6803670729642));
#37789=CARTESIAN_POINT('Ctrl Pts',(-5.1827169124532,1.05374890400015,14.7597389630177));
#37790=CARTESIAN_POINT('Ctrl Pts',(-5.05546693527891,-1.55344630213332,
14.839110853071));
#37791=CARTESIAN_POINT('Ctrl Pts',(-3.69671640275692,-3.78222542756219,
14.9184827431245));
#37792=CARTESIAN_POINT('Ctrl Pts',(-1.43745393706629,-5.08966281065088,
14.9978546331779));
#37793=CARTESIAN_POINT('Ctrl Pts',(1.17196912594334,-5.15726959884254,15.0772265232312));
#37794=CARTESIAN_POINT('Ctrl Pts',(3.49590310398282,-3.96857692817882,15.1565984132847));
#37795=CARTESIAN_POINT('Ctrl Pts',(4.96824282394235,-1.81314770210679,15.2359703033381));
#37796=CARTESIAN_POINT('Ctrl Pts',(5.23032958900857,0.783960290864088,15.3153421933915));
#37797=CARTESIAN_POINT('Ctrl Pts',(4.21831964333036,3.19009729224721,15.3947140834449));
#37798=CARTESIAN_POINT('Ctrl Pts',(2.17873636962922,4.81913365439941,15.4740859734983));
#37799=CARTESIAN_POINT('Ctrl Pts',(-0.391582261162836,5.27423972531144,
15.5534578635517));
#37800=CARTESIAN_POINT('Ctrl Pts',(-2.86651231988745,4.44455267346898,15.6328297536051));
#37801=CARTESIAN_POINT('Ctrl Pts',(-4.64316632240643,2.53218242822043,15.7122016436585));
#37802=CARTESIAN_POINT('Ctrl Pts',(-5.28875528625864,0.00297814834715876,
15.7915735337119));
#37803=CARTESIAN_POINT('Ctrl Pts',(-4.64601516884489,-2.52695160186966,
15.8709454237653));
#37804=CARTESIAN_POINT('Ctrl Pts',(-2.87151604007055,-4.44132153518687,
15.9503173138187));
#37805=CARTESIAN_POINT('Ctrl Pts',(-0.397521959947054,-5.27379537322474,
16.0296892038721));
#37806=CARTESIAN_POINT('Ctrl Pts',(2.1733075897557,-4.82158433170501,16.1090610939255));
#37807=CARTESIAN_POINT('Ctrl Pts',(4.21472422106055,-3.1948460193553,16.1884329839789));
#37808=CARTESIAN_POINT('Ctrl Pts',(5.22944336137754,-0.789850288404984,
16.2678048740323));
#37809=CARTESIAN_POINT('Ctrl Pts',(4.97028167379658,1.80755122457726,16.3471767640857));
#37810=CARTESIAN_POINT('Ctrl Pts',(3.50037037246945,3.9646372600474,16.4265486541391));
#37811=CARTESIAN_POINT('Ctrl Pts',(1.17777659548083,5.15594643483254,16.5059205441925));
#37812=CARTESIAN_POINT('Ctrl Pts',(-1.43172095156687,5.09127847004474,16.5852924342459));
#37813=CARTESIAN_POINT('Ctrl Pts',(-3.69245444696213,3.78638634033038,16.6646643242993));
#37814=CARTESIAN_POINT('Ctrl Pts',(-5.05371420635461,1.5591388772047,16.7440362143527));
#37815=CARTESIAN_POINT('Ctrl Pts',(-5.18390038229795,-1.04791136166686,
16.8234081044061));
#37816=CARTESIAN_POINT('Ctrl Pts',(-4.05129987868913,-3.39969271923294,
16.9027799944595));
#37817=CARTESIAN_POINT('Ctrl Pts',(-1.93181173129365,-4.9233164424874,16.9821518845129));
#37818=CARTESIAN_POINT('Ctrl Pts',(0.658261551986501,-5.24763120247215,
17.0615237745663));
#37819=CARTESIAN_POINT('Ctrl Pts',(3.08798363825942,-4.29363457062506,17.1408956646198));
#37820=CARTESIAN_POINT('Ctrl Pts',(4.76548000969996,-2.29371814868002,17.2202675546731));
#37821=CARTESIAN_POINT('Ctrl Pts',(5.28211549991427,0.264943102456271,17.2996394447266));
#37822=CARTESIAN_POINT('Ctrl Pts',(4.51204028846775,2.7590644882845,17.3790113347799));
#37823=CARTESIAN_POINT('Ctrl Pts',(2.64284027062647,4.58108446095533,17.4583832248334));
#37824=CARTESIAN_POINT('Ctrl Pts',(0.129853572473924,5.28716128664959,17.5377551148867));
#37825=CARTESIAN_POINT('Ctrl Pts',(-2.41477151246584,4.70529942618515,17.6171270049402));
#37826=CARTESIAN_POINT('Ctrl Pts',(-4.37115162329109,2.9772330746438,17.6964988949936));
#37827=CARTESIAN_POINT('Ctrl Pts',(-5.2627514922539,0.523926824466488,17.775870785047));
#37828=CARTESIAN_POINT('Ctrl Pts',(-4.87231403886184,-2.05702097999283,
17.8552426751004));
#37829=CARTESIAN_POINT('Ctrl Pts',(-3.29507231119166,-4.13685632854999,
17.9346145651538));
#37830=CARTESIAN_POINT('Ctrl Pts',(-0.915005995631555,-5.20901304408194,
18.0139864552072));
#37831=CARTESIAN_POINT('Ctrl Pts',(1.68766624540468,-5.01217052435341,18.0933583452606));
#37832=CARTESIAN_POINT('Ctrl Pts',(3.8797695997979,-3.59455409188004,18.172730235314));
#37833=CARTESIAN_POINT('Ctrl Pts',(5.12574462250332,-1.30097287489382,18.2521021253674));
#37834=CARTESIAN_POINT('Ctrl Pts',(5.12503498129813,1.3088817301615,18.3314740154208));
#37835=CARTESIAN_POINT('Ctrl Pts',(3.87222469260764,3.60110493868871,18.4108459054742));
#37836=CARTESIAN_POINT('Ctrl Pts',(1.68303999757325,5.01382783115876,18.4902177955276));
#37837=CARTESIAN_POINT('Ctrl Pts',(-0.929079443196312,5.2094618875472,18.569589685581));
#37838=CARTESIAN_POINT('Ctrl Pts',(-3.29092685490746,4.12830747359753,18.6489615756344));
#37839=CARTESIAN_POINT('Ctrl Pts',(-5.42625155540715,1.36247937795741,18.7547907623723));
#37840=CARTESIAN_POINT('Ctrl Pts',(-4.95432466322409,-3.37745298000962,
18.8870772457946));
#37841=CARTESIAN_POINT('Ctrl Pts',(0.158509478955228,-5.99736559883162,
19.0458210259014));
#37842=CARTESIAN_POINT('Ctrl Pts',(5.11967904485094,-3.11863163173532,19.2045648060083));
#37843=CARTESIAN_POINT('Ctrl Pts',(5.39954635636598,2.60828838171404,19.363308586115));
#37844=CARTESIAN_POINT('Ctrl Pts',(0.736723079475925,5.95134306184737,19.5220523662219));
#37845=CARTESIAN_POINT('Ctrl Pts',(-4.59927593805429,3.84720861430001,19.6807961463287));
#37846=CARTESIAN_POINT('Ctrl Pts',(-5.72720375155086,-1.77677009197966,
19.8395399264355));
#37847=CARTESIAN_POINT('Ctrl Pts',(-1.61419617037545,-5.77483540889735,
19.9982837065423));
#37848=CARTESIAN_POINT('Ctrl Pts',(3.97578039972893,-4.48936692070975,20.1570274866491));
#37849=CARTESIAN_POINT('Ctrl Pts',(5.92771323046147,0.905806267444479,20.3157712667559));
#37850=CARTESIAN_POINT('Ctrl Pts',(2.45559119020176,5.46873373673919,20.4745150468627));
#37851=CARTESIAN_POINT('Ctrl Pts',(-3.26379011618977,5.03400372054189,20.6332588269695));
#37852=CARTESIAN_POINT('Ctrl Pts',(-5.99600976813329,-0.0197068834827358,
20.7920026070763));
#37853=CARTESIAN_POINT('Ctrl Pts',(-3.70230252414087,-4.19446206534972,
20.9242890904987));
#37854=CARTESIAN_POINT('Ctrl Pts',(-0.376480053418488,-5.26605971579228,
21.0301182772365));
#37855=CARTESIAN_POINT('Ctrl Pts',(2.18257651229242,-4.8205851862161,21.10949016729));
#37856=CARTESIAN_POINT('Ctrl Pts',(4.22530652207796,-3.18086119603153,21.1888620573433));
#37857=CARTESIAN_POINT('Ctrl Pts',(5.23050112077121,-0.777135043026565,
21.2682339473968));
#37858=CARTESIAN_POINT('Ctrl Pts',(4.96594823061178,1.82167865277159,21.3476058374501));
#37859=CARTESIAN_POINT('Ctrl Pts',(3.48937383888172,3.97367066688458,21.4269777275036));
#37860=CARTESIAN_POINT('Ctrl Pts',(1.16402860508423,5.15930893371516,21.5063496175569));
#37861=CARTESIAN_POINT('Ctrl Pts',(-1.44552439996815,5.08729102078623,21.5857215076104));
#37862=CARTESIAN_POINT('Ctrl Pts',(-3.70260503654192,3.77647571272897,21.6650933976637));
#37863=CARTESIAN_POINT('Ctrl Pts',(-5.057922432142,1.54547807796832,21.7444652877172));
#37864=CARTESIAN_POINT('Ctrl Pts',(-5.18104412158608,-1.06186685398839,
21.8238371777705));
#37865=CARTESIAN_POINT('Ctrl Pts',(-4.04212630117128,-3.41061102326193,
21.903209067824));
#37866=CARTESIAN_POINT('Ctrl Pts',(-1.91852825506946,-4.92850206746972,
21.9825809578774));
#37867=CARTESIAN_POINT('Ctrl Pts',(0.672404619068471,-5.245839892308,22.0619528479308));
#37868=CARTESIAN_POINT('Ctrl Pts',(3.09954884704109,-4.28529268150223,22.1413247379842));
#37869=CARTESIAN_POINT('Ctrl Pts',(4.77164579536192,-2.28086298099128,22.2206966280376));
#37870=CARTESIAN_POINT('Ctrl Pts',(5.28138253005217,0.279182711729235,22.300068518091));
#37871=CARTESIAN_POINT('Ctrl Pts',(4.50458503707303,2.77121862106756,22.3794404081444));
#37872=CARTESIAN_POINT('Ctrl Pts',(2.63048120009391,4.58819259887664,22.4588122981978));
#37873=CARTESIAN_POINT('Ctrl Pts',(0.115597647321455,5.28749259670008,22.5381841882512));
#37874=CARTESIAN_POINT('Ctrl Pts',(-2.42744506809483,4.69877132337436,22.6175560783046));
#37875=CARTESIAN_POINT('Ctrl Pts',(-4.37916762715256,2.96543963879382,22.696927968358));
#37876=CARTESIAN_POINT('Ctrl Pts',(-5.26413459813381,0.509733484286287,
22.7762998584114));
#37877=CARTESIAN_POINT('Ctrl Pts',(-4.86677005798463,-2.07014265165558,
22.8556717484648));
#37878=CARTESIAN_POINT('Ctrl Pts',(-3.28387109087741,-4.14573660239302,
22.9350436385182));
#37879=CARTESIAN_POINT('Ctrl Pts',(-0.901028401772815,-5.21143830245831,
23.0144155285717));
#37880=CARTESIAN_POINT('Ctrl Pts',(1.70130281532621,-5.00764516247504,23.093787418625));
#37881=CARTESIAN_POINT('Ctrl Pts',(3.88920043041414,-3.58400074773866,23.1731593086785));
#37882=CARTESIAN_POINT('Ctrl Pts',(5.12969743029434,-1.28730168253193,23.2525311987318));
#37883=CARTESIAN_POINT('Ctrl Pts',(5.12061148999571,1.32298122241883,23.3319030887853));
#37884=CARTESIAN_POINT('Ctrl Pts',(3.86415592530766,3.6109888303426,23.4112749788386));
#37885=CARTESIAN_POINT('Ctrl Pts',(1.66640053022393,5.01936755177924,23.4906468688921));
#37886=CARTESIAN_POINT('Ctrl Pts',(-0.937286345425383,5.20503944789203,
23.5700187589454));
#37887=CARTESIAN_POINT('Ctrl Pts',(-3.31265234202061,4.12277525560054,23.6493906489989));
#37888=CARTESIAN_POINT('Ctrl Pts',(-4.88106356050821,2.03621213668325,23.7287625390522));
#37889=CARTESIAN_POINT('Ctrl Pts',(-5.26045849971908,-0.546367751667005,
23.8081344291057));
#37890=CARTESIAN_POINT('Ctrl Pts',(-4.35841739221935,-2.99585366506712,
23.887506319159));
#37891=CARTESIAN_POINT('Ctrl Pts',(-2.3946754551717,-4.71555625687105,23.9668782092125));
#37892=CARTESIAN_POINT('Ctrl Pts',(0.152404122233421,-5.28655978220554,
24.0462500992659));
#37893=CARTESIAN_POINT('Ctrl Pts',(2.66235839280233,-4.56976904619763,24.1256219893193));
#37894=CARTESIAN_POINT('Ctrl Pts',(4.52376805191542,-2.73979268554746,24.2049938793727));
#37895=CARTESIAN_POINT('Ctrl Pts',(5.28319782677237,-0.242408891126616,
24.2843657694261));
#37896=CARTESIAN_POINT('Ctrl Pts',(4.75565230518779,2.3140251726099,24.3637376594795));
#37897=CARTESIAN_POINT('Ctrl Pts',(3.0696404085172,4.30676782630642,24.4431095495329));
#37898=CARTESIAN_POINT('Ctrl Pts',(0.635870902865647,5.25039137038364,24.5224814395863));
#37899=CARTESIAN_POINT('Ctrl Pts',(-1.95279534724764,4.9150311981795,24.6018533296397));
#37900=CARTESIAN_POINT('Ctrl Pts',(-4.06576497321052,3.38238030533593,24.6812252196931));
#37901=CARTESIAN_POINT('Ctrl Pts',(-5.18832325111748,1.02578905688434,24.7605971097465));
#37902=CARTESIAN_POINT('Ctrl Pts',(-5.04701746921096,-1.58068213527875,
24.8399689997999));
#37903=CARTESIAN_POINT('Ctrl Pts',(-3.67626940318832,-3.80210265806849,
24.9193408898533));
#37904=CARTESIAN_POINT('Ctrl Pts',(-1.40999024783327,-5.09733938916421,
24.9987127799067));
#37905=CARTESIAN_POINT('Ctrl Pts',(1.19975941093347,-5.1508755278289,25.0780846699601));
#37906=CARTESIAN_POINT('Ctrl Pts',(3.51725033281924,-3.94966978918403,25.1574565600135));
#37907=CARTESIAN_POINT('Ctrl Pts',(4.97794685893178,-1.7863332323397,25.2368284500669));
#37908=CARTESIAN_POINT('Ctrl Pts',(5.226026548707,0.812150145920977,25.3162003401203));
#37909=CARTESIAN_POINT('Ctrl Pts',(4.20105773883081,3.21279554629917,25.3955722301737));
#37910=CARTESIAN_POINT('Ctrl Pts',(2.15272056265901,4.83081106300121,25.4749441202272));
#37911=CARTESIAN_POINT('Ctrl Pts',(-0.420014577610356,5.27205169757513,
25.5543160102805));
#37912=CARTESIAN_POINT('Ctrl Pts',(-2.89043509646038,4.42903220810823,25.6336879003339));
#37913=CARTESIAN_POINT('Ctrl Pts',(-4.65675202368223,2.50711027624266,25.7130597903873));
#37914=CARTESIAN_POINT('Ctrl Pts',(-5.28869446548081,-0.0255381695211706,
25.7924316804408));
#37915=CARTESIAN_POINT('Ctrl Pts',(-4.63232264181493,-2.55196557371741,
25.8718035704942));
#37916=CARTESIAN_POINT('Ctrl Pts',(-2.84752727607513,-4.45673981283608,
25.9511754605475));
#37917=CARTESIAN_POINT('Ctrl Pts',(-0.369080568778156,-5.27586209837409,
26.030547350601));
#37918=CARTESIAN_POINT('Ctrl Pts',(2.19927334812716,-4.80979605467087,26.1099192406543));
#37919=CARTESIAN_POINT('Ctrl Pts',(4.23188914543768,-3.17207433835284,26.1892911307078));
#37920=CARTESIAN_POINT('Ctrl Pts',(5.23362611404738,-0.761642334479479,
26.2686630207611));
#37921=CARTESIAN_POINT('Ctrl Pts',(4.96046334571002,1.83432405620638,26.3480349108146));
#37922=CARTESIAN_POINT('Ctrl Pts',(3.47894268615705,3.98345316700778,26.427406800868));
#37923=CARTESIAN_POINT('Ctrl Pts',(1.14995928876529,5.16222190355009,26.5067786909214));
#37924=CARTESIAN_POINT('Ctrl Pts',(-1.45915164597797,5.08348481077201,26.5861505809748));
#37925=CARTESIAN_POINT('Ctrl Pts',(-3.71281646953845,3.76642207019263,26.6655224710282));
#37926=CARTESIAN_POINT('Ctrl Pts',(-5.06204741929919,1.53186725014815,26.7448943610816));
#37927=CARTESIAN_POINT('Ctrl Pts',(-5.17817482237054,-1.07584704130177,
26.824266251135));
#37928=CARTESIAN_POINT('Ctrl Pts',(-4.032910300408,-3.42148737483758,26.9036381411884));
#37929=CARTESIAN_POINT('Ctrl Pts',(-1.90523775596165,-4.93366095719681,
26.9830100312419));
#37930=CARTESIAN_POINT('Ctrl Pts',(0.686546488664775,-5.24400565085624,
27.0623819212952));
#37931=CARTESIAN_POINT('Ctrl Pts',(3.11108952829732,-4.27692217537667,27.1417538113486));
#37932=CARTESIAN_POINT('Ctrl Pts',(4.77777804511651,-2.267989924782,27.221125701402));
#37933=CARTESIAN_POINT('Ctrl Pts',(5.28061040557762,0.293419651379019,27.3004975914554));
#37934=CARTESIAN_POINT('Ctrl Pts',(4.49709775967288,2.7833528499375,27.3798694815089));
#37935=CARTESIAN_POINT('Ctrl Pts',(2.61810205366886,4.59526745509821,27.4592413715622));
#37936=CARTESIAN_POINT('Ctrl Pts',(0.101342482461748,5.28778507964899,27.5386132616156));
#37937=CARTESIAN_POINT('Ctrl Pts',(-2.44010389315526,4.69220996311103,27.617985151669));
#37938=CARTESIAN_POINT('Ctrl Pts',(-4.38714636147802,2.95362288558985,27.6973570417224));
#37939=CARTESIAN_POINT('Ctrl Pts',(-5.26548968692851,0.495539810872365,
27.7767289317758));
#37940=CARTESIAN_POINT('Ctrl Pts',(-4.86117137960698,-2.08325566491491,
27.8561008218293));
#37941=CARTESIAN_POINT('Ctrl Pts',(-3.27268248423349,-4.15457467193712,
27.9354727118826));
#37942=CARTESIAN_POINT('Ctrl Pts',(-0.886975379660524,-5.21384848487045,
28.0148446019361));
#37943=CARTESIAN_POINT('Ctrl Pts',(1.71479696411104,-5.00304034754724,28.0942164919895));
#37944=CARTESIAN_POINT('Ctrl Pts',(3.89884856306386,-3.57350265560346,28.1735883820429));
#37945=CARTESIAN_POINT('Ctrl Pts',(5.1331492820092,-1.27346762656861,28.2529602720963));
#37946=CARTESIAN_POINT('Ctrl Pts',(5.11702619789033,1.3367812975255,28.3323321621497));
#37947=CARTESIAN_POINT('Ctrl Pts',(3.85440685831077,3.62139325645763,28.4117040522031));
#37948=CARTESIAN_POINT('Ctrl Pts',(1.6528625396316,5.02384183393471,28.4910759422564));
#37949=CARTESIAN_POINT('Ctrl Pts',(-0.951315435152638,5.20249366075061,
28.5704478323099));
#37950=CARTESIAN_POINT('Ctrl Pts',(-3.32375507563475,4.11382954733206,28.6498197223633));
#37951=CARTESIAN_POINT('Ctrl Pts',(-4.8865353366993,2.02304566199065,28.7291916124167));
#37952=CARTESIAN_POINT('Ctrl Pts',(-5.25896640590637,-0.560547668676075,
28.8085635024701));
#37953=CARTESIAN_POINT('Ctrl Pts',(-4.35032489915935,-3.00759282800452,
28.8879353925235));
#37954=CARTESIAN_POINT('Ctrl Pts',(-2.38195387625792,-4.72199503162487,
28.9673072825769));
#37955=CARTESIAN_POINT('Ctrl Pts',(0.166655838534471,-5.28612969750008,
29.0466791726303));
#37956=CARTESIAN_POINT('Ctrl Pts',(2.67466855994625,-4.56257486971391,29.1260510626837));
#37957=CARTESIAN_POINT('Ctrl Pts',(4.53113794043359,-2.72758690275364,29.2054229527372));
#37958=CARTESIAN_POINT('Ctrl Pts',(5.28383214813505,-0.228164803693758,
29.2847948427905));
#37959=CARTESIAN_POINT('Ctrl Pts',(4.74939654011487,2.32683773651173,29.3641667328439));
#37960=CARTESIAN_POINT('Ctrl Pts',(3.05801844753361,4.31502775447088,29.4435386228973));
#37961=CARTESIAN_POINT('Ctrl Pts',(0.621713829942241,5.25208656259286,29.5229105129507));
#37962=CARTESIAN_POINT('Ctrl Pts',(-1.96603890048284,4.90974870936366,29.6022824030042));
#37963=CARTESIAN_POINT('Ctrl Pts',(-4.07486890650364,3.37140693807791,29.6816542930575));
#37964=CARTESIAN_POINT('Ctrl Pts',(-5.19106986646947,1.01179789915904,29.7610261831109));
#37965=CARTESIAN_POINT('Ctrl Pts',(-5.04273769720158,-1.59428286841832,
29.8403980731643));
#37966=CARTESIAN_POINT('Ctrl Pts',(-3.66600578680595,-3.81199985813419,
29.9197699632177));
#37967=CARTESIAN_POINT('Ctrl Pts',(-1.39624298131062,-5.10112212012718,
29.9991418532712));
#37968=CARTESIAN_POINT('Ctrl Pts',(1.21364152390063,-5.1476223247995,30.0785137433246));
#37969=CARTESIAN_POINT('Ctrl Pts',(3.52788564023963,-3.94017312521939,30.157885633378));
#37970=CARTESIAN_POINT('Ctrl Pts',(4.98274462345863,-1.7729064737611,30.2372575234313));
#37971=CARTESIAN_POINT('Ctrl Pts',(5.22381804552127,0.826236270443475,30.3166294134848));
#37972=CARTESIAN_POINT('Ctrl Pts',(4.19238095442003,3.22410968801099,30.3960013035382));
#37973=CARTESIAN_POINT('Ctrl Pts',(2.13968914249988,4.83659712202475,30.4753731935916));
#37974=CARTESIAN_POINT('Ctrl Pts',(-0.434226208411599,5.27090020273941,
30.554745083645));
#37975=CARTESIAN_POINT('Ctrl Pts',(-2.90236501609743,4.4212236610065,30.6341169736984));
#37976=CARTESIAN_POINT('Ctrl Pts',(-4.66349413013793,2.49454682166501,30.7134888637518));
#37977=CARTESIAN_POINT('Ctrl Pts',(-5.28860639654603,-0.0397961018483339,
30.7928607538052));
#37978=CARTESIAN_POINT('Ctrl Pts',(-4.62542585088724,-2.56444478303865,
30.8722326438586));
#37979=CARTESIAN_POINT('Ctrl Pts',(-2.83550180615875,-4.46440039138299,
30.951604533912));
#37980=CARTESIAN_POINT('Ctrl Pts',(-0.354855797726762,-5.27683794616905,
31.0309764239654));
#37981=CARTESIAN_POINT('Ctrl Pts',(2.21223229757146,-4.80384945735102,31.1103483140188));
#37982=CARTESIAN_POINT('Ctrl Pts',(4.24042550187443,-3.16065387386267,31.1897202040722));
#37983=CARTESIAN_POINT('Ctrl Pts',(5.23566043994338,-0.747530002690045,
31.2690920941256));
#37984=CARTESIAN_POINT('Ctrl Pts',(4.95550008377996,1.84769052250822,31.348463984179));
#37985=CARTESIAN_POINT('Ctrl Pts',(3.46819087602115,3.99281772621712,31.4278358742324));
#37986=CARTESIAN_POINT('Ctrl Pts',(1.13603804757386,5.16530336977167,31.5072077642858));
#37987=CARTESIAN_POINT('Ctrl Pts',(-1.47285113468488,5.07953254565492,31.5865796543392));
#37988=CARTESIAN_POINT('Ctrl Pts',(-3.72295704063504,3.75639883677117,31.6659515443926));
#37989=CARTESIAN_POINT('Ctrl Pts',(-5.06615885211213,1.51821468589782,31.745323434446));
#37990=CARTESIAN_POINT('Ctrl Pts',(-5.17525558096714,-1.08980320194903,
31.8246953244994));
#37991=CARTESIAN_POINT('Ctrl Pts',(-4.02367150553249,-3.43234744203962,
31.9040672145529));
#37992=CARTESIAN_POINT('Ctrl Pts',(-1.89192995759591,-4.93877944262154,
31.9834391046062));
#37993=CARTESIAN_POINT('Ctrl Pts',(0.70068154029511,-5.24213570278371,32.0628109946597));
#37994=CARTESIAN_POINT('Ctrl Pts',(3.12260856590247,-4.26851930901834,32.142182884713));
#37995=CARTESIAN_POINT('Ctrl Pts',(4.78387505663285,-2.25510105978337,32.2215547747665));
#37996=CARTESIAN_POINT('Ctrl Pts',(5.27980017249531,0.307654816033343,32.3009266648198));
#37997=CARTESIAN_POINT('Ctrl Pts',(4.48957765297736,2.79546665964672,32.3802985548733));
#37998=CARTESIAN_POINT('Ctrl Pts',(2.60570395470567,4.60230901263064,32.4596704449267));
#37999=CARTESIAN_POINT('Ctrl Pts',(0.0870865406955613,5.28803907717593,
32.5390423349801));
#38000=CARTESIAN_POINT('Ctrl Pts',(-2.45274496186521,4.68561452739711,32.6184142250335));
#38001=CARTESIAN_POINT('Ctrl Pts',(-4.39509322077448,2.94178465017617,32.6977861150869));
#38002=CARTESIAN_POINT('Ctrl Pts',(-5.26680649947691,0.48134254370224,32.7771580051403));
#38003=CARTESIAN_POINT('Ctrl Pts',(-4.85553737278523,-2.09635354098391,
32.8565298951937));
#38004=CARTESIAN_POINT('Ctrl Pts',(-3.26147008963279,-4.16338254328624,
32.9359017852471));
#38005=CARTESIAN_POINT('Ctrl Pts',(-0.8729159117874,-5.21622077353502,33.0152736753005));
#38006=CARTESIAN_POINT('Ctrl Pts',(1.72827865000283,-4.99839916925953,33.0946455653539));
#38007=CARTESIAN_POINT('Ctrl Pts',(3.9084683581323,-3.5629785911213,33.1740174554073));
#38008=CARTESIAN_POINT('Ctrl Pts',(5.13656382546866,-1.25962431470524,33.2533893454607));
#38009=CARTESIAN_POINT('Ctrl Pts',(5.11340371451205,1.35057165664188,33.3327612355141));
#38010=CARTESIAN_POINT('Ctrl Pts',(3.84462977702742,3.63177136187071,33.4121331255675));
#38011=CARTESIAN_POINT('Ctrl Pts',(1.63931253580255,5.02827960213734,33.4915050156209));
#38012=CARTESIAN_POINT('Ctrl Pts',(-0.965337610587002,5.19991006123145,
33.5708769056743));
#38013=CARTESIAN_POINT('Ctrl Pts',(-3.33483365177614,4.1048539392153,33.6502487957277));
#38014=CARTESIAN_POINT('Ctrl Pts',(-4.89197159692173,2.00986448354636,33.7296206857811));
#38015=CARTESIAN_POINT('Ctrl Pts',(-5.25743608925264,-0.574723511554913,
33.8089925758345));
#38016=CARTESIAN_POINT('Ctrl Pts',(-4.34220078737896,-3.01931013137032,
33.888364465888));
#38017=CARTESIAN_POINT('Ctrl Pts',(-2.36921498499824,-4.72839948631349,
33.9677363559413));
#38018=CARTESIAN_POINT('Ctrl Pts',(0.18090634355963,-5.28566119252548,34.0471082459947));
#38019=CARTESIAN_POINT('Ctrl Pts',(2.68695928725581,-4.55534753185087,34.1264801360481));
#38020=CARTESIAN_POINT('Ctrl Pts',(4.53847489605999,-2.71536129550809,34.2058520261016));
#38021=CARTESIAN_POINT('Ctrl Pts',(5.28442806592769,-0.21391905792982,34.2852239161549));
#38022=CARTESIAN_POINT('Ctrl Pts',(4.74310625581857,2.3396333886583,34.3645958062084));
#38023=CARTESIAN_POINT('Ctrl Pts',(3.04637426047967,4.32325632045994,34.4439676962618));
#38024=CARTESIAN_POINT('Ctrl Pts',(0.607552238322964,5.25374358196314,34.5233395863151));
#38025=CARTESIAN_POINT('Ctrl Pts',(-1.97926816429518,4.90443053586424,34.6027114763686));
#38026=CARTESIAN_POINT('Ctrl Pts',(-4.08394322312674,3.36040906700167,34.6820833664219));
#38027=CARTESIAN_POINT('Ctrl Pts',(-5.19377875245966,0.997799387556786,
34.7614552564754));
#38028=CARTESIAN_POINT('Ctrl Pts',(-5.03842127392763,-1.60787201410546,
34.8408271465287));
#38029=CARTESIAN_POINT('Ctrl Pts',(-3.65571552542313,-3.82186935209593,
34.9201990365822));
#38030=CARTESIAN_POINT('Ctrl Pts',(-1.38248556671468,-5.10486777548014,
34.9995709266355));
#38031=CARTESIAN_POINT('Ctrl Pts',(1.22751481596557,-5.14433170819057,35.078942816689));
#38032=CARTESIAN_POINT('Ctrl Pts',(3.53849530653457,-3.93064782357091,35.1583147067423));
#38033=CARTESIAN_POINT('Ctrl Pts',(4.98750617275828,-1.75946682947078,35.2376865967958));
#38034=CARTESIAN_POINT('Ctrl Pts',(5.22157157495577,0.840316389774704,35.3170584868492));
#38035=CARTESIAN_POINT('Ctrl Pts',(4.18367369924664,3.23540039647985,35.3964303769026));
#38036=CARTESIAN_POINT('Ctrl Pts',(2.12664217080567,4.8423480280398,35.4758022669559));
#38037=CARTESIAN_POINT('Ctrl Pts',(-0.448434683200953,5.2697103983248,35.5551741570095));
#38038=CARTESIAN_POINT('Ctrl Pts',(-2.91427384097317,4.41338297988397,35.6345460470627));
#38039=CARTESIAN_POINT('Ctrl Pts',(-4.67020234172003,2.48196523640092,35.7139179371163));
#38040=CARTESIAN_POINT('Ctrl Pts',(-5.28847988934142,-0.0540537449324728,
35.7932898271696));
#38041=CARTESIAN_POINT('Ctrl Pts',(-4.61849544177097,-2.57690535364626,
35.872661717223));
#38042=CARTESIAN_POINT('Ctrl Pts',(-2.82345572745135,-4.47202852209511,
35.9520336072764));
#38043=CARTESIAN_POINT('Ctrl Pts',(-0.340628447537815,-5.27777544122882,
36.0314054973298));
#38044=CARTESIAN_POINT('Ctrl Pts',(2.22517516822766,-4.79786794503694,36.1107773873833));
#38045=CARTESIAN_POINT('Ctrl Pts',(4.2489310383545,-3.14921043733466,36.1901492774366));
#38046=CARTESIAN_POINT('Ctrl Pts',(5.23765671238758,-0.733412237756749,
36.2695211674901));
#38047=CARTESIAN_POINT('Ctrl Pts',(4.95050080463952,1.8610435595583,36.3488930575434));
#38048=CARTESIAN_POINT('Ctrl Pts',(3.45741385862894,4.002153265115,36.4282649475969));
#38049=CARTESIAN_POINT('Ctrl Pts',(1.12210854951209,5.16834729390565,36.5076368376502));
#38050=CARTESIAN_POINT('Ctrl Pts',(-1.4865399185207,5.07554336184357,36.5870087277037));
#38051=CARTESIAN_POINT('Ctrl Pts',(-3.73307055280216,3.74634830136112,36.666380617757));
#38052=CARTESIAN_POINT('Ctrl Pts',(-5.07023346343257,1.50455108706837,36.7457525078105));
#38053=CARTESIAN_POINT('Ctrl Pts',(-5.17229872514219,-1.10375144176689,
36.8251243978638));
#38054=CARTESIAN_POINT('Ctrl Pts',(-4.01440346609619,-3.44318256250012,
36.9044962879173));
#38055=CARTESIAN_POINT('Ctrl Pts',(-1.87860840844056,-4.94386203236358,
36.9838681779707));
#38056=CARTESIAN_POINT('Ctrl Pts',(0.71481149928202,-5.24022765419639,37.0632400680241));
#38057=CARTESIAN_POINT('Ctrl Pts',(3.13410490798792,-4.26008541851396,37.1426119580775));
#38058=CARTESIAN_POINT('Ctrl Pts',(4.78993729833158,-2.24219580442096,37.2219838481309));
#38059=CARTESIAN_POINT('Ctrl Pts',(5.27895156514787,0.321887744613352,37.3013557381843));
#38060=CARTESIAN_POINT('Ctrl Pts',(4.48202491545551,2.80756015154514,37.3807276282377));
#38061=CARTESIAN_POINT('Ctrl Pts',(2.59328691715162,4.6093171199916,37.4600995182911));
#38062=CARTESIAN_POINT('Ctrl Pts',(0.0728299659736646,5.28825464055466,
37.5394714083445));
#38063=CARTESIAN_POINT('Ctrl Pts',(-2.46536820371075,4.67898503603898,37.6188432983979));
#38064=CARTESIAN_POINT('Ctrl Pts',(-4.40300813596802,2.92992503348812,37.6982151884513));
#38065=CARTESIAN_POINT('Ctrl Pts',(-5.26808503220261,0.467141778084607,
37.7775870785047));
#38066=CARTESIAN_POINT('Ctrl Pts',(-4.84986807528987,-2.10943618050861,
37.8569589685581));
#38067=CARTESIAN_POINT('Ctrl Pts',(-3.2502339902585,-4.17216015459505,37.9363308586115));
#38068=CARTESIAN_POINT('Ctrl Pts',(-0.858850099431265,-5.21855515011692,
38.0157027486649));
#38069=CARTESIAN_POINT('Ctrl Pts',(1.74174777450972,-4.99372166181591,38.0950746387183));
#38070=CARTESIAN_POINT('Ctrl Pts',(3.91805974601555,-3.55242863073569,38.1744465287717));
#38071=CARTESIAN_POINT('Ctrl Pts',(5.13994103560184,-1.24577184719802,38.2538184188251));
#38072=CARTESIAN_POINT('Ctrl Pts',(5.10974406648872,1.36435219862427,38.3331903088785));
#38073=CARTESIAN_POINT('Ctrl Pts',(3.83482475204887,3.64212307300276,38.4125621989319));
#38074=CARTESIAN_POINT('Ctrl Pts',(1.62575061805696,5.03268082057242,38.4919340889853));
#38075=CARTESIAN_POINT('Ctrl Pts',(-0.979352771366501,5.19728867487039,
38.5713059790387));
#38076=CARTESIAN_POINT('Ctrl Pts',(-3.3458879870052,4.09584848370752,38.6506778690921));
#38077=CARTESIAN_POINT('Ctrl Pts',(-4.89737230716795,1.99666872129193,38.7300497591456));
#38078=CARTESIAN_POINT('Ctrl Pts',(-5.2558675504918,-0.588895222855594,
38.809421649199));
#38079=CARTESIAN_POINT('Ctrl Pts',(-4.33404513553914,-3.03100540392653,
38.8887935392523));
#38080=CARTESIAN_POINT('Ctrl Pts',(-2.35645883694701,-4.73476973691708,
38.9681654293058));
#38081=CARTESIAN_POINT('Ctrl Pts',(0.195155463808245,-5.28515396379923,
39.0475373193592));
#38082=CARTESIAN_POINT('Ctrl Pts',(2.69923061743519,-4.54808766460433,39.1269092094126));
#38083=CARTESIAN_POINT('Ctrl Pts',(4.5457786161602,-2.70311485851688,39.2062810994659));
#38084=CARTESIAN_POINT('Ctrl Pts',(5.28498604656423,-0.199673823356607,
39.2856529895194));
#38085=CARTESIAN_POINT('Ctrl Pts',(4.73678060915317,2.35241593705468,39.3650248795727));
#38086=CARTESIAN_POINT('Ctrl Pts',(3.03470961035893,4.33144609848054,39.4443967696262));
#38087=CARTESIAN_POINT('Ctrl Pts',(0.593383061700927,5.25537632570972,39.5237686596795));
#38088=CARTESIAN_POINT('Ctrl Pts',(-1.99247705733066,4.8990504464678,39.603140549733));
#38089=CARTESIAN_POINT('Ctrl Pts',(-4.09299916691649,3.34943642687039,39.6825124397864));
#38090=CARTESIAN_POINT('Ctrl Pts',(-5.19642846461573,0.983699440459269,
39.7618843298398));
#38091=CARTESIAN_POINT('Ctrl Pts',(-5.03410925482033,-1.62126816458454,
39.8412562198932));
#38092=CARTESIAN_POINT('Ctrl Pts',(-3.6453165085118,-3.83208153227987,39.9206281099466));
#38093=CARTESIAN_POINT('Ctrl Pts',(-2.12771778283764,-4.68247622999901,
39.9735427033155));
#38094=CARTESIAN_POINT('Ctrl Pts',(-1.31303618635638,-4.90075024188325,
40.));
#38095=CARTESIAN_POINT('Ctrl Pts',(-3.43378788736187,2.93584158412999,-1.38777878078145E-15));
#38096=CARTESIAN_POINT('Ctrl Pts',(-3.5274298169339,2.83894612463338,-1.38777878078145E-15));
#38097=CARTESIAN_POINT('Ctrl Pts',(-3.61644080326455,2.73799316940158,-1.70682494898246E-15));
#38098=CARTESIAN_POINT('Ctrl Pts',(-3.70070760607863,2.63340714286309,-1.68962066560141E-15));
#38099=CARTESIAN_POINT('Ctrl Pts',(-3.78643913867677,2.52700319677679,-1.67211733650556E-15));
#38100=CARTESIAN_POINT('Ctrl Pts',(-3.86726060843671,2.41683829132909,-1.52825423918462E-15));
#38101=CARTESIAN_POINT('Ctrl Pts',(-3.9430233259709,2.30331415642333,-1.42247325030098E-15));
#38102=CARTESIAN_POINT('Ctrl Pts',(-4.01958942326278,2.18858622372678,-1.31557057111923E-15));
#38103=CARTESIAN_POINT('Ctrl Pts',(-4.09098941448581,2.07042685422507,-1.45703061823736E-15));
#38104=CARTESIAN_POINT('Ctrl Pts',(-4.15703260143776,1.94921318851517,-1.40165656858926E-15));
#38105=CARTESIAN_POINT('Ctrl Pts',(-4.22276474819078,1.82857039656885,-1.34654331125317E-15));
#38106=CARTESIAN_POINT('Ctrl Pts',(-4.28319084758819,1.70490133278768,-1.76868280947178E-15));
#38107=CARTESIAN_POINT('Ctrl Pts',(-4.33807945470206,1.57855051046471,-1.88044024795886E-15));
#38108=CARTESIAN_POINT('Ctrl Pts',(-4.35502796120398,1.53953589802935,-1.91494871469599E-15));
#38109=CARTESIAN_POINT('Ctrl Pts',(-4.37144815676901,1.50026543549027,-1.30689270547165E-15));
#38110=CARTESIAN_POINT('Ctrl Pts',(-4.38733228779962,1.46074889051522,-1.32532873564628E-15));
#38111=CARTESIAN_POINT('Ctrl Pts',(-4.39376253093777,1.44475173009898,-1.33279204328941E-15));
#38112=CARTESIAN_POINT('Ctrl Pts',(-4.40010357988131,1.42871748389362,-1.28259685789569E-15));
#38113=CARTESIAN_POINT('Ctrl Pts',(-4.4063520165592,1.41265478977856,-1.29063426612674E-15));
#38114=CARTESIAN_POINT('Ctrl Pts',(-4.45729152748394,1.28170591015729,-1.35615811881152E-15));
#38115=CARTESIAN_POINT('Ctrl Pts',(-4.50214144181921,1.14871482526442,-2.13815754900839E-15));
#38116=CARTESIAN_POINT('Ctrl Pts',(-4.54074327371246,1.0140904790896,-2.05391259555654E-15));
#38117=CARTESIAN_POINT('Ctrl Pts',(-4.54547345988333,0.997593898764086,
-2.0435893985931E-15));
#38118=CARTESIAN_POINT('Ctrl Pts',(-4.55010977859188,0.981072752949281,
-1.00791691148873E-15));
#38119=CARTESIAN_POINT('Ctrl Pts',(-4.55465189605181,0.964527761093366,
-1.01307850997046E-15));
#38120=CARTESIAN_POINT('Ctrl Pts',(-4.59134817932549,0.830858891175244,
-1.05169067743968E-15));
#38121=CARTESIAN_POINT('Ctrl Pts',(-4.62189967399316,0.695635489793831,
-1.41485248297211E-15));
#38122=CARTESIAN_POINT('Ctrl Pts',(-4.64637428491341,0.559286455771474,
-1.36002320516582E-15));
#38123=CARTESIAN_POINT('Ctrl Pts',(-4.67110897469857,0.42148851201501,-1.30461128535625E-15));
#38124=CARTESIAN_POINT('Ctrl Pts',(-4.68963709540601,0.282540149701787,
-1.43104411647104E-15));
#38125=CARTESIAN_POINT('Ctrl Pts',(-4.70197867697062,0.142866308633218,
-1.36002320516582E-15));
#38126=CARTESIAN_POINT('Ctrl Pts',(-4.71314718957453,0.0164684846393732,
-1.29575284087739E-15));
#38127=CARTESIAN_POINT('Ctrl Pts',(-4.71924875509872,-0.110524098082,-1.66579323769632E-15));
#38128=CARTESIAN_POINT('Ctrl Pts',(-4.72026194547141,-0.237801095913712,
-1.67921232474555E-15));
#38129=CARTESIAN_POINT('Ctrl Pts',(-4.72045200129662,-0.261675913030809,
-1.68172949795545E-15));
#38130=CARTESIAN_POINT('Ctrl Pts',(-4.72046291446759,-0.285560737563283,
-9.9370225703457E-16));
#38131=CARTESIAN_POINT('Ctrl Pts',(-4.72029440609211,-0.309453515786201,
-9.71445146547012E-16));
#38132=CARTESIAN_POINT('Ctrl Pts',(-4.72016631155934,-0.327616021086772,
-9.54526022139039E-16));
#38133=CARTESIAN_POINT('Ctrl Pts',(-4.7199344986873,-0.345781850732525,
-1.1165476318937E-15));
#38134=CARTESIAN_POINT('Ctrl Pts',(-4.7195992402228,-0.363937763232007,
-1.12410081243297E-15));
#38135=CARTESIAN_POINT('Ctrl Pts',(-4.7169715342115,-0.506241106673104,
-1.18330151878048E-15));
#38136=CARTESIAN_POINT('Ctrl Pts',(-4.70799214533038,-0.648137600560786,
-1.67849620506959E-15));
#38137=CARTESIAN_POINT('Ctrl Pts',(-4.69273559502703,-0.789185289486343,
-1.60982338570648E-15));
#38138=CARTESIAN_POINT('Ctrl Pts',(-4.67736001919945,-0.931333376259461,
-1.5406148083796E-15));
#38139=CARTESIAN_POINT('Ctrl Pts',(-4.65560906635571,-1.07262015451611,
-1.29947818212301E-15));
#38140=CARTESIAN_POINT('Ctrl Pts',(-4.62750766548139,-1.21260443247969,
-1.38777878078145E-15));
#38141=CARTESIAN_POINT('Ctrl Pts',(-4.61688292082861,-1.26553052023664,
-1.42116399590398E-15));
#38142=CARTESIAN_POINT('Ctrl Pts',(-4.60534985624838,-1.31827046839259,
-1.10373700911438E-15));
#38143=CARTESIAN_POINT('Ctrl Pts',(-4.59290787692679,-1.37080047994465,
-1.0547118733939E-15));
#38144=CARTESIAN_POINT('Ctrl Pts',(-4.56011975477607,-1.50923186540429,
-9.25516823562078E-16));
#38145=CARTESIAN_POINT('Ctrl Pts',(-4.52102317103095,-1.64620611480812,
-1.41788356490645E-15));
#38146=CARTESIAN_POINT('Ctrl Pts',(-4.47583839059365,-1.78136570298785,
-1.36002320516582E-15));
#38147=CARTESIAN_POINT('Ctrl Pts',(-4.44941052359499,-1.86041841908909,
-1.32618159130998E-15));
#38148=CARTESIAN_POINT('Ctrl Pts',(-4.42089896739826,-1.93885019183042,
-1.30868430769761E-15));
#38149=CARTESIAN_POINT('Ctrl Pts',(-4.3903399301827,-2.01658705378289,-1.30451205393456E-15));
#38150=CARTESIAN_POINT('Ctrl Pts',(-4.37718466105246,-2.05005176450371,
-1.30271595280921E-15));
#38151=CARTESIAN_POINT('Ctrl Pts',(-4.36364988420426,-2.08338766611273,
-1.16152748166208E-15));
#38152=CARTESIAN_POINT('Ctrl Pts',(-4.3497381750326,-2.11658871139626,-1.13797860024079E-15));
#38153=CARTESIAN_POINT('Ctrl Pts',(-4.34244585283277,-2.13399223217085,
-1.12563460794976E-15));
#38154=CARTESIAN_POINT('Ctrl Pts',(-4.33504992528714,-2.15135862906508,
-1.92978013206096E-15));
#38155=CARTESIAN_POINT('Ctrl Pts',(-4.32755662758879,-2.16867384922929,
-1.9151347174784E-15));
#38156=CARTESIAN_POINT('Ctrl Pts',(-4.2701680431329,-2.30128515265925,-1.80297053483165E-15));
#38157=CARTESIAN_POINT('Ctrl Pts',(-4.20699158680529,-2.43109046195038,
-1.71043044263751E-15));
#38158=CARTESIAN_POINT('Ctrl Pts',(-4.13831811099888,-2.55774085897211,
-1.72084568816899E-15));
#38159=CARTESIAN_POINT('Ctrl Pts',(-4.0690864175418,-2.68542074352523,-1.73134559482798E-15));
#38160=CARTESIAN_POINT('Ctrl Pts',(-3.99426770892291,-2.80989493979695,
-1.80815084065395E-15));
#38161=CARTESIAN_POINT('Ctrl Pts',(-3.91410750939009,-2.93079631633735,
-1.80411241501588E-15));
#38162=CARTESIAN_POINT('Ctrl Pts',(-3.83416065570548,-3.05137591465264,
-1.8000847376213E-15));
#38163=CARTESIAN_POINT('Ctrl Pts',(-3.74890035710146,-3.16840239753955,
-1.26386791065628E-15));
#38164=CARTESIAN_POINT('Ctrl Pts',(-3.6585229556131,-3.28149127673775,-1.27675647831893E-15));
#38165=CARTESIAN_POINT('Ctrl Pts',(-3.59945026249498,-3.35540870018578,
-1.2851807347119E-15));
#38166=CARTESIAN_POINT('Ctrl Pts',(-3.5381904788592,-3.42764345712454,-1.45186396209174E-15));
#38167=CARTESIAN_POINT('Ctrl Pts',(-3.47478854700661,-3.49808125449704,
-1.41553435639707E-15));
#38168=CARTESIAN_POINT('Ctrl Pts',(-3.4391425896078,-3.5376829298883,-1.39540507371065E-15));
#38169=CARTESIAN_POINT('Ctrl Pts',(-3.40281937333393,-3.57671648450509,
-1.55816047969468E-15));
#38170=CARTESIAN_POINT('Ctrl Pts',(-3.36583573983685,-3.61517046963578,
-1.55431223447522E-15));
#38171=CARTESIAN_POINT('Ctrl Pts',(-3.34056943595204,-3.64144128139824,
-1.55168320849956E-15));
#38172=CARTESIAN_POINT('Ctrl Pts',(-3.31499488246685,-3.66744157776442,
-1.71311115652187E-15));
#38173=CARTESIAN_POINT('Ctrl Pts',(-3.28911728144163,-3.6931675174981,-1.69309011255336E-15));
#38174=CARTESIAN_POINT('Ctrl Pts',(-3.27259035745335,-3.70959758186502,
-1.68030352265613E-15));
#38175=CARTESIAN_POINT('Ctrl Pts',(-3.25594506354961,-3.7259104717157,-1.35072386705874E-15));
#38176=CARTESIAN_POINT('Ctrl Pts',(-3.23918904311522,-3.74209965697934,
-1.36002320516582E-15));
#38177=CARTESIAN_POINT('Ctrl Pts',(-3.13422859724164,-3.84350942251737,
-1.41827466635674E-15));
#38178=CARTESIAN_POINT('Ctrl Pts',(-3.02485537861799,-3.94013896638234,
-1.29586046630586E-15));
#38179=CARTESIAN_POINT('Ctrl Pts',(-2.91147703861897,-4.03180594754837,
-1.33226762955019E-15));
#38180=CARTESIAN_POINT('Ctrl Pts',(-2.80007805253152,-4.12187261071949,
-1.36803919819172E-15));
#38181=CARTESIAN_POINT('Ctrl Pts',(-2.68481190070853,-4.20714879945784,
-1.75330405072015E-15));
#38182=CARTESIAN_POINT('Ctrl Pts',(-2.5660285220091,-4.28743071443088,-1.77635683940025E-15));
#38183=CARTESIAN_POINT('Ctrl Pts',(-2.51557747120272,-4.32152897813987,
-1.78614808650622E-15));
#38184=CARTESIAN_POINT('Ctrl Pts',(-2.46449152304015,-4.35472587736193,
-1.31186991621621E-15));
#38185=CARTESIAN_POINT('Ctrl Pts',(-2.41279587231268,-4.38700384624999,
-1.27675647831893E-15));
#38186=CARTESIAN_POINT('Ctrl Pts',(-2.38543234505614,-4.40408921163422,
-1.2581702432788E-15));
#38187=CARTESIAN_POINT('Ctrl Pts',(-2.35789457340209,-4.42091901104391,
-1.50863034215941E-15));
#38188=CARTESIAN_POINT('Ctrl Pts',(-2.3302097471481,-4.43747675896359,-1.49880108324396E-15));
#38189=CARTESIAN_POINT('Ctrl Pts',(-2.2023530709709,-4.51394531233533,-1.45340667250483E-15));
#38190=CARTESIAN_POINT('Ctrl Pts',(-2.07127177001784,-4.58467311410489,
-7.9672741319199E-16));
#38191=CARTESIAN_POINT('Ctrl Pts',(-1.93736496285559,-4.64944928440847,
-4.9960036108132E-16));
#38192=CARTESIAN_POINT('Ctrl Pts',(-1.80364190208402,-4.71413656910759,
-2.02881025535331E-16));
#38193=CARTESIAN_POINT('Ctrl Pts',(-1.66710043882179,-4.77288900981815,
-3.16087603122754E-17));
#38194=CARTESIAN_POINT('Ctrl Pts',(-1.52810715957136,-4.82545526764581,
-5.55111512312578E-17));
#38195=CARTESIAN_POINT('Ctrl Pts',(-1.49120032503771,-4.83941316683462,
-6.1857944337824E-17));
#38196=CARTESIAN_POINT('Ctrl Pts',(-1.4541204835251,-4.85293465562285,3.75650465851052E-17));
#38197=CARTESIAN_POINT('Ctrl Pts',(-1.41687422066829,-4.86601447289862,
5.55111512312578E-17));
#38198=CARTESIAN_POINT('Ctrl Pts',(-1.38244754401982,-4.87810413251642,
1.27205291019773E-16));
#38199=CARTESIAN_POINT('Ctrl Pts',(-1.3478786871628,-4.88981645711078,2.24269765851654E-16));
#38200=CARTESIAN_POINT('Ctrl Pts',(-1.31317395760259,-4.90115117757553,
2.22044604925031E-16));
#38201=CARTESIAN_POINT('Ctrl Pts',(4.51755838390264,-0.00010457874560596,
1.61258330249198));
#38202=CARTESIAN_POINT('Ctrl Pts',(4.51776153214983,-0.238054206488734,
1.60420146868401));
#38203=CARTESIAN_POINT('Ctrl Pts',(4.49928771368086,-0.475972597056525,
1.59581963487604));
#38204=CARTESIAN_POINT('Ctrl Pts',(4.46186317968569,-0.710871726876144,
1.58743780106807));
#38205=CARTESIAN_POINT('Ctrl Pts',(4.34373246725773,-1.45233190264972,1.5609805043836));
#38206=CARTESIAN_POINT('Ctrl Pts',(4.03678590132105,-2.16370961033161,1.53452320769914));
#38207=CARTESIAN_POINT('Ctrl Pts',(3.57840923518442,-2.75835983566981,1.50806591101467));
#38208=CARTESIAN_POINT('Ctrl Pts',(3.1200325690478,-3.353010061008,1.4816086143302));
#38209=CARTESIAN_POINT('Ctrl Pts',(2.51022580271121,-3.8309328040025,1.45515131764573));
#38210=CARTESIAN_POINT('Ctrl Pts',(1.82326272299592,-4.13391759737134,1.42869402096126));
#38211=CARTESIAN_POINT('Ctrl Pts',(1.13629964328063,-4.43690239074017,1.4022367242768));
#38212=CARTESIAN_POINT('Ctrl Pts',(0.372180250186614,-4.56494923448333,
1.37577942759233));
#38213=CARTESIAN_POINT('Ctrl Pts',(-0.37602655530059,-4.50246217629702,
1.34932213090786));
#38214=CARTESIAN_POINT('Ctrl Pts',(-1.1242333607878,-4.4399751181107,1.32286483422339));
#38215=CARTESIAN_POINT('Ctrl Pts',(-1.85652757866819,-4.18695415799491,
1.29640753753892));
#38216=CARTESIAN_POINT('Ctrl Pts',(-2.48371659230757,-3.77421694705552,
1.26995024085446));
#38217=CARTESIAN_POINT('Ctrl Pts',(-3.11090560594693,-3.36147973611613,
1.24349294416999));
#38218=CARTESIAN_POINT('Ctrl Pts',(-3.63298941534527,-2.78902627435314,
1.21703564748552));
#38219=CARTESIAN_POINT('Ctrl Pts',(-3.98637877398998,-2.12658080103894,
1.19057835080105));
#38220=CARTESIAN_POINT('Ctrl Pts',(-4.3397681326347,-1.46413532772474,1.16412105411659));
#38221=CARTESIAN_POINT('Ctrl Pts',(-4.52446304052578,-0.711697842859317,
1.13766375743212));
#38222=CARTESIAN_POINT('Ctrl Pts',(-4.51796789313228,0.039085678406338,
1.11120646074765));
#38223=CARTESIAN_POINT('Ctrl Pts',(-4.51147274573878,0.789869199671988,
1.08474916406318));
#38224=CARTESIAN_POINT('Ctrl Pts',(-4.3137875430607,1.53899875733787,1.05829186737871));
#38225=CARTESIAN_POINT('Ctrl Pts',(-3.94899006576281,2.19523105353949,1.03183457069425));
#38226=CARTESIAN_POINT('Ctrl Pts',(-3.58419258846491,2.85146334974111,1.00537727400978));
#38227=CARTESIAN_POINT('Ctrl Pts',(-3.0522828365472,3.41479838447846,0.97891997732531));
#38228=CARTESIAN_POINT('Ctrl Pts',(-2.4180469390755,3.81662285121812,0.952462680640842));
#38229=CARTESIAN_POINT('Ctrl Pts',(-1.78381104160379,4.21844731795778,0.926005383956374));
#38230=CARTESIAN_POINT('Ctrl Pts',(-1.0472489985781,4.45876121669975,0.899548087271906));
#38231=CARTESIAN_POINT('Ctrl Pts',(-0.298073044029486,4.50829405706007,
0.873090790587439));
#38232=CARTESIAN_POINT('Ctrl Pts',(0.451102910519128,4.55782689742038,0.846633493902971));
#38233=CARTESIAN_POINT('Ctrl Pts',(1.21289277659066,4.41657867939905,0.820176197218503));
#38234=CARTESIAN_POINT('Ctrl Pts',(1.89451099954032,4.10175426806438,0.793718900534035));
#38235=CARTESIAN_POINT('Ctrl Pts',(2.57612922248998,3.7869298567297,0.767261603849567));
#38236=CARTESIAN_POINT('Ctrl Pts',(3.17757580231775,3.29852925208169,0.740804307165098));
#38237=CARTESIAN_POINT('Ctrl Pts',(3.6255959515189,2.69603724086577,0.71434701048063));
#38238=CARTESIAN_POINT('Ctrl Pts',(4.07361610072004,2.09354522964985,0.687889713796163));
#38239=CARTESIAN_POINT('Ctrl Pts',(4.36820981929455,1.37696181186601,0.661432417111696));
#38240=CARTESIAN_POINT('Ctrl Pts',(4.47349452055126,0.633569578843809,0.634975120427228));
#38241=CARTESIAN_POINT('Ctrl Pts',(4.50319667153093,0.423849191372714,0.627511181115478));
#38242=CARTESIAN_POINT('Ctrl Pts',(4.51783217716753,0.211995155346536,0.620047241803728));
#38243=CARTESIAN_POINT('Ctrl Pts',(4.51763087883895,0.00011359767064345,
0.612583302491977));
#38244=CARTESIAN_POINT('Ctrl Pts',(1.3130361863565,-4.90075024188322,0.));
#38245=CARTESIAN_POINT('Ctrl Pts',(2.12771778283771,-4.68247622999897,0.0264572966844678));
#38246=CARTESIAN_POINT('Ctrl Pts',(3.64531650851188,-3.8320815322798,0.0793718900534037));
#38247=CARTESIAN_POINT('Ctrl Pts',(5.03410925482037,-1.62126816458446,0.158743780106807));
#38248=CARTESIAN_POINT('Ctrl Pts',(5.19642846461569,0.98369944045933,0.238115670160212));
#38249=CARTESIAN_POINT('Ctrl Pts',(4.09299916691648,3.34943642687043,0.317487560213614));
#38250=CARTESIAN_POINT('Ctrl Pts',(1.99247705733062,4.89905044646781,0.396859450267019));
#38251=CARTESIAN_POINT('Ctrl Pts',(-0.593383061700938,5.2553763257097,0.476231340320422));
#38252=CARTESIAN_POINT('Ctrl Pts',(-3.03470961035893,4.33144609848054,0.555603230373826));
#38253=CARTESIAN_POINT('Ctrl Pts',(-4.73678060915323,2.35241593705463,0.634975120427228));
#38254=CARTESIAN_POINT('Ctrl Pts',(-5.28498604656423,-0.199673823356779,
0.714347010480634));
#38255=CARTESIAN_POINT('Ctrl Pts',(-4.5457786161601,-2.703114858517,0.793718900534037));
#38256=CARTESIAN_POINT('Ctrl Pts',(-2.69923061743508,-4.5480876646044,0.87309079058744));
#38257=CARTESIAN_POINT('Ctrl Pts',(-0.195155463808127,-5.28515396379925,
0.952462680640845));
#38258=CARTESIAN_POINT('Ctrl Pts',(2.35645883694709,-4.73476973691702,1.03183457069425));
#38259=CARTESIAN_POINT('Ctrl Pts',(4.33404513553918,-3.03100540392648,1.11120646074765));
#38260=CARTESIAN_POINT('Ctrl Pts',(5.25586755049182,-0.58889522285553,1.19057835080105));
#38261=CARTESIAN_POINT('Ctrl Pts',(4.89737230716791,1.99666872129196,1.26995024085446));
#38262=CARTESIAN_POINT('Ctrl Pts',(3.34588798700519,4.09584848370755,1.34932213090786));
#38263=CARTESIAN_POINT('Ctrl Pts',(0.979352771366438,5.19728867487042,1.42869402096127));
#38264=CARTESIAN_POINT('Ctrl Pts',(-1.6257506180571,5.03268082057239,1.50806591101467));
#38265=CARTESIAN_POINT('Ctrl Pts',(-3.83482475204895,3.64212307300266,1.58743780106807));
#38266=CARTESIAN_POINT('Ctrl Pts',(-5.10974406648874,1.36435219862418,1.66680969112148));
#38267=CARTESIAN_POINT('Ctrl Pts',(-5.13994103560183,-1.2457718471981,1.74618158117488));
#38268=CARTESIAN_POINT('Ctrl Pts',(-3.91805974601548,-3.55242863073578,
1.82555347122828));
#38269=CARTESIAN_POINT('Ctrl Pts',(-1.74174777450957,-4.99372166181597,
1.90492536128169));
#38270=CARTESIAN_POINT('Ctrl Pts',(0.858850099431454,-5.21855515011689,
1.98429725133509));
#38271=CARTESIAN_POINT('Ctrl Pts',(3.25023399025869,-4.17216015459491,2.0636691413885));
#38272=CARTESIAN_POINT('Ctrl Pts',(4.84986807528995,-2.10943618050841,2.1430410314419));
#38273=CARTESIAN_POINT('Ctrl Pts',(5.26808503220259,0.467141778084788,2.22241292149531));
#38274=CARTESIAN_POINT('Ctrl Pts',(4.40300813596794,2.92992503348825,2.3017848115487));
#38275=CARTESIAN_POINT('Ctrl Pts',(2.46536820371062,4.67898503603904,2.38115670160211));
#38276=CARTESIAN_POINT('Ctrl Pts',(-0.0728299659737919,5.28825464055465,
2.46052859165552));
#38277=CARTESIAN_POINT('Ctrl Pts',(-2.59328691715172,4.60931711999155,2.53990048170891));
#38278=CARTESIAN_POINT('Ctrl Pts',(-4.4820249154556,2.80756015154502,2.61927237176233));
#38279=CARTESIAN_POINT('Ctrl Pts',(-5.27895156514789,0.321887744613165,
2.69864426181572));
#38280=CARTESIAN_POINT('Ctrl Pts',(-4.7899372983315,-2.2421958044211,2.77801615186913));
#38281=CARTESIAN_POINT('Ctrl Pts',(-3.13410490798781,-4.26008541851404,
2.85738804192253));
#38282=CARTESIAN_POINT('Ctrl Pts',(-0.714811499281904,-5.2402276541964,
2.93675993197593));
#38283=CARTESIAN_POINT('Ctrl Pts',(1.8786084084407,-4.94386203236353,3.01613182202934));
#38284=CARTESIAN_POINT('Ctrl Pts',(4.01440346609632,-3.44318256249998,3.09550371208274));
#38285=CARTESIAN_POINT('Ctrl Pts',(5.17229872514222,-1.10375144176671,3.17487560213615));
#38286=CARTESIAN_POINT('Ctrl Pts',(5.07023346343252,1.50455108706853,3.25424749218955));
#38287=CARTESIAN_POINT('Ctrl Pts',(3.73307055280206,3.74634830136122,3.33361938224296));
#38288=CARTESIAN_POINT('Ctrl Pts',(1.48653991852054,5.07554336184363,3.41299127229636));
#38289=CARTESIAN_POINT('Ctrl Pts',(-1.12210854951228,5.16834729390561,3.49236316234976));
#38290=CARTESIAN_POINT('Ctrl Pts',(-3.45741385862906,4.00215326511488,3.57173505240317));
#38291=CARTESIAN_POINT('Ctrl Pts',(-4.95050080463958,1.86104355955814,3.65110694245657));
#38292=CARTESIAN_POINT('Ctrl Pts',(-5.23765671238755,-0.733412237756895,
3.73047883250997));
#38293=CARTESIAN_POINT('Ctrl Pts',(-4.24893103835441,-3.14921043733482,
3.80985072256337));
#38294=CARTESIAN_POINT('Ctrl Pts',(-2.22517516822744,-4.79786794503704,
3.88922261261678));
#38295=CARTESIAN_POINT('Ctrl Pts',(0.340628447538026,-5.2777754412288,3.96859450267018));
#38296=CARTESIAN_POINT('Ctrl Pts',(2.82345572745151,-4.472028522095,4.04796639272359));
#38297=CARTESIAN_POINT('Ctrl Pts',(4.61849544177105,-2.57690535364612,4.12733828277699));
#38298=CARTESIAN_POINT('Ctrl Pts',(5.28847988934143,-0.0540537449322821,
4.2067101728304));
#38299=CARTESIAN_POINT('Ctrl Pts',(4.67020234171992,2.48196523640112,4.2860820628838));
#38300=CARTESIAN_POINT('Ctrl Pts',(2.91427384097298,4.41338297988409,4.36545395293721));
#38301=CARTESIAN_POINT('Ctrl Pts',(0.44843468320075,5.26971039832481,4.44482584299061));
#38302=CARTESIAN_POINT('Ctrl Pts',(-2.12664217080585,4.84234802803972,4.52419773304401));
#38303=CARTESIAN_POINT('Ctrl Pts',(-4.18367369924674,3.23540039647972,4.60356962309741));
#38304=CARTESIAN_POINT('Ctrl Pts',(-5.22157157495578,0.840316389774564,
4.68294151315082));
#38305=CARTESIAN_POINT('Ctrl Pts',(-4.98750617275825,-1.75946682947089,
4.76231340320422));
#38306=CARTESIAN_POINT('Ctrl Pts',(-3.53849530653447,-3.93064782357102,
4.84168529325762));
#38307=CARTESIAN_POINT('Ctrl Pts',(-1.22751481596538,-5.14433170819062,
4.92105718331103));
#38308=CARTESIAN_POINT('Ctrl Pts',(1.3824855667149,-5.10486777548008,5.00042907336443));
#38309=CARTESIAN_POINT('Ctrl Pts',(3.65571552542333,-3.82186935209575,5.07980096341784));
#38310=CARTESIAN_POINT('Ctrl Pts',(5.03842127392769,-1.60787201410522,5.15917285347124));
#38311=CARTESIAN_POINT('Ctrl Pts',(5.1937787524596,0.997799387556994,5.23854474352464));
#38312=CARTESIAN_POINT('Ctrl Pts',(4.08394322312664,3.36040906700182,5.31791663357805));
#38313=CARTESIAN_POINT('Ctrl Pts',(1.979268164295,4.90443053586431,5.39728852363145));
#38314=CARTESIAN_POINT('Ctrl Pts',(-0.607552238323124,5.25374358196311,
5.47666041368485));
#38315=CARTESIAN_POINT('Ctrl Pts',(-3.04637426047979,4.32325632045987,5.55603230373826));
#38316=CARTESIAN_POINT('Ctrl Pts',(-4.74310625581864,2.33963338865815,5.63540419379165));
#38317=CARTESIAN_POINT('Ctrl Pts',(-5.28442806592769,-0.213919057930008,
5.71477608384507));
#38318=CARTESIAN_POINT('Ctrl Pts',(-4.53847489605989,-2.71536129550824,
5.79414797389846));
#38319=CARTESIAN_POINT('Ctrl Pts',(-2.68695928725567,-4.55534753185094,
5.87351986395187));
#38320=CARTESIAN_POINT('Ctrl Pts',(-0.180906343559476,-5.28566119252549,
5.95289175400528));
#38321=CARTESIAN_POINT('Ctrl Pts',(2.36921498499841,-4.72839948631341,6.03226364405867));
#38322=CARTESIAN_POINT('Ctrl Pts',(4.3422007873791,-3.01931013137013,6.1116355341121));
#38323=CARTESIAN_POINT('Ctrl Pts',(5.25743608925265,-0.574723511554695,
6.19100742416548));
#38324=CARTESIAN_POINT('Ctrl Pts',(4.89197159692165,2.00986448354653,6.2703793142189));
#38325=CARTESIAN_POINT('Ctrl Pts',(3.33483365177601,4.10485393921541,6.34975120427228));
#38326=CARTESIAN_POINT('Ctrl Pts',(0.96533761058682,5.19991006123149,6.42912309432572));
#38327=CARTESIAN_POINT('Ctrl Pts',(-1.63931253580277,5.02827960213728,6.50849498437909));
#38328=CARTESIAN_POINT('Ctrl Pts',(-3.84462977702757,3.63177136187054,6.58786687443252));
#38329=CARTESIAN_POINT('Ctrl Pts',(-5.11340371451209,1.35057165664169,6.6672387644859));
#38330=CARTESIAN_POINT('Ctrl Pts',(-5.13656382546863,-1.25962431470543,
6.74661065453933));
#38331=CARTESIAN_POINT('Ctrl Pts',(-3.90846835813217,-3.56297859112141,
6.82598254459271));
#38332=CARTESIAN_POINT('Ctrl Pts',(-1.72827865000271,-4.99839916925957,
6.90535443464612));
#38333=CARTESIAN_POINT('Ctrl Pts',(0.872915911787522,-5.21622077353501,
6.98472632469953));
#38334=CARTESIAN_POINT('Ctrl Pts',(3.26147008963291,-4.16338254328616,7.06409821475292));
#38335=CARTESIAN_POINT('Ctrl Pts',(4.85553737278532,-2.09635354098373,7.14347010480633));
#38336=CARTESIAN_POINT('Ctrl Pts',(5.26680649947689,0.481342543702463,7.22284199485974));
#38337=CARTESIAN_POINT('Ctrl Pts',(4.39509322077433,2.9417846501764,7.30221388491313));
#38338=CARTESIAN_POINT('Ctrl Pts',(2.45274496186498,4.68561452739722,7.38158577496654));
#38339=CARTESIAN_POINT('Ctrl Pts',(-0.0870865406957981,5.28803907717593,
7.46095766501995));
#38340=CARTESIAN_POINT('Ctrl Pts',(-2.60570395470586,4.60230901263053,7.54032955507335));
#38341=CARTESIAN_POINT('Ctrl Pts',(-4.48957765297745,2.79546665964655,7.61970144512676));
#38342=CARTESIAN_POINT('Ctrl Pts',(-5.27980017249532,0.307654816033177,
7.69907333518014));
#38343=CARTESIAN_POINT('Ctrl Pts',(-4.78387505663278,-2.25510105978351,
7.77844522523357));
#38344=CARTESIAN_POINT('Ctrl Pts',(-3.12260856590233,-4.26851930901846,
7.85781711528695));
#38345=CARTESIAN_POINT('Ctrl Pts',(-0.70068154029489,-5.24213570278374,
7.93718900534038));
#38346=CARTESIAN_POINT('Ctrl Pts',(1.8919299575961,-4.93877944262147,8.01656089539376));
#38347=CARTESIAN_POINT('Ctrl Pts',(4.02367150553262,-3.43234744203947,8.09593278544719));
#38348=CARTESIAN_POINT('Ctrl Pts',(5.1752555809672,-1.08980320194883,8.17530467550057));
#38349=CARTESIAN_POINT('Ctrl Pts',(5.06615885211206,1.51821468589804,8.25467656555398));
#38350=CARTESIAN_POINT('Ctrl Pts',(3.72295704063487,3.75639883677136,8.33404845560738));
#38351=CARTESIAN_POINT('Ctrl Pts',(1.47285113468463,5.07953254565499,8.41342034566079));
#38352=CARTESIAN_POINT('Ctrl Pts',(-1.1360380475741,5.16530336977162,8.49279223571419));
#38353=CARTESIAN_POINT('Ctrl Pts',(-3.46819087602133,3.99281772621695,8.57216412576759));
#38354=CARTESIAN_POINT('Ctrl Pts',(-4.95550008378004,1.84769052250801,8.651536015821));
#38355=CARTESIAN_POINT('Ctrl Pts',(-5.23566043994335,-0.74753000269027,
8.7309079058744));
#38356=CARTESIAN_POINT('Ctrl Pts',(-4.24042550187429,-3.16065387386283,
8.81027979592781));
#38357=CARTESIAN_POINT('Ctrl Pts',(-2.21223229757129,-4.8038494573511,8.88965168598121));
#38358=CARTESIAN_POINT('Ctrl Pts',(0.354855797726969,-5.27683794616905,
8.96902357603462));
#38359=CARTESIAN_POINT('Ctrl Pts',(2.83550180615889,-4.46440039138287,9.04839546608801));
#38360=CARTESIAN_POINT('Ctrl Pts',(4.6254258508873,-2.56444478303851,9.12776735614143));
#38361=CARTESIAN_POINT('Ctrl Pts',(5.28860639654605,-0.0397961018481786,
9.20713924619482));
#38362=CARTESIAN_POINT('Ctrl Pts',(4.66349413013784,2.49454682166519,9.28651113624823));
#38363=CARTESIAN_POINT('Ctrl Pts',(2.90236501609723,4.42122366100663,9.36588302630163));
#38364=CARTESIAN_POINT('Ctrl Pts',(0.434226208411351,5.27090020273944,9.44525491635504));
#38365=CARTESIAN_POINT('Ctrl Pts',(-2.13968914250016,4.83659712202464,9.52462680640844));
#38366=CARTESIAN_POINT('Ctrl Pts',(-4.1923809544202,3.22410968801074,9.60399869646184));
#38367=CARTESIAN_POINT('Ctrl Pts',(-5.22381804552131,0.826236270443201,
9.68337058651526));
#38368=CARTESIAN_POINT('Ctrl Pts',(-4.98274462345855,-1.77290647376134,
9.76274247656865));
#38369=CARTESIAN_POINT('Ctrl Pts',(-3.52788564023945,-3.94017312521954,
9.84211436662205));
#38370=CARTESIAN_POINT('Ctrl Pts',(-1.21364152390043,-5.14762232479954,
9.92148625667546));
#38371=CARTESIAN_POINT('Ctrl Pts',(1.39624298131078,-5.10112212012714,10.0008581467289));
#38372=CARTESIAN_POINT('Ctrl Pts',(3.66600578680612,-3.81199985813406,10.0802300367823));
#38373=CARTESIAN_POINT('Ctrl Pts',(5.04273769720163,-1.5942828684181,10.1596019268357));
#38374=CARTESIAN_POINT('Ctrl Pts',(5.19106986646944,1.01179789915923,10.2389738168891));
#38375=CARTESIAN_POINT('Ctrl Pts',(4.07486890650351,3.37140693807807,10.3183457069425));
#38376=CARTESIAN_POINT('Ctrl Pts',(1.96603890048266,4.90974870936374,10.3977175969959));
#38377=CARTESIAN_POINT('Ctrl Pts',(-0.621713829942471,5.25208656259283,
10.4770894870493));
#38378=CARTESIAN_POINT('Ctrl Pts',(-3.05801844753381,4.31502775447074,10.5564613771027));
#38379=CARTESIAN_POINT('Ctrl Pts',(-4.74939654011498,2.32683773651149,10.6358332671561));
#38380=CARTESIAN_POINT('Ctrl Pts',(-5.28383214813503,-0.228164803694007,
10.7152051572095));
#38381=CARTESIAN_POINT('Ctrl Pts',(-4.53113794043347,-2.72758690275384,
10.7945770472629));
#38382=CARTESIAN_POINT('Ctrl Pts',(-2.67466855994604,-4.56257486971405,
10.8739489373163));
#38383=CARTESIAN_POINT('Ctrl Pts',(-0.166655838534166,-5.2861296975001,
10.9533208273697));
#38384=CARTESIAN_POINT('Ctrl Pts',(2.38195387625819,-4.72199503162473,11.0326927174231));
#38385=CARTESIAN_POINT('Ctrl Pts',(4.3503248991595,-3.00759282800428,11.1120646074765));
#38386=CARTESIAN_POINT('Ctrl Pts',(5.2589664059064,-0.560547668675828,11.1914364975299));
#38387=CARTESIAN_POINT('Ctrl Pts',(4.8865353366992,2.02304566199086,11.2708083875833));
#38388=CARTESIAN_POINT('Ctrl Pts',(3.32375507563458,4.11382954733217,11.3501802776367));
#38389=CARTESIAN_POINT('Ctrl Pts',(0.951315435152466,5.20249366075065,11.4295521676901));
#38390=CARTESIAN_POINT('Ctrl Pts',(-1.6528625396318,5.02384183393465,11.5089240577436));
#38391=CARTESIAN_POINT('Ctrl Pts',(-3.85440685831092,3.62139325645746,11.5882959477969));
#38392=CARTESIAN_POINT('Ctrl Pts',(-5.11702619789041,1.33678129752526,11.6676678378503));
#38393=CARTESIAN_POINT('Ctrl Pts',(-5.13314928200913,-1.27346762656892,
11.7470397279037));
#38394=CARTESIAN_POINT('Ctrl Pts',(-3.89884856306365,-3.57350265560368,
11.8264116179572));
#38395=CARTESIAN_POINT('Ctrl Pts',(-1.71479696411077,-5.00304034754732,
11.9057835080105));
#38396=CARTESIAN_POINT('Ctrl Pts',(0.886975379660772,-5.21384848487043,
11.985155398064));
#38397=CARTESIAN_POINT('Ctrl Pts',(3.27268248423369,-4.15457467193696,12.0645272881174));
#38398=CARTESIAN_POINT('Ctrl Pts',(4.86117137960707,-2.08325566491467,12.1438991781708));
#38399=CARTESIAN_POINT('Ctrl Pts',(5.26548968692849,0.495539810872594,12.2232710682242));
#38400=CARTESIAN_POINT('Ctrl Pts',(4.38714636147788,2.95362288559007,12.3026429582776));
#38401=CARTESIAN_POINT('Ctrl Pts',(2.44010389315499,4.69220996311119,12.382014848331));
#38402=CARTESIAN_POINT('Ctrl Pts',(-0.101342482462103,5.28778507964898,
12.4613867383844));
#38403=CARTESIAN_POINT('Ctrl Pts',(-2.61810205366918,4.59526745509803,12.5407586284378));
#38404=CARTESIAN_POINT('Ctrl Pts',(-4.49709775967304,2.78335284993721,12.6201305184912));
#38405=CARTESIAN_POINT('Ctrl Pts',(-5.28061040557763,0.293419651378745,
12.6995024085446));
#38406=CARTESIAN_POINT('Ctrl Pts',(-4.7777780451164,-2.26798992478223,12.778874298598));
#38407=CARTESIAN_POINT('Ctrl Pts',(-3.11108952829712,-4.27692217537683,
12.8582461886514));
#38408=CARTESIAN_POINT('Ctrl Pts',(-0.686546488664521,-5.24400565085626,
12.9376180787048));
#38409=CARTESIAN_POINT('Ctrl Pts',(1.90523775596186,-4.93366095719673,13.0169899687582));
#38410=CARTESIAN_POINT('Ctrl Pts',(4.03291030040817,-3.42148737483739,13.0963618588116));
#38411=CARTESIAN_POINT('Ctrl Pts',(5.17817482237061,-1.07584704130148,13.175733748865));
#38412=CARTESIAN_POINT('Ctrl Pts',(5.06204741929909,1.53186725014844,13.2551056389184));
#38413=CARTESIAN_POINT('Ctrl Pts',(3.71281646953824,3.76642207019282,13.3344775289718));
#38414=CARTESIAN_POINT('Ctrl Pts',(1.45915164597774,5.08348481077208,13.4138494190252));
#38415=CARTESIAN_POINT('Ctrl Pts',(-1.14995928876559,5.16222190355004,13.4932213090786));
#38416=CARTESIAN_POINT('Ctrl Pts',(-3.47894268615732,3.98345316700755,13.572593199132));
#38417=CARTESIAN_POINT('Ctrl Pts',(-4.96046334571011,1.83432405620607,13.6519650891854));
#38418=CARTESIAN_POINT('Ctrl Pts',(-5.23362611404733,-0.761642334479749,
13.7313369792388));
#38419=CARTESIAN_POINT('Ctrl Pts',(-4.23188914543755,-3.17207433835303,
13.8107088692922));
#38420=CARTESIAN_POINT('Ctrl Pts',(-2.19927334812693,-4.80979605467098,
13.8900807593456));
#38421=CARTESIAN_POINT('Ctrl Pts',(0.369080568778457,-5.27586209837409,
13.9694526493991));
#38422=CARTESIAN_POINT('Ctrl Pts',(2.84752727607539,-4.45673981283591,14.0488245394524));
#38423=CARTESIAN_POINT('Ctrl Pts',(4.63232264181505,-2.55196557371717,14.1281964295059));
#38424=CARTESIAN_POINT('Ctrl Pts',(5.28869446548083,-0.0255381695209159,
14.2075683195592));
#38425=CARTESIAN_POINT('Ctrl Pts',(4.65675202368211,2.50711027624288,14.2869402096127));
#38426=CARTESIAN_POINT('Ctrl Pts',(2.89043509646017,4.42903220810837,14.3663120996661));
#38427=CARTESIAN_POINT('Ctrl Pts',(0.420014577610126,5.27205169757513,14.4456839897195));
#38428=CARTESIAN_POINT('Ctrl Pts',(-2.15272056265924,4.83081106300113,14.5250558797729));
#38429=CARTESIAN_POINT('Ctrl Pts',(-4.201057738831,3.21279554629894,14.6044277698263));
#38430=CARTESIAN_POINT('Ctrl Pts',(-5.22602654870706,0.81215014592063,14.6837996598797));
#38431=CARTESIAN_POINT('Ctrl Pts',(-4.97794685893165,-1.78633323234006,
14.7631715499331));
#38432=CARTESIAN_POINT('Ctrl Pts',(-3.51725033281897,-3.94966978918425,
14.8425434399865));
#38433=CARTESIAN_POINT('Ctrl Pts',(-1.19975941093315,-5.15087552782897,
14.9219153300399));
#38434=CARTESIAN_POINT('Ctrl Pts',(1.40999024783357,-5.09733938916413,15.0012872200933));
#38435=CARTESIAN_POINT('Ctrl Pts',(3.67626940318851,-3.8021026580683,15.0806591101467));
#38436=CARTESIAN_POINT('Ctrl Pts',(5.04701746921103,-1.5806821352785,15.1600310002001));
#38437=CARTESIAN_POINT('Ctrl Pts',(5.18832325111744,1.02578905688456,15.2394028902535));
#38438=CARTESIAN_POINT('Ctrl Pts',(4.06576497321036,3.38238030533612,15.3187747803069));
#38439=CARTESIAN_POINT('Ctrl Pts',(1.95279534724736,4.91503119817963,15.3981466703603));
#38440=CARTESIAN_POINT('Ctrl Pts',(-0.635870902865948,5.2503913703836,15.4775185604137));
#38441=CARTESIAN_POINT('Ctrl Pts',(-3.06964040851742,4.30676782630626,15.5568904504671));
#38442=CARTESIAN_POINT('Ctrl Pts',(-4.75565230518791,2.31402517260967,15.6362623405205));
#38443=CARTESIAN_POINT('Ctrl Pts',(-5.28319782677237,-0.24240889112691,
15.7156342305739));
#38444=CARTESIAN_POINT('Ctrl Pts',(-4.52376805191524,-2.73979268554778,
15.7950061206273));
#38445=CARTESIAN_POINT('Ctrl Pts',(-2.66235839280204,-4.56976904619777,
15.8743780106807));
#38446=CARTESIAN_POINT('Ctrl Pts',(-0.15240412223312,-5.28655978220556,
15.9537499007341));
#38447=CARTESIAN_POINT('Ctrl Pts',(2.39467545517194,-4.71555625687092,16.0331217907875));
#38448=CARTESIAN_POINT('Ctrl Pts',(4.35841739221953,-2.99585366506689,16.112493680841));
#38449=CARTESIAN_POINT('Ctrl Pts',(5.26045849971912,-0.546367751666672,
16.1918655708943));
#38450=CARTESIAN_POINT('Ctrl Pts',(4.88106356050808,2.03621213668353,16.2712374609478));
#38451=CARTESIAN_POINT('Ctrl Pts',(3.31265234202039,4.12277525560071,16.3506093510011));
#38452=CARTESIAN_POINT('Ctrl Pts',(0.937286345425132,5.20503944789207,16.4299812410546));
#38453=CARTESIAN_POINT('Ctrl Pts',(-1.66640053022416,5.01936755177917,16.509353131108));
#38454=CARTESIAN_POINT('Ctrl Pts',(-3.86415592530783,3.6109888303424,16.5887250211614));
#38455=CARTESIAN_POINT('Ctrl Pts',(-5.12061148999576,1.32298122241861,16.6680969112148));
#38456=CARTESIAN_POINT('Ctrl Pts',(-5.1296974302943,-1.28730168253218,16.7474688012682));
#38457=CARTESIAN_POINT('Ctrl Pts',(-3.88920043041393,-3.58400074773889,
16.8268406913216));
#38458=CARTESIAN_POINT('Ctrl Pts',(-1.70130281532588,-5.00764516247516,
16.906212581375));
#38459=CARTESIAN_POINT('Ctrl Pts',(0.90102840177319,-5.21143830245825,16.9855844714284));
#38460=CARTESIAN_POINT('Ctrl Pts',(3.28387109087768,-4.1457366023928,17.0649563614818));
#38461=CARTESIAN_POINT('Ctrl Pts',(4.86677005798476,-2.07014265165526,17.1443282515352));
#38462=CARTESIAN_POINT('Ctrl Pts',(5.26413459813378,0.50973348428664,17.2237001415886));
#38463=CARTESIAN_POINT('Ctrl Pts',(4.37916762715237,2.96543963879408,17.303072031642));
#38464=CARTESIAN_POINT('Ctrl Pts',(2.42744506809458,4.69877132337447,17.3824439216954));
#38465=CARTESIAN_POINT('Ctrl Pts',(-0.115597647321682,5.28749259670007,
17.4618158117488));
#38466=CARTESIAN_POINT('Ctrl Pts',(-2.63048120009413,4.58819259887652,17.5411877018022));
#38467=CARTESIAN_POINT('Ctrl Pts',(-4.5045850370732,2.7712186210673,17.6205595918556));
#38468=CARTESIAN_POINT('Ctrl Pts',(-5.28138253005218,0.27918271172893,17.699931481909));
#38469=CARTESIAN_POINT('Ctrl Pts',(-4.77164579536179,-2.28086298099153,
17.7793033719624));
#38470=CARTESIAN_POINT('Ctrl Pts',(-3.09954884704088,-4.28529268150238,
17.8586752620158));
#38471=CARTESIAN_POINT('Ctrl Pts',(-0.672404619068171,-5.24583989230806,
17.9380471520692));
#38472=CARTESIAN_POINT('Ctrl Pts',(1.91852825506979,-4.9285020674696,18.0174190421226));
#38473=CARTESIAN_POINT('Ctrl Pts',(4.04212630117149,-3.41061102326166,18.096790932176));
#38474=CARTESIAN_POINT('Ctrl Pts',(5.18104412158612,-1.06186685398811,18.1761628222294));
#38475=CARTESIAN_POINT('Ctrl Pts',(5.05792243214194,1.54547807796858,18.2555347122829));
#38476=CARTESIAN_POINT('Ctrl Pts',(3.70260503654169,3.77647571272922,18.3349066023362));
#38477=CARTESIAN_POINT('Ctrl Pts',(1.44552439996779,5.08729102078633,18.4142784923897));
#38478=CARTESIAN_POINT('Ctrl Pts',(-1.16402860508455,5.15930893371508,18.4936503824431));
#38479=CARTESIAN_POINT('Ctrl Pts',(-3.48937383888192,3.97367066688439,18.5730222724965));
#38480=CARTESIAN_POINT('Ctrl Pts',(-4.96594823061187,1.82167865277138,18.6523941625499));
#38481=CARTESIAN_POINT('Ctrl Pts',(-5.23050112077116,-0.77713504302674,
18.7317660526033));
#38482=CARTESIAN_POINT('Ctrl Pts',(-4.22530652207786,-3.18086119603167,
18.8111379426567));
#38483=CARTESIAN_POINT('Ctrl Pts',(-2.18257651229225,-4.82058518621618,
18.8905098327101));
#38484=CARTESIAN_POINT('Ctrl Pts',(0.37648005341871,-5.26605971579227,18.9698817227635));
#38485=CARTESIAN_POINT('Ctrl Pts',(3.70230252414111,-4.19446206534953,19.0757109095013));
#38486=CARTESIAN_POINT('Ctrl Pts',(5.99600976813328,-0.0197068834824163,
19.2079973929237));
#38487=CARTESIAN_POINT('Ctrl Pts',(3.26379011618947,5.03400372054209,19.3667411730305));
#38488=CARTESIAN_POINT('Ctrl Pts',(-2.45559119020206,5.46873373673905,19.5254849531373));
#38489=CARTESIAN_POINT('Ctrl Pts',(-5.92771323046149,0.905806267444168,
19.6842287332441));
#38490=CARTESIAN_POINT('Ctrl Pts',(-3.97578039972873,-4.48936692070992,
19.8429725133509));
#38491=CARTESIAN_POINT('Ctrl Pts',(1.61419617037569,-5.77483540889728,20.0017162934577));
#38492=CARTESIAN_POINT('Ctrl Pts',(5.72720375155094,-1.77677009197941,20.1604600735645));
#38493=CARTESIAN_POINT('Ctrl Pts',(4.59927593805412,3.84720861430021,20.3192038536713));
#38494=CARTESIAN_POINT('Ctrl Pts',(-0.73672307947618,5.95134306184733,20.4779476337782));
#38495=CARTESIAN_POINT('Ctrl Pts',(-5.3995463563661,2.60828838171381,20.6366914138849));
#38496=CARTESIAN_POINT('Ctrl Pts',(-5.1196790448508,-3.11863163173554,20.7954351939918));
#38497=CARTESIAN_POINT('Ctrl Pts',(-0.158509478954971,-5.99736559883163,
20.9541789740985));
#38498=CARTESIAN_POINT('Ctrl Pts',(4.95432466322423,-3.37745298000941,21.1129227542054));
#38499=CARTESIAN_POINT('Ctrl Pts',(5.4262515554071,1.3624793779577,21.2452092376277));
#38500=CARTESIAN_POINT('Ctrl Pts',(3.29092685490723,4.12830747359771,21.3510384243656));
#38501=CARTESIAN_POINT('Ctrl Pts',(0.929079443196039,5.20946188754723,21.430410314419));
#38502=CARTESIAN_POINT('Ctrl Pts',(-1.68303999757346,5.01382783115869,21.5097822044724));
#38503=CARTESIAN_POINT('Ctrl Pts',(-3.8722246926078,3.60110493868854,21.5891540945258));
#38504=CARTESIAN_POINT('Ctrl Pts',(-5.12503498129818,1.30888173016128,21.6685259845792));
#38505=CARTESIAN_POINT('Ctrl Pts',(-5.12574462250326,-1.300972874894,21.7478978746326));
#38506=CARTESIAN_POINT('Ctrl Pts',(-3.87976959979778,-3.59455409188016,
21.827269764686));
#38507=CARTESIAN_POINT('Ctrl Pts',(-1.68766624540451,-5.01217052435348,
21.9066416547394));
#38508=CARTESIAN_POINT('Ctrl Pts',(0.915005995631755,-5.2090130440819,21.9860135447928));
#38509=CARTESIAN_POINT('Ctrl Pts',(3.29507231119182,-4.13685632854986,22.0653854348462));
#38510=CARTESIAN_POINT('Ctrl Pts',(4.87231403886192,-2.05702097999265,22.1447573248996));
#38511=CARTESIAN_POINT('Ctrl Pts',(5.26275149225388,0.523926824466718,22.2241292149531));
#38512=CARTESIAN_POINT('Ctrl Pts',(4.37115162329097,2.97723307464397,22.3035011050064));
#38513=CARTESIAN_POINT('Ctrl Pts',(2.4147715124657,4.70529942618521,22.3828729950599));
#38514=CARTESIAN_POINT('Ctrl Pts',(-0.129853572474074,5.28716128664959,
22.4622448851132));
#38515=CARTESIAN_POINT('Ctrl Pts',(-2.64284027062663,4.58108446095525,22.5416167751666));
#38516=CARTESIAN_POINT('Ctrl Pts',(-4.51204028846786,2.7590644882843,22.62098866522));
#38517=CARTESIAN_POINT('Ctrl Pts',(-5.28211549991429,0.264943102456049,
22.7003605552734));
#38518=CARTESIAN_POINT('Ctrl Pts',(-4.76548000969985,-2.2937181486802,22.7797324453269));
#38519=CARTESIAN_POINT('Ctrl Pts',(-3.08798363825926,-4.29363457062517,
22.8591043353802));
#38520=CARTESIAN_POINT('Ctrl Pts',(-0.658261551986295,-5.24763120247219,
22.9384762254337));
#38521=CARTESIAN_POINT('Ctrl Pts',(1.93181173129385,-4.92331644248731,23.017848115487));
#38522=CARTESIAN_POINT('Ctrl Pts',(4.05129987868926,-3.39969271923279,23.0972200055405));
#38523=CARTESIAN_POINT('Ctrl Pts',(5.18390038229797,-1.0479113616667,23.1765918955939));
#38524=CARTESIAN_POINT('Ctrl Pts',(5.05371420635457,1.55913887720483,23.2559637856473));
#38525=CARTESIAN_POINT('Ctrl Pts',(3.69245444696201,3.78638634033052,23.3353356757007));
#38526=CARTESIAN_POINT('Ctrl Pts',(1.43172095156667,5.09127847004479,23.4147075657541));
#38527=CARTESIAN_POINT('Ctrl Pts',(-1.17777659548102,5.1559464348325,23.4940794558075));
#38528=CARTESIAN_POINT('Ctrl Pts',(-3.50037037246962,3.96463726004727,23.5734513458609));
#38529=CARTESIAN_POINT('Ctrl Pts',(-4.97028167379665,1.80755122457705,23.6528232359143));
#38530=CARTESIAN_POINT('Ctrl Pts',(-5.22944336137752,-0.789850288405212,
23.7321951259677));
#38531=CARTESIAN_POINT('Ctrl Pts',(-4.21472422106041,-3.19484601935549,
23.8115670160211));
#38532=CARTESIAN_POINT('Ctrl Pts',(-2.17330758975551,-4.82158433170509,
23.8909389060745));
#38533=CARTESIAN_POINT('Ctrl Pts',(0.397521959947206,-5.27379537322471,
23.9703107961279));
#38534=CARTESIAN_POINT('Ctrl Pts',(2.87151604007067,-4.4413215351868,24.0496826861813));
#38535=CARTESIAN_POINT('Ctrl Pts',(4.64601516884499,-2.5269516018695,24.1290545762347));
#38536=CARTESIAN_POINT('Ctrl Pts',(5.28875528625864,0.00297814834736192,
24.2084264662881));
#38537=CARTESIAN_POINT('Ctrl Pts',(4.64316632240633,2.53218242822061,24.2877983563415));
#38538=CARTESIAN_POINT('Ctrl Pts',(2.86651231988729,4.4445526734691,24.3671702463949));
#38539=CARTESIAN_POINT('Ctrl Pts',(0.391582261162602,5.27423972531146,24.4465421364484));
#38540=CARTESIAN_POINT('Ctrl Pts',(-2.1787363696294,4.81913365439931,24.5259140265017));
#38541=CARTESIAN_POINT('Ctrl Pts',(-4.21831964333045,3.19009729224708,24.6052859165552));
#38542=CARTESIAN_POINT('Ctrl Pts',(-5.23032958900859,0.783960290863936,
24.6846578066085));
#38543=CARTESIAN_POINT('Ctrl Pts',(-4.9682428239423,-1.81314770210696,24.764029696662));
#38544=CARTESIAN_POINT('Ctrl Pts',(-3.49590310398264,-3.96857692817898,
24.8434015867153));
#38545=CARTESIAN_POINT('Ctrl Pts',(-1.17196912594307,-5.15726959884261,
24.9227734767688));
#38546=CARTESIAN_POINT('Ctrl Pts',(1.43745393706658,-5.08966281065081,25.0021453668222));
#38547=CARTESIAN_POINT('Ctrl Pts',(3.69671640275713,-3.78222542756197,25.0815172568756));
#38548=CARTESIAN_POINT('Ctrl Pts',(5.05546693527898,-1.55344630213307,25.160889146929));
#38549=CARTESIAN_POINT('Ctrl Pts',(5.18271691245315,1.05374890400037,25.2402610369824));
#38550=CARTESIAN_POINT('Ctrl Pts',(4.04746852150308,3.40425320955296,25.3196329270358));
#38551=CARTESIAN_POINT('Ctrl Pts',(1.92626575763449,4.92548896844514,25.3990048170892));
#38552=CARTESIAN_POINT('Ctrl Pts',(-0.664171081076968,5.24688651700902,
25.4783767071426));
#38553=CARTESIAN_POINT('Ctrl Pts',(-3.09281731455583,4.2901541238158,25.5577485971959));
#38554=CARTESIAN_POINT('Ctrl Pts',(-4.76806009604388,2.2883496821561,25.6371204872494));
#38555=CARTESIAN_POINT('Ctrl Pts',(-5.28181399205765,-0.2708916769007,25.7164923773028));
#38556=CARTESIAN_POINT('Ctrl Pts',(-4.50892969070311,-2.76414442307307,
25.7958642673562));
#38557=CARTESIAN_POINT('Ctrl Pts',(-2.63768009703987,-4.58405770611471,
25.8752361574096));
#38558=CARTESIAN_POINT('Ctrl Pts',(-0.123897470143628,-5.28730467858643,
25.9546080474629));
#38559=CARTESIAN_POINT('Ctrl Pts',(2.42006630623721,-4.70257593460492,26.0339799375165));
#38560=CARTESIAN_POINT('Ctrl Pts',(4.37450728714461,-2.97231010192892,26.1133518275698));
#38561=CARTESIAN_POINT('Ctrl Pts',(5.26332797571122,-0.517996107519831,
26.1927237176232));
#38562=CARTESIAN_POINT('Ctrl Pts',(4.8700136195734,2.06250059211614,26.2720956076766));
#38563=CARTESIAN_POINT('Ctrl Pts',(3.29037472529985,4.14057671278022,26.35146749773));
#38564=CARTESIAN_POINT('Ctrl Pts',(0.909207831064193,5.21001751122215,26.4308393877834));
#38565=CARTESIAN_POINT('Ctrl Pts',(-1.69344007832135,5.01030957610855,26.5102112778369));
#38566=CARTESIAN_POINT('Ctrl Pts',(-3.88356973299385,3.59010131838702,26.5895831678902));
#38567=CARTESIAN_POINT('Ctrl Pts',(-5.12767039684481,1.29535232606086,26.6689550579437));
#38568=CARTESIAN_POINT('Ctrl Pts',(-5.12268190193029,-1.31494162567991,
26.748326947997));
#38569=CARTESIAN_POINT('Ctrl Pts',(-3.86981943456965,-3.604918707979,26.8276988380504));
#38570=CARTESIAN_POINT('Ctrl Pts',(-1.67427751864785,-5.01674557236666,
26.9070707281038));
#38571=CARTESIAN_POINT('Ctrl Pts',(0.929114694866165,-5.20650431970375,
26.9864426181573));
#38572=CARTESIAN_POINT('Ctrl Pts',(3.30617662527125,-4.12797013916282,27.0658145082107));
#38573=CARTESIAN_POINT('Ctrl Pts',(4.8778612478581,-2.04387156982875,27.145186398264));
#38574=CARTESIAN_POINT('Ctrl Pts',(5.26130966742943,0.538109589882639,27.2245582883175));
#38575=CARTESIAN_POINT('Ctrl Pts',(4.36311469772634,2.98900844458398,27.3039301783709));
#38576=CARTESIAN_POINT('Ctrl Pts',(2.40207464524773,4.7117914582426,27.3833020684242));
#38577=CARTESIAN_POINT('Ctrl Pts',(-0.144105473911181,5.28679250204684,
27.4626739584777));
#38578=CARTESIAN_POINT('Ctrl Pts',(-2.65518181859737,4.57394259446923,27.542045848531));
#38579=CARTESIAN_POINT('Ctrl Pts',(-4.51946174941854,2.74689039512913,27.6214177385845));
#38580=CARTESIAN_POINT('Ctrl Pts',(-5.28281080174027,0.25070177567431,27.7007896286378));
#38581=CARTESIAN_POINT('Ctrl Pts',(-4.75927883606144,-2.30655724141581,
27.7801615186913));
#38582=CARTESIAN_POINT('Ctrl Pts',(-3.07639708040302,-4.30194401997489,
27.8595334087447));
#38583=CARTESIAN_POINT('Ctrl Pts',(-0.644111805447875,-5.24938675745965,
27.9389052987981));
#38584=CARTESIAN_POINT('Ctrl Pts',(1.94507767959709,-4.91809050014772,28.0182771888515));
#38585=CARTESIAN_POINT('Ctrl Pts',(4.06045054724861,-3.38875828300845,28.0976490789049));
#38586=CARTESIAN_POINT('Ctrl Pts',(5.18670664924518,-1.03393204901761,28.1770209689583));
#38587=CARTESIAN_POINT('Ctrl Pts',(5.0494924920661,1.57275774354414,28.2563928590118));
#38588=CARTESIAN_POINT('Ctrl Pts',(3.68223314068176,3.79632723101881,28.3357647490651));
#38589=CARTESIAN_POINT('Ctrl Pts',(1.41798994671214,5.09511980804509,28.4151366391186));
#38590=CARTESIAN_POINT('Ctrl Pts',(-1.19167245960906,5.15275247768794,28.4945085291719));
#38591=CARTESIAN_POINT('Ctrl Pts',(-3.51104609249168,3.9551860491902,28.5738804192253));
#38592=CARTESIAN_POINT('Ctrl Pts',(-4.97513666881207,1.79414505376557,28.6532523092787));
#38593=CARTESIAN_POINT('Ctrl Pts',(-5.22729496488809,-0.803945705483672,
28.7326241993322));
#38594=CARTESIAN_POINT('Ctrl Pts',(-4.2060957779385,-3.20619707038074,28.8119960893855));
#38595=CARTESIAN_POINT('Ctrl Pts',(-2.16030096951815,-4.82742592572986,
28.891367979439));
#38596=CARTESIAN_POINT('Ctrl Pts',(0.41173837333167,-5.27270451089724,28.9707398694923));
#38597=CARTESIAN_POINT('Ctrl Pts',(2.88347915980534,-4.43356394814356,29.0501117595458));
#38598=CARTESIAN_POINT('Ctrl Pts',(4.65281080542333,-2.51441702114943,29.1294836495991));
#38599=CARTESIAN_POINT('Ctrl Pts',(5.28872803766221,0.0172363266290461,
29.2088555396526));
#38600=CARTESIAN_POINT('Ctrl Pts',(4.6363228263275,2.54469094339263,29.2882274297059));
#38601=CARTESIAN_POINT('Ctrl Pts',(2.85451963682592,4.45226447892365,29.3675993197594));
#38602=CARTESIAN_POINT('Ctrl Pts',(0.377361782165573,5.2752762423091,29.4469712098127));
#38603=CARTESIAN_POINT('Ctrl Pts',(-2.19172056735417,4.81324238969394,29.5263430998662));
#38604=CARTESIAN_POINT('Ctrl Pts',(-4.22690463795758,3.17871334488069,29.6057149899195));
#38605=CARTESIAN_POINT('Ctrl Pts',(-5.23242409484928,0.769856765217166,
29.6850868799731));
#38606=CARTESIAN_POINT('Ctrl Pts',(-4.96333662400999,-1.82653521840426,
29.7644587700263));
#38607=CARTESIAN_POINT('Ctrl Pts',(-3.48519133772112,-3.97798726578954,
29.8438306600798));
#38608=CARTESIAN_POINT('Ctrl Pts',(-1.15806115590354,-5.16041042035391,
29.9232025501331));
#38609=CARTESIAN_POINT('Ctrl Pts',(1.45117016016719,-5.08576901889481,30.0025744401866));
#38610=CARTESIAN_POINT('Ctrl Pts',(3.70689963733188,-3.77224554159173,30.08194633024));
#38611=CARTESIAN_POINT('Ctrl Pts',(5.05963656792573,-1.53981140008078,30.1613182202934));
#38612=CARTESIAN_POINT('Ctrl Pts',(5.17985722988845,1.06771739017516,30.2406901103468));
#38613=CARTESIAN_POINT('Ctrl Pts',(4.0382761360698,3.41515258753676,30.3200620004003));
#38614=CARTESIAN_POINT('Ctrl Pts',(1.91297991407722,4.93066417388641,30.3994338904535));
#38615=CARTESIAN_POINT('Ctrl Pts',(-0.678313980675348,5.24507688131741,
30.4788057805071));
#38616=CARTESIAN_POINT('Ctrl Pts',(-3.10437209115798,4.28180047024023,30.5581776705604));
#38617=CARTESIAN_POINT('Ctrl Pts',(-4.77421203164559,2.2754869422171,30.6375495606138));
#38618=CARTESIAN_POINT('Ctrl Pts',(-5.28106448876339,-0.285130168225216,
30.7169214506672));
#38619=CARTESIAN_POINT('Ctrl Pts',(-4.50146132585641,-2.77629020081278,
30.7962933407206));
#38620=CARTESIAN_POINT('Ctrl Pts',(-2.62531214778642,-4.59115208569648,
30.8756652307741));
#38621=CARTESIAN_POINT('Ctrl Pts',(-0.109642741545517,-5.28761948484725,
30.9550371208274));
#38622=CARTESIAN_POINT('Ctrl Pts',(2.43273539384572,-4.69603448143646,31.0344090108809));
#38623=CARTESIAN_POINT('Ctrl Pts',(4.38250457206463,-2.96050587284378,31.1137809009342));
#38624=CARTESIAN_POINT('Ctrl Pts',(5.26470533703794,-0.503804586594991,
31.1931527909877));
#38625=CARTESIAN_POINT('Ctrl Pts',(4.86443553513645,2.07562238179582,31.272524681041));
#38626=CARTESIAN_POINT('Ctrl Pts',(3.27920000412114,4.14943233229341,31.3518965710945));
#38627=CARTESIAN_POINT('Ctrl Pts',(0.895158610487983,5.21244975125701,31.4312684611478));
#38628=CARTESIAN_POINT('Ctrl Pts',(-1.70694143926006,5.00572594837619,31.5106403512013));
#38629=CARTESIAN_POINT('Ctrl Pts',(-3.89323433265515,3.57961838445739,31.5900122412546));
#38630=CARTESIAN_POINT('Ctrl Pts',(-5.13114396014345,1.28152370543563,31.6693841313081));
#38631=CARTESIAN_POINT('Ctrl Pts',(-5.11911827653528,-1.32874731162563,
31.7487560213615));
#38632=CARTESIAN_POINT('Ctrl Pts',(-3.86008671173927,-3.61533842470713,
31.8281279114149));
#38633=CARTESIAN_POINT('Ctrl Pts',(-1.6607465681206,-5.02124109994587,31.9074998014683));
#38634=CARTESIAN_POINT('Ctrl Pts',(0.943147763492109,-5.20398055756647,
31.9868716915216));
#38635=CARTESIAN_POINT('Ctrl Pts',(3.31729338754031,-4.11904187017945,32.0662435815751));
#38636=CARTESIAN_POINT('Ctrl Pts',(4.88335368508803,-2.03071370056122,32.1456154716285));
#38637=CARTESIAN_POINT('Ctrl Pts',(5.25983983406835,0.552291831605133,32.2249873616819));
#38638=CARTESIAN_POINT('Ctrl Pts',(4.35504064192764,3.00076029606972,32.3043592517354));
#38639=CARTESIAN_POINT('Ctrl Pts',(2.3893631891323,4.71825019448202,32.3837311417886));
#38640=CARTESIAN_POINT('Ctrl Pts',(-0.158357847769981,5.28638478918814,
32.4631030318421));
#38641=CARTESIAN_POINT('Ctrl Pts',(-2.66750326347463,4.56676775046226,32.5424749218955));
#38642=CARTESIAN_POINT('Ctrl Pts',(-4.52685078861515,2.73469619609277,32.6218468119489));
#38643=CARTESIAN_POINT('Ctrl Pts',(-5.28346748166331,0.23645870150246,32.7012187020024));
#38644=CARTESIAN_POINT('Ctrl Pts',(-4.75304319093522,-2.31937960938145,
32.7805905920557));
#38645=CARTESIAN_POINT('Ctrl Pts',(-3.06478809957792,-4.3102221812797,32.8599624821091));
#38646=CARTESIAN_POINT('Ctrl Pts',(-0.629957410956834,-5.25110417033318,
32.9393343721625));
#38647=CARTESIAN_POINT('Ctrl Pts',(1.95832950858626,-4.91282880661543,33.0187062622159));
#38648=CARTESIAN_POINT('Ctrl Pts',(4.06957169452659,-3.37779921996823,33.0980781522693));
#38649=CARTESIAN_POINT('Ctrl Pts',(5.18947522352436,-1.01994521996853,33.1774500423228));
#38650=CARTESIAN_POINT('Ctrl Pts',(5.04523407478018,1.586365178005,33.2568219323761));
#38651=CARTESIAN_POINT('Ctrl Pts',(3.67198507285579,3.80624052997629,33.3361938224296));
#38652=CARTESIAN_POINT('Ctrl Pts',(1.40424863498483,5.09892411381589,33.4155657124829));
#38653=CARTESIAN_POINT('Ctrl Pts',(-1.20555966211678,5.14952106980705,33.4949376025364));
#38654=CARTESIAN_POINT('Ctrl Pts',(-3.52169629398785,3.94570609146478,33.5743094925897));
#38655=CARTESIAN_POINT('Ctrl Pts',(-4.979955503786,1.78072584291395,33.6536813826432));
#38656=CARTESIAN_POINT('Ctrl Pts',(-5.22510857580638,-0.818035279400921,
33.7330532726965));
#38657=CARTESIAN_POINT('Ctrl Pts',(-4.19743676434199,-3.2175248183441,33.81242516275));
#38658=CARTESIAN_POINT('Ctrl Pts',(-2.14727864795256,-4.83323243340904,
33.8917970528034));
#38659=CARTESIAN_POINT('Ctrl Pts',(0.425951794157462,-5.27157532587404,
33.9711689428568));
#38660=CARTESIAN_POINT('Ctrl Pts',(2.89542132203897,-4.4257741373902,34.0505408329101));
#38661=CARTESIAN_POINT('Ctrl Pts',(4.6595726247782,-2.50186416532303,34.1299127229636));
#38662=CARTESIAN_POINT('Ctrl Pts',(5.28866234991056,0.0314943796344648,
34.209284613017));
#38663=CARTESIAN_POINT('Ctrl Pts',(4.62944563286023,2.55718096342464,34.2886565030704));
#38664=CARTESIAN_POINT('Ctrl Pts',(2.84250620674923,4.45994392474861,34.3680283931238));
#38665=CARTESIAN_POINT('Ctrl Pts',(0.363138560454883,5.27627441792225,34.4474002831772));
#38666=CARTESIAN_POINT('Ctrl Pts',(-2.20468883537271,4.80731614172534,34.5267721732306));
#38667=CARTESIAN_POINT('Ctrl Pts',(-4.23545891089946,3.1673062942179,34.606144063284));
#38668=CARTESIAN_POINT('Ctrl Pts',(-5.23448057076036,0.755747644152594,
34.6855159533374));
#38669=CARTESIAN_POINT('Ctrl Pts',(-4.95839434991029,-1.83990945920924,
34.7648878433908));
#38670=CARTESIAN_POINT('Ctrl Pts',(-3.47445424064183,-3.98736869087822,
34.8442597334442));
#38671=CARTESIAN_POINT('Ctrl Pts',(-1.14414476892706,-5.16351373534018,
34.9236316234976));
#38672=CARTESIAN_POINT('Ctrl Pts',(1.4648758359769,-5.0818382631171,35.003003513551));
#38673=CARTESIAN_POINT('Ctrl Pts',(3.71705592968454,-3.76223823845686,35.0823754036044));
#38674=CARTESIAN_POINT('Ctrl Pts',(5.06376942648477,-1.52616530648161,35.1617472936578));
#38675=CARTESIAN_POINT('Ctrl Pts',(5.1769598994568,1.08167811604296,35.2411191837112));
#38676=CARTESIAN_POINT('Ctrl Pts',(4.02905439992751,3.42602714375337,35.3204910737646));
#38677=CARTESIAN_POINT('Ctrl Pts',(1.8996801667365,4.93580354262787,35.3998629638181));
#38678=CARTESIAN_POINT('Ctrl Pts',(-0.69245195020073,5.24322912373406,35.4792348538714));
#38679=CARTESIAN_POINT('Ctrl Pts',(-3.11590430478548,4.27341569598948,35.5586067439249));
#38680=CARTESIAN_POINT('Ctrl Pts',(-4.78032926766171,2.26260766374704,35.6379786339782));
#38681=CARTESIAN_POINT('Ctrl Pts',(-5.28027660201491,-0.299366587187078,
35.7173505240316));
#38682=CARTESIAN_POINT('Ctrl Pts',(-4.49396024381123,-2.78841580011912,
35.7967224140851));
#38683=CARTESIAN_POINT('Ctrl Pts',(-2.61292511742748,-4.59821309619579,
35.8760943041384));
#38684=CARTESIAN_POINT('Ctrl Pts',(-0.0953872160500441,-5.28789586001125,
35.9554661941919));
#38685=CARTESIAN_POINT('Ctrl Pts',(2.4453868000212,-4.68945889688694,36.0348380842453));
#38686=CARTESIAN_POINT('Ctrl Pts',(4.39047000437915,-2.94868012642215,36.1142099742987));
#38687=CARTESIAN_POINT('Ctrl Pts',(5.26604443381084,-0.489609403953667,
36.1935818643521));
#38688=CARTESIAN_POINT('Ctrl Pts',(4.85882209535785,2.08872908558584,36.2729537544055));
#38689=CARTESIAN_POINT('Ctrl Pts',(3.26800144929601,4.15825779320007,36.3523256444589));
#38690=CARTESIAN_POINT('Ctrl Pts',(0.881102883784141,5.2148441065383,36.4316975345123));
#38691=CARTESIAN_POINT('Ctrl Pts',(-1.72043039392939,5.00110593838543,36.5110694245656));
#38692=CARTESIAN_POINT('Ctrl Pts',(-3.90287063578981,3.56910943340206,36.5904413146191));
#38693=CARTESIAN_POINT('Ctrl Pts',(-5.13458022962944,1.26768577053169,36.6698132046725));
#38694=CARTESIAN_POINT('Ctrl Pts',(-5.11551744473188,-1.34254334006536,
36.7491850947259));
#38695=CARTESIAN_POINT('Ctrl Pts',(-3.85032593330342,-3.62573186469175,
36.8285569847793));
#38696=CARTESIAN_POINT('Ctrl Pts',(-1.64720354707418,-5.02570013250056,
36.9079288748327));
#38697=CARTESIAN_POINT('Ctrl Pts',(0.957173977199105,-5.20141897223083,
36.9873007648861));
#38698=CARTESIAN_POINT('Ctrl Pts',(3.32838603929536,-4.11008366347129,37.0666726549395));
#38699=CARTESIAN_POINT('Ctrl Pts',(4.88881062947681,-2.01754107180608,37.1460445449929));
#38700=CARTESIAN_POINT('Ctrl Pts',(5.25833177151655,0.566470059199757,37.2254164350463));
#38701=CARTESIAN_POINT('Ctrl Pts',(4.34693493313475,3.01249033764469,37.3047883250998));
#38702=CARTESIAN_POINT('Ctrl Pts',(2.37663436681862,4.72467463787371,37.3841602151531));
#38703=CARTESIAN_POINT('Ctrl Pts',(-0.17260907066365,5.28593865420645,37.4635321052065));
#38704=CARTESIAN_POINT('Ctrl Pts',(-2.67980532059584,4.55955971460153,37.54290399526));
#38705=CARTESIAN_POINT('Ctrl Pts',(-4.53420692607955,2.72248212093334,37.6222758853133));
#38706=CARTESIAN_POINT('Ctrl Pts',(-5.28408576066665,0.222213908718847,
37.7016477753668));
#38707=CARTESIAN_POINT('Ctrl Pts',(-4.74677300008161,-2.33218511979937,
37.7810196654201));
#38708=CARTESIAN_POINT('Ctrl Pts',(-3.05315684347904,-4.31846901533503,
37.8603915554736));
#38709=CARTESIAN_POINT('Ctrl Pts',(-0.615798437855754,-5.25278341751105,
37.9397634455269));
#38710=CARTESIAN_POINT('Ctrl Pts',(1.97156710418767,-4.90753140600709,38.0191353355804));
#38711=CARTESIAN_POINT('Ctrl Pts',(4.07866326363087,-3.36681560666115,38.0985072256337));
#38712=CARTESIAN_POINT('Ctrl Pts',(5.19220608004019,-1.00595097780572,38.1778791156872));
#38713=CARTESIAN_POINT('Ctrl Pts',(5.04093898806991,1.59996108252017,38.2572510057405));
#38714=CARTESIAN_POINT('Ctrl Pts',(3.66171031660113,3.81612616476472,38.336622895794));
#38715=CARTESIAN_POINT('Ctrl Pts',(1.39049711694169,5.10269135980963,38.4159947858473));
#38716=CARTESIAN_POINT('Ctrl Pts',(-1.21943810235573,5.14625223481529,38.4953666759008));
#38717=CARTESIAN_POINT('Ctrl Pts',(-3.53232089954511,3.93619745533324,38.5747385659542));
#38718=CARTESIAN_POINT('Ctrl Pts',(-4.98473814342406,1.76729369047725,38.6541104560076));
#38719=CARTESIAN_POINT('Ctrl Pts',(-5.22288421068334,-0.832118909543577,
38.733482346061));
#38720=CARTESIAN_POINT('Ctrl Pts',(-4.18874724188046,-3.22882917750522,
38.8128542361144));
#38721=CARTESIAN_POINT('Ctrl Pts',(-2.13424072225093,-4.83900381899058,
38.8922261261678));
#38722=CARTESIAN_POINT('Ctrl Pts',(0.440162123945958,-5.27040781417516,
38.9715980162212));
#38723=CARTESIAN_POINT('Ctrl Pts',(2.90734243084964,-4.41795218255951,39.0509699062746));
#38724=CARTESIAN_POINT('Ctrl Pts',(4.66630059499982,-2.48929308216594,39.130341796328));
#38725=CARTESIAN_POINT('Ctrl Pts',(5.288558190933,0.0457521216721363,39.2097136863814));
#38726=CARTESIAN_POINT('Ctrl Pts',(4.62253485344793,2.56965255248844,39.2890855764349));
#38727=CARTESIAN_POINT('Ctrl Pts',(2.83047200092405,4.46759066254981,39.3684574664882));
#38728=CARTESIAN_POINT('Ctrl Pts',(0.34891291852996,5.27723479734496,39.4478293565417));
#38729=CARTESIAN_POINT('Ctrl Pts',(-2.21764149317963,4.80135391043001,39.527201246595));
#38730=CARTESIAN_POINT('Ctrl Pts',(-4.24398161873814,3.15587819282133,39.6065731366485));
#38731=CARTESIAN_POINT('Ctrl Pts',(-5.23650047694821,0.74162931109825,39.6859450267018));
#38732=CARTESIAN_POINT('Ctrl Pts',(-4.9534132521342,-1.85326330477585,39.7653169167553));
#38733=CARTESIAN_POINT('Ctrl Pts',(-3.46369715057683,-3.99673439595749,
39.8446888068086));
#38734=CARTESIAN_POINT('Ctrl Pts',(-1.13021013185916,-5.16655447652188,
39.9240606968621));
#38735=CARTESIAN_POINT('Ctrl Pts',(1.47855208450035,-5.0779179090888,40.0034325869154));
#38736=CARTESIAN_POINT('Ctrl Pts',(3.72722085031374,-3.75211381890458,40.0828044769689));
#38737=CARTESIAN_POINT('Ctrl Pts',(5.06779668194711,-1.51268081279862,40.1621763670222));
#38738=CARTESIAN_POINT('Ctrl Pts',(5.17416686787614,1.09598291074358,40.2415482570757));
#38739=CARTESIAN_POINT('Ctrl Pts',(4.40436067122798,2.65600709442752,40.2944628504446));
#38740=CARTESIAN_POINT('Ctrl Pts',(3.85627053850219,3.29705846079199,40.3209201471291));
#38741=CARTESIAN_POINT('Ctrl Pts',(1.26508527942741,-4.72177922709091,-0.106973382376351));
#38742=CARTESIAN_POINT('Ctrl Pts',(2.05001543279104,-4.51147638686031,-0.0805160856918833));
#38743=CARTESIAN_POINT('Ctrl Pts',(3.5121928105948,-3.69213734276823,-0.0276014923229477));
#38744=CARTESIAN_POINT('Ctrl Pts',(4.85026808817394,-1.56206090154413,0.0517703977304561));
#38745=CARTESIAN_POINT('Ctrl Pts',(5.00665954563268,0.947775616877177,0.13114228778386));
#38746=CARTESIAN_POINT('Ctrl Pts',(3.94352649879584,3.22711800485082,0.210514177837264));
#38747=CARTESIAN_POINT('Ctrl Pts',(1.91971357759781,4.72014150668349,0.289886067890667));
#38748=CARTESIAN_POINT('Ctrl Pts',(-0.571713243107534,5.06345468357225,
0.369257957944071));
#38749=CARTESIAN_POINT('Ctrl Pts',(-2.92388473013463,4.17326556172555,0.448629847997474));
#38750=CARTESIAN_POINT('Ctrl Pts',(-4.56379761866667,2.26650781142313,0.528001738050878));
#38751=CARTESIAN_POINT('Ctrl Pts',(-5.091983083909,-0.192381913949067,0.607373628104282));
#38752=CARTESIAN_POINT('Ctrl Pts',(-4.37977084759389,-2.6043995219968,0.686745518157685));
#38753=CARTESIAN_POINT('Ctrl Pts',(-2.60065712992448,-4.3819955716546,0.766117408211089));
#38754=CARTESIAN_POINT('Ctrl Pts',(-0.188028560849166,-5.09214486895681,
0.845489298264494));
#38755=CARTESIAN_POINT('Ctrl Pts',(2.27040306822816,-4.56186018168567,0.924861188317896));
#38756=CARTESIAN_POINT('Ctrl Pts',(4.17576968427582,-2.92031579800744,1.0042330783713));
#38757=CARTESIAN_POINT('Ctrl Pts',(5.06392796926476,-0.567389296122094,
1.0836049684247));
#38758=CARTESIAN_POINT('Ctrl Pts',(4.71852465152963,1.92375216574099,1.16297685847811));
#38759=CARTESIAN_POINT('Ctrl Pts',(3.22369915083516,3.94627176108661,1.24234874853151));
#38760=CARTESIAN_POINT('Ctrl Pts',(0.943587684251177,5.00748834177841,1.32172063858492));
#38761=CARTESIAN_POINT('Ctrl Pts',(-1.5663796598258,4.84889181906687,1.40109252863832));
#38762=CARTESIAN_POINT('Ctrl Pts',(-3.69478038260539,3.50911599649364,1.48046441869172));
#38763=CARTESIAN_POINT('Ctrl Pts',(-4.92314078418047,1.3145272768326,1.55983630874512));
#38764=CARTESIAN_POINT('Ctrl Pts',(-4.9522349869947,-1.20027737376273,1.63920819879853));
#38765=CARTESIAN_POINT('Ctrl Pts',(-3.77497570905141,-3.4226971150208,1.71858008885193));
#38766=CARTESIAN_POINT('Ctrl Pts',(-1.67814070389166,-4.81135541393673,
1.79795197890534));
#38767=CARTESIAN_POINT('Ctrl Pts',(0.827485662097738,-5.02797818437314,
1.87732386895874));
#38768=CARTESIAN_POINT('Ctrl Pts',(3.13153835248109,-4.01979659801894,1.95669575901214));
#38769=CARTESIAN_POINT('Ctrl Pts',(4.6727552317042,-2.03240145822472,2.03606764906555));
#38770=CARTESIAN_POINT('Ctrl Pts',(5.07569927947279,0.450082178237972,2.11543953911895));
#38771=CARTESIAN_POINT('Ctrl Pts',(4.24221421762082,2.82292679227462,2.19481142917235));
#38772=CARTESIAN_POINT('Ctrl Pts',(2.37533516234403,4.50811268818069,2.27418331922576));
#38773=CARTESIAN_POINT('Ctrl Pts',(-0.0701702807675918,5.09513231177087,
2.35355520927916));
#38774=CARTESIAN_POINT('Ctrl Pts',(-2.49858239880191,4.44098898210475,2.43292709933257));
#38775=CARTESIAN_POINT('Ctrl Pts',(-4.31834537500726,2.70503056635658,2.51229898938597));
#38776=CARTESIAN_POINT('Ctrl Pts',(-5.08616897635574,0.310132692129504,
2.59167087943937));
#38777=CARTESIAN_POINT('Ctrl Pts',(-4.61501307310829,-2.16031281943427,
2.67104276949278));
#38778=CARTESIAN_POINT('Ctrl Pts',(-3.01965020040969,-4.10451090995464,
2.75041465954618));
#38779=CARTESIAN_POINT('Ctrl Pts',(-0.688707222773715,-5.04885922799114,
2.82978654959958));
#38780=CARTESIAN_POINT('Ctrl Pts',(1.8100033099024,-4.7633166135492,2.90915843965299));
#38781=CARTESIAN_POINT('Ctrl Pts',(3.86780104266064,-3.31744061546923,2.98853032970639));
#38782=CARTESIAN_POINT('Ctrl Pts',(4.98341100265916,-1.06344342649117,3.0679022197598));
#38783=CARTESIAN_POINT('Ctrl Pts',(4.88507307300304,1.44960622728803,3.1472741098132));
#38784=CARTESIAN_POINT('Ctrl Pts',(3.59674215568923,3.60953501274882,3.2266459998666));
#38785=CARTESIAN_POINT('Ctrl Pts',(1.43225281050325,4.89018905867422,3.30601788992001));
#38786=CARTESIAN_POINT('Ctrl Pts',(-1.0811301490835,4.97960387415649,3.38538977997341));
#38787=CARTESIAN_POINT('Ctrl Pts',(-3.3311521973945,3.85599820806045,3.46476167002682));
#38788=CARTESIAN_POINT('Ctrl Pts',(-4.76971294380054,1.79307991358813,3.54413356008021));
#38789=CARTESIAN_POINT('Ctrl Pts',(-5.04638217467727,-0.706628678919173,
3.62350545013362));
#38790=CARTESIAN_POINT('Ctrl Pts',(-4.09376387778011,-3.03420408933784,
3.70287734018702));
#38791=CARTESIAN_POINT('Ctrl Pts',(-2.14391376164834,-4.62265409969061,
3.78224923024043));
#38792=CARTESIAN_POINT('Ctrl Pts',(0.328189001348338,-5.08503580343006,
3.86162112029383));
#38793=CARTESIAN_POINT('Ctrl Pts',(2.72034565005059,-4.30871404098977,3.94099301034724));
#38794=CARTESIAN_POINT('Ctrl Pts',(4.44983211978348,-2.48279907534115,4.02036490040064));
#38795=CARTESIAN_POINT('Ctrl Pts',(5.09534933467345,-0.0520797505219637,
4.09973679045404));
#38796=CARTESIAN_POINT('Ctrl Pts',(4.49965073000142,2.39132608624781,4.17910868050745));
#38797=CARTESIAN_POINT('Ctrl Pts',(2.80784716730899,4.25221018151813,4.25848057056085));
#38798=CARTESIAN_POINT('Ctrl Pts',(0.432058249724383,5.07726528867822,4.33785246061425));
#38799=CARTESIAN_POINT('Ctrl Pts',(-2.04897910114838,4.66550980985238,4.41722435066766));
#38800=CARTESIAN_POINT('Ctrl Pts',(-4.03088967831969,3.1172464682773,4.49659624072106));
#38801=CARTESIAN_POINT('Ctrl Pts',(-5.0308844520753,0.809628786937908,4.57596813077447));
#38802=CARTESIAN_POINT('Ctrl Pts',(-4.80536690897923,-1.69521267481664,
4.65534002082787));
#38803=CARTESIAN_POINT('Ctrl Pts',(-3.40927262335505,-3.78710408127548,
4.73471191088127));
#38804=CARTESIAN_POINT('Ctrl Pts',(-1.18268707297853,-4.9564653161483,4.81408380093467));
#38805=CARTESIAN_POINT('Ctrl Pts',(1.33199843054213,-4.91844257095729,4.89345569098808));
#38806=CARTESIAN_POINT('Ctrl Pts',(3.52221206471124,-3.68229810226904,4.97282758104148));
#38807=CARTESIAN_POINT('Ctrl Pts',(4.85442263620086,-1.54915396649666,5.05219947109489));
#38808=CARTESIAN_POINT('Ctrl Pts',(5.00410659859419,0.961360646520152,5.13157136114829));
#38809=CARTESIAN_POINT('Ctrl Pts',(3.93480126997208,3.23768993398037,5.21094325120169));
#38810=CARTESIAN_POINT('Ctrl Pts',(1.90698706151963,4.72532512002807,5.2903151412551));
#38811=CARTESIAN_POINT('Ctrl Pts',(-0.585364974074726,5.06188156616668,
5.3696870313085));
#38812=CARTESIAN_POINT('Ctrl Pts',(-2.93512339766788,4.1653748670719,5.44905892136191));
#38813=CARTESIAN_POINT('Ctrl Pts',(-4.56989225837456,2.25419207025927,5.52843081141531));
#38814=CARTESIAN_POINT('Ctrl Pts',(-5.09144548022617,-0.206106925298976,
5.60780270146872));
#38815=CARTESIAN_POINT('Ctrl Pts',(-4.37273385281808,-2.61619873006436,
5.68717459152211));
#38816=CARTESIAN_POINT('Ctrl Pts',(-2.58883393774572,-4.38899031504372,
5.76654648157553));
#38817=CARTESIAN_POINT('Ctrl Pts',(-0.174299805725225,-5.09263357414371,
5.84591837162892));
#38818=CARTESIAN_POINT('Ctrl Pts',(2.28269337316386,-4.5557225669355,5.92529026168233));
#38819=CARTESIAN_POINT('Ctrl Pts',(4.18362749900631,-2.90904762634266,6.00466215173574));
#38820=CARTESIAN_POINT('Ctrl Pts',(5.0654392263932,-0.553735123040447,6.08403404178913));
#38821=CARTESIAN_POINT('Ctrl Pts',(4.71332117039027,1.9364660305625,6.16340593184254));
#38822=CARTESIAN_POINT('Ctrl Pts',(3.21304851003972,3.95494834541529,6.24277782189595));
#38823=CARTESIAN_POINT('Ctrl Pts',(0.93008434460575,5.01001399745458,6.32214971194934));
#38824=CARTESIAN_POINT('Ctrl Pts',(-1.57944630846742,4.84465132919185,6.40152160200275));
#38825=CARTESIAN_POINT('Ctrl Pts',(-3.70422733684302,3.49914232059178,6.48089349205615));
#38826=CARTESIAN_POINT('Ctrl Pts',(-4.92666678513181,1.30124998791572,6.56026538210956));
#38827=CARTESIAN_POINT('Ctrl Pts',(-4.94898110955443,-1.21362396154863,
6.63963727216295));
#38828=CARTESIAN_POINT('Ctrl Pts',(-3.76573459007348,-3.43286180029078,
6.71900916221637));
#38829=CARTESIAN_POINT('Ctrl Pts',(-1.66516345976277,-4.81586210299283,
6.79838105226976));
#38830=CARTESIAN_POINT('Ctrl Pts',(0.841037803569352,-5.02572905713577,
6.87775294232318));
#38831=CARTESIAN_POINT('Ctrl Pts',(3.14236411955759,-4.01133953722303,6.95712483237658));
#38832=CARTESIAN_POINT('Ctrl Pts',(4.6782174915266,-2.0197965849922,7.03649672242998));
#38833=CARTESIAN_POINT('Ctrl Pts',(5.0744674376185,0.463764344598802,7.11586861248339));
#38834=CARTESIAN_POINT('Ctrl Pts',(4.23458834804968,2.83435330637052,7.19524050253678));
#38835=CARTESIAN_POINT('Ctrl Pts',(2.36317290999828,4.51450007644499,7.2746123925902));
#38836=CARTESIAN_POINT('Ctrl Pts',(-0.0839062181341898,5.09492462057389,
7.35398428264359));
#38837=CARTESIAN_POINT('Ctrl Pts',(-2.51054597725242,4.43423680455535,7.433356172697));
#38838=CARTESIAN_POINT('Ctrl Pts',(-4.32562229331123,2.69337871796382,7.5127280627504));
#38839=CARTESIAN_POINT('Ctrl Pts',(-5.08698659332198,0.296419537368979,
7.5920999528038));
#38840=CARTESIAN_POINT('Ctrl Pts',(-4.60917221905333,-2.17274678641544,
7.67147184285721));
#38841=CARTESIAN_POINT('Ctrl Pts',(-3.00857369445294,-4.11263680232249,
7.75084373291061));
#38842=CARTESIAN_POINT('Ctrl Pts',(-0.675093277248738,-5.05069759635094,
7.83021562296402));
#38843=CARTESIAN_POINT('Ctrl Pts',(1.82283836799964,-4.7584196354378,7.90958751301742));
#38844=CARTESIAN_POINT('Ctrl Pts',(3.8767306215876,-3.30700118391521,7.98895940307083));
#38845=CARTESIAN_POINT('Ctrl Pts',(4.9862598767545,-1.05000456391383,8.06833129312422));
#38846=CARTESIAN_POINT('Ctrl Pts',(4.881147262843,1.46277084371127,8.14770318317763));
#38847=CARTESIAN_POINT('Ctrl Pts',(3.58699797993919,3.61921851159664,8.22707507323104));
#38848=CARTESIAN_POINT('Ctrl Pts',(1.41906392880751,4.89403256106139,8.30644696328444));
#38849=CARTESIAN_POINT('Ctrl Pts',(-1.09455095433695,4.97667111140887,8.38581885333784));
#38850=CARTESIAN_POINT('Ctrl Pts',(-3.34153564775234,3.84700359469183,8.46519074339125));
#38851=CARTESIAN_POINT('Ctrl Pts',(-4.77452965373897,1.7802145175059,8.54456263344465));
#38852=CARTESIAN_POINT('Ctrl Pts',(-5.04445880431694,-0.720230875706447,
8.62393452349805));
#38853=CARTESIAN_POINT('Ctrl Pts',(-4.08556895588349,-3.04522962180074,
8.70330641355146));
#38854=CARTESIAN_POINT('Ctrl Pts',(-2.1314435530503,-4.62841717252583,8.78267830360486));
#38855=CARTESIAN_POINT('Ctrl Pts',(0.341896781435676,-5.08413254485124,
8.86205019365827));
#38856=CARTESIAN_POINT('Ctrl Pts',(2.73195181673958,-4.30136448278739,8.94142208371167));
#38857=CARTESIAN_POINT('Ctrl Pts',(4.45650943655852,-2.47079355362535,9.02079397376506));
#38858=CARTESIAN_POINT('Ctrl Pts',(5.09547122194811,-0.0383427838088964,
9.10016586381848));
#38859=CARTESIAN_POINT('Ctrl Pts',(4.49318749630538,2.40344820327308,9.17953775387187));
#38860=CARTESIAN_POINT('Ctrl Pts',(2.79637324206448,4.25976452798008,9.25890964392529));
#38861=CARTESIAN_POINT('Ctrl Pts',(0.418368655723882,5.07841164249998,9.33828153397869));
#38862=CARTESIAN_POINT('Ctrl Pts',(-2.06154960910779,4.65996892178041,9.41765342403209));
#38863=CARTESIAN_POINT('Ctrl Pts',(-4.03927895232343,3.10636808638134,9.49702531408549));
#38864=CARTESIAN_POINT('Ctrl Pts',(-5.03304888354539,0.79606286096894,9.5763972041389));
#38865=CARTESIAN_POINT('Ctrl Pts',(-4.80077924720044,-1.70816151532024,
9.6557690941923));
#38866=CARTESIAN_POINT('Ctrl Pts',(-3.39905041258209,-3.7962815274288,9.7351409842457));
#38867=CARTESIAN_POINT('Ctrl Pts',(-1.16932042112922,-4.95963576238233,
9.81451287429911));
#38868=CARTESIAN_POINT('Ctrl Pts',(1.34525343666388,-4.91483370358709,9.89388476435251));
#38869=CARTESIAN_POINT('Ctrl Pts',(3.53212653495364,-3.67278903339792,9.97325665440591));
#38870=CARTESIAN_POINT('Ctrl Pts',(4.85858142755815,-1.53606108425365,10.0526285444593));
#38871=CARTESIAN_POINT('Ctrl Pts',(5.00149663869711,0.974847945001263,10.1320004345127));
#38872=CARTESIAN_POINT('Ctrl Pts',(3.92605833927446,3.24828617264322,10.2113723245661));
#38873=CARTESIAN_POINT('Ctrl Pts',(1.89424091858727,4.73044907858876,10.2907442146195));
#38874=CARTESIAN_POINT('Ctrl Pts',(-0.599009397036607,5.0602850596615,10.3701161046729));
#38875=CARTESIAN_POINT('Ctrl Pts',(-2.94634234942717,4.15744680095171,10.4494879947264));
#38876=CARTESIAN_POINT('Ctrl Pts',(-4.57595282711548,2.24186370388246,10.5288598847797));
#38877=CARTESIAN_POINT('Ctrl Pts',(-5.09087132481819,-0.219832429171425,
10.6082317748331));
#38878=CARTESIAN_POINT('Ctrl Pts',(-4.36566483624775,-2.62797786906995,
10.6876036648866));
#38879=CARTESIAN_POINT('Ctrl Pts',(-2.57699205680257,-4.39595371699339,
10.7669755549399));
#38880=CARTESIAN_POINT('Ctrl Pts',(-0.160569716395434,-5.09308496973576,
10.8463474449934));
#38881=CARTESIAN_POINT('Ctrl Pts',(2.2949670515106,-4.54955199720284,10.9257193350468));
#38882=CARTESIAN_POINT('Ctrl Pts',(4.19145492549203,-2.89775822841384,11.0050912251002));
#38883=CARTESIAN_POINT('Ctrl Pts',(5.06691365725173,-0.540076969262297,
11.0844631151535));
#38884=CARTESIAN_POINT('Ctrl Pts',(4.70808343752805,1.94916584416147,11.163835005207));
#38885=CARTESIAN_POINT('Ctrl Pts',(3.20237451358847,3.96359617235289,11.2432068952604));
#38886=CARTESIAN_POINT('Ctrl Pts',(0.916574246474504,5.01250324623051,11.3225787853138));
#38887=CARTESIAN_POINT('Ctrl Pts',(-1.59250147827797,4.84037562431409,11.4019506753672));
#38888=CARTESIAN_POINT('Ctrl Pts',(-3.71364736786416,3.4891432143045,11.4813225654206));
#38889=CARTESIAN_POINT('Ctrl Pts',(-4.93015697865768,1.28796324037784,11.560694455474));
#38890=CARTESIAN_POINT('Ctrl Pts',(-4.94569126216756,-1.22696172804661,
11.6400663455274));
#38891=CARTESIAN_POINT('Ctrl Pts',(-3.75646610131532,-3.44300153535262,
11.7194382355808));
#38892=CARTESIAN_POINT('Ctrl Pts',(-1.65217411297936,-4.82033378960134,
11.7988101256342));
#38893=CARTESIAN_POINT('Ctrl Pts',(0.854583832252985,-5.02344340233105,
11.8781820156876));
#38894=CARTESIAN_POINT('Ctrl Pts',(3.15316704753777,-4.00285332145629,11.957553905741));
#38895=CARTESIAN_POINT('Ctrl Pts',(4.6836457494592,-2.00717703164028,12.0369257957944));
#38896=CARTESIAN_POINT('Ctrl Pts',(5.07319871388639,0.477443140272258,12.1162976858478));
#38897=CARTESIAN_POINT('Ctrl Pts',(4.22693170094574,2.84575922001696,12.1956695759012));
#38898=CARTESIAN_POINT('Ctrl Pts',(2.35099348180933,4.52085465274672,12.2750414659546));
#38899=CARTESIAN_POINT('Ctrl Pts',(-0.0976415456600611,5.09467989880942,
12.354413356008));
#38900=CARTESIAN_POINT('Ctrl Pts',(-2.52249130873252,4.4274523984048,12.4337852460614));
#38901=CARTESIAN_POINT('Ctrl Pts',(-4.33286777243754,2.68170729374847,12.5131571361148));
#38902=CARTESIAN_POINT('Ctrl Pts',(-5.08776723741693,0.282704228193439,
12.5925290261682));
#38903=CARTESIAN_POINT('Ctrl Pts',(-4.60329786494335,-2.18516496159434,
12.6719009162216));
#38904=CARTESIAN_POINT('Ctrl Pts',(-2.99747532179655,-4.12073280351837,
12.751272806275));
#38905=CARTESIAN_POINT('Ctrl Pts',(-0.661474425059184,-5.05249925559264,
12.8306446963284));
#38906=CARTESIAN_POINT('Ctrl Pts',(1.83566017747378,-4.75348807252195,12.9100165863819));
#38907=CARTESIAN_POINT('Ctrl Pts',(3.885632023939,-3.29653771665232,12.9893884764353));
#38908=CARTESIAN_POINT('Ctrl Pts',(4.98907251007332,-1.03655806976862,13.0687603664887));
#38909=CARTESIAN_POINT('Ctrl Pts',(4.87718597587842,1.47592482852836,13.1481322565421));
#38910=CARTESIAN_POINT('Ctrl Pts',(3.5772277334276,3.62887570549998,13.2275041465955));
#38911=CARTESIAN_POINT('Ctrl Pts',(1.4058647331731,4.89784049299196,13.3068760366489));
#38912=CARTESIAN_POINT('Ctrl Pts',(-1.10796380425358,4.97370217757714,13.3862479267023));
#38913=CARTESIAN_POINT('Ctrl Pts',(-3.35189481140037,3.83798102080754,13.4656198167557));
#38914=CARTESIAN_POINT('Ctrl Pts',(-4.77931166178332,1.76733618259613,13.5449917068091));
#38915=CARTESIAN_POINT('Ctrl Pts',(-5.0424987701828,-0.733827837763376,
13.6243635968625));
#38916=CARTESIAN_POINT('Ctrl Pts',(-4.07734433954749,-3.0562330211441,13.7037354869159));
#38917=CARTESIAN_POINT('Ctrl Pts',(-2.11895785284703,-4.6341466054312,13.7831073769693));
#38918=CARTESIAN_POINT('Ctrl Pts',(0.355602076573349,-5.08319233414479,
13.8624792670227));
#38919=CARTESIAN_POINT('Ctrl Pts',(2.74353812725229,-4.29398366171607,13.9418511570761));
#38920=CARTESIAN_POINT('Ctrl Pts',(4.4631543628512,-2.45877007386494,14.0212230471295));
#38921=CARTESIAN_POINT('Ctrl Pts',(5.09555607468418,-0.024605538415575,
14.1005949371829));
#38922=CARTESIAN_POINT('Ctrl Pts',(4.48669160554615,2.41555285172843,14.1799668272363));
#38923=CARTESIAN_POINT('Ctrl Pts',(2.78487899242048,4.26728791392691,14.2593387172897));
#38924=CARTESIAN_POINT('Ctrl Pts',(0.404676020966283,5.07952108577437,14.3387106073431));
#38925=CARTESIAN_POINT('Ctrl Pts',(-2.07410513346011,4.65439416445642,14.4180824973965));
#38926=CARTESIAN_POINT('Ctrl Pts',(-4.0476388683295,3.09546712700361,14.4974543874499));
#38927=CARTESIAN_POINT('Ctrl Pts',(-5.03517673417046,0.782491149112972,
14.5768262775033));
#38928=CARTESIAN_POINT('Ctrl Pts',(-4.79615669274215,-1.72109794068678,
14.6561981675567));
#38929=CARTESIAN_POINT('Ctrl Pts',(-3.38880349707463,-3.80543138172091,
14.7355700576101));
#38930=CARTESIAN_POINT('Ctrl Pts',(-1.15594527050905,-4.96277016134733,
14.8149419476636));
#38931=CARTESIAN_POINT('Ctrl Pts',(1.35849866531108,-4.91118911457496,14.8943138377169));
#38932=CARTESIAN_POINT('Ctrl Pts',(3.54201533324722,-3.66325327022487,14.9736857277704));
#38933=CARTESIAN_POINT('Ctrl Pts',(4.86270490612231,-1.52295703772157,15.0530576178238));
#38934=CARTESIAN_POINT('Ctrl Pts',(4.99885032728073,0.988328158162469,15.1324295078772));
#38935=CARTESIAN_POINT('Ctrl Pts',(3.91728687348112,3.25885880234541,15.2118013979306));
#38936=CARTESIAN_POINT('Ctrl Pts',(1.8814810080689,4.73553865563863,15.291173287984));
#38937=CARTESIAN_POINT('Ctrl Pts',(-0.612649466321345,5.05865177435528,
15.3705451780374));
#38938=CARTESIAN_POINT('Ctrl Pts',(-2.95753988679226,4.14948851797474,15.4499170680908));
#38939=CARTESIAN_POINT('Ctrl Pts',(-4.58198013724412,2.22951904335266,15.5292889581442));
#38940=CARTESIAN_POINT('Ctrl Pts',(-5.09026016830427,-0.233556335273548,
15.6086608481976));
#38941=CARTESIAN_POINT('Ctrl Pts',(-4.35856408946536,-2.63973790759512,
15.688032738251));
#38942=CARTESIAN_POINT('Ctrl Pts',(-2.56513144595043,-4.40288516858759,
15.7674046283044));
#38943=CARTESIAN_POINT('Ctrl Pts',(-0.146838460024607,-5.09349934813251,
15.8467765183578));
#38944=CARTESIAN_POINT('Ctrl Pts',(2.3072240497427,-4.54334836074314,15.9261484084112));
#38945=CARTESIAN_POINT('Ctrl Pts',(4.19925188794477,-2.88644776920547,16.0055202984646));
#38946=CARTESIAN_POINT('Ctrl Pts',(5.06835126113318,-0.526414890137456,
16.084892188518));
#38947=CARTESIAN_POINT('Ctrl Pts',(4.70281148570858,1.96185149097663,16.1642640785714));
#38948=CARTESIAN_POINT('Ctrl Pts',(3.19167724187374,3.97221519135797,16.2436359686248));
#38949=CARTESIAN_POINT('Ctrl Pts',(0.90305748655408,5.01495606350291,16.3230078586782));
#38950=CARTESIAN_POINT('Ctrl Pts',(-1.60554507356452,4.83606473894038,16.4023797487316));
#38951=CARTESIAN_POINT('Ctrl Pts',(-3.72304040765551,3.47911874852373,16.481751638785));
#38952=CARTESIAN_POINT('Ctrl Pts',(-4.93361133910263,1.27466713166901,16.5611235288384));
#38953=CARTESIAN_POINT('Ctrl Pts',(-4.94236546898943,-1.24029057666156,
16.6404954188918));
#38954=CARTESIAN_POINT('Ctrl Pts',(-3.74717030983909,-3.45311624655429,
16.7198673089452));
#38955=CARTESIAN_POINT('Ctrl Pts',(-1.6391727584367,-4.82477044080732,16.7992391989986));
#38956=CARTESIAN_POINT('Ctrl Pts',(0.868123650569205,-5.02112123762451,
16.8786110890521));
#38957=CARTESIAN_POINT('Ctrl Pts',(3.16394705627606,-3.99433801030565,16.9579829791054));
#38958=CARTESIAN_POINT('Ctrl Pts',(4.68903996911093,-1.99454289389466,17.0373548691589));
#38959=CARTESIAN_POINT('Ctrl Pts',(5.07189311172224,0.491118473430398,17.1167267592122));
#38960=CARTESIAN_POINT('Ctrl Pts',(4.21924434286031,2.85714443596481,17.1960986492657));
#38961=CARTESIAN_POINT('Ctrl Pts',(2.33879694571596,4.52717639800277,17.275470539319));
#38962=CARTESIAN_POINT('Ctrl Pts',(-0.11137612465114,5.09439809707615,17.3548424293725));
#38963=CARTESIAN_POINT('Ctrl Pts',(-2.53441837980398,4.42063590960358,17.4342143194259));
#38964=CARTESIAN_POINT('Ctrl Pts',(-4.34008162116489,2.67001619606203,17.5135862094793));
#38965=CARTESIAN_POINT('Ctrl Pts',(-5.08851116459639,0.268987208843763,
17.5929580995327));
#38966=CARTESIAN_POINT('Ctrl Pts',(-4.59738955946409,-2.19756790530666,
17.6723299895861));
#38967=CARTESIAN_POINT('Ctrl Pts',(-2.98635609589589,-4.12879762624818,
17.7517018796395));
#38968=CARTESIAN_POINT('Ctrl Pts',(-0.647849003889666,-5.05426651218747,
17.8310737696929));
#38969=CARTESIAN_POINT('Ctrl Pts',(1.84846531944351,-4.7485175808327,17.9104456597463));
#38970=CARTESIAN_POINT('Ctrl Pts',(3.89451146459875,-3.28605855970652,17.9898175497997));
#38971=CARTESIAN_POINT('Ctrl Pts',(4.99183702504825,-1.02308842638974,18.0691894398531));
#38972=CARTESIAN_POINT('Ctrl Pts',(4.87321162956217,1.48903860109228,18.1485613299065));
#38973=CARTESIAN_POINT('Ctrl Pts',(3.5673892128293,3.63856219800459,18.2279332199599));
#38974=CARTESIAN_POINT('Ctrl Pts',(1.39273514199697,4.90150770362139,18.3073051100133));
#38975=CARTESIAN_POINT('Ctrl Pts',(-1.12151932172649,4.97089558679471,18.3866770000667));
#38976=CARTESIAN_POINT('Ctrl Pts',(-3.36194502775882,3.82855576883779,18.4660488901201));
#38977=CARTESIAN_POINT('Ctrl Pts',(-4.78459624359504,1.75515257798274,18.5454207801735));
#38978=CARTESIAN_POINT('Ctrl Pts',(-5.03948789886558,-0.748754766453475,
18.6247926702269));
#38979=CARTESIAN_POINT('Ctrl Pts',(-4.0710021077043,-3.06469899064074,18.7041645602803));
#38980=CARTESIAN_POINT('Ctrl Pts',(-2.10287077052062,-4.64454172754396,
18.7835364503337));
#38981=CARTESIAN_POINT('Ctrl Pts',(0.36273133865386,-5.07374792580598,18.8629083403871));
#38982=CARTESIAN_POINT('Ctrl Pts',(3.56709774791096,-4.04128406294332,18.968737527125));
#38983=CARTESIAN_POINT('Ctrl Pts',(5.77704085522352,-0.0189872057267309,
19.1010240105473));
#38984=CARTESIAN_POINT('Ctrl Pts',(3.14459942081972,4.8501664079131,19.2597677906541));
#38985=CARTESIAN_POINT('Ctrl Pts',(-2.36591519662263,5.26902047281295,19.418511570761));
#38986=CARTESIAN_POINT('Ctrl Pts',(-5.71123844601178,0.872727032859995,
19.5772553508678));
#38987=CARTESIAN_POINT('Ctrl Pts',(-3.83058845612596,-4.3254192567976,19.7359991309746));
#38988=CARTESIAN_POINT('Ctrl Pts',(1.55524717023751,-5.5639435857319,19.8947429110814));
#38989=CARTESIAN_POINT('Ctrl Pts',(5.51805139390222,-1.71188403765725,20.0534866911882));
#38990=CARTESIAN_POINT('Ctrl Pts',(4.43131449514919,3.70671199728542,20.212230471295));
#38991=CARTESIAN_POINT('Ctrl Pts',(-0.709818611660639,5.73400533709385,
20.3709742514018));
#38992=CARTESIAN_POINT('Ctrl Pts',(-5.20235975367858,2.51303602329798,20.5297180315086));
#38993=CARTESIAN_POINT('Ctrl Pts',(-4.93271294602024,-3.0047419943643,20.6884618116154));
#38994=CARTESIAN_POINT('Ctrl Pts',(-0.152720854580618,-5.77834717219765,
20.8472055917222));
#38995=CARTESIAN_POINT('Ctrl Pts',(4.77339715849037,-3.25411141853181,21.005949371829));
#38996=CARTESIAN_POINT('Ctrl Pts',(5.22808970274015,1.3127228499015,21.1382358552514));
#38997=CARTESIAN_POINT('Ctrl Pts',(3.1707451501151,3.97754537770267,21.2440650419892));
#38998=CARTESIAN_POINT('Ctrl Pts',(0.895150293052777,5.019216999618,21.3234369320426));
#38999=CARTESIAN_POINT('Ctrl Pts',(-1.62157688245131,4.83072732396133,21.402808822096));
#39000=CARTESIAN_POINT('Ctrl Pts',(-3.73081451079173,3.46959580775127,21.4821807121495));
#39001=CARTESIAN_POINT('Ctrl Pts',(-4.93787328845979,1.26108254025601,21.5615526022028));
#39002=CARTESIAN_POINT('Ctrl Pts',(-4.93855701420288,-1.25346250930809,
21.6409244922563));
#39003=CARTESIAN_POINT('Ctrl Pts',(-3.73808388472054,-3.46328419200818,
21.7202963823096));
#39004=CARTESIAN_POINT('Ctrl Pts',(-1.62603418385006,-4.82913054051807,
21.7996682723631));
#39005=CARTESIAN_POINT('Ctrl Pts',(0.881590795203928,-5.01878454751451,
21.8790401624164));
#39006=CARTESIAN_POINT('Ctrl Pts',(3.17473921804455,-3.98578203611947,21.9584120524699));
#39007=CARTESIAN_POINT('Ctrl Pts',(4.69438148876591,-1.98190041394297,22.0377839425233));
#39008=CARTESIAN_POINT('Ctrl Pts',(5.0705605156318,0.504793485523968,22.1171558325767));
#39009=CARTESIAN_POINT('Ctrl Pts',(4.21152107628908,2.86850718608746,22.1965277226301));
#39010=CARTESIAN_POINT('Ctrl Pts',(2.32658621700133,4.53346610033867,22.2758996126835));
#39011=CARTESIAN_POINT('Ctrl Pts',(-0.125111436169825,5.09407888617233,
22.3552715027369));
#39012=CARTESIAN_POINT('Ctrl Pts',(-2.54632610813663,4.41378735452051,22.4346433927903));
#39013=CARTESIAN_POINT('Ctrl Pts',(-4.34726461344783,2.6583059213356,22.5140152828437));
#39014=CARTESIAN_POINT('Ctrl Pts',(-5.08921736705482,0.255267617363269,
22.5933871728972));
#39015=CARTESIAN_POINT('Ctrl Pts',(-4.59144894277882,-2.20995361377114,
22.6727590629504));
#39016=CARTESIAN_POINT('Ctrl Pts',(-2.97521323819314,-4.13683487704257,
22.7521309530039));
#39017=CARTESIAN_POINT('Ctrl Pts',(-0.634222428965717,-5.05599240530685,
22.8315028430573));
#39018=CARTESIAN_POINT('Ctrl Pts',(1.8612636949988,-4.74352133023588,22.9108747331107));
#39019=CARTESIAN_POINT('Ctrl Pts',(3.90335003127195,-3.27553898237365,22.9902466231641));
#39020=CARTESIAN_POINT('Ctrl Pts',(4.99458897767401,-1.00964257616381,23.0696185132175));
#39021=CARTESIAN_POINT('Ctrl Pts',(4.86915708441603,1.5022005201609,23.1489904032709));
#39022=CARTESIAN_POINT('Ctrl Pts',(3.55760931370069,3.6481108983516,23.2283622933243));
#39023=CARTESIAN_POINT('Ctrl Pts',(1.37943578318338,4.90534953479997,23.3077341833777));
#39024=CARTESIAN_POINT('Ctrl Pts',(-1.13476524781216,4.96765588336336,23.3871060734311));
#39025=CARTESIAN_POINT('Ctrl Pts',(-3.37253997777701,3.81985225393738,23.4664779634845));
#39026=CARTESIAN_POINT('Ctrl Pts',(-4.78877143331127,1.74154107082816,23.545849853538));
#39027=CARTESIAN_POINT('Ctrl Pts',(-5.03846876789875,-0.76100566244534,
23.6252217435914));
#39028=CARTESIAN_POINT('Ctrl Pts',(-4.06080626285345,-3.07817310072711,
23.7045936336447));
#39029=CARTESIAN_POINT('Ctrl Pts',(-2.09394034074327,-4.64550438513341,
23.7839655236982));
#39030=CARTESIAN_POINT('Ctrl Pts',(0.383004813579298,-5.08120108394905,
23.8633374137515));
#39031=CARTESIAN_POINT('Ctrl Pts',(2.76665084304599,-4.27912844577405,23.942709303805));
#39032=CARTESIAN_POINT('Ctrl Pts',(4.47634685104287,-2.43466958989253,24.0220811938583));
#39033=CARTESIAN_POINT('Ctrl Pts',(5.0956146743416,0.00286938903386649,
24.1014530839118));
#39034=CARTESIAN_POINT('Ctrl Pts',(4.47360204192767,2.4397093911446,24.1808249739652));
#39035=CARTESIAN_POINT('Ctrl Pts',(2.76182985424755,4.28224158577674,24.2601968640186));
#39036=CARTESIAN_POINT('Ctrl Pts',(0.377282027280861,5.08162920869509,24.339568754072));
#39037=CARTESIAN_POINT('Ctrl Pts',(-2.09917086643256,4.64314320437055,24.4189406441253));
#39038=CARTESIAN_POINT('Ctrl Pts',(-4.06427038351852,3.07359779288466,24.4983125341788));
#39039=CARTESIAN_POINT('Ctrl Pts',(-5.03932263128953,0.755330762345285,
24.5776844242322));
#39040=CARTESIAN_POINT('Ctrl Pts',(-4.78680704042971,-1.74693317000509,
24.6570563142856));
#39041=CARTESIAN_POINT('Ctrl Pts',(-3.36823584993892,-3.82364804891321,
24.736428204339));
#39042=CARTESIAN_POINT('Ctrl Pts',(-1.12916986186658,-4.96893072660747,
24.8158000943924));
#39043=CARTESIAN_POINT('Ctrl Pts',(1.38495940518137,-4.90379287784174,24.8951719844458));
#39044=CARTESIAN_POINT('Ctrl Pts',(3.56171562668277,-3.64410193839515,24.9745438744992));
#39045=CARTESIAN_POINT('Ctrl Pts',(4.87084580524804,-1.49671583283838,25.0539157645526));
#39046=CARTESIAN_POINT('Ctrl Pts',(4.99344872708924,1.01526693667351,25.133287654606));
#39047=CARTESIAN_POINT('Ctrl Pts',(3.8996585918228,3.27993292766699,25.2126595446594));
#39048=CARTESIAN_POINT('Ctrl Pts',(1.85592025533624,4.7456145174892,25.2920314347128));
#39049=CARTESIAN_POINT('Ctrl Pts',(-0.639916147340462,5.05527491509063,
25.3714033247662));
#39050=CARTESIAN_POINT('Ctrl Pts',(-2.9798703929554,4.13348153303719,25.4507752148196));
#39051=CARTESIAN_POINT('Ctrl Pts',(-4.59393480667762,2.20478119884206,25.5301471048731));
#39052=CARTESIAN_POINT('Ctrl Pts',(-5.08892686999539,-0.260998955190596,
25.6095189949264));
#39053=CARTESIAN_POINT('Ctrl Pts',(-4.34426761193083,-2.66320034145021,
25.6888908849798));
#39054=CARTESIAN_POINT('Ctrl Pts',(-2.54135437947314,-4.41665201942651,
25.7682627750333));
#39055=CARTESIAN_POINT('Ctrl Pts',(-0.119372845368366,-5.09421704156391,
25.8476346650866));
#39056=CARTESIAN_POINT('Ctrl Pts',(2.33168764964084,-4.53084206823456,25.9270065551401));
#39057=CARTESIAN_POINT('Ctrl Pts',(4.21475419430065,-2.86376399593205,26.0063784451934));
#39058=CARTESIAN_POINT('Ctrl Pts',(5.07111594642898,-0.49907935305457,26.0857503352469));
#39059=CARTESIAN_POINT('Ctrl Pts',(4.69216507873193,1.98717991553359,26.1651222253003));
#39060=CARTESIAN_POINT('Ctrl Pts',(3.17021318378706,3.98936655524586,26.2444941153537));
#39061=CARTESIAN_POINT('Ctrl Pts',(0.876004374419533,5.01975233241337,26.3238660054071));
#39062=CARTESIAN_POINT('Ctrl Pts',(-1.63159716155383,4.82733755243831,26.4032378954604));
#39063=CARTESIAN_POINT('Ctrl Pts',(-3.74174524045176,3.4589940298197,26.4826097855139));
#39064=CARTESIAN_POINT('Ctrl Pts',(-4.94041246098821,1.2480472178904,26.5619816755672));
#39065=CARTESIAN_POINT('Ctrl Pts',(-4.93560614144543,-1.26692113381128,
26.6413535656207));
#39066=CARTESIAN_POINT('Ctrl Pts',(-3.72849709062547,-3.4732703015989,26.7207254556741));
#39067=CARTESIAN_POINT('Ctrl Pts',(-1.61313440141745,-4.8335385118705,26.8000973457275));
#39068=CARTESIAN_POINT('Ctrl Pts',(0.895184257363441,-5.01636743950643,
26.8794692357809));
#39069=CARTESIAN_POINT('Ctrl Pts',(3.18543801250735,-3.97722036241957,26.9588411258343));
#39070=CARTESIAN_POINT('Ctrl Pts',(4.69972611865188,-1.96923120847525,27.0382130158877));
#39071=CARTESIAN_POINT('Ctrl Pts',(5.06917134496014,0.51845830903431,27.1175849059411));
#39072=CARTESIAN_POINT('Ctrl Pts',(4.20377765205651,2.8798525300511,27.1969567959945));
#39073=CARTESIAN_POINT('Ctrl Pts',(2.31435302801598,4.53972104919287,27.2763286860479));
#39074=CARTESIAN_POINT('Ctrl Pts',(-0.138842870915707,5.09372356925338,
27.3557005761014));
#39075=CARTESIAN_POINT('Ctrl Pts',(-2.5582169538158,4.40690630260968,27.4350724661547));
#39076=CARTESIAN_POINT('Ctrl Pts',(-4.35441504928357,2.64657641517193,27.5144443562082));
#39077=CARTESIAN_POINT('Ctrl Pts',(-5.08988727708012,0.241546371095803,
27.5938162462615));
#39078=CARTESIAN_POINT('Ctrl Pts',(-4.58547423045432,-2.22232383432546,
27.6731881363149));
#39079=CARTESIAN_POINT('Ctrl Pts',(-2.96404981106488,-4.14484087273538,
27.7525600263683));
#39080=CARTESIAN_POINT('Ctrl Pts',(-0.620589418513009,-5.05768384899663,
27.8319319164217));
#39081=CARTESIAN_POINT('Ctrl Pts',(1.87404518273727,-4.73848623463559,27.9113038064751));
#39082=CARTESIAN_POINT('Ctrl Pts',(3.91216652560138,-3.26500386197866,27.9906756965286));
#39083=CARTESIAN_POINT('Ctrl Pts',(4.9972927622627,-0.99617377550726,28.0700475865819));
#39084=CARTESIAN_POINT('Ctrl Pts',(4.86508954335677,1.51532203768447,28.1494194766354));
#39085=CARTESIAN_POINT('Ctrl Pts',(3.54776128038217,3.65768875660473,28.2287913666887));
#39086=CARTESIAN_POINT('Ctrl Pts',(1.36620622234286,4.90905059057282,28.3081632567422));
#39087=CARTESIAN_POINT('Ctrl Pts',(-1.148153647413,4.96457856667651,28.3875351467955));
#39088=CARTESIAN_POINT('Ctrl Pts',(-3.382825830054,3.81074619284609,28.466907036849));
#39089=CARTESIAN_POINT('Ctrl Pts',(-4.79344912825184,1.72862448138202,28.5462789269024));
#39090=CARTESIAN_POINT('Ctrl Pts',(-5.03639882892723,-0.774586327501372,
28.6256508169557));
#39091=CARTESIAN_POINT('Ctrl Pts',(-4.05249292275565,-3.08910962152317,
28.7050227070092));
#39092=CARTESIAN_POINT('Ctrl Pts',(-2.0814087106417,-4.65113264937009,28.7843945970626));
#39093=CARTESIAN_POINT('Ctrl Pts',(0.39670205626447,-5.08015005893792,28.863766487116));
#39094=CARTESIAN_POINT('Ctrl Pts',(2.77817708034974,-4.27165415886996,28.9431383771694));
#39095=CARTESIAN_POINT('Ctrl Pts',(4.48289431705251,-2.42259276084734,29.0225102672228));
#39096=CARTESIAN_POINT('Ctrl Pts',(5.09558842083954,0.016606871399571,29.1018821572762));
#39097=CARTESIAN_POINT('Ctrl Pts',(4.46700846420369,2.45176110653224,29.1812540473296));
#39098=CARTESIAN_POINT('Ctrl Pts',(2.75027513324334,4.28967176299481,29.260625937383));
#39099=CARTESIAN_POINT('Ctrl Pts',(0.363580867455653,5.08262787301922,29.3399978274364));
#39100=CARTESIAN_POINT('Ctrl Pts',(-2.11168089287163,4.6374670833821,29.4193697174898));
#39101=CARTESIAN_POINT('Ctrl Pts',(-4.07254186182172,3.0626295770924,29.4987416075432));
#39102=CARTESIAN_POINT('Ctrl Pts',(-5.04134064765058,0.741742284838609,
29.5781134975966));
#39103=CARTESIAN_POINT('Ctrl Pts',(-4.78208001053002,-1.75983178618322,
29.6574853876501));
#39104=CARTESIAN_POINT('Ctrl Pts',(-3.35791526779889,-3.8327147294124,29.7368572777034));
#39105=CARTESIAN_POINT('Ctrl Pts',(-1.11576979845131,-4.97195684812685,
29.8162291677569));
#39106=CARTESIAN_POINT('Ctrl Pts',(1.3981747240844,-4.90004128387741,29.8956010578102));
#39107=CARTESIAN_POINT('Ctrl Pts',(3.57152697864042,-3.63448650893289,29.9749729478637));
#39108=CARTESIAN_POINT('Ctrl Pts',(4.87486316664055,-1.48357886521172,30.054344837917));
#39109=CARTESIAN_POINT('Ctrl Pts',(4.99069347757362,1.02872530622892,30.1337167279705));
#39110=CARTESIAN_POINT('Ctrl Pts',(3.89080190408237,3.29043427011703,30.2130886180238));
#39111=CARTESIAN_POINT('Ctrl Pts',(1.84311959890063,4.75060072905731,30.2924605080773));
#39112=CARTESIAN_POINT('Ctrl Pts',(-0.653542560897256,5.05353136567563,
30.3718323981307));
#39113=CARTESIAN_POINT('Ctrl Pts',(-2.99100319945254,4.12543294741732,30.4512042881841));
#39114=CARTESIAN_POINT('Ctrl Pts',(-4.59986207909447,2.19238819465906,30.5305761782375));
#39115=CARTESIAN_POINT('Ctrl Pts',(-5.08820473789096,-0.274717469549192,
30.6099480682909));
#39116=CARTESIAN_POINT('Ctrl Pts',(-4.33707198508738,-2.67490256625206,
30.6893199583443));
#39117=CARTESIAN_POINT('Ctrl Pts',(-2.52943809666249,-4.42348731861233,
30.7686918483976));
#39118=CARTESIAN_POINT('Ctrl Pts',(-0.10563868670687,-5.09452035138171,
30.8480637384511));
#39119=CARTESIAN_POINT('Ctrl Pts',(2.34389407350322,-4.52453950308404,30.9274356285044));
#39120=CARTESIAN_POINT('Ctrl Pts',(4.22245942552948,-2.85239084673345,31.006807518558));
#39121=CARTESIAN_POINT('Ctrl Pts',(5.07244300775219,-0.485406093778655,
31.0861794086112));
#39122=CARTESIAN_POINT('Ctrl Pts',(4.68679070094865,1.99982250919246,31.1655512986648));
#39123=CARTESIAN_POINT('Ctrl Pts',(3.15944655342927,3.99789877545637,31.2449231887181));
#39124=CARTESIAN_POINT('Ctrl Pts',(0.862468218810821,5.02209574921795,31.3242950787715));
#39125=CARTESIAN_POINT('Ctrl Pts',(-1.64460546486892,4.82292131469039,31.4036669688249));
#39126=CARTESIAN_POINT('Ctrl Pts',(-3.75105689757904,3.44889392325951,31.4830388588783));
#39127=CARTESIAN_POINT('Ctrl Pts',(-4.94375917286251,1.23472360611981,31.5624107489317));
#39128=CARTESIAN_POINT('Ctrl Pts',(-4.93217265646195,-1.28022264845634,
31.6417826389851));
#39129=CARTESIAN_POINT('Ctrl Pts',(-3.7191197981263,-3.48330949959324,31.7211545290385));
#39130=CARTESIAN_POINT('Ctrl Pts',(-1.60009758909914,-4.83786986680406,
31.8005264190919));
#39131=CARTESIAN_POINT('Ctrl Pts',(0.908704850876668,-5.01393584290474,
31.8798983091453));
#39132=CARTESIAN_POINT('Ctrl Pts',(3.196148800563,-3.96861814583255,31.9592701991988));
#39133=CARTESIAN_POINT('Ctrl Pts',(4.70501797698753,-1.9565538528228,32.0386420892521));
#39134=CARTESIAN_POINT('Ctrl Pts',(5.06775518859854,0.532122627976042,32.1180139793055));
#39135=CARTESIAN_POINT('Ctrl Pts',(4.19599845355282,2.89117521443338,32.1973858693589));
#39136=CARTESIAN_POINT('Ctrl Pts',(2.30210578290666,4.54594391816259,32.2767577594124));
#39137=CARTESIAN_POINT('Ctrl Pts',(-0.152574760830862,5.09333074570355,
32.3561296494657));
#39138=CARTESIAN_POINT('Ctrl Pts',(-2.57008843054848,4.39999347748749,32.4355015395192));
#39139=CARTESIAN_POINT('Ctrl Pts',(-4.3615342473787,2.63482753737587,32.5148734295725));
#39140=CARTESIAN_POINT('Ctrl Pts',(-5.09051997563981,0.227823441251348,
32.594245319626));
#39141=CARTESIAN_POINT('Ctrl Pts',(-4.57946630550992,-2.23467794088343,
32.6736172096794));
#39142=CARTESIAN_POINT('Ctrl Pts',(-2.95286477983452,-4.1528167229947,32.7529890997328));
#39143=CARTESIAN_POINT('Ctrl Pts',(-0.60695192984675,-5.05933854348835,
32.8323609897862));
#39144=CARTESIAN_POINT('Ctrl Pts',(1.88681306678638,-4.73341669344416,32.9117328798396));
#39145=CARTESIAN_POINT('Ctrl Pts',(3.92095457674023,-3.25444501411708,32.991104769893));
#39146=CARTESIAN_POINT('Ctrl Pts',(4.99996023068588,-0.982697732942914,
33.0704766599464));
#39147=CARTESIAN_POINT('Ctrl Pts',(4.8609866396607,1.52843254081155,33.1498485499997));
#39148=CARTESIAN_POINT('Ctrl Pts',(3.53788746282564,3.66724003075238,33.2292204400532));
#39149=CARTESIAN_POINT('Ctrl Pts',(1.35296673102733,4.91271596650007,33.3085923301066));
#39150=CARTESIAN_POINT('Ctrl Pts',(-1.16153370170815,4.96146516692072,33.38796422016));
#39151=CARTESIAN_POINT('Ctrl Pts',(-3.39308709571883,3.80161243469636,33.4673361102134));
#39152=CARTESIAN_POINT('Ctrl Pts',(-4.79809198368328,1.71569532810634,33.5467080002668));
#39153=CARTESIAN_POINT('Ctrl Pts',(-5.03429228481892,-0.788161362783202,
33.6260798903202));
#39154=CARTESIAN_POINT('Ctrl Pts',(-4.04415012858963,-3.10002369026433,
33.7054517803737));
#39155=CARTESIAN_POINT('Ctrl Pts',(-2.06886195261037,-4.65672710858312,
33.784823670427));
#39156=CARTESIAN_POINT('Ctrl Pts',(0.41039641567654,-5.07906211074165,33.8641955604805));
#39157=CARTESIAN_POINT('Ctrl Pts',(2.78968312550164,-4.26414882503682,33.9435674505338));
#39158=CARTESIAN_POINT('Ctrl Pts',(4.48940920081343,-2.41049832408638,34.0229393405872));
#39159=CARTESIAN_POINT('Ctrl Pts',(5.09552513194581,0.0303442330639926,
34.1023112306406));
#39160=CARTESIAN_POINT('Ctrl Pts',(4.46038241968974,2.46379500220581,34.181683120694));
#39161=CARTESIAN_POINT('Ctrl Pts',(2.73870042288625,4.29707076232801,34.2610550107475));
#39162=CARTESIAN_POINT('Ctrl Pts',(0.349877065078239,5.0835895961519,34.3404269008008));
#39163=CARTESIAN_POINT('Ctrl Pts',(-2.1241755713431,4.63175725668789,34.4197987908543));
#39164=CARTESIAN_POINT('Ctrl Pts',(-4.08078374036812,3.05163910171546,34.4991706809076));
#39165=CARTESIAN_POINT('Ctrl Pts',(-5.04332202290104,0.728148416253786,
34.5785425709611));
#39166=CARTESIAN_POINT('Ctrl Pts',(-4.77731822385925,-1.77271761167814,
34.6579144610144));
#39167=CARTESIAN_POINT('Ctrl Pts',(-3.3475702798999,-3.84175355324914,34.7372863510679));
#39168=CARTESIAN_POINT('Ctrl Pts',(-1.10236162547809,-4.97494683282594,
34.8166582411212));
#39169=CARTESIAN_POINT('Ctrl Pts',(1.41137988087415,-4.8962540757844,34.8960301311747));
#39170=CARTESIAN_POINT('Ctrl Pts',(3.58131237228184,-3.62484466355631,34.9754020212281));
#39171=CARTESIAN_POINT('Ctrl Pts',(4.87884509690211,-1.47043111474347,35.0547739112815));
#39172=CARTESIAN_POINT('Ctrl Pts',(4.98790195505749,1.04217619887681,35.1341458013349));
#39173=CARTESIAN_POINT('Ctrl Pts',(3.88191693749454,3.3009116972686,35.2135176913883));
#39174=CARTESIAN_POINT('Ctrl Pts',(1.8303055464353,4.75555241264984,35.2928895814417));
#39175=CARTESIAN_POINT('Ctrl Pts',(-0.667164224422912,5.05175108654629,
35.3722614714951));
#39176=CARTESIAN_POINT('Ctrl Pts',(-3.00211426695468,4.11735437762148,35.4516333615485));
#39177=CARTESIAN_POINT('Ctrl Pts',(-4.60575591912355,2.17997925591738,35.5310052516019));
#39178=CARTESIAN_POINT('Ctrl Pts',(-5.08744562406171,-0.288433987225976,
35.6103771416553));
#39179=CARTESIAN_POINT('Ctrl Pts',(-4.32984483584829,-2.68658534951887,
35.6897490317088));
#39180=CARTESIAN_POINT('Ctrl Pts',(-2.51750342957125,-4.43029046732475,
35.7691209217621));
#39181=CARTESIAN_POINT('Ctrl Pts',(-0.0919037602499935,-5.09478663357195,
35.8484928118156));
#39182=CARTESIAN_POINT('Ctrl Pts',(2.35608346164268,-4.51820405299999,35.9278647018689));
#39183=CARTESIAN_POINT('Ctrl Pts',(4.23013396738149,-2.84099696599223,36.0072365919223));
#39184=CARTESIAN_POINT('Ctrl Pts',(5.07373320190884,-0.471729306508876,
36.0866084819757));
#39185=CARTESIAN_POINT('Ctrl Pts',(4.68138225896918,2.01245056788487,36.1659803720291));
#39186=CARTESIAN_POINT('Ctrl Pts',(3.14865695980852,4.00640193842567,36.2453522620825));
#39187=CARTESIAN_POINT('Ctrl Pts',(0.84892579467244,5.02440266478627,36.3247241521359));
#39188=CARTESIAN_POINT('Ctrl Pts',(-1.65760181498048,4.81847002333159,36.4040960421893));
#39189=CARTESIAN_POINT('Ctrl Pts',(-3.76034129154353,3.43876874969578,36.4834679322427));
#39190=CARTESIAN_POINT('Ctrl Pts',(-4.94706995286084,1.22139102021962,36.5628398222961));
#39191=CARTESIAN_POINT('Ctrl Pts',(-4.92870332381484,-1.2935148582789,36.6422117123495));
#39192=CARTESIAN_POINT('Ctrl Pts',(-3.70971547458727,-3.49332338044723,
36.721583602403));
#39193=CARTESIAN_POINT('Ctrl Pts',(-1.58704914706622,-4.84216605947875,
36.8009554924563));
#39194=CARTESIAN_POINT('Ctrl Pts',(0.922218839806455,-5.01146780437405,
36.8803273825098));
#39195=CARTESIAN_POINT('Ctrl Pts',(3.20683635859905,-3.95998708481968,36.9596992725631));
#39196=CARTESIAN_POINT('Ctrl Pts',(4.71027563864883,-1.94386227668601,37.0390711626166));
#39197=CARTESIAN_POINT('Ctrl Pts',(5.06630219914206,0.545783079382256,37.1184430526699));
#39198=CARTESIAN_POINT('Ctrl Pts',(4.18818875799396,2.90247688538333,37.1978149427234));
#39199=CARTESIAN_POINT('Ctrl Pts',(2.28984180579711,4.55213374662869,37.2771868327768));
#39200=CARTESIAN_POINT('Ctrl Pts',(-0.1663055418131,5.0929009031723,37.3565587228302));
#39201=CARTESIAN_POINT('Ctrl Pts',(-2.58194122754862,4.39304867264833,37.4359306128836));
#39202=CARTESIAN_POINT('Ctrl Pts',(-4.36862174528344,2.62305950931498,37.515302502937));
#39203=CARTESIAN_POINT('Ctrl Pts',(-5.09111567564704,0.214098855557291,
37.5946743929904));
#39204=CARTESIAN_POINT('Ctrl Pts',(-4.57342509641719,-2.24701580551625,
37.6740462830439));
#39205=CARTESIAN_POINT('Ctrl Pts',(-2.94165828680345,-4.16076239004767,
37.7534181730971));
#39206=CARTESIAN_POINT('Ctrl Pts',(-0.593310029777194,-5.06095646606148,
37.8327900631507));
#39207=CARTESIAN_POINT('Ctrl Pts',(1.89956723723832,-4.72831274916718,37.912161953204));
#39208=CARTESIAN_POINT('Ctrl Pts',(3.92971412987383,-3.2438625125424,37.9915338432574));
#39209=CARTESIAN_POINT('Ctrl Pts',(5.00259135876467,-0.969214547985126,
38.0709057333108));
#39210=CARTESIAN_POINT('Ctrl Pts',(4.85684840567486,1.54153193505625,38.1502776233642));
#39211=CARTESIAN_POINT('Ctrl Pts',(3.52798793147795,3.67676465100168,38.2296495134176));
#39212=CARTESIAN_POINT('Ctrl Pts',(1.3397174061215,4.91634563604017,38.309021403471));
#39213=CARTESIAN_POINT('Ctrl Pts',(-1.17490531372475,4.95831570685867,38.3883932935245));
#39214=CARTESIAN_POINT('Ctrl Pts',(-3.40332370018554,3.79245104545026,38.4677651835778));
#39215=CARTESIAN_POINT('Ctrl Pts',(-4.80269996560014,1.70275370586069,38.5471370736313));
#39216=CARTESIAN_POINT('Ctrl Pts',(-5.03214915152033,-0.801730671351773,
38.6265089636846));
#39217=CARTESIAN_POINT('Ctrl Pts',(-4.03577793971505,-3.11091522434137,
38.705880853738));
#39218=CARTESIAN_POINT('Ctrl Pts',(-2.05630016029208,-4.6622877283261,38.7852527437914));
#39219=CARTESIAN_POINT('Ctrl Pts',(0.424087796933226,-5.0779372355256,38.8646246338449));
#39220=CARTESIAN_POINT('Ctrl Pts',(2.80116888608276,-4.2566125209993,38.9439965238982));
#39221=CARTESIAN_POINT('Ctrl Pts',(4.49589147158116,-2.39838632564053,39.0233684139517));
#39222=CARTESIAN_POINT('Ctrl Pts',(5.09542477676094,0.0440812951169324,
39.1027403040051));
#39223=CARTESIAN_POINT('Ctrl Pts',(4.45372401575944,2.47581113999364,39.1821121940585));
#39224=CARTESIAN_POINT('Ctrl Pts',(2.72710569549243,4.30443824810521,39.2614840841118));
#39225=CARTESIAN_POINT('Ctrl Pts',(0.336170930870647,5.08451490337722,39.3408559741653));
#39226=CARTESIAN_POINT('Ctrl Pts',(-2.1366552096739,4.62601276074587,39.4202278642187));
#39227=CARTESIAN_POINT('Ctrl Pts',(-4.08899520654064,3.04062834435872,39.4995997542721));
#39228=CARTESIAN_POINT('Ctrl Pts',(-5.04526816392185,0.714545672092809,
39.5789716443255));
#39229=CARTESIAN_POINT('Ctrl Pts',(-4.77251903131803,-1.78558378675053,
39.6583435343789));
#39230=CARTESIAN_POINT('Ctrl Pts',(-3.33720602914116,-3.85077723115716,
39.7377154244323));
#39231=CARTESIAN_POINT('Ctrl Pts',(-1.08893586889047,-4.97787652885981,
39.8170873144857));
#39232=CARTESIAN_POINT('Ctrl Pts',(1.42455668503583,-4.8924768895782,39.8964592045391));
#39233=CARTESIAN_POINT('Ctrl Pts',(3.59110607910284,-3.61508997874913,39.9758310945925));
#39234=CARTESIAN_POINT('Ctrl Pts',(4.88272528059762,-1.45743906270703,40.0552029846459));
#39235=CARTESIAN_POINT('Ctrl Pts',(4.98521092249161,1.05595859527154,40.1345748746994));
#39236=CARTESIAN_POINT('Ctrl Pts',(4.2435173595031,2.5590120913109,40.1874894680683));
#39237=CARTESIAN_POINT('Ctrl Pts',(3.71544298812202,3.17665283523806,40.2139467647527));
#39238=CARTESIAN_POINT('Ctrl Pts',(1.21713437249832,-4.5428082122986,-0.213946764752702));
#39239=CARTESIAN_POINT('Ctrl Pts',(1.97231308274437,-4.34047654372165,-0.187489468068234));
#39240=CARTESIAN_POINT('Ctrl Pts',(3.37906911267772,-3.55219315325666,-0.134574874699299));
#39241=CARTESIAN_POINT('Ctrl Pts',(4.66642692152752,-1.5028536385038,-0.055202984645895));
#39242=CARTESIAN_POINT('Ctrl Pts',(4.81689062664967,0.911851793295018,0.0241689054075086));
#39243=CARTESIAN_POINT('Ctrl Pts',(3.79405383067521,3.10479958283122,0.103540795460912));
#39244=CARTESIAN_POINT('Ctrl Pts',(1.84695009786499,4.54123256689918,0.182912685514316));
#39245=CARTESIAN_POINT('Ctrl Pts',(-0.550043424514128,4.8715330414348,0.26228457556772));
#39246=CARTESIAN_POINT('Ctrl Pts',(-2.81305984991034,4.01508502497055,0.341656465621123));
#39247=CARTESIAN_POINT('Ctrl Pts',(-4.39081462818011,2.18059968579164,0.421028355674527));
#39248=CARTESIAN_POINT('Ctrl Pts',(-4.89898012125377,-0.18509000454136,
0.500400245727931));
#39249=CARTESIAN_POINT('Ctrl Pts',(-4.21376307902768,-2.5056841854766,0.579772135781334));
#39250=CARTESIAN_POINT('Ctrl Pts',(-2.50208364241389,-4.21590347870479,
0.659144025834738));
#39251=CARTESIAN_POINT('Ctrl Pts',(-0.180901657890204,-4.89913577411436,
0.738515915888141));
#39252=CARTESIAN_POINT('Ctrl Pts',(2.18434729950923,-4.38895062645432,0.817887805941546));
#39253=CARTESIAN_POINT('Ctrl Pts',(4.01749423301245,-2.8096261920884,0.897259695994948));
#39254=CARTESIAN_POINT('Ctrl Pts',(4.87198838803769,-0.545883369388664,
0.976631586048353));
#39255=CARTESIAN_POINT('Ctrl Pts',(4.53967699589134,1.85083561019003,1.05600347610176));
#39256=CARTESIAN_POINT('Ctrl Pts',(3.10151031466513,3.79669503846566,1.13537536615516));
#39257=CARTESIAN_POINT('Ctrl Pts',(0.907822597135906,4.81768800868641,1.21474725620856));
#39258=CARTESIAN_POINT('Ctrl Pts',(-1.50700870159448,4.66510281756135,1.29411914626197));
#39259=CARTESIAN_POINT('Ctrl Pts',(-3.55473601316185,3.37610891998462,1.37349103631537));
#39260=CARTESIAN_POINT('Ctrl Pts',(-4.73653750187219,1.26470235504102,1.45286292636877));
#39261=CARTESIAN_POINT('Ctrl Pts',(-4.76452893838759,-1.15478290032736,
1.53223481642218));
#39262=CARTESIAN_POINT('Ctrl Pts',(-3.63189167208734,-3.29296559930584,
1.61160670647558));
#39263=CARTESIAN_POINT('Ctrl Pts',(-1.61453363327375,-4.62898916605748,
1.69097859652899));
#39264=CARTESIAN_POINT('Ctrl Pts',(0.796121224764031,-4.8374012186294,1.77035048658239));
#39265=CARTESIAN_POINT('Ctrl Pts',(3.01284271470348,-3.86743304144296,1.8497223766358));
#39266=CARTESIAN_POINT('Ctrl Pts',(4.49564238811846,-1.95536673594104,1.92909426668919));
#39267=CARTESIAN_POINT('Ctrl Pts',(4.88331352674298,0.433022578391154,2.0084661567426));
#39268=CARTESIAN_POINT('Ctrl Pts',(4.08142029927371,2.71592855106099,2.087838046796));
#39269=CARTESIAN_POINT('Ctrl Pts',(2.28530212097744,4.33724034032234,2.16720993684941));
#39270=CARTESIAN_POINT('Ctrl Pts',(-0.067510595561391,4.90200998298708,
2.24658182690281));
#39271=CARTESIAN_POINT('Ctrl Pts',(-2.4038778804521,4.27266084421796,2.32595371695622));
#39272=CARTESIAN_POINT('Ctrl Pts',(-4.15466583455893,2.60250098116813,2.40532560700962));
#39273=CARTESIAN_POINT('Ctrl Pts',(-4.8933863875636,0.298377639645852,2.48469749706302));
#39274=CARTESIAN_POINT('Ctrl Pts',(-4.44008884788507,-2.07842983444745,
2.56406938711643));
#39275=CARTESIAN_POINT('Ctrl Pts',(-2.90519549283157,-3.94893640139523,
2.64344127716983));
#39276=CARTESIAN_POINT('Ctrl Pts',(-0.662602946265526,-4.85749080178588,
2.72281316722323));
#39277=CARTESIAN_POINT('Ctrl Pts',(1.7413982113641,-4.58277119473486,2.80218505727664));
#39278=CARTESIAN_POINT('Ctrl Pts',(3.72119861922498,-3.19169866843848,2.88155694733003));
#39279=CARTESIAN_POINT('Ctrl Pts',(4.79452328017608,-1.02313541121562,2.96092883738345));
#39280=CARTESIAN_POINT('Ctrl Pts',(4.69991268257356,1.39466136750753,3.04030072743684));
#39281=CARTESIAN_POINT('Ctrl Pts',(3.46041375857639,3.47272172413642,3.11967261749026));
#39282=CARTESIAN_POINT('Ctrl Pts',(1.37796570248595,4.70483475550482,3.19904450754365));
#39283=CARTESIAN_POINT('Ctrl Pts',(-1.04015174865471,4.79086045440737,3.27841639759706));
#39284=CARTESIAN_POINT('Ctrl Pts',(-3.20489053615995,3.70984315100601,3.35778828765046));
#39285=CARTESIAN_POINT('Ctrl Pts',(-4.5889250829615,1.72511626761812,3.43716017770387));
#39286=CARTESIAN_POINT('Ctrl Pts',(-4.85510763696699,-0.679845120081458,
3.51653206775727));
#39287=CARTESIAN_POINT('Ctrl Pts',(-3.9385967172058,-2.91919774134084,3.59590395781068));
#39288=CARTESIAN_POINT('Ctrl Pts',(-2.06265235506924,-4.44744025434419,
3.67527584786408));
#39289=CARTESIAN_POINT('Ctrl Pts',(0.315749555158651,-4.89229616563132,
3.75464773791748));
#39290=CARTESIAN_POINT('Ctrl Pts',(2.61723557264967,-4.14539955988454,3.83401962797088));
#39291=CARTESIAN_POINT('Ctrl Pts',(4.2811687977959,-2.38869279703619,3.91339151802429));
#39292=CARTESIAN_POINT('Ctrl Pts',(4.90221878000547,-0.0501057561116431,
3.99276340807769));
#39293=CARTESIAN_POINT('Ctrl Pts',(4.32909911828292,2.3006869360945,4.0721352981311));
#39294=CARTESIAN_POINT('Ctrl Pts',(2.701420493645,4.09103738315217,4.1515071881845));
#39295=CARTESIAN_POINT('Ctrl Pts',(0.415681816248014,4.88482017903163,4.2308790782379));
#39296=CARTESIAN_POINT('Ctrl Pts',(-1.97131603149091,4.48867159166503,4.31025096829131));
#39297=CARTESIAN_POINT('Ctrl Pts',(-3.87810565739265,2.9990925400749,4.38962285834471));
#39298=CARTESIAN_POINT('Ctrl Pts',(-4.84019732919483,0.778941184101248,
4.46899474839812));
#39299=CARTESIAN_POINT('Ctrl Pts',(-4.62322764520021,-1.63095852016239,
4.54836663845152));
#39300=CARTESIAN_POINT('Ctrl Pts',(-3.28004994017564,-3.64356033897994,
4.62773852850492));
#39301=CARTESIAN_POINT('Ctrl Pts',(-1.13785932999167,-4.76859892410598,
4.70711041855833));
#39302=CARTESIAN_POINT('Ctrl Pts',(1.28151129436936,-4.73201736643448,4.78648230861172));
#39303=CARTESIAN_POINT('Ctrl Pts',(3.38870860399915,-3.54272685244233,4.86585419866514));
#39304=CARTESIAN_POINT('Ctrl Pts',(4.67042399847401,-1.4904359188881,4.94522608871853));
#39305=CARTESIAN_POINT('Ctrl Pts',(4.81443444472878,0.924921905483315,5.02459797877194));
#39306=CARTESIAN_POINT('Ctrl Pts',(3.78565931681752,3.1149708009589,5.10396986882535));
#39307=CARTESIAN_POINT('Ctrl Pts',(1.83470595874426,4.54621970419184,5.18334175887875));
#39308=CARTESIAN_POINT('Ctrl Pts',(-0.563177709826337,4.87001955037026,
5.26271364893215));
#39309=CARTESIAN_POINT('Ctrl Pts',(-2.82387253485596,4.00749341368393,5.34208553898556));
#39310=CARTESIAN_POINT('Ctrl Pts',(-4.39667826093048,2.1687507518604,5.42145742903895));
#39311=CARTESIAN_POINT('Ctrl Pts',(-4.89846289452463,-0.198294792667946,
5.50082931909237));
#39312=CARTESIAN_POINT('Ctrl Pts',(-4.20699280957627,-2.51703616462048,
5.58020120914576));
#39313=CARTESIAN_POINT('Ctrl Pts',(-2.49070858823577,-4.2226330982365,5.65957309919917));
#39314=CARTESIAN_POINT('Ctrl Pts',(-0.16769326789098,-4.89960595576194,
5.73894498925257));
#39315=CARTESIAN_POINT('Ctrl Pts',(2.19617176132931,-4.38304564755759,5.81831687930597));
#39316=CARTESIAN_POINT('Ctrl Pts',(4.0250542106335,-2.7987851213152,5.89768876935939));
#39317=CARTESIAN_POINT('Ctrl Pts',(4.87344236353376,-0.532746734526196,
5.97706065941277));
#39318=CARTESIAN_POINT('Ctrl Pts',(4.53467074385888,1.86306757757847,6.05643254946619));
#39319=CARTESIAN_POINT('Ctrl Pts',(3.09126336830344,3.80504275161517,6.13580443951959));
#39320=CARTESIAN_POINT('Ctrl Pts',(0.894831078624676,4.82011793367768,6.215176329573));
#39321=CARTESIAN_POINT('Ctrl Pts',(-1.51958008113206,4.6610230562464,6.2945482196264));
#39322=CARTESIAN_POINT('Ctrl Pts',(-3.56382489665849,3.36651327931302,6.3739201096798));
#39323=CARTESIAN_POINT('Ctrl Pts',(-4.73992985575151,1.25192831918974,6.45329199973321));
#39324=CARTESIAN_POINT('Ctrl Pts',(-4.76139839364024,-1.16762360839183,
6.53266388978661));
#39325=CARTESIAN_POINT('Ctrl Pts',(-3.62300082201479,-3.30274500946015,
6.61203577984002));
#39326=CARTESIAN_POINT('Ctrl Pts',(-1.60204826952283,-4.63332503672608,
6.69140766989341));
#39327=CARTESIAN_POINT('Ctrl Pts',(0.809159695351183,-4.83523734073654,
6.77077955994682));
#39328=CARTESIAN_POINT('Ctrl Pts',(3.02325814948227,-3.8592965311599,6.85015145000022));
#39329=CARTESIAN_POINT('Ctrl Pts',(4.50089761026788,-1.94323962900068,6.92952334005363));
#39330=CARTESIAN_POINT('Ctrl Pts',(4.8821283757601,0.446186145495144,7.00889523010703));
#39331=CARTESIAN_POINT('Ctrl Pts',(4.07408347532503,2.72692196256463,7.08826712016044));
#39332=CARTESIAN_POINT('Ctrl Pts',(2.27360085813158,4.34338562549276,7.16763901021384));
#39333=CARTESIAN_POINT('Ctrl Pts',(-0.0807258955725768,4.90181016397186,
7.24701090026724));
#39334=CARTESIAN_POINT('Ctrl Pts',(-2.41538799979899,4.26616459648018,7.32638279032065));
#39335=CARTESIAN_POINT('Ctrl Pts',(-4.16166693364502,2.59129077628108,7.40575468037405));
#39336=CARTESIAN_POINT('Ctrl Pts',(-4.89417301414864,0.285184258704783,
7.48512657042745));
#39337=CARTESIAN_POINT('Ctrl Pts',(-4.43446938147388,-2.09039251304738,
7.56449846048085));
#39338=CARTESIAN_POINT('Ctrl Pts',(-2.89453882300355,-3.95675429562653,
7.64387035053426));
#39339=CARTESIAN_POINT('Ctrl Pts',(-0.649505014202585,-4.85925948991814,
7.72324224058766));
#39340=CARTESIAN_POINT('Ctrl Pts',(1.75374677840318,-4.57805982825413,7.80261413064107));
#39341=CARTESIAN_POINT('Ctrl Pts',(3.72978973764259,-3.18165492579096,7.88198602069447));
#39342=CARTESIAN_POINT('Ctrl Pts',(4.79726417254181,-1.01020592587881,7.96135791074788));
#39343=CARTESIAN_POINT('Ctrl Pts',(4.69613567357394,1.40732700152449,8.04072980080128));
#39344=CARTESIAN_POINT('Ctrl Pts',(3.45103891924351,3.48203818642192,8.12010169085468));
#39345=CARTESIAN_POINT('Ctrl Pts',(1.36527672293039,4.70853257646778,8.19947358090808));
#39346=CARTESIAN_POINT('Ctrl Pts',(-1.05306386109979,4.78803885304614,8.2788454709615));
#39347=CARTESIAN_POINT('Ctrl Pts',(-3.21488041948337,3.7011894631667,8.35821736101489));
#39348=CARTESIAN_POINT('Ctrl Pts',(-4.5935592236979,1.7127385125038,8.4375892510683));
#39349=CARTESIAN_POINT('Ctrl Pts',(-4.85325716869052,-0.692931748722623,
8.51696114112171));
#39350=CARTESIAN_POINT('Ctrl Pts',(-3.93071240989269,-2.92980536973865,
8.59633303117509));
#39351=CARTESIAN_POINT('Ctrl Pts',(-2.05065480852931,-4.45298488770055,
8.67570492122852));
#39352=CARTESIAN_POINT('Ctrl Pts',(0.328937765144378,-4.89142714353344,
8.7550768112819));
#39353=CARTESIAN_POINT('Ctrl Pts',(2.62840182732027,-4.1383285741919,8.83444870133532));
#39354=CARTESIAN_POINT('Ctrl Pts',(4.28759302222971,-2.37714232421218,8.91382059138872));
#39355=CARTESIAN_POINT('Ctrl Pts',(4.90233604735019,-0.0368894657696129,
8.99319248144213));
#39356=CARTESIAN_POINT('Ctrl Pts',(4.32288086247292,2.31234958488097,9.07256437149553));
#39357=CARTESIAN_POINT('Ctrl Pts',(2.69038146803174,4.09830539495352,9.15193626154892));
#39358=CARTESIAN_POINT('Ctrl Pts',(0.402511103036409,4.88592308226053,9.23130815160233));
#39359=CARTESIAN_POINT('Ctrl Pts',(-1.9834100757154,4.48334072153617,9.31068004165575));
#39360=CARTESIAN_POINT('Ctrl Pts',(-3.88617695022667,2.98862648475194,9.39005193170914));
#39361=CARTESIAN_POINT('Ctrl Pts',(-4.84227972156947,0.765889451494674,
9.46942382176256));
#39362=CARTESIAN_POINT('Ctrl Pts',(-4.61881387094234,-1.64341655687914,
9.54879571181594));
#39363=CARTESIAN_POINT('Ctrl Pts',(-3.27021518492473,-3.65238992963806,
9.62816760186936));
#39364=CARTESIAN_POINT('Ctrl Pts',(-1.124999318358,-4.77164919996512,9.70753949192275));
#39365=CARTESIAN_POINT('Ctrl Pts',(1.29426389201697,-4.72854528704705,9.78691138197616));
#39366=CARTESIAN_POINT('Ctrl Pts',(3.39824728310117,-3.53357820866179,9.86628327202957));
#39367=CARTESIAN_POINT('Ctrl Pts',(4.67442515791466,-1.4778393000892,9.94565516208296));
#39368=CARTESIAN_POINT('Ctrl Pts',(4.81192341092478,0.937897990843289,10.0250270521364));
#39369=CARTESIAN_POINT('Ctrl Pts',(3.7772477720454,3.12516540720838,10.1043989421898));
#39370=CARTESIAN_POINT('Ctrl Pts',(1.82244293669188,4.55114944781378,10.1837708322432));
#39371=CARTESIAN_POINT('Ctrl Pts',(-0.576304964130747,4.86848355673017,
10.2631427222966));
#39372=CARTESIAN_POINT('Ctrl Pts',(-2.83466625132052,3.99986584743267,10.34251461235));
#39373=CARTESIAN_POINT('Ctrl Pts',(-4.40250911411597,2.15688967125344,10.4218865024034));
#39374=CARTESIAN_POINT('Ctrl Pts',(-4.89791050150136,-0.211500054648842,
10.5012583924568));
#39375=CARTESIAN_POINT('Ctrl Pts',(-4.20019173206204,-2.52836883538606,
10.5806302825102));
#39376=CARTESIAN_POINT('Ctrl Pts',(-2.47931555365911,-4.22933256427274,
10.6600021725636));
#39377=CARTESIAN_POINT('Ctrl Pts',(-0.154483594256702,-4.90004024197143,
10.739374062617));
#39378=CARTESIAN_POINT('Ctrl Pts',(2.20798022676301,-4.37710896278096,10.8187459526704));
#39379=CARTESIAN_POINT('Ctrl Pts',(4.03258495182456,-2.7879236288234,10.8981178427238));
#39380=CARTESIAN_POINT('Ctrl Pts',(4.87486090859705,-0.519606269848766,
10.9774897327772));
#39381=CARTESIAN_POINT('Ctrl Pts',(4.52963153835691,1.87528602633207,11.0568616228306));
#39382=CARTESIAN_POINT('Ctrl Pts',(3.08099395154235,3.81336279737362,11.136233512884));
#39383=CARTESIAN_POINT('Ctrl Pts',(0.881833057796546,4.82251283171035,11.2156054029374));
#39384=CARTESIAN_POINT('Ctrl Pts',(-1.53214041692415,4.65690941469354,11.2949772929908));
#39385=CARTESIAN_POINT('Ctrl Pts',(-3.5728878774174,3.35689317215153,11.3743491830443));
#39386=CARTESIAN_POINT('Ctrl Pts',(-4.74328775942496,1.23914518323042,11.4537210730976));
#39387=CARTESIAN_POINT('Ctrl Pts',(-4.75823324232597,-1.1804558295243,11.533092963151));
#39388=CARTESIAN_POINT('Ctrl Pts',(-3.614083639567,-3.31250041510156,11.6124648532044));
#39389=CARTESIAN_POINT('Ctrl Pts',(-1.58955126184795,-4.63762723165536,
11.6918367432579));
#39390=CARTESIAN_POINT('Ctrl Pts',(0.822192284845203,-4.83303831979168,
11.7712086333112));
#39391=CARTESIAN_POINT('Ctrl Pts',(3.03365161084184,-3.85113197097562,11.8505805233647));
#39392=CARTESIAN_POINT('Ctrl Pts',(4.50612011931135,-1.9310983983659,11.9299524134181));
#39393=CARTESIAN_POINT('Ctrl Pts',(4.88090774084429,0.459346469671929,12.0093243034715));
#39394=CARTESIAN_POINT('Ctrl Pts',(4.06671704041361,2.73789555444384,12.0886961935249));
#39395=CARTESIAN_POINT('Ctrl Pts',(2.26188307046365,4.34949934238227,12.1680680835783));
#39396=CARTESIAN_POINT('Ctrl Pts',(-0.0939406088580155,4.90157471796985,
12.2474399736317));
#39397=CARTESIAN_POINT('Ctrl Pts',(-2.42688056379585,4.25963734171157,12.3268118636851));
#39398=CARTESIAN_POINT('Ctrl Pts',(-4.16863778520202,2.58006173755973,12.4061837537385));
#39399=CARTESIAN_POINT('Ctrl Pts',(-4.89492406925624,0.271988805008134,
12.4855556437919));
#39400=CARTESIAN_POINT('Ctrl Pts',(-4.4288176847703,-2.10233999840645,12.5649275338453));
#39401=CARTESIAN_POINT('Ctrl Pts',(-2.88386111529598,-3.96454343165991,
12.6442994238987));
#39402=CARTESIAN_POINT('Ctrl Pts',(-0.636402361453836,-4.86099286032903,
12.7236713139521));
#39403=CARTESIAN_POINT('Ctrl Pts',(1.76608259898569,-4.57331518784718,12.8030432040055));
#39404=CARTESIAN_POINT('Ctrl Pts',(3.73835374746984,-3.17158805846724,12.8824150940589));
#39405=CARTESIAN_POINT('Ctrl Pts',(4.79997019777602,-0.997269098235751,
12.9617869841123));
#39406=CARTESIAN_POINT('Ctrl Pts',(4.69232453245774,1.41998240690827,13.0411588741657));
#39407=CARTESIAN_POINT('Ctrl Pts',(3.44163899731696,3.49132934080715,13.1205307642191));
#39408=CARTESIAN_POINT('Ctrl Pts',(1.35257782036847,4.71219617521183,13.1999026542725));
#39409=CARTESIAN_POINT('Ctrl Pts',(-1.06596831974157,4.78518245160425,13.2792745443259));
#39410=CARTESIAN_POINT('Ctrl Pts',(-3.22484693664342,3.69250887460753,13.3586464343793));
#39411=CARTESIAN_POINT('Ctrl Pts',(-4.59815997785652,1.70034830898619,13.4380183244327));
#39412=CARTESIAN_POINT('Ctrl Pts',(-4.85137142631828,-0.706013341047003,
13.5173902144861));
#39413=CARTESIAN_POINT('Ctrl Pts',(-3.92279953365742,-2.94039170393519,
13.5967621045396));
#39414=CARTESIAN_POINT('Ctrl Pts',(-2.03864235756713,-4.45849715619141,
13.6761339945929));
#39415=CARTESIAN_POINT('Ctrl Pts',(0.342123584368241,-4.8905225699155,13.7555058846463));
#39416=CARTESIAN_POINT('Ctrl Pts',(2.63954897842921,-4.13122751059623,13.8348777746997));
#39417=CARTESIAN_POINT('Ctrl Pts',(4.29398608388735,-2.36557457401273,13.9142496647532));
#39418=CARTESIAN_POINT('Ctrl Pts',(4.90241768388754,-0.0236729073102294,
13.9936215548065));
#39419=CARTESIAN_POINT('Ctrl Pts',(4.31663118741021,2.32399542721397,14.07299344486));
#39420=CARTESIAN_POINT('Ctrl Pts',(2.67932288838078,4.10554361974547,14.1523653349134));
#39421=CARTESIAN_POINT('Ctrl Pts',(0.389337464322444,4.8869904739736,14.2317372249668));
#39422=CARTESIAN_POINT('Ctrl Pts',(-1.99548970426098,4.47797726591172,14.3111091150202));
#39423=CARTESIAN_POINT('Ctrl Pts',(-3.894219997828,2.97813870770829,14.3904810050736));
#39424=CARTESIAN_POINT('Ctrl Pts',(-4.84432691963384,0.752832152305313,
14.469852895127));
#39425=CARTESIAN_POINT('Ctrl Pts',(-4.61436652655265,-1.6558626490335,14.5492247851804));
#39426=CARTESIAN_POINT('Ctrl Pts',(-3.26035666133029,-3.66119297425757,
14.6285966752338));
#39427=CARTESIAN_POINT('Ctrl Pts',(-1.11213113008494,-4.77466479486569,
14.7079685652872));
#39428=CARTESIAN_POINT('Ctrl Pts',(1.30700708278859,-4.72503883998578,14.7873404553406));
#39429=CARTESIAN_POINT('Ctrl Pts',(3.40776126330594,-3.52440388238144,14.866712345394));
#39430=CARTESIAN_POINT('Ctrl Pts',(4.67839234303357,-1.46523194016464,14.9460842354474));
#39431=CARTESIAN_POINT('Ctrl Pts',(4.80937740344404,0.95086725944037,15.0254561255008));
#39432=CARTESIAN_POINT('Ctrl Pts',(3.76880877375186,3.13533729935469,15.1048280155542));
#39433=CARTESIAN_POINT('Ctrl Pts',(1.81016666889045,4.55604611309762,15.1841999056076));
#39434=CARTESIAN_POINT('Ctrl Pts',(-0.58942802977675,4.86691217832697,15.263571795661));
#39435=CARTESIAN_POINT('Ctrl Pts',(-2.84543936506709,3.99220920964323,15.3429436857144));
#39436=CARTESIAN_POINT('Ctrl Pts',(-4.40830796930035,2.14501291409566,15.4223155757678));
#39437=CARTESIAN_POINT('Ctrl Pts',(-4.89732250983615,-0.224703779420184,
15.5016874658212));
#39438=CARTESIAN_POINT('Ctrl Pts',(-4.19336012701549,-2.53968312964247,
15.5810593558746));
#39439=CARTESIAN_POINT('Ctrl Pts',(-2.46790449909881,-4.23600129097741,
15.6604312459281));
#39440=CARTESIAN_POINT('Ctrl Pts',(-0.141272797816101,-4.90043891405947,
15.7398031359814));
#39441=CARTESIAN_POINT('Ctrl Pts',(2.21977264431347,-4.37114046461536,15.8191750260349));
#39442=CARTESIAN_POINT('Ctrl Pts',(4.04008638367001,-2.77704187334405,15.8985469160882));
#39443=CARTESIAN_POINT('Ctrl Pts',(4.87624402254724,-0.50646202860824,15.9779188061417));
#39444=CARTESIAN_POINT('Ctrl Pts',(4.52455941090906,1.88749084526974,16.057290696195));
#39445=CARTESIAN_POINT('Ctrl Pts',(3.0707021417271,3.82165512711525,16.1366625862485));
#39446=CARTESIAN_POINT('Ctrl Pts',(0.868828627683026,4.82487267911372,16.2160344763019));
#39447=CARTESIAN_POINT('Ctrl Pts',(-1.54468961690488,4.65276192610161,16.2954063663553));
#39448=CARTESIAN_POINT('Ctrl Pts',(-3.58192489000319,3.34724866670505,16.3747782564087));
#39449=CARTESIAN_POINT('Ctrl Pts',(-4.74661118820951,1.22635304091943,16.4541501464621));
#39450=CARTESIAN_POINT('Ctrl Pts',(-4.75503350768456,-1.19327947079094,
16.5335220365155));
#39451=CARTESIAN_POINT('Ctrl Pts',(-3.60514018926425,-3.32223174536968,
16.6128939265689));
#39452=CARTESIAN_POINT('Ctrl Pts',(-1.57704270154751,-4.64189571913949,
16.6922658166223));
#39453=CARTESIAN_POINT('Ctrl Pts',(0.835218899365215,-4.83080417279076,
16.7716377066757));
#39454=CARTESIAN_POINT('Ctrl Pts',(3.04402302167444,-3.84293941821851,16.8510095967291));
#39455=CARTESIAN_POINT('Ctrl Pts',(4.5113098802371,-1.91894313613405,16.9303814867825));
#39456=CARTESIAN_POINT('Ctrl Pts',(4.87965162531072,0.47250346257415,17.0097533768359));
#39457=CARTESIAN_POINT('Ctrl Pts',(4.05932105856824,2.74884923313555,17.0891252668893));
#39458=CARTESIAN_POINT('Ctrl Pts',(2.25014882333735,4.35558147263106,17.1684971569427));
#39459=CARTESIAN_POINT('Ctrl Pts',(-0.107154601980602,4.90130359745223,
17.2478690469961));
#39460=CARTESIAN_POINT('Ctrl Pts',(-2.43835555951383,4.25307922033065,17.3272409370495));
#39461=CARTESIAN_POINT('Ctrl Pts',(-4.17557820525659,2.56881377105676,17.4066128271029));
#39462=CARTESIAN_POINT('Ctrl Pts',(-4.8956397991406,0.258791705958601,17.4859847171563));
#39463=CARTESIAN_POINT('Ctrl Pts',(-4.42313332356637,-2.11427282962181,
17.5653566072097));
#39464=CARTESIAN_POINT('Ctrl Pts',(-2.8731633447509,-3.97230257099397,17.6447284972631));
#39465=CARTESIAN_POINT('Ctrl Pts',(-0.623293388711154,-4.8626931320669,
17.7241003873165));
#39466=CARTESIAN_POINT('Ctrl Pts',(1.77840238381723,-4.56853309419578,17.8034722773699));
#39467=CARTESIAN_POINT('Ctrl Pts',(3.74689662802603,-3.1615060961514,17.8828441674233));
#39468=CARTESIAN_POINT('Ctrl Pts',(4.80262992851038,-0.984309998791364,
17.9622160574768));
#39469=CARTESIAN_POINT('Ctrl Pts',(4.6885008269824,1.43259912421597,18.0415879475301));
#39470=CARTESIAN_POINT('Ctrl Pts',(3.43217338911689,3.50064868327997,18.1209598375836));
#39471=CARTESIAN_POINT('Ctrl Pts',(1.33994588402617,4.71572438645645,18.2003317276369));
#39472=CARTESIAN_POINT('Ctrl Pts',(-1.07901003836845,4.78248223987434,18.2797036176904));
#39473=CARTESIAN_POINT('Ctrl Pts',(-3.23451621663571,3.68344087079119,18.3590755077438));
#39474=CARTESIAN_POINT('Ctrl Pts',(-4.60324425657823,1.68862650319409,18.4384473977972));
#39475=CARTESIAN_POINT('Ctrl Pts',(-4.84847467695998,-0.720374489880202,
18.5178192878506));
#39476=CARTESIAN_POINT('Ctrl Pts',(-3.91669769333075,-2.94853678524982,
18.597191177904));
#39477=CARTESIAN_POINT('Ctrl Pts',(-2.02316502874899,-4.46849826887172,
18.6765630679574));
#39478=CARTESIAN_POINT('Ctrl Pts',(0.348982623889014,-4.88143613581971,
18.7559349580108));
#39479=CARTESIAN_POINT('Ctrl Pts',(3.43189297168081,-3.8881060605371,18.8617641447486));
#39480=CARTESIAN_POINT('Ctrl Pts',(5.55807194231376,-0.0182675279710476,
18.994050628171));
#39481=CARTESIAN_POINT('Ctrl Pts',(3.02540872544997,4.66632909528411,19.1527944082778));
#39482=CARTESIAN_POINT('Ctrl Pts',(-2.2762392030432,5.06930720888685,19.3115381883846));
#39483=CARTESIAN_POINT('Ctrl Pts',(-5.49476366156208,0.839647798275813,
19.4702819684914));
#39484=CARTESIAN_POINT('Ctrl Pts',(-3.68539651252317,-4.16147159288528,
19.6290257485982));
#39485=CARTESIAN_POINT('Ctrl Pts',(1.49629817009931,-5.35305176256653,19.787769528705));
#39486=CARTESIAN_POINT('Ctrl Pts',(5.30889903625351,-1.64699798333508,19.9465133088118));
#39487=CARTESIAN_POINT('Ctrl Pts',(4.26335305224425,3.56621538027062,20.1052570889186));
#39488=CARTESIAN_POINT('Ctrl Pts',(-0.682914143845088,5.51666761234037,
20.2640008690254));
#39489=CARTESIAN_POINT('Ctrl Pts',(-5.00517315099108,2.41778366488215,20.4227446491323));
#39490=CARTESIAN_POINT('Ctrl Pts',(-4.74574684718966,-2.89085235699305,
20.581488429239));
#39491=CARTESIAN_POINT('Ctrl Pts',(-0.146932230206273,-5.55932874556366,
20.7402322093459));
#39492=CARTESIAN_POINT('Ctrl Pts',(4.59246965375652,-3.13076985705421,20.8989759894527));
#39493=CARTESIAN_POINT('Ctrl Pts',(5.0299278500732,1.2629663218453,21.031262472875));
#39494=CARTESIAN_POINT('Ctrl Pts',(3.05056344532296,3.82678328180762,21.1370916596129));
#39495=CARTESIAN_POINT('Ctrl Pts',(0.861221142909519,4.82897211168878,21.2164635496663));
#39496=CARTESIAN_POINT('Ctrl Pts',(-1.56011376732917,4.64762681676397,21.2958354397197));
#39497=CARTESIAN_POINT('Ctrl Pts',(-3.58940432897566,3.338086676814,21.3752073297731));
#39498=CARTESIAN_POINT('Ctrl Pts',(-4.75071159562141,1.21328335035074,21.4545792198265));
#39499=CARTESIAN_POINT('Ctrl Pts',(-4.75136940590249,-1.2059521437222,21.5339511098799));
#39500=CARTESIAN_POINT('Ctrl Pts',(-3.59639816964331,-3.33201429213618,
21.6133229999333));
#39501=CARTESIAN_POINT('Ctrl Pts',(-1.56440212229559,-4.64609055668268,
21.6926948899867));
#39502=CARTESIAN_POINT('Ctrl Pts',(0.848175594776096,-4.82855605094712,
21.7720667800401));
#39503=CARTESIAN_POINT('Ctrl Pts',(3.05440612489727,-3.83470774368908,21.8514386700935));
#39504=CARTESIAN_POINT('Ctrl Pts',(4.5164489386699,-1.90677984789329,21.9308105601469));
#39505=CARTESIAN_POINT('Ctrl Pts',(4.87836953900972,0.485660146581216,22.0101824502003));
#39506=CARTESIAN_POINT('Ctrl Pts',(4.0518905292872,2.75978129753096,22.0895543402537));
#39507=CARTESIAN_POINT('Ctrl Pts',(2.23840092153696,4.36163277449212,22.1689262303071));
#39508=CARTESIAN_POINT('Ctrl Pts',(-0.120369299865574,4.90099648569508,
22.2482981203605));
#39509=CARTESIAN_POINT('Ctrl Pts',(-2.44981194564663,4.24649024808576,22.327670010414));
#39510=CARTESIAN_POINT('Ctrl Pts',(-4.18248893842781,2.55754735438689,22.4070419004673));
#39511=CARTESIAN_POINT('Ctrl Pts',(-4.89631923419535,0.245592132270486,
22.4864137905208));
#39512=CARTESIAN_POINT('Ctrl Pts',(-4.41741787585779,-2.12618907886207,
22.5657856805741));
#39513=CARTESIAN_POINT('Ctrl Pts',(-2.86244283812702,-3.98003518345998,
22.6451575706276));
#39514=CARTESIAN_POINT('Ctrl Pts',(-0.610183305945143,-4.86435360814152,
22.724529460681));
#39515=CARTESIAN_POINT('Ctrl Pts',(1.79071565870375,-4.56372621798445,22.8039013507344));
#39516=CARTESIAN_POINT('Ctrl Pts',(3.75540018385464,-3.15138524551451,22.8832732407878));
#39517=CARTESIAN_POINT('Ctrl Pts',(4.80527757305005,-0.971373790660912,
22.9626451308412));
#39518=CARTESIAN_POINT('Ctrl Pts',(4.68459996247748,1.44526216311697,23.0420170208946));
#39519=CARTESIAN_POINT('Ctrl Pts',(3.42276418043937,3.50983545637268,23.121388910948));
#39520=CARTESIAN_POINT('Ctrl Pts',(1.3271506148001,4.71942059955514,23.2007608010014));
#39521=CARTESIAN_POINT('Ctrl Pts',(-1.09175390014331,4.7793653318942,23.2801326910548));
#39522=CARTESIAN_POINT('Ctrl Pts',(-3.2447095830844,3.67506724782751,23.3595045811082));
#39523=CARTESIAN_POINT('Ctrl Pts',(-4.60726119282589,1.67553091707926,23.4388764711616));
#39524=CARTESIAN_POINT('Ctrl Pts',(-4.84749417441997,-0.732161036485464,
23.518248361215));
#39525=CARTESIAN_POINT('Ctrl Pts',(-3.90688830464649,-2.96150018209874,
23.5976202512684));
#39526=CARTESIAN_POINT('Ctrl Pts',(-2.01457309173102,-4.46942443856173,
23.6769921413218));
#39527=CARTESIAN_POINT('Ctrl Pts',(0.368487667211392,-4.88860679467339,
23.7563640313752));
#39528=CARTESIAN_POINT('Ctrl Pts',(2.66178564602131,-4.1169353563613,23.8357359214286));
#39529=CARTESIAN_POINT('Ctrl Pts',(4.30667853324075,-2.34238757791555,23.915107811482));
#39530=CARTESIAN_POINT('Ctrl Pts',(4.90247406242456,0.00276062972037378,
23.9944797015354));
#39531=CARTESIAN_POINT('Ctrl Pts',(4.30403776144901,2.34723635406859,24.0738515915888));
#39532=CARTESIAN_POINT('Ctrl Pts',(2.65714738860781,4.1199304980844,24.1532234816422));
#39533=CARTESIAN_POINT('Ctrl Pts',(0.362981793399119,4.88901869207872,24.2325953716956));
#39534=CARTESIAN_POINT('Ctrl Pts',(-2.01960536323572,4.46715275434179,24.311967261749));
#39535=CARTESIAN_POINT('Ctrl Pts',(-3.9102211237066,2.95709829352223,24.3913391518025));
#39536=CARTESIAN_POINT('Ctrl Pts',(-4.84831567357046,0.726701233826634,
24.4707110418558));
#39537=CARTESIAN_POINT('Ctrl Pts',(-4.60537125691712,-1.68071863790322,
24.5500829319093));
#39538=CARTESIAN_POINT('Ctrl Pts',(-3.2405685958952,-3.67871916964745,24.6294548219626));
#39539=CARTESIAN_POINT('Ctrl Pts',(-1.08637059779009,-4.78059185437233,
24.7088267120161));
#39540=CARTESIAN_POINT('Ctrl Pts',(1.33246487329615,-4.71792294503267,24.7881986020694));
#39541=CARTESIAN_POINT('Ctrl Pts',(3.42671485060842,-3.50597844922833,24.8675704921229));
#39542=CARTESIAN_POINT('Ctrl Pts',(4.68622467521711,-1.43998536354369,24.9469423821763));
#39543=CARTESIAN_POINT('Ctrl Pts',(4.80418054172532,0.976784969346655,25.0263142722297));
#39544=CARTESIAN_POINT('Ctrl Pts',(3.75184866214253,3.15561264578101,25.105686162283));
#39545=CARTESIAN_POINT('Ctrl Pts',(1.785574753038,4.56574006653325,25.1850580523365));
#39546=CARTESIAN_POINT('Ctrl Pts',(-0.615661213603954,4.86366331317224,
25.2644299423898));
#39547=CARTESIAN_POINT('Ctrl Pts',(-2.86692347135497,3.97680894225859,25.3438018324433));
#39548=CARTESIAN_POINT('Ctrl Pts',(-4.41980951731136,2.12121271552801,25.4231737224967));
#39549=CARTESIAN_POINT('Ctrl Pts',(-4.89603974793313,-0.25110623348048,
25.5025456125501));
#39550=CARTESIAN_POINT('Ctrl Pts',(-4.17960553315853,-2.56225625982736,
25.5819175026035));
#39551=CARTESIAN_POINT('Ctrl Pts',(-2.44502866190641,-4.24924633273829,
25.6612893926569));
#39552=CARTESIAN_POINT('Ctrl Pts',(-0.114848220593104,-4.9011294045414,
25.7406612827103));
#39553=CARTESIAN_POINT('Ctrl Pts',(2.24330899304448,-4.35910820186418,25.8200331727637));
#39554=CARTESIAN_POINT('Ctrl Pts',(4.05500110145669,-2.75521788993518,25.8994050628171));
#39555=CARTESIAN_POINT('Ctrl Pts',(4.87890391714675,-0.480162598589303,
25.9787769528705));
#39556=CARTESIAN_POINT('Ctrl Pts',(4.51431653789045,1.91185923895103,26.0581488429239));
#39557=CARTESIAN_POINT('Ctrl Pts',(3.05005164227427,3.83815639771151,26.1375207329773));
#39558=CARTESIAN_POINT('Ctrl Pts',(0.842800917774871,4.82948715360457,26.2168926230307));
#39559=CARTESIAN_POINT('Ctrl Pts',(-1.56975424478632,4.64436552876808,26.2962645130841));
#39560=CARTESIAN_POINT('Ctrl Pts',(-3.59992074790968,3.32788674125238,26.3756364031376));
#39561=CARTESIAN_POINT('Ctrl Pts',(-4.7531545251316,1.20074210971995,26.4550082931909));
#39562=CARTESIAN_POINT('Ctrl Pts',(-4.74853038096058,-1.21890064194263,
26.5343801832443));
#39563=CARTESIAN_POINT('Ctrl Pts',(-3.58717474668129,-3.34162189521881,
26.6137520732977));
#39564=CARTESIAN_POINT('Ctrl Pts',(-1.55199128418706,-4.65033145137433,
26.6931239633511));
#39565=CARTESIAN_POINT('Ctrl Pts',(0.861253819860729,-4.82623055930912,
26.7724958534045));
#39566=CARTESIAN_POINT('Ctrl Pts',(3.06469939974342,-3.82647058567632,26.851867743458));
#39567=CARTESIAN_POINT('Ctrl Pts',(4.52159098944567,-1.89459084712176,26.9312396335114));
#39568=CARTESIAN_POINT('Ctrl Pts',(4.87703302249084,0.49880702818598,27.0106115235648));
#39569=CARTESIAN_POINT('Ctrl Pts',(4.0444406063867,2.77069661551822,27.0899834136182));
#39570=CARTESIAN_POINT('Ctrl Pts',(2.22663141078423,4.36765064014314,27.1693553036716));
#39571=CARTESIAN_POINT('Ctrl Pts',(-0.133580267920228,4.90065463645992,
27.248727193725));
#39572=CARTESIAN_POINT('Ctrl Pts',(-2.46125208903423,4.23987001075014,27.3280990837784));
#39573=CARTESIAN_POINT('Ctrl Pts',(-4.1893683491486,2.54626243521474,27.4074709738318));
#39574=CARTESIAN_POINT('Ctrl Pts',(-4.89696375241997,0.232390966517291,
27.4868428638852));
#39575=CARTESIAN_POINT('Ctrl Pts',(-4.41166962484721,-2.13809042723509,
27.5662147539386));
#39576=CARTESIAN_POINT('Ctrl Pts',(-2.85170254172674,-3.98773772549588,
27.645586643992));
#39577=CARTESIAN_POINT('Ctrl Pts',(-0.597067031578144,-4.8659809405336,
27.7249585340454));
#39578=CARTESIAN_POINT('Ctrl Pts',(1.80301268587744,-4.55888196912345,27.8043304240988));
#39579=CARTESIAN_POINT('Ctrl Pts',(3.76388250395415,-3.14124944094887,27.8837023141522));
#39580=CARTESIAN_POINT('Ctrl Pts',(4.80787887528022,-0.958415501996903,
27.9630742042056));
#39581=CARTESIAN_POINT('Ctrl Pts',(4.68068659464744,1.45788633182479,28.042446094259));
#39582=CARTESIAN_POINT('Ctrl Pts',(3.41328942008259,3.51905028219065,28.1218179843124));
#39583=CARTESIAN_POINT('Ctrl Pts',(1.31442249797358,4.72298137310056,28.2011898743658));
#39584=CARTESIAN_POINT('Ctrl Pts',(-1.10463483521695,4.77640465566507,28.2805617644192));
#39585=CARTESIAN_POINT('Ctrl Pts',(-3.25460556761632,3.66630633650198,28.3599336544726));
#39586=CARTESIAN_POINT('Ctrl Pts',(-4.6117615876916,1.66310390899846,28.439305544526));
#39587=CARTESIAN_POINT('Ctrl Pts',(-4.84550269296638,-0.745226949519058,
28.5186774345794));
#39588=CARTESIAN_POINT('Ctrl Pts',(-3.89889006757279,-2.97202217266562,
28.5980493246329));
#39589=CARTESIAN_POINT('Ctrl Pts',(-2.00251645176526,-4.4748393730103,28.6774212146862));
#39590=CARTESIAN_POINT('Ctrl Pts',(0.381665739197275,-4.88759560697863,
28.7567931047396));
#39591=CARTESIAN_POINT('Ctrl Pts',(2.67287500089413,-4.10974436959635,28.8361649947931));
#39592=CARTESIAN_POINT('Ctrl Pts',(4.31297782868169,-2.33076850054527,28.9155368848464));
#39593=CARTESIAN_POINT('Ctrl Pts',(4.90244880401687,0.015977416170102,28.9949087748999));
#39594=CARTESIAN_POINT('Ctrl Pts',(4.29769410207987,2.35883126967183,29.0742806649532));
#39595=CARTESIAN_POINT('Ctrl Pts',(2.64603062966077,4.12707904706596,29.1536525550067));
#39596=CARTESIAN_POINT('Ctrl Pts',(0.349799952745733,4.88997950372933,29.23302444506));
#39597=CARTESIAN_POINT('Ctrl Pts',(-2.03164121838909,4.46169177707024,29.3123963351135));
#39598=CARTESIAN_POINT('Ctrl Pts',(-3.91817908568586,2.94654580930412,29.3917682251669));
#39599=CARTESIAN_POINT('Ctrl Pts',(-4.85025720045188,0.71362780446005,29.4711401152203));
#39600=CARTESIAN_POINT('Ctrl Pts',(-4.60082339705005,-1.69312835396218,
29.5505120052737));
#39601=CARTESIAN_POINT('Ctrl Pts',(-3.23063919787666,-3.68744219303526,
29.6298838953271));
#39602=CARTESIAN_POINT('Ctrl Pts',(-1.07347844099907,-4.78350327589979,
29.7092557853805));
#39603=CARTESIAN_POINT('Ctrl Pts',(1.34517928800161,-4.71431354886002,29.7886276754339));
#39604=CARTESIAN_POINT('Ctrl Pts',(3.43615431994896,-3.49672747627405,29.8679995654873));
#39605=CARTESIAN_POINT('Ctrl Pts',(4.69008976535537,-1.42734633034267,29.9473714555407));
#39606=CARTESIAN_POINT('Ctrl Pts',(4.8015297252588,0.989733222282683,30.0267433455941));
#39607=CARTESIAN_POINT('Ctrl Pts',(3.74332767209493,3.16571595269729,30.1061152356475));
#39608=CARTESIAN_POINT('Ctrl Pts',(1.77325928372404,4.57053728422822,30.1854871257009));
#39609=CARTESIAN_POINT('Ctrl Pts',(-0.628771141119161,4.86198585003386,
30.2648590157543));
#39610=CARTESIAN_POINT('Ctrl Pts',(-2.8776343077471,3.9690654245944,30.3442309058078));
#39611=CARTESIAN_POINT('Ctrl Pts',(-4.42551212654334,2.10928944710103,30.4236027958611));
#39612=CARTESIAN_POINT('Ctrl Pts',(-4.89534498701853,-0.264304770873174,
30.5029746859146));
#39613=CARTESIAN_POINT('Ctrl Pts',(-4.17268264431835,-2.57351493169134,
30.5823465759679));
#39614=CARTESIAN_POINT('Ctrl Pts',(-2.43356404553856,-4.25582255152819,
30.6617184660214));
#39615=CARTESIAN_POINT('Ctrl Pts',(-0.101634631868219,-4.90142121791616,
30.7410903560747));
#39616=CARTESIAN_POINT('Ctrl Pts',(2.25505275316072,-4.35304452473163,30.8204622461282));
#39617=CARTESIAN_POINT('Ctrl Pts',(4.06241427899435,-2.74427582062311,30.8998341361815));
#39618=CARTESIAN_POINT('Ctrl Pts',(4.88018067846643,-0.467007600962325,
30.979206026235));
#39619=CARTESIAN_POINT('Ctrl Pts',(4.50914586676086,1.9240226365891,31.0585779162884));
#39620=CARTESIAN_POINT('Ctrl Pts',(3.0396931027374,3.84636521861933,31.1379498063418));
#39621=CARTESIAN_POINT('Ctrl Pts',(0.829777827133663,4.83174174717888,31.2173216963951));
#39622=CARTESIAN_POINT('Ctrl Pts',(-1.58226949047778,4.64011668100458,31.2966935864486));
#39623=CARTESIAN_POINT('Ctrl Pts',(-3.60887946250293,3.31816946206164,31.376065476502));
#39624=CARTESIAN_POINT('Ctrl Pts',(-4.75637438558157,1.18792350680397,31.4554373665554));
#39625=CARTESIAN_POINT('Ctrl Pts',(-4.74522703638862,-1.23169798528705,
31.5348092566087));
#39626=CARTESIAN_POINT('Ctrl Pts',(-3.57815288451333,-3.35128057447936,
31.6141811466622));
#39627=CARTESIAN_POINT('Ctrl Pts',(-1.53944861007768,-4.65449863366224,
31.6935530367156));
#39628=CARTESIAN_POINT('Ctrl Pts',(0.874261938261232,-4.823891128243,31.772924926769));
#39629=CARTESIAN_POINT('Ctrl Pts',(3.07500421358568,-3.81819442148565,31.8522968168224));
#39630=CARTESIAN_POINT('Ctrl Pts',(4.52668226888703,-1.88239400508438,31.9316687068758));
#39631=CARTESIAN_POINT('Ctrl Pts',(4.87567054312872,0.511953424346944,32.0110405969291));
#39632=CARTESIAN_POINT('Ctrl Pts',(4.036956265178,2.78159013279705,32.0904124869827));
#39633=CARTESIAN_POINT('Ctrl Pts',(2.21484837668102,4.37363764184315,32.169784377036));
#39634=CARTESIAN_POINT('Ctrl Pts',(-0.146791673891742,4.90027670221896,
32.2491562670894));
#39635=CARTESIAN_POINT('Ctrl Pts',(-2.47267359762233,4.23321920451271,32.3285281571428));
#39636=CARTESIAN_POINT('Ctrl Pts',(-4.19621770614226,2.53495887865897,32.4079000471962));
#39637=CARTESIAN_POINT('Ctrl Pts',(-4.89757246961631,0.219188181000233,
32.4872719372496));
#39638=CARTESIAN_POINT('Ctrl Pts',(-4.40588942008463,-2.1499762723854,32.566643827303));
#39639=CARTESIAN_POINT('Ctrl Pts',(-2.84094146009112,-3.99541126470971,
32.6460157173564));
#39640=CARTESIAN_POINT('Ctrl Pts',(-0.583946448736662,-4.86757291664353,
32.7253876074098));
#39641=CARTESIAN_POINT('Ctrl Pts',(1.81529662498649,-4.55400458027289,32.8047594974633));
#39642=CARTESIAN_POINT('Ctrl Pts',(3.77233745895388,-3.13109080826592,32.8841313875166));
#39643=CARTESIAN_POINT('Ctrl Pts',(4.81044523784739,-0.945450245917296,
32.96350327757));
#39644=CARTESIAN_POINT('Ctrl Pts',(4.67673920454123,1.4704999036181,33.0428751676234));
#39645=CARTESIAN_POINT('Ctrl Pts',(3.40378985279549,3.52823953152847,33.1222470576768));
#39646=CARTESIAN_POINT('Ctrl Pts',(1.30168482706983,4.72650781918426,33.2016189477302));
#39647=CARTESIAN_POINT('Ctrl Pts',(-1.11750774129953,4.7734092640344,33.2809908377837));
#39648=CARTESIAN_POINT('Ctrl Pts',(-3.2644778974498,3.65751877792795,33.360362727837));
#39649=CARTESIAN_POINT('Ctrl Pts',(-4.61622846358057,1.65066481329873,33.4397346178904));
#39650=CARTESIAN_POINT('Ctrl Pts',(-4.84347599383145,-0.75828744616548,
33.5191065079439));
#39651=CARTESIAN_POINT('Ctrl Pts',(-3.89086349283728,-2.98252256218456,
33.5984783979973));
#39652=CARTESIAN_POINT('Ctrl Pts',(-1.99044525726817,-4.4802217837572,33.6778502880507));
#39653=CARTESIAN_POINT('Ctrl Pts',(0.394841037195618,-4.88654889560926,
33.7572221781041));
#39654=CARTESIAN_POINT('Ctrl Pts',(2.68394492896431,-4.10252351268344,33.8365940681574));
#39655=CARTESIAN_POINT('Ctrl Pts',(4.31924577684866,-2.31913248284973,33.9159659582109));
#39656=CARTESIAN_POINT('Ctrl Pts',(4.90238791398107,0.029194086493524,33.9953378482642));
#39657=CARTESIAN_POINT('Ctrl Pts',(4.29131920651926,2.37040904098698,34.0747097383177));
#39658=CARTESIAN_POINT('Ctrl Pts',(2.63489463902328,4.13419759990741,34.1540816283711));
#39659=CARTESIAN_POINT('Ctrl Pts',(0.336615569701593,4.89090477438156,34.2334535184245));
#39660=CARTESIAN_POINT('Ctrl Pts',(-2.04366230731349,4.45619837165044,34.3128254084779));
#39661=CARTESIAN_POINT('Ctrl Pts',(-3.92610856983677,2.93597190921303,34.3921972985313));
#39662=CARTESIAN_POINT('Ctrl Pts',(-4.85216347504172,0.700549188354975,
34.4715691885847));
#39663=CARTESIAN_POINT('Ctrl Pts',(-4.59624209780822,-1.70552576414703,
34.5509410786381));
#39664=CARTESIAN_POINT('Ctrl Pts',(-3.22068631915797,-3.69613841562006,
34.6303129686915));
#39665=CARTESIAN_POINT('Ctrl Pts',(-1.06057848202912,-4.7863799303117,34.709684858745));
#39666=CARTESIAN_POINT('Ctrl Pts',(1.35788392577142,-4.71066988845169,34.7890567487982));
#39667=CARTESIAN_POINT('Ctrl Pts',(3.44556881487913,-3.48745108865577,34.8684286388518));
#39668=CARTESIAN_POINT('Ctrl Pts',(4.69392076731947,-1.41469692300534,34.9478005289051));
#39669=CARTESIAN_POINT('Ctrl Pts',(4.79884401065818,1.00267428171067,35.0271724189586));
#39670=CARTESIAN_POINT('Ctrl Pts',(3.73477947506157,3.17579625078383,35.1065443090119));
#39671=CARTESIAN_POINT('Ctrl Pts',(1.76093092613411,4.57530128267181,35.1859161990653));
#39672=CARTESIAN_POINT('Ctrl Pts',(-0.64187649864509,4.86027304935852,35.2652880891187));
#39673=CARTESIAN_POINT('Ctrl Pts',(-2.88832422912388,3.96129305925348,35.3446599791721));
#39674=CARTESIAN_POINT('Ctrl Pts',(-4.43118257058537,2.09735084808771,35.4240318692256));
#39675=CARTESIAN_POINT('Ctrl Pts',(-4.89461464610851,-0.277501387264873,
35.5034037592789));
#39676=CARTESIAN_POINT('Ctrl Pts',(-4.16572942788534,-2.58475489891863,
35.5827756493324));
#39677=CARTESIAN_POINT('Ctrl Pts',(-2.42208174171502,-4.2623678384537,35.6621475393857));
#39678=CARTESIAN_POINT('Ctrl Pts',(-0.0884203044499451,-4.90167740713266,
35.7415194294392));
#39679=CARTESIAN_POINT('Ctrl Pts',(2.26678012326416,-4.34694920911302,35.8208913194925));
#39680=CARTESIAN_POINT('Ctrl Pts',(4.06979793038381,-2.73331380556231,35.900263209546));
#39681=CARTESIAN_POINT('Ctrl Pts',(4.88142197000686,-0.453849209064084,
35.9796350995994));
#39682=CARTESIAN_POINT('Ctrl Pts',(4.50394242258051,1.9361720501839,36.0590069896528));
#39683=CARTESIAN_POINT('Ctrl Pts',(3.02931247032103,3.85454608365127,36.1383788797062));
#39684=CARTESIAN_POINT('Ctrl Pts',(0.816748705560739,4.83396122303424,36.2177507697595));
#39685=CARTESIAN_POINT('Ctrl Pts',(-1.59477323603157,4.63583410827775,36.297122659813));
#39686=CARTESIAN_POINT('Ctrl Pts',(-3.61781194729725,3.3084280659895,36.3764945498664));
#39687=CARTESIAN_POINT('Ctrl Pts',(-4.75955967609224,1.17509626990754,36.4558664399198));
#39688=CARTESIAN_POINT('Ctrl Pts',(-4.74188920289779,-1.24448637649244,
36.5352383299732));
#39689=CARTESIAN_POINT('Ctrl Pts',(-3.56910501587113,-3.36091489620272,
36.6146102200266));
#39690=CARTESIAN_POINT('Ctrl Pts',(-1.52689474705826,-4.65863198645693,
36.69398211008));
#39691=CARTESIAN_POINT('Ctrl Pts',(0.887263702413796,-4.82151663651726,
36.7733540001334));
#39692=CARTESIAN_POINT('Ctrl Pts',(3.08528667790275,-3.80989050616806,36.8527258901868));
#39693=CARTESIAN_POINT('Ctrl Pts',(4.53174064782084,-1.87018348156595,36.9320977802402));
#39694=CARTESIAN_POINT('Ctrl Pts',(4.87427262676759,0.525096099564754,37.0114696702936));
#39695=CARTESIAN_POINT('Ctrl Pts',(4.02944258285317,2.79246343312197,37.090841560347));
#39696=CARTESIAN_POINT('Ctrl Pts',(2.20304924477561,4.37959285538367,37.1702134504005));
#39697=CARTESIAN_POINT('Ctrl Pts',(-0.160002012962556,4.89986315213815,
37.2495853404538));
#39698=CARTESIAN_POINT('Ctrl Pts',(-2.48407713450139,4.22653763069513,37.3289572305073));
#39699=CARTESIAN_POINT('Ctrl Pts',(-4.20303656448734,2.52363689769662,37.4083291205606));
#39700=CARTESIAN_POINT('Ctrl Pts',(-4.89814559062741,0.20598380239574,37.4877010106141));
#39701=CARTESIAN_POINT('Ctrl Pts',(-4.40007719275278,-2.16184649123314,
37.5670729006674));
#39702=CARTESIAN_POINT('Ctrl Pts',(-2.83015973012786,-4.0030557647603,37.6464447907209));
#39703=CARTESIAN_POINT('Ctrl Pts',(-0.570821621698638,-4.86912951461192,
37.7258166807742));
#39704=CARTESIAN_POINT('Ctrl Pts',(1.82756737028896,-4.54909409232726,37.8051885708277));
#39705=CARTESIAN_POINT('Ctrl Pts',(3.78076499611679,-3.12090941842365,37.884560460881));
#39706=CARTESIAN_POINT('Ctrl Pts',(4.81297663748916,-0.932478118164531,
37.9639323509345));
#39707=CARTESIAN_POINT('Ctrl Pts',(4.6727578232798,1.48310278759233,38.0433042409879));
#39708=CARTESIAN_POINT('Ctrl Pts',(3.39426554635479,3.53740313723864,38.1226761310413));
#39709=CARTESIAN_POINT('Ctrl Pts',(1.2889376953013,4.72999991227071,38.2020480210947));
#39710=CARTESIAN_POINT('Ctrl Pts',(-1.13037252509376,4.77037917890205,38.2814199111481));
#39711=CARTESIAN_POINT('Ctrl Pts',(-3.27432650082598,3.64870463556727,38.3607918012015));
#39712=CARTESIAN_POINT('Ctrl Pts',(-4.62066178777622,1.63821372124413,38.4401636912549));
#39713=CARTESIAN_POINT('Ctrl Pts',(-4.84141409235733,-0.771342433159972,
38.5195355813083));
#39714=CARTESIAN_POINT('Ctrl Pts',(-3.88280863754963,-2.99300127117752,
38.5989074713617));
#39715=CARTESIAN_POINT('Ctrl Pts',(-1.97835959833324,-4.48557163766163,
38.6782793614151));
#39716=CARTESIAN_POINT('Ctrl Pts',(0.4080134699205,-4.88546665687603,38.7576512514685));
#39717=CARTESIAN_POINT('Ctrl Pts',(2.69499534131588,-4.09527285943909,38.8370231415219));
#39718=CARTESIAN_POINT('Ctrl Pts',(4.32548234816251,-2.30747956911512,38.9163950315754));
#39719=CARTESIAN_POINT('Ctrl Pts',(4.90229136258888,0.0424104685617285,
38.9957669216287));
#39720=CARTESIAN_POINT('Ctrl Pts',(4.28491317807095,2.38196972749885,39.0751388116822));
#39721=CARTESIAN_POINT('Ctrl Pts',(2.62373939006081,4.14128583366062,39.1545107017355));
#39722=CARTESIAN_POINT('Ctrl Pts',(0.323428943211332,4.89179500940948,39.233882591789));
#39723=CARTESIAN_POINT('Ctrl Pts',(-2.05566892616818,4.45067161106171,39.3132544818423));
#39724=CARTESIAN_POINT('Ctrl Pts',(-3.93400879434316,2.92537849589611,39.3926263718958));
#39725=CARTESIAN_POINT('Ctrl Pts',(-4.85403585089548,0.68746203308737,39.4719982619491));
#39726=CARTESIAN_POINT('Ctrl Pts',(-4.59162481050186,-1.71790426872522,
39.5513701520026));
#39727=CARTESIAN_POINT('Ctrl Pts',(-3.21071490770548,-3.70482006635682,
39.6307420420559));
#39728=CARTESIAN_POINT('Ctrl Pts',(-1.04766160592177,-4.78919858119775,
39.7101139321094));
#39729=CARTESIAN_POINT('Ctrl Pts',(1.37056128557131,-4.7070358700676,39.7894858221627));
#39730=CARTESIAN_POINT('Ctrl Pts',(3.45499130789194,-3.47806613859367,39.8688577122162));
#39731=CARTESIAN_POINT('Ctrl Pts',(4.69765387924814,-1.40219731261544,39.9482296022695));
#39732=CARTESIAN_POINT('Ctrl Pts',(4.79625497710706,1.0159342797995,40.027601492323));
#39733=CARTESIAN_POINT('Ctrl Pts',(4.08267404777822,2.46201708819427,40.0805160856919));
#39734=CARTESIAN_POINT('Ctrl Pts',(3.57461543774186,3.05624720968413,40.1069733823764));
#39735=CARTESIAN_POINT('Ctrl Pts',(1.16918346556923,-4.36383719750629,-0.320920147129053));
#39736=CARTESIAN_POINT('Ctrl Pts',(1.8946107326977,-4.16947670058299,-0.294462850444586));
#39737=CARTESIAN_POINT('Ctrl Pts',(3.24594541476064,-3.41224896374509,-0.24154825707565));
#39738=CARTESIAN_POINT('Ctrl Pts',(4.48258575488109,-1.44364637546346,-0.162176367022246));
#39739=CARTESIAN_POINT('Ctrl Pts',(4.62712170766666,0.875927969712858,-0.0828044769688426));
#39740=CARTESIAN_POINT('Ctrl Pts',(3.64458116255458,2.98248116081162,-0.00343258691543892));
#39741=CARTESIAN_POINT('Ctrl Pts',(1.77418661813218,4.36232362711486,0.0759393031379646));
#39742=CARTESIAN_POINT('Ctrl Pts',(-0.52837360592073,4.67961139929734,0.155311193191369));
#39743=CARTESIAN_POINT('Ctrl Pts',(-2.70223496968603,3.85690448821556,0.234683083244771));
#39744=CARTESIAN_POINT('Ctrl Pts',(-4.21783163769356,2.09469156016015,0.314054973298176));
#39745=CARTESIAN_POINT('Ctrl Pts',(-4.70597715859854,-0.177798095133649,
0.393426863351579));
#39746=CARTESIAN_POINT('Ctrl Pts',(-4.04775531046147,-2.4069688489564,0.472798753404983));
#39747=CARTESIAN_POINT('Ctrl Pts',(-2.40351015490329,-4.04981138575499,
0.552170643458387));
#39748=CARTESIAN_POINT('Ctrl Pts',(-0.173774754931243,-4.70612667927193,
0.631542533511791));
#39749=CARTESIAN_POINT('Ctrl Pts',(2.0982915307903,-4.21604107122297,0.710914423565194));
#39750=CARTESIAN_POINT('Ctrl Pts',(3.85921878174909,-2.69893658616936,0.790286313618597));
#39751=CARTESIAN_POINT('Ctrl Pts',(4.68004880681062,-0.524377442655228,
0.869658203672002));
#39752=CARTESIAN_POINT('Ctrl Pts',(4.36082934025305,1.77791905463906,0.949030093725404));
#39753=CARTESIAN_POINT('Ctrl Pts',(2.97932147849509,3.64711831584472,1.02840198377881));
#39754=CARTESIAN_POINT('Ctrl Pts',(0.872057510020645,4.62788767559441,1.10777387383221));
#39755=CARTESIAN_POINT('Ctrl Pts',(-1.44763774336318,4.48131381605584,1.18714576388562));
#39756=CARTESIAN_POINT('Ctrl Pts',(-3.4146916437183,3.2431018434756,1.26651765393902));
#39757=CARTESIAN_POINT('Ctrl Pts',(-4.54993421956391,1.21487743324944,1.34588954399242));
#39758=CARTESIAN_POINT('Ctrl Pts',(-4.57682288978047,-1.10928842689199,
1.42526143404583));
#39759=CARTESIAN_POINT('Ctrl Pts',(-3.48880763512327,-3.16323408359086,
1.50463332409923));
#39760=CARTESIAN_POINT('Ctrl Pts',(-1.55092656265583,-4.44662291817823,
1.58400521415264));
#39761=CARTESIAN_POINT('Ctrl Pts',(0.764756787430318,-4.64682425288564,
1.66337710420604));
#39762=CARTESIAN_POINT('Ctrl Pts',(2.89414707692588,-3.71506948486699,1.74274899425944));
#39763=CARTESIAN_POINT('Ctrl Pts',(4.31852954453272,-1.87833201365734,1.82212088431284));
#39764=CARTESIAN_POINT('Ctrl Pts',(4.69092777401317,0.415962978544339,1.90149277436625));
#39765=CARTESIAN_POINT('Ctrl Pts',(3.92062638092659,2.60893030984735,1.98086466441965));
#39766=CARTESIAN_POINT('Ctrl Pts',(2.19526907961086,4.166367992464,2.06023655447306));
#39767=CARTESIAN_POINT('Ctrl Pts',(-0.0648509103551908,4.70888765420329,
2.13960844452646));
#39768=CARTESIAN_POINT('Ctrl Pts',(-2.30917336210229,4.10433270633116,2.21898033457986));
#39769=CARTESIAN_POINT('Ctrl Pts',(-3.99098629411059,2.49997139597969,2.29835222463327));
#39770=CARTESIAN_POINT('Ctrl Pts',(-4.70060379877146,0.286622587162194,
2.37772411468667));
#39771=CARTESIAN_POINT('Ctrl Pts',(-4.26516462266185,-1.99654684946062,
2.45709600474007));
#39772=CARTESIAN_POINT('Ctrl Pts',(-2.79074078525346,-3.79336189283582,
2.53646789479348));
#39773=CARTESIAN_POINT('Ctrl Pts',(-0.636498669757338,-4.66612237558061,
2.61583978484688));
#39774=CARTESIAN_POINT('Ctrl Pts',(1.6727931128258,-4.40222577592052,2.69521167490029));
#39775=CARTESIAN_POINT('Ctrl Pts',(3.5745961957893,-3.06595672140773,2.77458356495369));
#39776=CARTESIAN_POINT('Ctrl Pts',(4.60563555769302,-0.982827395940078,
2.85395545500709));
#39777=CARTESIAN_POINT('Ctrl Pts',(4.51475229214408,1.33971650772703,2.9333273450605));
#39778=CARTESIAN_POINT('Ctrl Pts',(3.32408536146356,3.33590843552402,3.0126992351139));
#39779=CARTESIAN_POINT('Ctrl Pts',(1.32367859446866,4.51948045233543,3.0920711251673));
#39780=CARTESIAN_POINT('Ctrl Pts',(-0.99917334822593,4.60211703465825,3.17144301522071));
#39781=CARTESIAN_POINT('Ctrl Pts',(-3.07862887492539,3.56368809395157,3.25081490527411));
#39782=CARTESIAN_POINT('Ctrl Pts',(-4.40813722212245,1.65715262164811,3.33018679532752));
#39783=CARTESIAN_POINT('Ctrl Pts',(-4.66383309925671,-0.653061561243739,
3.40955868538092));
#39784=CARTESIAN_POINT('Ctrl Pts',(-3.7834295566315,-2.80419139334385,3.48893057543432));
#39785=CARTESIAN_POINT('Ctrl Pts',(-1.98139094849014,-4.27222640899777,
3.56830246548773));
#39786=CARTESIAN_POINT('Ctrl Pts',(0.303310108968963,-4.69955652783259,
3.64767435554113));
#39787=CARTESIAN_POINT('Ctrl Pts',(2.51412549524875,-3.98208507877931,3.72704624559453));
#39788=CARTESIAN_POINT('Ctrl Pts',(4.11250547580833,-2.29458651873122,3.80641813564794));
#39789=CARTESIAN_POINT('Ctrl Pts',(4.70908822533748,-0.0481317617013215,
3.88579002570134));
#39790=CARTESIAN_POINT('Ctrl Pts',(4.15854750656441,2.21004778594118,3.96516191575474));
#39791=CARTESIAN_POINT('Ctrl Pts',(2.59499381998102,3.92986458478622,4.04453380580815));
#39792=CARTESIAN_POINT('Ctrl Pts',(0.399305382771643,4.69237506938503,4.12390569586155));
#39793=CARTESIAN_POINT('Ctrl Pts',(-1.89365296183344,4.3118333734777,4.20327758591496));
#39794=CARTESIAN_POINT('Ctrl Pts',(-3.72532163646561,2.88093861187248,4.28264947596836));
#39795=CARTESIAN_POINT('Ctrl Pts',(-4.64951020631435,0.748253581264596,
4.36202136602176));
#39796=CARTESIAN_POINT('Ctrl Pts',(-4.44108838142119,-1.56670436550815,
4.44139325607517));
#39797=CARTESIAN_POINT('Ctrl Pts',(-3.15082725699623,-3.5000165966844,4.52076514612857));
#39798=CARTESIAN_POINT('Ctrl Pts',(-1.09303158700481,-4.58073253206366,
4.60013703618198));
#39799=CARTESIAN_POINT('Ctrl Pts',(1.23102415819659,-4.54559216191169,4.67950892623538));
#39800=CARTESIAN_POINT('Ctrl Pts',(3.25520514328707,-3.40315560261561,4.75888081628878));
#39801=CARTESIAN_POINT('Ctrl Pts',(4.48642536074717,-1.43171787127954,4.83825270634219));
#39802=CARTESIAN_POINT('Ctrl Pts',(4.62476229086337,0.888483164446475,4.91762459639559));
#39803=CARTESIAN_POINT('Ctrl Pts',(3.63651736366295,2.99225166793745,4.99699648644899));
#39804=CARTESIAN_POINT('Ctrl Pts',(1.76242485596889,4.36711428835561,5.0763683765024));
#39805=CARTESIAN_POINT('Ctrl Pts',(-0.540990445577951,4.67815753457383,
5.15574026655579));
#39806=CARTESIAN_POINT('Ctrl Pts',(-2.71262167204403,3.84961196029596,5.23511215660921));
#39807=CARTESIAN_POINT('Ctrl Pts',(-4.22346426348642,2.08330943346152,5.3144840466626));
#39808=CARTESIAN_POINT('Ctrl Pts',(-4.70548030882309,-0.190482660036918,
5.39385593671601));
#39809=CARTESIAN_POINT('Ctrl Pts',(-4.04125176633447,-2.41787359917659,
5.47322782676941));
#39810=CARTESIAN_POINT('Ctrl Pts',(-2.39258323872581,-4.05627588142928,
5.55259971682282));
#39811=CARTESIAN_POINT('Ctrl Pts',(-0.161086730056731,-4.70657833738016,
5.63197160687622));
#39812=CARTESIAN_POINT('Ctrl Pts',(2.10965014949475,-4.21036872817968,5.71134349692963));
#39813=CARTESIAN_POINT('Ctrl Pts',(3.86648092226071,-2.68852261628773,5.79071538698303));
#39814=CARTESIAN_POINT('Ctrl Pts',(4.68144550067431,-0.511758346011949,
5.87008727703643));
#39815=CARTESIAN_POINT('Ctrl Pts',(4.3560203173275,1.78966912459444,5.94945916708984));
#39816=CARTESIAN_POINT('Ctrl Pts',(2.96947822656715,3.65513715781504,6.02883105714324));
#39817=CARTESIAN_POINT('Ctrl Pts',(0.859577812643608,4.63022186990077,6.10820294719665));
#39818=CARTESIAN_POINT('Ctrl Pts',(-1.45971385379671,4.47739478330096,6.18757483725004));
#39819=CARTESIAN_POINT('Ctrl Pts',(-3.42342245647396,3.23388423803426,6.26694672730346));
#39820=CARTESIAN_POINT('Ctrl Pts',(-4.55319292637122,1.20260665046377,6.34631861735685));
#39821=CARTESIAN_POINT('Ctrl Pts',(-4.57381567772605,-1.12162325523503,
6.42569050741026));
#39822=CARTESIAN_POINT('Ctrl Pts',(-3.48026705395609,-3.17262821862952,
6.50506239746367));
#39823=CARTESIAN_POINT('Ctrl Pts',(-1.5389330792829,-4.45078797045933,6.58443428751706));
#39824=CARTESIAN_POINT('Ctrl Pts',(0.777281587133017,-4.64474562433731,
6.66380617757047));
#39825=CARTESIAN_POINT('Ctrl Pts',(2.90415217940695,-3.70725352509678,6.74317806762387));
#39826=CARTESIAN_POINT('Ctrl Pts',(4.32357772900916,-1.86668267300916,6.82254995767728));
#39827=CARTESIAN_POINT('Ctrl Pts',(4.68978931390171,0.428607946391479,6.90192184773068));
#39828=CARTESIAN_POINT('Ctrl Pts',(3.91357860260037,2.61949061875875,6.98129373778408));
#39829=CARTESIAN_POINT('Ctrl Pts',(2.18402880626489,4.17227117454053,7.06066562783749));
#39830=CARTESIAN_POINT('Ctrl Pts',(-0.0775455730109682,4.70869570736982,
7.14003751789088));
#39831=CARTESIAN_POINT('Ctrl Pts',(-2.32023002234555,4.09809238840499,7.2194094079443));
#39832=CARTESIAN_POINT('Ctrl Pts',(-3.9977115739788,2.48920283459836,7.29878129799769));
#39833=CARTESIAN_POINT('Ctrl Pts',(-4.70135943497531,0.273948980040579,
7.37815318805111));
#39834=CARTESIAN_POINT('Ctrl Pts',(-4.25976654389442,-2.00803823967931,
7.4575250781045));
#39835=CARTESIAN_POINT('Ctrl Pts',(-2.78050395155417,-3.80087178893057,
7.53689696815791));
#39836=CARTESIAN_POINT('Ctrl Pts',(-0.623916751156424,-4.66782138348534,
7.61626885821132));
#39837=CARTESIAN_POINT('Ctrl Pts',(1.68465518880672,-4.39770002107047,7.69564074826471));
#39838=CARTESIAN_POINT('Ctrl Pts',(3.58284885369757,-3.05630866766671,7.77501263831812));
#39839=CARTESIAN_POINT('Ctrl Pts',(4.6082684683291,-0.970407287843808,7.85438452837152));
#39840=CARTESIAN_POINT('Ctrl Pts',(4.51112408430488,1.35188315933773,7.93375641842493));
#39841=CARTESIAN_POINT('Ctrl Pts',(3.31507985854782,3.3448578612472,8.01312830847833));
#39842=CARTESIAN_POINT('Ctrl Pts',(1.31148951705327,4.52303259187419,8.09250019853174));
#39843=CARTESIAN_POINT('Ctrl Pts',(-1.01157676786264,4.5994065946834,8.17187208858514));
#39844=CARTESIAN_POINT('Ctrl Pts',(-3.08822519121439,3.55537533164157,8.25124397863854));
#39845=CARTESIAN_POINT('Ctrl Pts',(-4.41258879365683,1.64526250750169,8.33061586869195));
#39846=CARTESIAN_POINT('Ctrl Pts',(-4.66205553306411,-0.665632621738795,
8.40998775874535));
#39847=CARTESIAN_POINT('Ctrl Pts',(-3.77585586390188,-2.81438111767656,
8.48935964879875));
#39848=CARTESIAN_POINT('Ctrl Pts',(-1.96986606400833,-4.27755260287526,
8.56873153885216));
#39849=CARTESIAN_POINT('Ctrl Pts',(0.315978748853086,-4.69872174221563,
8.64810342890556));
#39850=CARTESIAN_POINT('Ctrl Pts',(2.52485183790096,-3.97529266559641,8.72747531895897));
#39851=CARTESIAN_POINT('Ctrl Pts',(4.11867660790092,-2.28349109479901,8.80684720901236));
#39852=CARTESIAN_POINT('Ctrl Pts',(4.70920087275226,-0.0354361477303297,
8.88621909906579));
#39853=CARTESIAN_POINT('Ctrl Pts',(4.15257422864046,2.22125096648886,8.96559098911916));
#39854=CARTESIAN_POINT('Ctrl Pts',(2.58438969399899,3.93684626192698,9.04496287917259));
#39855=CARTESIAN_POINT('Ctrl Pts',(0.386653550348944,4.69343452202107,9.12433476922598));
#39856=CARTESIAN_POINT('Ctrl Pts',(-1.90527054232303,4.30671252129195,9.20370665927939));
#39857=CARTESIAN_POINT('Ctrl Pts',(-3.7330749481299,2.87088488312254,9.28307854933279));
#39858=CARTESIAN_POINT('Ctrl Pts',(-4.65151055959357,0.735716042020416,
9.3624504393862));
#39859=CARTESIAN_POINT('Ctrl Pts',(-4.43684849468422,-1.57867159843805,
9.4418223294396));
#39860=CARTESIAN_POINT('Ctrl Pts',(-3.14137995726738,-3.50849833184732,
9.52119421949301));
#39861=CARTESIAN_POINT('Ctrl Pts',(-1.08067821558679,-4.58366263754791,
9.6005661095464));
#39862=CARTESIAN_POINT('Ctrl Pts',(1.24327434737007,-4.54225687050701,9.67993799959982));
#39863=CARTESIAN_POINT('Ctrl Pts',(3.26436803124868,-3.39436738392564,9.75930988965321));
#39864=CARTESIAN_POINT('Ctrl Pts',(4.49026888827119,-1.41961751592476,9.83868177970662));
#39865=CARTESIAN_POINT('Ctrl Pts',(4.62235018315245,0.900948036685318,9.91805366976003));
#39866=CARTESIAN_POINT('Ctrl Pts',(3.62843720481635,3.00204464177353,9.99742555981342));
#39867=CARTESIAN_POINT('Ctrl Pts',(1.7506449547965,4.37184981703879,10.0767974498668));
#39868=CARTESIAN_POINT('Ctrl Pts',(-0.553600531224886,4.67668205379884,
10.1561693399202));
#39869=CARTESIAN_POINT('Ctrl Pts',(-2.72299015321387,3.84228489391363,10.2355412299736));
#39870=CARTESIAN_POINT('Ctrl Pts',(-4.22906540111646,2.07191563862441,10.314913120027));
#39871=CARTESIAN_POINT('Ctrl Pts',(-4.70494967818453,-0.203167680126261,
10.3942850100804));
#39872=CARTESIAN_POINT('Ctrl Pts',(-4.03471862787632,-2.42875980170217,
10.4736569001339));
#39873=CARTESIAN_POINT('Ctrl Pts',(-2.38163905051565,-4.06271141155209,
10.5530287901872));
#39874=CARTESIAN_POINT('Ctrl Pts',(-0.148397472117971,-4.70699551420709,
10.6324006802407));
#39875=CARTESIAN_POINT('Ctrl Pts',(2.12099340201542,-4.20466592835908,10.7117725702941));
#39876=CARTESIAN_POINT('Ctrl Pts',(3.87371497815709,-2.67808902923296,10.7911444603475));
#39877=CARTESIAN_POINT('Ctrl Pts',(4.68280815994238,-0.499135570435235,
10.8705163504009));
#39878=CARTESIAN_POINT('Ctrl Pts',(4.35117963918574,1.80140620850268,10.9498882404543));
#39879=CARTESIAN_POINT('Ctrl Pts',(2.95961338949625,3.66312942239435,11.0292601305077));
#39880=CARTESIAN_POINT('Ctrl Pts',(0.847091869118581,4.6325224171902,11.1086320205611));
#39881=CARTESIAN_POINT('Ctrl Pts',(-1.47177935557031,4.47344320507298,11.1880039106145));
#39882=CARTESIAN_POINT('Ctrl Pts',(-3.43212838697064,3.22464312999856,11.2673758006679));
#39883=CARTESIAN_POINT('Ctrl Pts',(-4.55641854019224,1.19032712608301,11.3467476907213));
#39884=CARTESIAN_POINT('Ctrl Pts',(-4.5707752224844,-1.13394993100199,11.4261195807747));
#39885=CARTESIAN_POINT('Ctrl Pts',(-3.47170117781866,-3.1819992948505,11.5054914708281));
#39886=CARTESIAN_POINT('Ctrl Pts',(-1.52692841071655,-4.45492067370938,
11.5848633608815));
#39887=CARTESIAN_POINT('Ctrl Pts',(0.789800737437414,-4.64263323725232,
11.6642352509349));
#39888=CARTESIAN_POINT('Ctrl Pts',(2.91413617414593,-3.69941062049495,11.7436071409883));
#39889=CARTESIAN_POINT('Ctrl Pts',(4.32859448916348,-1.85501976509151,11.8229790310417));
#39890=CARTESIAN_POINT('Ctrl Pts',(4.68861676780219,0.441249799071602,11.9023509210951));
#39891=CARTESIAN_POINT('Ctrl Pts',(3.90650237988148,2.63003188887072,11.9817228111485));
#39892=CARTESIAN_POINT('Ctrl Pts',(2.17277265911798,4.17814403201782,12.0610947012019));
#39893=CARTESIAN_POINT('Ctrl Pts',(-0.0902396720559702,4.70846953713027,
12.1404665912553));
#39894=CARTESIAN_POINT('Ctrl Pts',(-2.33126981885919,4.09182228501836,12.2198384813087));
#39895=CARTESIAN_POINT('Ctrl Pts',(-4.00440779796651,2.47841618137099,12.2992103713621));
#39896=CARTESIAN_POINT('Ctrl Pts',(-4.70208090109554,0.261273381822832,
12.3785822614155));
#39897=CARTESIAN_POINT('Ctrl Pts',(-4.25433750459725,-2.01951503521857,
12.4579541514689));
#39898=CARTESIAN_POINT('Ctrl Pts',(-2.7702469087954,-3.80835405980145,12.5373260415224));
#39899=CARTESIAN_POINT('Ctrl Pts',(-0.611330297848498,-4.66948646506541,
12.6166979315757));
#39900=CARTESIAN_POINT('Ctrl Pts',(1.69650502049761,-4.3931423031724,12.6960698216292));
#39901=CARTESIAN_POINT('Ctrl Pts',(3.59107547100067,-3.04663840028217,12.7754417116826));
#39902=CARTESIAN_POINT('Ctrl Pts',(4.61086788547872,-0.957980126702884,
12.854813601736));
#39903=CARTESIAN_POINT('Ctrl Pts',(4.50746308903707,1.36403998528818,12.9341854917894));
#39904=CARTESIAN_POINT('Ctrl Pts',(3.30605026120632,3.35378297611432,13.0135573818428));
#39905=CARTESIAN_POINT('Ctrl Pts',(1.29929090756384,4.52655185743172,13.0929292718962));
#39906=CARTESIAN_POINT('Ctrl Pts',(-1.02397283522957,4.59666272563134,13.1723011619496));
#39907=CARTESIAN_POINT('Ctrl Pts',(-3.09779906188647,3.54703672840752,13.251673052003));
#39908=CARTESIAN_POINT('Ctrl Pts',(-4.41700829392973,1.63336043537625,13.3310449420564));
#39909=CARTESIAN_POINT('Ctrl Pts',(-4.66024408245374,-0.67819884433063,
13.4104168321098));
#39910=CARTESIAN_POINT('Ctrl Pts',(-3.76825472776737,-2.82455038672626,
13.4897887221632));
#39911=CARTESIAN_POINT('Ctrl Pts',(-1.95832686228722,-4.28284770695163,
13.5691606122166));
#39912=CARTESIAN_POINT('Ctrl Pts',(0.328645092163131,-4.69785280568621,
13.64853250227));
#39913=CARTESIAN_POINT('Ctrl Pts',(2.53555982960612,-3.96847135947639,13.7279043923234));
#39914=CARTESIAN_POINT('Ctrl Pts',(4.12481780492351,-2.2723790741605,13.8072762823768));
#39915=CARTESIAN_POINT('Ctrl Pts',(4.7092792930909,-0.0227402762048894,
13.8866481724302));
#39916=CARTESIAN_POINT('Ctrl Pts',(4.14657076927425,2.23243800269952,13.9660200624836));
#39917=CARTESIAN_POINT('Ctrl Pts',(2.57376678434109,3.94379932556401,14.045391952537));
#39918=CARTESIAN_POINT('Ctrl Pts',(0.373998907678603,4.69445986217284,14.1247638425904));
#39919=CARTESIAN_POINT('Ctrl Pts',(-1.91687427506185,4.30156036736702,14.2041357326438));
#39920=CARTESIAN_POINT('Ctrl Pts',(-3.7408011273265,2.86081028841297,14.2835076226972));
#39921=CARTESIAN_POINT('Ctrl Pts',(-4.65347710509724,0.723173155497658,
14.3628795127506));
#39922=CARTESIAN_POINT('Ctrl Pts',(-4.43257636036315,-1.59062735738022,
14.442251402804));
#39923=CARTESIAN_POINT('Ctrl Pts',(-3.13190982558595,-3.51695456679423,
14.5216232928574));
#39924=CARTESIAN_POINT('Ctrl Pts',(-1.06831698966085,-4.58655942838405,
14.6009951829108));
#39925=CARTESIAN_POINT('Ctrl Pts',(1.25551550026611,-4.53888856539661,14.6803670729642));
#39926=CARTESIAN_POINT('Ctrl Pts',(3.27350719336465,-3.38555449453801,14.7597389630177));
#39927=CARTESIAN_POINT('Ctrl Pts',(4.49407977994485,-1.40750684260771,14.839110853071));
#39928=CARTESIAN_POINT('Ctrl Pts',(4.61990447960734,0.913406360718275,14.9184827431245));
#39929=CARTESIAN_POINT('Ctrl Pts',(3.62033067402261,3.01181579636398,14.9978546331779));
#39930=CARTESIAN_POINT('Ctrl Pts',(1.73885232971199,4.37655357055661,15.0772265232313));
#39931=CARTESIAN_POINT('Ctrl Pts',(-0.566206593232149,4.67517258229866,
15.1565984132847));
#39932=CARTESIAN_POINT('Ctrl Pts',(-2.73333884334193,3.83492990131171,15.2359703033381));
#39933=CARTESIAN_POINT('Ctrl Pts',(-4.23463580135657,2.06050678483865,15.3153421933915));
#39934=CARTESIAN_POINT('Ctrl Pts',(-4.70438485136804,-0.21585122356682,
15.3947140834449));
#39935=CARTESIAN_POINT('Ctrl Pts',(-4.02815616456562,-2.43962835168982,
15.4740859734983));
#39936=CARTESIAN_POINT('Ctrl Pts',(-2.3706775522472,-4.06911741336723,15.5534578635517));
#39937=CARTESIAN_POINT('Ctrl Pts',(-0.135707135607595,-4.70737847998642,
15.6328297536051));
#39938=CARTESIAN_POINT('Ctrl Pts',(2.13232123888424,-4.19893256848759,15.7122016436585));
#39939=CARTESIAN_POINT('Ctrl Pts',(3.88092087939525,-2.66763597748263,15.7915735337119));
#39940=CARTESIAN_POINT('Ctrl Pts',(4.6841367839613,-0.486509167079024,15.8709454237653));
#39941=CARTESIAN_POINT('Ctrl Pts',(4.34630733610955,1.81313019956284,15.9503173138187));
#39942=CARTESIAN_POINT('Ctrl Pts',(2.94972704158046,3.67109506287253,16.0296892038721));
#39943=CARTESIAN_POINT('Ctrl Pts',(0.834599768811967,4.63478929472454,16.1090610939255));
#39944=CARTESIAN_POINT('Ctrl Pts',(-1.48383416024523,4.46945911326284,16.1884329839789));
#39945=CARTESIAN_POINT('Ctrl Pts',(-3.44080937235088,3.21537858488636,16.2678048740323));
#39946=CARTESIAN_POINT('Ctrl Pts',(-4.55961103731638,1.17803895016983,16.3471767640857));
#39947=CARTESIAN_POINT('Ctrl Pts',(-4.5677015463797,-1.14626836492032,16.4265486541391));
#39948=CARTESIAN_POINT('Ctrl Pts',(-3.4631100686894,-3.19134724418507,16.5059205441925));
#39949=CARTESIAN_POINT('Ctrl Pts',(-1.51491264465833,-4.45902099747165,
16.5852924342459));
#39950=CARTESIAN_POINT('Ctrl Pts',(0.802314148161232,-4.64048710795702,
16.6646643242993));
#39951=CARTESIAN_POINT('Ctrl Pts',(2.92409898707282,-3.69154082613136,16.7440362143527));
#39952=CARTESIAN_POINT('Ctrl Pts',(4.33357979136326,-1.84334337837345,16.8234081044061));
#39953=CARTESIAN_POINT('Ctrl Pts',(4.68741013889918,0.453888451717908,16.9027799944596));
#39954=CARTESIAN_POINT('Ctrl Pts',(3.89939777427618,2.64055403030628,16.9821518845129));
#39955=CARTESIAN_POINT('Ctrl Pts',(2.16150070095874,4.18398654725935,17.0615237745663));
#39956=CARTESIAN_POINT('Ctrl Pts',(-0.102933079310061,4.70820909782832,
17.1408956646198));
#39957=CARTESIAN_POINT('Ctrl Pts',(-2.34229273922368,4.08552253105771,17.2202675546731));
#39958=CARTESIAN_POINT('Ctrl Pts',(-4.01107478934828,2.46761134605149,17.2996394447266));
#39959=CARTESIAN_POINT('Ctrl Pts',(-4.70276843368481,0.248596203073432,
17.37901133478));
#39960=CARTESIAN_POINT('Ctrl Pts',(-4.24887708766866,-2.03097775393694,
17.4583832248334));
#39961=CARTESIAN_POINT('Ctrl Pts',(-2.75997059360591,-3.81580751573978,
17.5377551148868));
#39962=CARTESIAN_POINT('Ctrl Pts',(-0.598737773532647,-4.6711197519463,
17.6171270049402));
#39963=CARTESIAN_POINT('Ctrl Pts',(1.70833944819094,-4.38854860755889,17.6964988949936));
#39964=CARTESIAN_POINT('Ctrl Pts',(3.5992817914533,-3.03695363259626,17.775870785047));
#39965=CARTESIAN_POINT('Ctrl Pts',(4.61342283197251,-0.945531571192997,
17.8552426751004));
#39966=CARTESIAN_POINT('Ctrl Pts',(4.50379002440264,1.37615964733967,17.9346145651538));
#39967=CARTESIAN_POINT('Ctrl Pts',(3.29695756540449,3.36273516855535,18.0139864552072));
#39968=CARTESIAN_POINT('Ctrl Pts',(1.28715662605536,4.52994106929151,18.0933583452606));
#39969=CARTESIAN_POINT('Ctrl Pts',(-1.03650075501039,4.59406889295398,18.172730235314));
#39970=CARTESIAN_POINT('Ctrl Pts',(-3.10708740551261,3.53832597274458,18.2521021253674));
#39971=CARTESIAN_POINT('Ctrl Pts',(-4.42189226956141,1.62210042840545,18.3314740154208));
#39972=CARTESIAN_POINT('Ctrl Pts',(-4.65746145505438,-0.691994213306935,
18.4108459054742));
#39973=CARTESIAN_POINT('Ctrl Pts',(-3.7623932789572,-2.83237457985889,18.4902177955276));
#39974=CARTESIAN_POINT('Ctrl Pts',(-1.94345928697736,-4.29245481019949,
18.569589685581));
#39975=CARTESIAN_POINT('Ctrl Pts',(0.335233909124166,-4.68912434583344,
18.6489615756345));
#39976=CARTESIAN_POINT('Ctrl Pts',(3.29668819545067,-3.73492805813089,18.7547907623723));
#39977=CARTESIAN_POINT('Ctrl Pts',(5.339103029404,-0.0175478502153651,18.8870772457947));
#39978=CARTESIAN_POINT('Ctrl Pts',(2.90621803008022,4.48249178265512,19.0458210259014));
#39979=CARTESIAN_POINT('Ctrl Pts',(-2.18656320946377,4.86959394496076,19.2045648060083));
#39980=CARTESIAN_POINT('Ctrl Pts',(-5.27828887711238,0.806568563691633,
19.363308586115));
#39981=CARTESIAN_POINT('Ctrl Pts',(-3.54020456892039,-3.99752392897296,
19.5220523662219));
#39982=CARTESIAN_POINT('Ctrl Pts',(1.43734916996113,-5.14215993940115,19.6807961463287));
#39983=CARTESIAN_POINT('Ctrl Pts',(5.09974667860479,-1.58211192901293,19.8395399264355));
#39984=CARTESIAN_POINT('Ctrl Pts',(4.09539160933933,3.42571876325583,19.9982837065423));
#39985=CARTESIAN_POINT('Ctrl Pts',(-0.656009676029552,5.29932988758688,
20.1570274866491));
#39986=CARTESIAN_POINT('Ctrl Pts',(-4.80798654830356,2.32253130646633,20.3157712667559));
#39987=CARTESIAN_POINT('Ctrl Pts',(-4.5587807483591,-2.77696271962182,20.4745150468627));
#39988=CARTESIAN_POINT('Ctrl Pts',(-0.141143605831918,-5.34031031892967,
20.6332588269695));
#39989=CARTESIAN_POINT('Ctrl Pts',(4.41154214902265,-3.00742829557661,20.7920026070763));
#39990=CARTESIAN_POINT('Ctrl Pts',(4.83176599740626,1.2132097937891,20.9242890904987));
#39991=CARTESIAN_POINT('Ctrl Pts',(2.93038174053082,3.67602118591258,21.0301182772365));
#39992=CARTESIAN_POINT('Ctrl Pts',(0.82729199276626,4.63872722375956,21.1094901672899));
#39993=CARTESIAN_POINT('Ctrl Pts',(-1.49865065220701,4.46452630956661,21.1888620573433));
#39994=CARTESIAN_POINT('Ctrl Pts',(-3.44799414715959,3.20657754587673,21.2682339473967));
#39995=CARTESIAN_POINT('Ctrl Pts',(-4.56354990278301,1.16548416044547,21.3476058374502));
#39996=CARTESIAN_POINT('Ctrl Pts',(-4.56418179760212,-1.1584417781363,21.4269777275035));
#39997=CARTESIAN_POINT('Ctrl Pts',(-3.45471245456607,-3.20074439226419,
21.506349617557));
#39998=CARTESIAN_POINT('Ctrl Pts',(-1.50277006074114,-4.46305057284728,
21.5857215076104));
#39999=CARTESIAN_POINT('Ctrl Pts',(0.814760394348267,-4.63832755437973,
21.6650933976638));
#40000=CARTESIAN_POINT('Ctrl Pts',(2.93407303175,-3.6836334512587,21.7444652877172));
#40001=CARTESIAN_POINT('Ctrl Pts',(4.33851638857388,-1.83165928184362,21.8238371777706));
#40002=CARTESIAN_POINT('Ctrl Pts',(4.68617856238765,0.466526807638465,21.903209067824));
#40003=CARTESIAN_POINT('Ctrl Pts',(3.89225998228531,2.65105540897445,21.9825809578774));
#40004=CARTESIAN_POINT('Ctrl Pts',(2.1502156260726,4.18979944864558,22.0619528479308));
#40005=CARTESIAN_POINT('Ctrl Pts',(-0.115627163561327,4.70791408521783,
22.1413247379842));
#40006=CARTESIAN_POINT('Ctrl Pts',(-2.35329778315663,4.07919314165102,22.2206966280376));
#40007=CARTESIAN_POINT('Ctrl Pts',(-4.01771326340777,2.45678878743819,22.300068518091));
#40008=CARTESIAN_POINT('Ctrl Pts',(-4.7034211013359,0.235916647177708,22.3794404081444));
#40009=CARTESIAN_POINT('Ctrl Pts',(-4.24338680893675,-2.04242454395301,
22.4588122981978));
#40010=CARTESIAN_POINT('Ctrl Pts',(-2.74967243806091,-3.82323548987737,
22.5381841882512));
#40011=CARTESIAN_POINT('Ctrl Pts',(-0.586144182924564,-4.67271481097619,
22.6175560783046));
#40012=CARTESIAN_POINT('Ctrl Pts',(1.7201676224087,-4.38393110573301,22.696927968358));
#40013=CARTESIAN_POINT('Ctrl Pts',(3.60745033643733,-3.02723150865538,22.7762998584114));
#40014=CARTESIAN_POINT('Ctrl Pts',(4.61596616842609,-0.933105005158016,
22.8556717484649));
#40015=CARTESIAN_POINT('Ctrl Pts',(4.50004284053894,1.38832380607303,22.9350436385182));
#40016=CARTESIAN_POINT('Ctrl Pts',(3.28791904717806,3.37156001439376,23.0144155285717));
#40017=CARTESIAN_POINT('Ctrl Pts',(1.27486544641681,4.53349166431032,23.093787418625));
#40018=CARTESIAN_POINT('Ctrl Pts',(-1.04874255247445,4.59107478042505,23.1731593086785));
#40019=CARTESIAN_POINT('Ctrl Pts',(-3.11687918839179,3.53028224171763,23.2525311987318));
#40020=CARTESIAN_POINT('Ctrl Pts',(-4.42575095234051,1.60952076333037,23.3319030887853));
#40021=CARTESIAN_POINT('Ctrl Pts',(-4.6565195809412,-0.703316410525592,
23.4112749788386));
#40022=CARTESIAN_POINT('Ctrl Pts',(-3.75297034643954,-2.84482726347037,
23.4906468688921));
#40023=CARTESIAN_POINT('Ctrl Pts',(-1.93520584271877,-4.29334449199004,
23.5700187589454));
#40024=CARTESIAN_POINT('Ctrl Pts',(0.353970520843478,-4.69601250539774,
23.6493906489989));
#40025=CARTESIAN_POINT('Ctrl Pts',(2.55692044899663,-3.95474226694855,23.7287625390522));
#40026=CARTESIAN_POINT('Ctrl Pts',(4.13701021543862,-2.25010556593857,23.8081344291057));
#40027=CARTESIAN_POINT('Ctrl Pts',(4.70933345050753,0.00265187040687223,
23.887506319159));
#40028=CARTESIAN_POINT('Ctrl Pts',(4.13447348097035,2.25476331699259,23.9668782092125));
#40029=CARTESIAN_POINT('Ctrl Pts',(2.55246492296808,3.95761941039203,24.0462500992659));
#40030=CARTESIAN_POINT('Ctrl Pts',(0.348681559517371,4.69640817546236,24.1256219893193));
#40031=CARTESIAN_POINT('Ctrl Pts',(-1.94003986003887,4.29116230431301,24.2049938793727));
#40032=CARTESIAN_POINT('Ctrl Pts',(-3.75617186389469,2.84059879415982,24.2843657694261));
#40033=CARTESIAN_POINT('Ctrl Pts',(-4.65730871585138,0.698071705307978,
24.3637376594795));
#40034=CARTESIAN_POINT('Ctrl Pts',(-4.42393547340455,-1.61450410580135,
24.4431095495329));
#40035=CARTESIAN_POINT('Ctrl Pts',(-3.11290134185147,-3.5337902903817,24.5224814395863));
#40036=CARTESIAN_POINT('Ctrl Pts',(-1.0435713337136,-4.59225298213718,24.6018533296397));
#40037=CARTESIAN_POINT('Ctrl Pts',(1.27997034141094,-4.5320530122236,24.6812252196931));
#40038=CARTESIAN_POINT('Ctrl Pts',(3.29171407453406,-3.36785496006151,24.7605971097465));
#40039=CARTESIAN_POINT('Ctrl Pts',(4.50160354518617,-1.38325489424899,24.8399689997999));
#40040=CARTESIAN_POINT('Ctrl Pts',(4.61491235636141,0.938303002019797,24.9193408898533));
#40041=CARTESIAN_POINT('Ctrl Pts',(3.60403873246226,3.03129236389504,24.9987127799067));
#40042=CARTESIAN_POINT('Ctrl Pts',(1.71522925073975,4.3858656155773,25.0780846699601));
#40043=CARTESIAN_POINT('Ctrl Pts',(-0.591406279867446,4.67205171125385,
25.1574565600135));
#40044=CARTESIAN_POINT('Ctrl Pts',(-2.75397654975454,3.82013635147998,25.2368284500669));
#40045=CARTESIAN_POINT('Ctrl Pts',(-4.2456842279451,2.03764423221396,25.3162003401203));
#40046=CARTESIAN_POINT('Ctrl Pts',(-4.70315262587087,-0.24121351177037,
25.3955722301737));
#40047=CARTESIAN_POINT('Ctrl Pts',(-4.01494345438624,-2.4613121782045,25.4749441202271));
#40048=CARTESIAN_POINT('Ctrl Pts',(-2.34870294433969,-4.08184064605008,
25.5543160102806));
#40049=CARTESIAN_POINT('Ctrl Pts',(-0.110323595817837,-4.70804176751889,
25.6336879003339));
#40050=CARTESIAN_POINT('Ctrl Pts',(2.15493033644811,-4.1873743354938,25.7130597903874));
#40051=CARTESIAN_POINT('Ctrl Pts',(3.89524800861274,-2.64667178393831,25.7924316804407));
#40052=CARTESIAN_POINT('Ctrl Pts',(4.68669188786451,-0.461245844124039,
25.8718035704942));
#40053=CARTESIAN_POINT('Ctrl Pts',(4.33646799704899,1.83653856236848,25.9511754605475));
#40054=CARTESIAN_POINT('Ctrl Pts',(2.92989010076147,3.68694624017715,26.030547350601));
#40055=CARTESIAN_POINT('Ctrl Pts',(0.809597461130217,4.63922197479579,26.1099192406544));
#40056=CARTESIAN_POINT('Ctrl Pts',(-1.50791132801882,4.46139350509784,26.1892911307078));
#40057=CARTESIAN_POINT('Ctrl Pts',(-3.45809625536759,3.19677945268506,26.2686630207611));
#40058=CARTESIAN_POINT('Ctrl Pts',(-4.56589658927499,1.15343700154949,26.3480349108146));
#40059=CARTESIAN_POINT('Ctrl Pts',(-4.56145462047572,-1.170880150074,26.427406800868));
#40060=CARTESIAN_POINT('Ctrl Pts',(-3.44585240273711,-3.20997348883872,
26.5067786909214));
#40061=CARTESIAN_POINT('Ctrl Pts',(-1.49084816695666,-4.46712439087817,
26.5861505809748));
#40062=CARTESIAN_POINT('Ctrl Pts',(0.827323382358012,-4.6360936791118,26.6655224710282));
#40063=CARTESIAN_POINT('Ctrl Pts',(2.9439607869795,-3.67572080893307,26.7448943610816));
#40064=CARTESIAN_POINT('Ctrl Pts',(4.34345586023946,-1.81995048576826,26.824266251135));
#40065=CARTESIAN_POINT('Ctrl Pts',(4.68489470002155,0.479155747337646,26.9036381411885));
#40066=CARTESIAN_POINT('Ctrl Pts',(3.88510356071688,2.66154070098535,26.9830100312418));
#40067=CARTESIAN_POINT('Ctrl Pts',(2.13890979355249,4.1955802310934,27.0623819212952));
#40068=CARTESIAN_POINT('Ctrl Pts',(-0.128317664924755,4.70758570366646,
27.1417538113486));
#40069=CARTESIAN_POINT('Ctrl Pts',(-2.36428722425266,4.07283371889059,27.221125701402));
#40070=CARTESIAN_POINT('Ctrl Pts',(-4.02432164901364,2.44594845525754,27.3004975914554));
#40071=CARTESIAN_POINT('Ctrl Pts',(-4.70404022775981,0.223235561938782,
27.3798694815088));
#40072=CARTESIAN_POINT('Ctrl Pts',(-4.2378650192401,-2.05385702014473,27.4592413715622));
#40073=CARTESIAN_POINT('Ctrl Pts',(-2.73935527238859,-3.83063457825638,
27.5386132616157));
#40074=CARTESIAN_POINT('Ctrl Pts',(-0.573544644643281,-4.67427803207058,
27.617985151669));
#40075=CARTESIAN_POINT('Ctrl Pts',(1.73198018901762,-4.37927770361132,27.6973570417225));
#40076=CARTESIAN_POINT('Ctrl Pts',(3.61559848230692,-3.01749501991908,27.7767289317758));
#40077=CARTESIAN_POINT('Ctrl Pts',(4.61846498829774,-0.920657228486544,
27.8561008218292));
#40078=CARTESIAN_POINT('Ctrl Pts',(4.49628364593812,1.4004506259651,27.9354727118827));
#40079=CARTESIAN_POINT('Ctrl Pts',(3.278817559783,3.38041180777658,28.014844601936));
#40080=CARTESIAN_POINT('Ctrl Pts',(1.2626387736043,4.53691215562828,28.0942164919895));
#40081=CARTESIAN_POINT('Ctrl Pts',(-1.0611160230209,4.58823074465364,28.1735883820429));
#40082=CARTESIAN_POINT('Ctrl Pts',(-3.12638530517863,3.52186648015787,28.2529602720962));
#40083=CARTESIAN_POINT('Ctrl Pts',(-4.43007404713138,1.59758333661492,28.3323321621497));
#40084=CARTESIAN_POINT('Ctrl Pts',(-4.65460655700551,-0.715867571536754,
28.4117040522031));
#40085=CARTESIAN_POINT('Ctrl Pts',(-3.74528721238995,-2.85493472380806,
28.4910759422565));
#40086=CARTESIAN_POINT('Ctrl Pts',(-1.9236241928888,-4.29854609665053,28.5704478323099));
#40087=CARTESIAN_POINT('Ctrl Pts',(0.366629422130075,-4.69504115501931,
28.6498197223633));
#40088=CARTESIAN_POINT('Ctrl Pts',(2.56757292143854,-3.94783458032276,28.7291916124167));
#40089=CARTESIAN_POINT('Ctrl Pts',(4.14306134031087,-2.23894424024318,28.8085635024701));
#40090=CARTESIAN_POINT('Ctrl Pts',(4.70930918719419,0.0153479609406268,
28.8879353925235));
#40091=CARTESIAN_POINT('Ctrl Pts',(4.12837973995606,2.26590143281143,28.9673072825769));
#40092=CARTESIAN_POINT('Ctrl Pts',(2.54178612607819,3.96448633113712,29.0466791726303));
#40093=CARTESIAN_POINT('Ctrl Pts',(0.336019038035816,4.69733113443944,29.1260510626837));
#40094=CARTESIAN_POINT('Ctrl Pts',(-1.95160154390656,4.2859164707584,29.2054229527371));
#40095=CARTESIAN_POINT('Ctrl Pts',(-3.76381630954999,2.83046204151583,29.2847948427905));
#40096=CARTESIAN_POINT('Ctrl Pts',(-4.65917375325318,0.68551332408149,29.364166732844));
#40097=CARTESIAN_POINT('Ctrl Pts',(-4.41956678357008,-1.62642492174114,
29.4435386228973));
#40098=CARTESIAN_POINT('Ctrl Pts',(-3.10336312795443,-3.54216965665813,
29.5229105129507));
#40099=CARTESIAN_POINT('Ctrl Pts',(-1.03118708354684,-4.59504970367272,
29.6022824030041));
#40100=CARTESIAN_POINT('Ctrl Pts',(1.29218385191882,-4.52858581384264,29.6816542930575));
#40101=CARTESIAN_POINT('Ctrl Pts',(3.30078166125751,-3.3589684436152,29.761026183111));
#40102=CARTESIAN_POINT('Ctrl Pts',(4.50531636407018,-1.37111379547362,29.8403980731643));
#40103=CARTESIAN_POINT('Ctrl Pts',(4.61236597294397,0.950741138336453,29.9197699632178));
#40104=CARTESIAN_POINT('Ctrl Pts',(3.59585344010749,3.04099763527755,29.9991418532711));
#40105=CARTESIAN_POINT('Ctrl Pts',(1.70339896854746,4.39047383939912,30.0785137433246));
#40106=CARTESIAN_POINT('Ctrl Pts',(-0.603999721341074,4.67044033439209,
30.157885633378));
#40107=CARTESIAN_POINT('Ctrl Pts',(-2.76426541604165,3.81269790177148,30.2372575234314));
#40108=CARTESIAN_POINT('Ctrl Pts',(-4.25116217399222,2.02619069954299,30.3166294134847));
#40109=CARTESIAN_POINT('Ctrl Pts',(-4.70248523614609,-0.253892072197153,
30.3960013035382));
#40110=CARTESIAN_POINT('Ctrl Pts',(-4.00829330354932,-2.47212729713062,
30.4753731935915));
#40111=CARTESIAN_POINT('Ctrl Pts',(-2.33768999441463,-4.08815778444404,
30.554745083645));
#40112=CARTESIAN_POINT('Ctrl Pts',(-0.0976305770295779,-4.70832208445062,
30.6341169736984));
#40113=CARTESIAN_POINT('Ctrl Pts',(2.16621143281822,-4.18154954637921,30.7134888637517));
#40114=CARTESIAN_POINT('Ctrl Pts',(3.90236913245919,-2.63616079451278,30.7928607538052));
#40115=CARTESIAN_POINT('Ctrl Pts',(4.68791834918069,-0.448609108145992,
30.8722326438586));
#40116=CARTESIAN_POINT('Ctrl Pts',(4.33150103257305,1.84822276398574,30.951604533912));
#40117=CARTESIAN_POINT('Ctrl Pts',(2.91993965204555,3.69483166178228,31.0309764239654));
#40118=CARTESIAN_POINT('Ctrl Pts',(0.797087435456495,4.64138774513982,31.1103483140188));
#40119=CARTESIAN_POINT('Ctrl Pts',(-1.51993351608663,4.45731204731877,31.1897202040722));
#40120=CARTESIAN_POINT('Ctrl Pts',(-3.46670202742684,3.18744500086376,31.2690920941256));
#40121=CARTESIAN_POINT('Ctrl Pts',(-4.56898959830062,1.14112340748814,31.348463984179));
#40122=CARTESIAN_POINT('Ctrl Pts',(-4.5582814163153,-1.18317332211776,31.4278358742324));
#40123=CARTESIAN_POINT('Ctrl Pts',(-3.43718597090036,-3.21925164936547,
31.5072077642858));
#40124=CARTESIAN_POINT('Ctrl Pts',(-1.47879963105622,-4.47112740052042,
31.5865796543392));
#40125=CARTESIAN_POINT('Ctrl Pts',(0.839819025645787,-4.63384641358128,
31.6659515443926));
#40126=CARTESIAN_POINT('Ctrl Pts',(2.95385962660838,-3.66777069713875,31.745323434446));
#40127=CARTESIAN_POINT('Ctrl Pts',(4.34834656078651,-1.80823415734596,31.8246953244994));
#40128=CARTESIAN_POINT('Ctrl Pts',(4.68358589765892,0.491784220717852,31.9040672145528));
#40129=CARTESIAN_POINT('Ctrl Pts',(3.87791407680318,2.67200505116071,31.9834391046062));
#40130=CARTESIAN_POINT('Ctrl Pts',(2.12759097045539,4.20133136552371,32.0628109946597));
#40131=CARTESIAN_POINT('Ctrl Pts',(-0.141008586952624,4.70722265873437,
32.142182884713));
#40132=CARTESIAN_POINT('Ctrl Pts',(-2.37525876469618,4.06644493153793,32.2215547747665));
#40133=CARTESIAN_POINT('Ctrl Pts',(-4.03090116490581,2.43509021994207,32.3009266648198));
#40134=CARTESIAN_POINT('Ctrl Pts',(-4.7046249635928,0.21055292074912,32.3802985548733));
#40135=CARTESIAN_POINT('Ctrl Pts',(-4.23231253465933,-2.06527460388738,
32.4596704449267));
#40136=CARTESIAN_POINT('Ctrl Pts',(-2.72901814034772,-3.83800580642471,
32.5390423349801));
#40137=CARTESIAN_POINT('Ctrl Pts',(-0.560940967626579,-4.67580728979871,
32.6184142250335));
#40138=CARTESIAN_POINT('Ctrl Pts',(1.74378018318661,-4.37459246710163,32.6977861150869));
#40139=CARTESIAN_POINT('Ctrl Pts',(3.62372034116752,-3.00773660241476,32.7771580051403));
#40140=CARTESIAN_POINT('Ctrl Pts',(4.62093024500891,-0.90820275889168,32.8565298951936));
#40141=CARTESIAN_POINT('Ctrl Pts',(4.49249176942175,1.41256726642465,32.9359017852471));
#40142=CARTESIAN_POINT('Ctrl Pts',(3.26969224276534,3.38923903230456,33.0152736753005));
#40143=CARTESIAN_POINT('Ctrl Pts',(1.25040292311233,4.54029967186844,33.0946455653539));
#40144=CARTESIAN_POINT('Ctrl Pts',(-1.0734817808909,4.58535336114807,33.1740174554073));
#40145=CARTESIAN_POINT('Ctrl Pts',(-3.13586869918079,3.51342512115953,33.2533893454607));
#40146=CARTESIAN_POINT('Ctrl Pts',(-4.43436494347784,1.58563429849111,33.3327612355141));
#40147=CARTESIAN_POINT('Ctrl Pts',(-4.65265970284399,-0.728413529547759,
33.4121331255675));
#40148=CARTESIAN_POINT('Ctrl Pts',(-3.73757685708491,-2.8650214341048,33.4915050156209));
#40149=CARTESIAN_POINT('Ctrl Pts',(-1.91202856192598,-4.30371645893127,
33.5708769056743));
#40150=CARTESIAN_POINT('Ctrl Pts',(0.379285658714694,-4.69403568047687,
33.6502487957277));
#40151=CARTESIAN_POINT('Ctrl Pts',(2.57820673242699,-3.94089820033005,33.7296206857811));
#40152=CARTESIAN_POINT('Ctrl Pts',(4.14908235288389,-2.22776664161308,33.8089925758346));
#40153=CARTESIAN_POINT('Ctrl Pts',(4.70925069601633,0.0280439399230538,
33.8883644658879));
#40154=CARTESIAN_POINT('Ctrl Pts',(4.12225599334877,2.27702307976815,33.9677363559414));
#40155=CARTESIAN_POINT('Ctrl Pts',(2.53108885516031,3.9713244374868,34.0471082459947));
#40156=CARTESIAN_POINT('Ctrl Pts',(0.323354074324944,4.69821995261122,34.1264801360482));
#40157=CARTESIAN_POINT('Ctrl Pts',(-1.96314904328387,4.28063948661298,34.2058520261016));
#40158=CARTESIAN_POINT('Ctrl Pts',(-3.77143339930544,2.8203047167106,34.2852239161549));
#40159=CARTESIAN_POINT('Ctrl Pts',(-4.66100492718239,0.672949960456159,
34.3645958062084));
#40160=CARTESIAN_POINT('Ctrl Pts',(-4.41516597175719,-1.63833391661592,
34.4439676962618));
#40161=CARTESIAN_POINT('Ctrl Pts',(-3.09380235841604,-3.55052327799099,
34.5233395863151));
#40162=CARTESIAN_POINT('Ctrl Pts',(-1.01879533858015,-4.59781302779744,
34.6027114763686));
#40163=CARTESIAN_POINT('Ctrl Pts',(1.30438797066869,-4.52508570111899,34.6820833664219));
#40164=CARTESIAN_POINT('Ctrl Pts',(3.30982525747642,-3.35005751375522,34.7614552564754));
#40165=CARTESIAN_POINT('Ctrl Pts',(4.50899643773683,-1.3589627312672,34.8408271465288));
#40166=CARTESIAN_POINT('Ctrl Pts',(4.60978606625886,0.963172364544519,34.9201990365822));
#40167=CARTESIAN_POINT('Ctrl Pts',(3.58764201262861,3.05068080429907,34.9995709266356));
#40168=CARTESIAN_POINT('Ctrl Pts',(1.69155630583291,4.39505015269376,35.078942816689));
#40169=CARTESIAN_POINT('Ctrl Pts',(-0.616588772867267,4.66879501217076,
35.1583147067424));
#40170=CARTESIAN_POINT('Ctrl Pts',(-2.77453419129308,3.80523174088547,35.2376865967958));
#40171=CARTESIAN_POINT('Ctrl Pts',(-4.2566092220472,2.01472244025804,35.3170584868492));
#40172=CARTESIAN_POINT('Ctrl Pts',(-4.70178366815532,-0.266568787303772,
35.3964303769026));
#40173=CARTESIAN_POINT('Ctrl Pts',(-4.00161401992238,-2.48292444831838,
35.475802266956));
#40174=CARTESIAN_POINT('Ctrl Pts',(-2.3266600538588,-4.09444520958265,35.5551741570094));
#40175=CARTESIAN_POINT('Ctrl Pts',(-0.0849368486498902,-4.70856818069336,
35.6345460470628));
#40176=CARTESIAN_POINT('Ctrl Pts',(2.17747678488564,-4.17569436522607,35.7139179371162));
#40177=CARTESIAN_POINT('Ctrl Pts',(3.90946189338614,-2.62563064513239,35.7932898271696));
#40178=CARTESIAN_POINT('Ctrl Pts',(4.68911073810487,-0.435969111619298,
35.872661717223));
#40179=CARTESIAN_POINT('Ctrl Pts',(4.32650258619184,1.85989353248294,35.9520336072764));
#40180=CARTESIAN_POINT('Ctrl Pts',(2.90996798083354,3.70269022887686,36.0314054973299));
#40181=CARTESIAN_POINT('Ctrl Pts',(0.784571616449035,4.64351978128221,36.1107773873832));
#40182=CARTESIAN_POINT('Ctrl Pts',(-1.53194465708265,4.4531981932239,36.1901492774366));
#40183=CARTESIAN_POINT('Ctrl Pts',(-3.47528260305097,3.17808738228323,36.2695211674901));
#40184=CARTESIAN_POINT('Ctrl Pts',(-4.57204939932363,1.12880151959547,36.3488930575434));
#40185=CARTESIAN_POINT('Ctrl Pts',(-4.55507508198074,-1.19545789470598,
36.4282649475969));
#40186=CARTESIAN_POINT('Ctrl Pts',(-3.42849455715498,-3.2285064119582,36.5076368376502));
#40187=CARTESIAN_POINT('Ctrl Pts',(-1.4667403470503,-4.47509791343512,36.5870087277037));
#40188=CARTESIAN_POINT('Ctrl Pts',(0.852308565021146,-4.63156546866048,
36.6663806177571));
#40189=CARTESIAN_POINT('Ctrl Pts',(2.96373699720644,-3.65979392751645,36.7457525078104));
#40190=CARTESIAN_POINT('Ctrl Pts',(4.35320565699285,-1.79650468644589,36.8251243978639));
#40191=CARTESIAN_POINT('Ctrl Pts',(4.68224305439311,0.504409119747259,36.9044962879172));
#40192=CARTESIAN_POINT('Ctrl Pts',(3.87069640771237,2.68244998086059,36.9838681779707));
#40193=CARTESIAN_POINT('Ctrl Pts',(2.1162566837541,4.20705196413867,37.0632400680241));
#40194=CARTESIAN_POINT('Ctrl Pts',(-0.153698484112011,4.70682540110399,
37.1426119580775));
#40195=CARTESIAN_POINT('Ctrl Pts',(-2.38621304145417,4.06002658874194,37.2219838481309));
#40196=CARTESIAN_POINT('Ctrl Pts',(-4.03745138369124,2.42421428607825,37.3013557381843));
#40197=CARTESIAN_POINT('Ctrl Pts',(-4.7051755056078,0.197868749234187,37.3807276282377));
#40198=CARTESIAN_POINT('Ctrl Pts',(-4.22672928908836,-2.07667717695002,
37.4600995182911));
#40199=CARTESIAN_POINT('Ctrl Pts',(-2.71866117345227,-3.84534913947293,
37.5394714083445));
#40200=CARTESIAN_POINT('Ctrl Pts',(-0.548333213620079,-4.67730256316236,
37.6188432983979));
#40201=CARTESIAN_POINT('Ctrl Pts',(1.75556750333961,-4.36987543548734,37.6982151884513));
#40202=CARTESIAN_POINT('Ctrl Pts',(3.63181586235974,-2.99795632430491,37.7775870785047));
#40203=CARTESIAN_POINT('Ctrl Pts',(4.62336191621364,-0.895741688343936,
37.8569589685581));
#40204=CARTESIAN_POINT('Ctrl Pts',(4.48866724088475,1.42467364012841,37.9363308586115));
#40205=CARTESIAN_POINT('Ctrl Pts',(3.26054316123161,3.3980416234756,38.0157027486649));
#40206=CARTESIAN_POINT('Ctrl Pts',(1.23815798448111,4.54365418850126,38.0950746387183));
#40207=CARTESIAN_POINT('Ctrl Pts',(-1.08583973646279,4.58244265094544,38.1744465287717));
#40208=CARTESIAN_POINT('Ctrl Pts',(-3.1453293014664,3.50495822568428,38.2538184188251));
#40209=CARTESIAN_POINT('Ctrl Pts',(-4.43862360995231,1.57367373662757,38.3331903088785));
#40210=CARTESIAN_POINT('Ctrl Pts',(-4.65067903319431,-0.740954194968168,
38.412562198932));
#40211=CARTESIAN_POINT('Ctrl Pts',(-3.72983933538423,-2.87508731801368,
38.4919340889853));
#40212=CARTESIAN_POINT('Ctrl Pts',(-1.9004190363744,-4.30885554699714,38.5713059790388));
#40213=CARTESIAN_POINT('Ctrl Pts',(0.391939142907767,-4.69299607822647,
38.6506778690921));
#40214=CARTESIAN_POINT('Ctrl Pts',(2.588821796549,-3.93393319787887,38.7300497591456));
#40215=CARTESIAN_POINT('Ctrl Pts',(4.15507322474385,-2.21657281258971,38.8094216491989));
#40216=CARTESIAN_POINT('Ctrl Pts',(4.70915794841682,0.040739642006525,38.8887935392524));
#40217=CARTESIAN_POINT('Ctrl Pts',(4.11610234038245,2.28812831500406,38.9681654293058));
#40218=CARTESIAN_POINT('Ctrl Pts',(2.52037308462918,3.97813341921603,39.0475373193591));
#40219=CARTESIAN_POINT('Ctrl Pts',(0.310686955552019,4.69907511544173,39.1269092094126));
#40220=CARTESIAN_POINT('Ctrl Pts',(-1.97468264266246,4.27533046137757,39.2062810994659));
#40221=CARTESIAN_POINT('Ctrl Pts',(-3.77902238214566,2.81012864743349,39.2856529895194));
#40222=CARTESIAN_POINT('Ctrl Pts',(-4.66280353786911,0.660378394081937,
39.3650248795728));
#40223=CARTESIAN_POINT('Ctrl Pts',(-4.41073058968569,-1.65022475069991,
39.4443967696262));
#40224=CARTESIAN_POINT('Ctrl Pts',(-3.0842237862698,-3.55886290155649,39.5237686596796));
#40225=CARTESIAN_POINT('Ctrl Pts',(-1.00638734295308,-4.60052063353569,
39.603140549733));
#40226=CARTESIAN_POINT('Ctrl Pts',(1.3165658861068,-4.521594850557,39.6825124397864));
#40227=CARTESIAN_POINT('Ctrl Pts',(3.31887653668104,-3.34104229843822,39.7618843298398));
#40228=CARTESIAN_POINT('Ctrl Pts',(4.51258247789865,-1.34695556252384,39.8412562198932));
#40229=CARTESIAN_POINT('Ctrl Pts',(4.60729903172253,0.975909964327458,39.9206281099466));
#40230=CARTESIAN_POINT('Ctrl Pts',(3.92183073605334,2.36502208507764,39.9735427033156));
#40231=CARTESIAN_POINT('Ctrl Pts',(3.43378788736169,2.9358415841302,40.));
#40232=CARTESIAN_POINT('Ctrl Pts',(4.5177656910975,-0.000116631996953637,
0.887416697508071));
#40233=CARTESIAN_POINT('Ctrl Pts',(4.51716522512143,0.582848551743655,0.907954496247182));
#40234=CARTESIAN_POINT('Ctrl Pts',(4.40381632429852,1.16604045169665,0.928492294986294));
#40235=CARTESIAN_POINT('Ctrl Pts',(4.18378127438632,1.70573618195762,0.949030093725405));
#40236=CARTESIAN_POINT('Ctrl Pts',(3.90032671966707,2.40098547504095,0.975487390409873));
#40237=CARTESIAN_POINT('Ctrl Pts',(3.43982409908107,3.02405189544283,1.00194468709434));
#40238=CARTESIAN_POINT('Ctrl Pts',(2.85836212737567,3.49904666560206,1.02840198377881));
#40239=CARTESIAN_POINT('Ctrl Pts',(2.27690015567027,3.97404143576128,1.05485928046328));
#40240=CARTESIAN_POINT('Ctrl Pts',(1.57447883284546,4.30096455567785,1.08131657714775));
#40241=CARTESIAN_POINT('Ctrl Pts',(0.83665229586908,4.43999713904637,1.10777387383221));
#40242=CARTESIAN_POINT('Ctrl Pts',(0.0988257588927,4.57902972241489,1.13423117051668));
#40243=CARTESIAN_POINT('Ctrl Pts',(-0.674405992235245,4.53017176923536,
1.16068846720115));
#40244=CARTESIAN_POINT('Ctrl Pts',(-1.38886418452507,4.29937413054889,1.18714576388562));
#40245=CARTESIAN_POINT('Ctrl Pts',(-2.1033223768149,4.06857649186242,1.21360306057009));
#40246=CARTESIAN_POINT('Ctrl Pts',(-2.7590070102666,3.65583916766901,1.24006035725455));
#40247=CARTESIAN_POINT('Ctrl Pts',(-3.27605642296673,3.11143310386793,1.26651765393902));
#40248=CARTESIAN_POINT('Ctrl Pts',(-3.79310583566684,2.56702704006687,1.29297495062349));
#40249=CARTESIAN_POINT('Ctrl Pts',(-4.17152002761538,1.89095223665816,1.31943224730795));
#40250=CARTESIAN_POINT('Ctrl Pts',(-4.36520856862574,1.16555385826357,1.34588954399242));
#40251=CARTESIAN_POINT('Ctrl Pts',(-4.5588971096361,0.440155479868968,1.37234684067689));
#40252=CARTESIAN_POINT('Ctrl Pts',(-4.56785999970828,-0.334566473511511,
1.39880413736136));
#40253=CARTESIAN_POINT('Ctrl Pts',(-4.39100556896818,-1.06425172631823,
1.42526143404583));
#40254=CARTESIAN_POINT('Ctrl Pts',(-4.21415113822807,-1.79393697912495,
1.4517187307303));
#40255=CARTESIAN_POINT('Ctrl Pts',(-3.85147938667567,-2.4785855313579,1.47817602741476));
#40256=CARTESIAN_POINT('Ctrl Pts',(-3.3471633321549,-3.03480794657228,1.50463332409923));
#40257=CARTESIAN_POINT('Ctrl Pts',(-2.84284727763412,-3.59103036178665,
1.5310906207837));
#40258=CARTESIAN_POINT('Ctrl Pts',(-2.19688692014498,-4.01882663998244,
1.55754791746817));
#40259=CARTESIAN_POINT('Ctrl Pts',(-1.48795951638605,-4.26609166819824,
1.58400521415264));
#40260=CARTESIAN_POINT('Ctrl Pts',(-0.779032112627116,-4.51335669641404,
1.6104625108371));
#40261=CARTESIAN_POINT('Ctrl Pts',(-0.0071376625983989,-4.58009047464984,
1.63691980752157));
#40262=CARTESIAN_POINT('Ctrl Pts',(0.733707943998554,-4.4581649024313,1.66337710420604));
#40263=CARTESIAN_POINT('Ctrl Pts',(1.47455355059551,-4.33623933021276,1.68983440089051));
#40264=CARTESIAN_POINT('Ctrl Pts',(2.18435031376069,-4.02565440753988,1.71629169757498));
#40265=CARTESIAN_POINT('Ctrl Pts',(2.77664577327776,-3.56423903433516,1.74274899425944));
#40266=CARTESIAN_POINT('Ctrl Pts',(3.36894123279483,-3.10282366113044,1.76920629094391));
#40267=CARTESIAN_POINT('Ctrl Pts',(3.84373538866378,-2.49057783739389,1.79566358762838));
#40268=CARTESIAN_POINT('Ctrl Pts',(4.14319883817832,-1.80207242682533,1.82212088431285));
#40269=CARTESIAN_POINT('Ctrl Pts',(4.38955443642782,-1.23566887208905,1.84388615537792));
#40270=CARTESIAN_POINT('Ctrl Pts',(4.51725253079926,-0.617655577060232,
1.865651426443));
#40271=CARTESIAN_POINT('Ctrl Pts',(4.51787557461174,0.000108094638884985,
1.88741669750807));
#40272=CARTESIAN_POINT('Ctrl Pts',(1.3130361863565,-4.90075024188322,0.));
#40273=CARTESIAN_POINT('Ctrl Pts',(1.45293783176837,-4.85499972547219,-2.12441198790355E-17));
#40274=CARTESIAN_POINT('Ctrl Pts',(1.59048961161953,-4.80314405262584,1.00940613638452E-17));
#40275=CARTESIAN_POINT('Ctrl Pts',(1.72536214292615,-4.74546564178603,1.90819582357449E-17));
#40276=CARTESIAN_POINT('Ctrl Pts',(1.86158804346972,-4.68720846085782,2.81600435471549E-17));
#40277=CARTESIAN_POINT('Ctrl Pts',(1.9950813260058,-4.62301070705921,2.02661125299078E-16));
#40278=CARTESIAN_POINT('Ctrl Pts',(2.12548189098024,-4.5531145507957,1.45716771982052E-16));
#40279=CARTESIAN_POINT('Ctrl Pts',(2.25528319940241,-4.4835396027235,8.90341067708004E-17));
#40280=CARTESIAN_POINT('Ctrl Pts',(2.38202075670042,-4.40831802172382,2.31151513749735E-16));
#40281=CARTESIAN_POINT('Ctrl Pts',(2.50530950004123,-4.32764726500609,1.45716771982052E-16));
#40282=CARTESIAN_POINT('Ctrl Pts',(2.62711997854446,-4.24794377212644,6.13064155008212E-17));
#40283=CARTESIAN_POINT('Ctrl Pts',(2.74556437761014,-4.16292050991704,2.71959880884896E-17));
#40284=CARTESIAN_POINT('Ctrl Pts',(2.86023373369319,-4.07273466802712,-6.93889390390723E-17));
#40285=CARTESIAN_POINT('Ctrl Pts',(2.90383704830196,-4.03844127202745,-1.06115603492979E-16));
#40286=CARTESIAN_POINT('Ctrl Pts',(2.94689409015111,-4.00340109988822,-3.37664978924697E-16));
#40287=CARTESIAN_POINT('Ctrl Pts',(2.98938067979849,-3.96762172921426,-3.7470027081099E-16));
#40288=CARTESIAN_POINT('Ctrl Pts',(3.0045493035191,-3.95484772651792,-3.87922664316067E-16));
#40289=CARTESIAN_POINT('Ctrl Pts',(3.0196457209465,-3.94197897848992,-6.77418652234536E-17));
#40290=CARTESIAN_POINT('Ctrl Pts',(3.03465663588118,-3.92902653262601,-5.55111512312578E-17));
#40291=CARTESIAN_POINT('Ctrl Pts',(3.14512636784121,-3.83370567916447,3.44982654016709E-17));
#40292=CARTESIAN_POINT('Ctrl Pts',(3.25112830521826,-3.73372148501147,-5.43481287766778E-16));
#40293=CARTESIAN_POINT('Ctrl Pts',(3.35231677944077,-3.62929621080565,-5.13478148889135E-16));
#40294=CARTESIAN_POINT('Ctrl Pts',(3.36921809466263,-3.61185425914028,-5.08466782607427E-16));
#40295=CARTESIAN_POINT('Ctrl Pts',(3.38598504383309,-3.59428832049142,-2.69772873285687E-16));
#40296=CARTESIAN_POINT('Ctrl Pts',(3.40261591802407,-3.57659932769537,-2.63677968348475E-16));
#40297=CARTESIAN_POINT('Ctrl Pts',(3.50230123740107,-3.4705716543402,-2.26333319460949E-16));
#40298=CARTESIAN_POINT('Ctrl Pts',(3.59710111637371,-3.36012540834712,3.61502860778476E-17));
#40299=CARTESIAN_POINT('Ctrl Pts',(3.68681562587056,-3.2456540248488,-6.93889390390723E-17));
#40300=CARTESIAN_POINT('Ctrl Pts',(3.77658274630639,-3.13111551233192,-1.74990055122844E-16));
#40301=CARTESIAN_POINT('Ctrl Pts',(3.86125888590103,-3.01254641429341,-2.14930374901985E-16));
#40302=CARTESIAN_POINT('Ctrl Pts',(3.94059800782458,-2.89031628889591,-9.71445146547012E-17));
#40303=CARTESIAN_POINT('Ctrl Pts',(4.01127293754548,-2.78143424794555,7.77859507059291E-18));
#40304=CARTESIAN_POINT('Ctrl Pts',(4.07771240145114,-2.66964644715424,3.21618427330635E-16));
#40305=CARTESIAN_POINT('Ctrl Pts',(4.13970845878657,-2.55520469810914,3.46944695195361E-16));
#40306=CARTESIAN_POINT('Ctrl Pts',(4.1548365715119,-2.52727892743195,3.53124743599032E-16));
#40307=CARTESIAN_POINT('Ctrl Pts',(4.16969994577116,-2.49919510449128,-5.38761705143296E-16));
#40308=CARTESIAN_POINT('Ctrl Pts',(4.18429524804614,-2.47095685207318,-5.41233724504764E-16));
#40309=CARTESIAN_POINT('Ctrl Pts',(4.1935591046312,-2.45303361104087,-5.42802752155488E-16));
#40310=CARTESIAN_POINT('Ctrl Pts',(4.20271084368267,-2.4350560800449,-1.54877819716967E-16));
#40311=CARTESIAN_POINT('Ctrl Pts',(4.21174771778014,-2.41702978670704,-1.66533453693773E-16));
#40312=CARTESIAN_POINT('Ctrl Pts',(4.27617843190164,-2.28850670005169,-2.49635288749205E-16));
#40313=CARTESIAN_POINT('Ctrl Pts',(4.33481139244535,-2.15743447779131,-2.0244448216388E-16));
#40314=CARTESIAN_POINT('Ctrl Pts',(4.38745860743762,-2.0241905870822,-2.77555756156289E-16));
#40315=CARTESIAN_POINT('Ctrl Pts',(4.43978289169495,-1.89176399596928,-3.52206307982929E-16));
#40316=CARTESIAN_POINT('Ctrl Pts',(4.48619490051256,-1.75719157307499,-5.94819252645897E-16));
#40317=CARTESIAN_POINT('Ctrl Pts',(4.52646203441684,-1.6208264292839,-5.55111512312578E-16));
#40318=CARTESIAN_POINT('Ctrl Pts',(4.54111387023209,-1.5712078072459,-5.40663220727154E-16));
#40319=CARTESIAN_POINT('Ctrl Pts',(4.55495165294679,-1.52135171714656,-2.34210881400015E-17));
#40320=CARTESIAN_POINT('Ctrl Pts',(4.56796247846719,-1.47127487515823,-2.77555756156289E-17));
#40321=CARTESIAN_POINT('Ctrl Pts',(4.60395075905375,-1.33276103239401,-1.11900177134892E-17));
#40322=CARTESIAN_POINT('Ctrl Pts',(4.63361579821919,-1.19255796729143,2.91143634808383E-16));
#40323=CARTESIAN_POINT('Ctrl Pts',(4.65692008513065,-1.05110298842804,2.77555756156289E-16));
#40324=CARTESIAN_POINT('Ctrl Pts',(4.67001847025983,-0.971596938805809,
2.69918566125548E-16));
#40325=CARTESIAN_POINT('Ctrl Pts',(4.68110649292123,-0.891695424459561,
-5.05694400348962E-17));
#40326=CARTESIAN_POINT('Ctrl Pts',(4.69017032387523,-0.811477248591749,
-5.55111512312578E-17));
#40327=CARTESIAN_POINT('Ctrl Pts',(4.69376322527145,-0.779678774244579,
-5.74700448985431E-17));
#40328=CARTESIAN_POINT('Ctrl Pts',(4.69703800287417,-0.74783055663592,9.2602246089847E-18));
#40329=CARTESIAN_POINT('Ctrl Pts',(4.69999357182281,-0.715937571621207,
0.));
#40330=CARTESIAN_POINT('Ctrl Pts',(4.7021844555123,-0.692296160477742,-6.86435519161465E-18));
#40331=CARTESIAN_POINT('Ctrl Pts',(4.70420012738525,-0.668626688781088,
-5.81512878434173E-17));
#40332=CARTESIAN_POINT('Ctrl Pts',(4.70603832259692,-0.644957088113592,
-5.55111512312578E-17));
#40333=CARTESIAN_POINT('Ctrl Pts',(4.7169850543804,-0.50400101974599,-3.97887365597508E-17));
#40334=CARTESIAN_POINT('Ctrl Pts',(4.72166050160268,-0.362862391559157,
3.85433575684503E-16));
#40335=CARTESIAN_POINT('Ctrl Pts',(4.72009704228143,-0.221963242879035,
3.88578058618805E-16));
#40336=CARTESIAN_POINT('Ctrl Pts',(4.71853510529174,-0.0812012869083159,
3.91719479787741E-16));
#40337=CARTESIAN_POINT('Ctrl Pts',(4.71074633224057,0.0593224521016401,
3.13145818824179E-16));
#40338=CARTESIAN_POINT('Ctrl Pts',(4.69671116060458,0.199185274316974,2.22044604925031E-16));
#40339=CARTESIAN_POINT('Ctrl Pts',(4.68289306772495,0.336884870581422,1.3235243244906E-16));
#40340=CARTESIAN_POINT('Ctrl Pts',(4.6630201315191,0.473944543714825,-1.38004669694731E-16));
#40341=CARTESIAN_POINT('Ctrl Pts',(4.63702542177262,0.609947964574148,-1.38777878078145E-16));
#40342=CARTESIAN_POINT('Ctrl Pts',(4.62055356019607,0.696128173708246,-1.39267830902609E-16));
#40343=CARTESIAN_POINT('Ctrl Pts',(4.60162268181677,0.781883974967431,8.79945197126988E-17));
#40344=CARTESIAN_POINT('Ctrl Pts',(4.58020591978812,0.867104757427645,1.11022302462516E-16));
#40345=CARTESIAN_POINT('Ctrl Pts',(4.56733705680351,0.918312058113609,6.78760316859931E-17));
#40346=CARTESIAN_POINT('Ctrl Pts',(4.55357049340461,0.96932610659445,-4.99175148350681E-16));
#40347=CARTESIAN_POINT('Ctrl Pts',(4.53891402393445,1.0201248132638,-5.55111512312578E-16));
#40348=CARTESIAN_POINT('Ctrl Pts',(4.5307224586103,1.04851643410481,-5.86374592437204E-16));
#40349=CARTESIAN_POINT('Ctrl Pts',(4.52225289509851,1.0768407763045,9.91752405205522E-17));
#40350=CARTESIAN_POINT('Ctrl Pts',(4.51350658698018,1.10509389044702,1.11022302462516E-16));
#40351=CARTESIAN_POINT('Ctrl Pts',(4.50742875670279,1.12472704654475,1.19254853933931E-16));
#40352=CARTESIAN_POINT('Ctrl Pts',(4.50121763562789,1.14432449467847,-5.35474147175706E-16));
#40353=CARTESIAN_POINT('Ctrl Pts',(4.49487767268156,1.16387312026907,-5.27355936696949E-16));
#40354=CARTESIAN_POINT('Ctrl Pts',(4.45189774593679,1.2963973168547,-4.72320900273343E-16));
#40355=CARTESIAN_POINT('Ctrl Pts',(4.40295499932666,1.42682794112182,5.0484926233065E-16));
#40356=CARTESIAN_POINT('Ctrl Pts',(4.34826585417728,1.55478882374,3.88578058618805E-16));
#40357=CARTESIAN_POINT('Ctrl Pts',(4.29692960608226,1.67490464560194,2.79435241634665E-16));
#40358=CARTESIAN_POINT('Ctrl Pts',(4.24052923074577,1.79284458992044,2.95867102710926E-16));
#40359=CARTESIAN_POINT('Ctrl Pts',(4.17920839057011,1.90827559700852,4.9960036108132E-16));
#40360=CARTESIAN_POINT('Ctrl Pts',(4.15338816346376,1.95687986938296,5.85385862147007E-16));
#40361=CARTESIAN_POINT('Ctrl Pts',(4.12669516016291,2.0050390084677,-2.10958088174218E-16));
#40362=CARTESIAN_POINT('Ctrl Pts',(4.09913850024111,2.05272668507128,-1.66533453693773E-16));
#40363=CARTESIAN_POINT('Ctrl Pts',(4.08221130669435,2.08201973197734,-1.3924479141655E-16));
#40364=CARTESIAN_POINT('Ctrl Pts',(4.06495515473503,2.11113968242291,3.92725569055683E-16));
#40365=CARTESIAN_POINT('Ctrl Pts',(4.04738928099658,2.14005245629164,3.33066907387547E-16));
#40366=CARTESIAN_POINT('Ctrl Pts',(3.97588097586157,2.2577524629574,9.02045342409376E-17));
#40367=CARTESIAN_POINT('Ctrl Pts',(3.89920169633387,2.37209762967783,1.73844745989399E-16));
#40368=CARTESIAN_POINT('Ctrl Pts',(3.81753428055142,2.4827050770719,1.11022302462516E-16));
#40369=CARTESIAN_POINT('Ctrl Pts',(3.73700167373633,2.59177557950503,4.90728077314622E-17));
#40370=CARTESIAN_POINT('Ctrl Pts',(3.65161810526706,2.69721206501942,-2.17511715066662E-16));
#40371=CARTESIAN_POINT('Ctrl Pts',(3.56152350731999,2.79861134980753,-2.22044604925031E-16));
#40372=CARTESIAN_POINT('Ctrl Pts',(3.54164701408898,2.82098186084422,-2.23044642181868E-16));
#40373=CARTESIAN_POINT('Ctrl Pts',(3.52154110171521,2.8431557130462,3.77586732270394E-16));
#40374=CARTESIAN_POINT('Ctrl Pts',(3.50120707213069,2.86512829543052,4.44089209850063E-16));
#40375=CARTESIAN_POINT('Ctrl Pts',(3.47910313325541,2.88901340959032,5.16017817963063E-16));
#40376=CARTESIAN_POINT('Ctrl Pts',(3.45672963690434,2.91266069254474,2.77193395410128E-16));
#40377=CARTESIAN_POINT('Ctrl Pts',(3.43409108914483,2.93606647242265,2.77555756156289E-16));
#40378=CARTESIAN_POINT('Origin',(0.,0.,20.5));
#40379=CARTESIAN_POINT('Origin',(0.,0.,41.));
#40380=CARTESIAN_POINT('',(-4.,4.89858719658941E-16,41.));
#40381=CARTESIAN_POINT('Origin',(0.,0.,41.));
#40382=CARTESIAN_POINT('Origin',(-4.45462538595717E-16,-1.65775395963113E-16,
375.));
#40383=CARTESIAN_POINT('Ctrl Pts',(-3.43378788736335,2.93584158412826,375.));
#40384=CARTESIAN_POINT('Ctrl Pts',(-3.52812472271588,2.83822707478694,375.));
#40385=CARTESIAN_POINT('Ctrl Pts',(-3.61783741229297,2.73641228828402,375.));
#40386=CARTESIAN_POINT('Ctrl Pts',(-3.70278930559469,2.6308098016192,375.));
#40387=CARTESIAN_POINT('Ctrl Pts',(-3.78883118430305,2.52385236964479,375.));
#40388=CARTESIAN_POINT('Ctrl Pts',(-3.86998980756465,2.41300886934011,375.));
#40389=CARTESIAN_POINT('Ctrl Pts',(-3.94608965952372,2.29866645157891,375.));
#40390=CARTESIAN_POINT('Ctrl Pts',(-3.98412572654406,2.24151606621978,375.));
#40391=CARTESIAN_POINT('Ctrl Pts',(-4.02089745503991,2.18349099620346,375.));
#40392=CARTESIAN_POINT('Ctrl Pts',(-4.0563792513302,2.12463643972661,375.));
#40393=CARTESIAN_POINT('Ctrl Pts',(-4.0706431485814,2.10097655116059,375.));
#40394=CARTESIAN_POINT('Ctrl Pts',(-4.08469915763129,2.07718134398868,375.));
#40395=CARTESIAN_POINT('Ctrl Pts',(-4.09853534340515,2.05327180953563,375.));
#40396=CARTESIAN_POINT('Ctrl Pts',(-4.16827482663706,1.93275893089092,375.));
#40397=CARTESIAN_POINT('Ctrl Pts',(-4.23249571495574,1.80924176863962,375.));
#40398=CARTESIAN_POINT('Ctrl Pts',(-4.29102780012401,1.68312480250504,375.));
#40399=CARTESIAN_POINT('Ctrl Pts',(-4.34427585815273,1.56839313846413,375.));
#40400=CARTESIAN_POINT('Ctrl Pts',(-4.3928156984662,1.45150902581472,375.));
#40401=CARTESIAN_POINT('Ctrl Pts',(-4.4364893782082,1.33275463175064,375.));
#40402=CARTESIAN_POINT('Ctrl Pts',(-4.46204208504677,1.2632735109649,375.));
#40403=CARTESIAN_POINT('Ctrl Pts',(-4.48592844490179,1.19315178813539,375.));
#40404=CARTESIAN_POINT('Ctrl Pts',(-4.50811171504532,1.12244350259313,375.));
#40405=CARTESIAN_POINT('Ctrl Pts',(-4.5141904988611,1.10306762252609,375.));
#40406=CARTESIAN_POINT('Ctrl Pts',(-4.52013855791141,1.08365664730297,375.));
#40407=CARTESIAN_POINT('Ctrl Pts',(-4.52595509671778,1.06421299497352,375.));
#40408=CARTESIAN_POINT('Ctrl Pts',(-4.53519138586709,1.0333377268782,375.));
#40409=CARTESIAN_POINT('Ctrl Pts',(-4.54409635013865,1.00237910104441,375.));
#40410=CARTESIAN_POINT('Ctrl Pts',(-4.55266817723945,0.971342071123453,
375.));
#40411=CARTESIAN_POINT('Ctrl Pts',(-4.58939773349738,0.838351015289689,
375.));
#40412=CARTESIAN_POINT('Ctrl Pts',(-4.62001434120323,0.703922655316075,
375.));
#40413=CARTESIAN_POINT('Ctrl Pts',(-4.6446125449424,0.568489655194437,375.));
#40414=CARTESIAN_POINT('Ctrl Pts',(-4.6695978975114,0.43092508774079,375.));
#40415=CARTESIAN_POINT('Ctrl Pts',(-4.68837408722962,0.292323323451818,
375.));
#40416=CARTESIAN_POINT('Ctrl Pts',(-4.7009917947161,0.153114389433896,375.));
#40417=CARTESIAN_POINT('Ctrl Pts',(-4.71369611133585,0.0129499121739395,
375.));
#40418=CARTESIAN_POINT('Ctrl Pts',(-4.72015723771216,-0.127830868720726,
375.));
#40419=CARTESIAN_POINT('Ctrl Pts',(-4.72037601386282,-0.2688014592115,375.));
#40420=CARTESIAN_POINT('Ctrl Pts',(-4.72051776383518,-0.360139464952745,
375.));
#40421=CARTESIAN_POINT('Ctrl Pts',(-4.71803791594725,-0.451557379168488,
375.));
#40422=CARTESIAN_POINT('Ctrl Pts',(-4.7129250253839,-0.542939603201634,
375.));
#40423=CARTESIAN_POINT('Ctrl Pts',(-4.71050429468246,-0.586205100974703,
375.));
#40424=CARTESIAN_POINT('Ctrl Pts',(-4.70749320436126,-0.629462591214061,
375.));
#40425=CARTESIAN_POINT('Ctrl Pts',(-4.70388981020381,-0.672699721412066,
375.));
#40426=CARTESIAN_POINT('Ctrl Pts',(-4.70250698353675,-0.689292260011098,
375.));
#40427=CARTESIAN_POINT('Ctrl Pts',(-4.7010370790231,-0.705879562100339,
375.));
#40428=CARTESIAN_POINT('Ctrl Pts',(-4.69948096449077,-0.722452069367425,
375.));
#40429=CARTESIAN_POINT('Ctrl Pts',(-4.68606574819498,-0.865323153038659,
375.));
#40430=CARTESIAN_POINT('Ctrl Pts',(-4.66623214709618,-1.0072815713457,375.));
#40431=CARTESIAN_POINT('Ctrl Pts',(-4.64004375541204,-1.14788248706686,
375.));
#40432=CARTESIAN_POINT('Ctrl Pts',(-4.6270279916287,-1.21776185685865,375.));
#40433=CARTESIAN_POINT('Ctrl Pts',(-4.61244171628795,-1.28730612660771,
375.));
#40434=CARTESIAN_POINT('Ctrl Pts',(-4.59628803251995,-1.35646150527604,
375.));
#40435=CARTESIAN_POINT('Ctrl Pts',(-4.56399682193468,-1.4947030932479,375.));
#40436=CARTESIAN_POINT('Ctrl Pts',(-4.52544561415923,-1.63139110841489,
375.));
#40437=CARTESIAN_POINT('Ctrl Pts',(-4.48088607305284,-1.76617553752727,
375.));
#40438=CARTESIAN_POINT('Ctrl Pts',(-4.43597574851398,-1.90202102210641,
375.));
#40439=CARTESIAN_POINT('Ctrl Pts',(-4.38496188398045,-2.03593355195248,
375.));
#40440=CARTESIAN_POINT('Ctrl Pts',(-4.32805045687434,-2.16754392308446,
375.));
#40441=CARTESIAN_POINT('Ctrl Pts',(-4.30216783694698,-2.22739870775111,
375.));
#40442=CARTESIAN_POINT('Ctrl Pts',(-4.27506473176287,-2.28677711825493,
375.));
#40443=CARTESIAN_POINT('Ctrl Pts',(-4.24675722722924,-2.34564306219817,
375.));
#40444=CARTESIAN_POINT('Ctrl Pts',(-4.22863084786129,-2.38333718074896,
375.));
#40445=CARTESIAN_POINT('Ctrl Pts',(-4.21001058428347,-2.42082115169986,
375.));
#40446=CARTESIAN_POINT('Ctrl Pts',(-4.190900240747,-2.45808525714998,375.));
#40447=CARTESIAN_POINT('Ctrl Pts',(-4.18310501328873,-2.47328551649951,
375.));
#40448=CARTESIAN_POINT('Ctrl Pts',(-4.17522954608524,-2.48844657780472,
375.));
#40449=CARTESIAN_POINT('Ctrl Pts',(-4.16727814768109,-2.50356042854303,
375.));
#40450=CARTESIAN_POINT('Ctrl Pts',(-4.09969026676857,-2.63203005010014,
375.));
#40451=CARTESIAN_POINT('Ctrl Pts',(-4.02654009074559,-2.75724655837471,
375.));
#40452=CARTESIAN_POINT('Ctrl Pts',(-3.94810710693448,-2.87885707775794,
375.));
#40453=CARTESIAN_POINT('Ctrl Pts',(-3.86905485941559,-3.00142776692534,
375.));
#40454=CARTESIAN_POINT('Ctrl Pts',(-3.78463578072622,-3.12033603731368,
375.));
#40455=CARTESIAN_POINT('Ctrl Pts',(-3.69508499761951,-3.23520722691392,
375.));
#40456=CARTESIAN_POINT('Ctrl Pts',(-3.62943480927899,-3.31941994924341,
375.));
#40457=CARTESIAN_POINT('Ctrl Pts',(-3.56102553573526,-3.40146273807253,
375.));
#40458=CARTESIAN_POINT('Ctrl Pts',(-3.48993392179959,-3.48117995730746,
375.));
#40459=CARTESIAN_POINT('Ctrl Pts',(-3.39320786765338,-3.58964186493951,
375.));
#40460=CARTESIAN_POINT('Ctrl Pts',(-3.29151757709749,-3.69380035593463,
375.));
#40461=CARTESIAN_POINT('Ctrl Pts',(-3.18521993250538,-3.79343311373674,
375.));
#40462=CARTESIAN_POINT('Ctrl Pts',(-3.1484894856507,-3.82786055311678,375.));
#40463=CARTESIAN_POINT('Ctrl Pts',(-3.1112085895158,-3.86174730075506,375.));
#40464=CARTESIAN_POINT('Ctrl Pts',(-3.07339099123149,-3.89508311993719,
375.));
#40465=CARTESIAN_POINT('Ctrl Pts',(-3.05466088259105,-3.91159351571128,
375.));
#40466=CARTESIAN_POINT('Ctrl Pts',(-3.03579911530405,-3.92796876126283,
375.));
#40467=CARTESIAN_POINT('Ctrl Pts',(-3.01680731961894,-3.94420755857869,
375.));
#40468=CARTESIAN_POINT('Ctrl Pts',(-3.00397674416022,-3.95517824917451,
375.));
#40469=CARTESIAN_POINT('Ctrl Pts',(-2.99108750647465,-3.96608603020355,
375.));
#40470=CARTESIAN_POINT('Ctrl Pts',(-2.97814807270005,-3.97692398964623,
375.));
#40471=CARTESIAN_POINT('Ctrl Pts',(-2.86441519405387,-4.07218567941864,
375.));
#40472=CARTESIAN_POINT('Ctrl Pts',(-2.74664729621727,-4.16219378118691,
375.));
#40473=CARTESIAN_POINT('Ctrl Pts',(-2.62528201158405,-4.24677543677276,
375.));
#40474=CARTESIAN_POINT('Ctrl Pts',(-2.50379141827822,-4.33144442223239,
375.));
#40475=CARTESIAN_POINT('Ctrl Pts',(-2.3786953776454,-4.41067622052404,375.));
#40476=CARTESIAN_POINT('Ctrl Pts',(-2.25039003171722,-4.4842647871821,375.));
#40477=CARTESIAN_POINT('Ctrl Pts',(-2.12228319217728,-4.5577395019934,375.));
#40478=CARTESIAN_POINT('Ctrl Pts',(-1.9909763337868,-4.62558889864692,375.));
#40479=CARTESIAN_POINT('Ctrl Pts',(-1.85683056691249,-4.68756837108862,
375.));
#40480=CARTESIAN_POINT('Ctrl Pts',(-1.72268480003817,-4.74954784353032,
375.));
#40481=CARTESIAN_POINT('Ctrl Pts',(-1.58569949586696,-4.80565788540407,
375.));
#40482=CARTESIAN_POINT('Ctrl Pts',(-1.44621200484621,-4.85560714827263,
375.));
#40483=CARTESIAN_POINT('Ctrl Pts',(-1.40211572701684,-4.87139764358304,
375.));
#40484=CARTESIAN_POINT('Ctrl Pts',(-1.35776924324391,-4.88657205481219,
375.));
#40485=CARTESIAN_POINT('Ctrl Pts',(-1.31318542874385,-4.90112866933901,
375.));
#40486=CARTESIAN_POINT('Ctrl Pts',(1.31303618635831,-4.90075024188273,375.));
#40487=CARTESIAN_POINT('Ctrl Pts',(1.45436548505342,-4.85453285551617,375.));
#40488=CARTESIAN_POINT('Ctrl Pts',(1.5934293761686,-4.80203848222433,375.));
#40489=CARTESIAN_POINT('Ctrl Pts',(1.72987023226972,-4.74352674861442,375.));
#40490=CARTESIAN_POINT('Ctrl Pts',(1.86675271207831,-4.68482562767973,375.));
#40491=CARTESIAN_POINT('Ctrl Pts',(2.00099581082903,-4.620067688427,375.));
#40492=CARTESIAN_POINT('Ctrl Pts',(2.13221219437754,-4.54946990611926,375.));
#40493=CARTESIAN_POINT('Ctrl Pts',(2.19270449791029,-4.5169234941499,375.));
#40494=CARTESIAN_POINT('Ctrl Pts',(2.25255310159603,-4.48313534130926,375.));
#40495=CARTESIAN_POINT('Ctrl Pts',(2.31171758991926,-4.44812388272337,375.));
#40496=CARTESIAN_POINT('Ctrl Pts',(2.3344624112488,-4.43466429923687,375.));
#40497=CARTESIAN_POINT('Ctrl Pts',(2.35710754237018,-4.42102302699321,375.));
#40498=CARTESIAN_POINT('Ctrl Pts',(2.37964612843956,-4.40720380568676,375.));
#40499=CARTESIAN_POINT('Ctrl Pts',(2.50549113115601,-4.33004368847728,375.));
#40500=CARTESIAN_POINT('Ctrl Pts',(2.62778788875034,-4.24748071485227,375.));
#40501=CARTESIAN_POINT('Ctrl Pts',(2.74616817727066,-4.15974114711123,375.));
#40502=CARTESIAN_POINT('Ctrl Pts',(2.86286389724632,-4.07325012604791,375.));
#40503=CARTESIAN_POINT('Ctrl Pts',(2.97575433427861,-3.98172826743118,375.));
#40504=CARTESIAN_POINT('Ctrl Pts',(3.08445220151971,-3.8853563473526,375.));
#40505=CARTESIAN_POINT('Ctrl Pts',(3.13995990370008,-3.83614301894012,375.));
#40506=CARTESIAN_POINT('Ctrl Pts',(3.19437368596074,-3.78566438686541,375.));
#40507=CARTESIAN_POINT('Ctrl Pts',(3.24763776430821,-3.73394147802337,375.));
#40508=CARTESIAN_POINT('Ctrl Pts',(3.2699643084639,-3.71226094127233,375.));
#40509=CARTESIAN_POINT('Ctrl Pts',(3.29209335275734,-3.69035703897681,375.));
#40510=CARTESIAN_POINT('Ctrl Pts',(3.31399620763943,-3.66825627851417,375.));
#40511=CARTESIAN_POINT('Ctrl Pts',(3.34216498231236,-3.63983298187436,375.));
#40512=CARTESIAN_POINT('Ctrl Pts',(3.36996576521876,-3.6110784436862,375.));
#40513=CARTESIAN_POINT('Ctrl Pts',(3.39739154337912,-3.58199736557932,375.));
#40514=CARTESIAN_POINT('Ctrl Pts',(3.49658091940006,-3.47682135290355,375.));
#40515=CARTESIAN_POINT('Ctrl Pts',(3.59086820857194,-3.3673769231021,375.));
#40516=CARTESIAN_POINT('Ctrl Pts',(3.6800850008747,-3.25406730243395,375.));
#40517=CARTESIAN_POINT('Ctrl Pts',(3.76996985501536,-3.13990921107455,375.));
#40518=CARTESIAN_POINT('Ctrl Pts',(3.85470838531078,-3.02182713075438,375.));
#40519=CARTESIAN_POINT('Ctrl Pts',(3.93408537345353,-2.90020291820586,375.));
#40520=CARTESIAN_POINT('Ctrl Pts',(4.01274556585136,-2.77967700530409,375.));
#40521=CARTESIAN_POINT('Ctrl Pts',(4.08614088023802,-2.65567191437214,375.));
#40522=CARTESIAN_POINT('Ctrl Pts',(4.15401504305787,-2.52854018053819,375.));
#40523=CARTESIAN_POINT('Ctrl Pts',(4.19807507197777,-2.44601352184147,375.));
#40524=CARTESIAN_POINT('Ctrl Pts',(4.23980760353704,-2.36216897889331,375.));
#40525=CARTESIAN_POINT('Ctrl Pts',(4.27913099033935,-2.27710078886137,375.));
#40526=CARTESIAN_POINT('Ctrl Pts',(4.29645860907187,-2.23961599207746,375.));
#40527=CARTESIAN_POINT('Ctrl Pts',(4.31331832747089,-2.20189359019125,375.));
#40528=CARTESIAN_POINT('Ctrl Pts',(4.32970256286081,-2.16394161183312,375.));
#40529=CARTESIAN_POINT('Ctrl Pts',(4.33919451441291,-2.14195472435813,375.));
#40530=CARTESIAN_POINT('Ctrl Pts',(4.34852813367479,-2.11988754210219,375.));
#40531=CARTESIAN_POINT('Ctrl Pts',(4.35769217797944,-2.0977656675703,375.));
#40532=CARTESIAN_POINT('Ctrl Pts',(4.41245445040556,-1.96557030933995,375.));
#40533=CARTESIAN_POINT('Ctrl Pts',(4.46123822222855,-1.83125898605536,375.));
#40534=CARTESIAN_POINT('Ctrl Pts',(4.50384926204605,-1.6951979775962,375.));
#40535=CARTESIAN_POINT('Ctrl Pts',(4.52559692351824,-1.62575567428212,375.));
#40536=CARTESIAN_POINT('Ctrl Pts',(4.54573592530189,-1.55585726815914,375.));
#40537=CARTESIAN_POINT('Ctrl Pts',(4.56423545664257,-1.48554983900212,375.));
#40538=CARTESIAN_POINT('Ctrl Pts',(4.60056463169787,-1.34748088717324,375.));
#40539=CARTESIAN_POINT('Ctrl Pts',(4.63057447100037,-1.20783464517222,375.));
#40540=CARTESIAN_POINT('Ctrl Pts',(4.65426082259252,-1.06704756524395,375.));
#40541=CARTESIAN_POINT('Ctrl Pts',(4.67788678995459,-0.926619397467839,
375.));
#40542=CARTESIAN_POINT('Ctrl Pts',(4.69522141344644,-0.785055397710089,
375.));
#40543=CARTESIAN_POINT('Ctrl Pts',(4.7062090782541,-0.642791899249072,375.));
#40544=CARTESIAN_POINT('Ctrl Pts',(4.71102657060836,-0.58041710641334,375.));
#40545=CARTESIAN_POINT('Ctrl Pts',(4.71462329627092,-0.5179079594038,375.));
#40546=CARTESIAN_POINT('Ctrl Pts',(4.71699147233722,-0.455302034234564,
375.));
#40547=CARTESIAN_POINT('Ctrl Pts',(4.71854674616479,-0.414186275042497,
375.));
#40548=CARTESIAN_POINT('Ctrl Pts',(4.71957210036622,-0.373028786701393,
375.));
#40549=CARTESIAN_POINT('Ctrl Pts',(4.72006488912048,-0.331840385723362,
375.));
#40550=CARTESIAN_POINT('Ctrl Pts',(4.72028902811531,-0.313106340528846,
375.));
#40551=CARTESIAN_POINT('Ctrl Pts',(4.72040288834379,-0.294371677101196,
375.));
#40552=CARTESIAN_POINT('Ctrl Pts',(4.72040648677608,-0.275644826658347,
375.));
#40553=CARTESIAN_POINT('Ctrl Pts',(4.72043355701338,-0.134766732053278,
375.));
#40554=CARTESIAN_POINT('Ctrl Pts',(4.71422662120245,0.0057990813089247,
375.));
#40555=CARTESIAN_POINT('Ctrl Pts',(4.70180390274057,0.145635587850549,375.));
#40556=CARTESIAN_POINT('Ctrl Pts',(4.68946458626375,0.284533278764535,375.));
#40557=CARTESIAN_POINT('Ctrl Pts',(4.67099254981089,0.422712188593173,375.));
#40558=CARTESIAN_POINT('Ctrl Pts',(4.6463550982981,0.559757549565289,375.));
#40559=CARTESIAN_POINT('Ctrl Pts',(4.62907635772754,0.655870219230258,375.));
#40560=CARTESIAN_POINT('Ctrl Pts',(4.60876410990094,0.751425238603689,375.));
#40561=CARTESIAN_POINT('Ctrl Pts',(4.58539251247819,0.846274706840598,375.));
#40562=CARTESIAN_POINT('Ctrl Pts',(4.55189132819966,0.982233300369681,375.));
#40563=CARTESIAN_POINT('Ctrl Pts',(4.51210568697928,1.11674373042915,375.));
#40564=CARTESIAN_POINT('Ctrl Pts',(4.46619637471526,1.24939846486887,375.));
#40565=CARTESIAN_POINT('Ctrl Pts',(4.4514821415469,1.29191517002461,375.));
#40566=CARTESIAN_POINT('Ctrl Pts',(4.43613853638538,1.33424101402745,375.));
#40567=CARTESIAN_POINT('Ctrl Pts',(4.42016997732094,1.37636185265469,375.));
#40568=CARTESIAN_POINT('Ctrl Pts',(4.41229563070378,1.39713229799154,375.));
#40569=CARTESIAN_POINT('Ctrl Pts',(4.40426931219602,1.41785288761014,375.));
#40570=CARTESIAN_POINT('Ctrl Pts',(4.39609151624634,1.43852188916379,375.));
#40571=CARTESIAN_POINT('Ctrl Pts',(4.38944561986513,1.45531908531226,375.));
#40572=CARTESIAN_POINT('Ctrl Pts',(4.38270019096179,1.4720807922257,375.));
#40573=CARTESIAN_POINT('Ctrl Pts',(4.37586028060643,1.48879486186589,375.));
#40574=CARTESIAN_POINT('Ctrl Pts',(4.32342038722716,1.61693748133431,375.));
#40575=CARTESIAN_POINT('Ctrl Pts',(4.26535943234438,1.74246391819237,375.));
#40576=CARTESIAN_POINT('Ctrl Pts',(4.20190818178381,1.86501937630542,375.));
#40577=CARTESIAN_POINT('Ctrl Pts',(4.13850743678452,1.98747728343019,375.));
#40578=CARTESIAN_POINT('Ctrl Pts',(4.06972452623307,2.10696961603591,375.));
#40579=CARTESIAN_POINT('Ctrl Pts',(3.99574428312086,2.22311713285455,375.));
#40580=CARTESIAN_POINT('Ctrl Pts',(3.9230204444275,2.3372921196134,375.));
#40581=CARTESIAN_POINT('Ctrl Pts',(3.84527380385539,2.44823547455532,375.));
#40582=CARTESIAN_POINT('Ctrl Pts',(3.7626432675861,2.55555363817714,375.));
#40583=CARTESIAN_POINT('Ctrl Pts',(3.68595020843944,2.65516037730487,375.));
#40584=CARTESIAN_POINT('Ctrl Pts',(3.60504931330013,2.75164424921775,375.));
#40585=CARTESIAN_POINT('Ctrl Pts',(3.52002795172102,2.84465807652531,375.));
#40586=CARTESIAN_POINT('Ctrl Pts',(3.49183173897392,2.87550488507407,375.));
#40587=CARTESIAN_POINT('Ctrl Pts',(3.46318217104164,2.90596975880766,375.));
#40588=CARTESIAN_POINT('Ctrl Pts',(3.43408816985932,2.93604417002309,375.));
#40589=CARTESIAN_POINT('Origin',(0.,0.,402.208336844637));
#40590=CARTESIAN_POINT('Ctrl Pts',(-5.07353386009457,0.000128968315485402,
399.708336844637));
#40591=CARTESIAN_POINT('Ctrl Pts',(-5.07374798994712,0.217328374468673,
399.701523610908));
#40592=CARTESIAN_POINT('Ctrl Pts',(-5.00706367321595,1.27523772951867,399.668334418693));
#40593=CARTESIAN_POINT('Ctrl Pts',(-4.28603436807985,3.09622957226831,399.608769267991));
#40594=CARTESIAN_POINT('Ctrl Pts',(-2.29040909926245,4.7655795591539,399.529641392531));
#40595=CARTESIAN_POINT('Ctrl Pts',(0.259800278618912,5.28102545063066,399.450513517072));
#40596=CARTESIAN_POINT('Ctrl Pts',(2.7471033957984,4.51775909222651,399.371385641611));
#40597=CARTESIAN_POINT('Ctrl Pts',(4.56924148852249,2.66059337678593,399.292257766152));
#40598=CARTESIAN_POINT('Ctrl Pts',(5.2850143906551,0.159209483399153,399.213129890692));
#40599=CARTESIAN_POINT('Ctrl Pts',(4.7211096918349,-2.38072426286758,399.134002015232));
#40600=CARTESIAN_POINT('Ctrl Pts',(3.01406746059458,-4.34420558161996,399.054874139772));
#40601=CARTESIAN_POINT('Ctrl Pts',(0.577219342712345,-5.25581036421826,
398.975746264313));
#40602=CARTESIAN_POINT('Ctrl Pts',(-1.99939275815206,-4.89480881878609,
398.896618388853));
#40603=CARTESIAN_POINT('Ctrl Pts',(-4.09188543486623,-3.34861140683646,
398.817490513394));
#40604=CARTESIAN_POINT('Ctrl Pts',(-4.96571105424643,-1.479143747598,398.754729998654));
#40605=CARTESIAN_POINT('Ctrl Pts',(-5.07346848196321,-0.319197162169717,
398.718345442402));
#40606=CARTESIAN_POINT('Ctrl Pts',(-5.07327504304777,-8.56681209025073E-5,
398.708336844637));
#40607=CARTESIAN_POINT('Ctrl Pts',(-5.07330191118131,0.000105688062508012,
399.791663155363));
#40608=CARTESIAN_POINT('Ctrl Pts',(-5.07350034043644,0.308800908665525,
399.781980894782));
#40609=CARTESIAN_POINT('Ctrl Pts',(-4.97021252404761,1.45829359598981,399.745922675715));
#40610=CARTESIAN_POINT('Ctrl Pts',(-4.11241943286933,3.32339561801255,399.683488498161));
#40611=CARTESIAN_POINT('Ctrl Pts',(-2.02945797892606,4.8824090247121,399.604360622701));
#40612=CARTESIAN_POINT('Ctrl Pts',(0.54487554882432,5.2592655238007,399.525232747241));
#40613=CARTESIAN_POINT('Ctrl Pts',(2.98728943775363,4.36266186092565,399.446104871781));
#40614=CARTESIAN_POINT('Ctrl Pts',(4.70637522433117,2.40972094089285,399.366976996322));
#40615=CARTESIAN_POINT('Ctrl Pts',(5.28589404837916,-0.126697339701679,
399.287849120862));
#40616=CARTESIAN_POINT('Ctrl Pts',(4.58552092441564,-2.6324361653814,399.208721245402));
#40617=CARTESIAN_POINT('Ctrl Pts',(2.77484145336967,-4.50077558224301,399.129593369943));
#40618=CARTESIAN_POINT('Ctrl Pts',(0.292280359106768,-5.27932726882375,
399.050465494482));
#40619=CARTESIAN_POINT('Ctrl Pts',(-2.26105137922953,-4.77957858969287,
398.971337619023));
#40620=CARTESIAN_POINT('Ctrl Pts',(-4.26690751412045,-3.12253502339944,
398.892209743563));
#40621=CARTESIAN_POINT('Ctrl Pts',(-5.00313619365009,-1.29606201606178,
398.832318255676));
#40622=CARTESIAN_POINT('Ctrl Pts',(-5.07372209014652,-0.227734309753026,
398.798802726276));
#40623=CARTESIAN_POINT('Ctrl Pts',(-5.07350261625086,-0.000127405426567848,
398.791663155363));
#40624=CARTESIAN_POINT('Ctrl Pts',(3.43378788736214,2.93584158412968,400.));
#40625=CARTESIAN_POINT('Ctrl Pts',(3.92033033613488,2.36677696691239,399.973624041513));
#40626=CARTESIAN_POINT('Ctrl Pts',(4.60446627899797,0.982571495138102,399.92087212454));
#40627=CARTESIAN_POINT('Ctrl Pts',(4.51560363134058,-1.33271150407048,399.84174424908));
#40628=CARTESIAN_POINT('Ctrl Pts',(3.3333277577492,-3.32493526877752,399.762616373621));
#40629=CARTESIAN_POINT('Ctrl Pts',(1.34394627169084,-4.51226606526834,399.683488498161));
#40630=CARTESIAN_POINT('Ctrl Pts',(-0.97085300939813,-4.60694214684371,
399.604360622701));
#40631=CARTESIAN_POINT('Ctrl Pts',(-3.05057500858779,-3.58616495104857,
399.525232747241));
#40632=CARTESIAN_POINT('Ctrl Pts',(-4.391652180308,-1.69703895278099,399.446104871782));
#40633=CARTESIAN_POINT('Ctrl Pts',(-4.66936408063869,0.602987533589634,
399.366976996322));
#40634=CARTESIAN_POINT('Ctrl Pts',(-3.81646794512629,2.7570149696695,399.287849120862));
#40635=CARTESIAN_POINT('Ctrl Pts',(-2.03947802510898,4.24347545201977,399.208721245402));
#40636=CARTESIAN_POINT('Ctrl Pts',(0.231337257318392,4.70245047492642,399.129593369942));
#40637=CARTESIAN_POINT('Ctrl Pts',(2.44613812014511,4.02280553037415,399.050465494483));
#40638=CARTESIAN_POINT('Ctrl Pts',(4.06864765349505,2.36910590664905,398.971337619023));
#40639=CARTESIAN_POINT('Ctrl Pts',(4.70600239738688,0.141766919667795,398.892209743563));
#40640=CARTESIAN_POINT('Ctrl Pts',(4.20387758402063,-2.11989850176798,398.813081868103));
#40641=CARTESIAN_POINT('Ctrl Pts',(2.68385431845262,-3.86826607662479,398.733953992643));
#40642=CARTESIAN_POINT('Ctrl Pts',(0.513980740606018,-4.67999788571173,
398.654826117184));
#40643=CARTESIAN_POINT('Ctrl Pts',(-1.78034465333125,-4.35854670077871,
398.575698241724));
#40644=CARTESIAN_POINT('Ctrl Pts',(-3.64358944799884,-2.98174652775848,
398.496570366264));
#40645=CARTESIAN_POINT('Ctrl Pts',(-4.62460016500653,-0.88296644150622,
398.417442490804));
#40646=CARTESIAN_POINT('Ctrl Pts',(-4.48584151198124,1.42960916071621,398.338314615345));
#40647=CARTESIAN_POINT('Ctrl Pts',(-3.2609115695794,3.39602888062287,398.259186739885));
#40648=CARTESIAN_POINT('Ctrl Pts',(-1.24640657987359,4.54015716254393,398.180058864425));
#40649=CARTESIAN_POINT('Ctrl Pts',(1.06989485946835,4.5849625311949,398.100930988966));
#40650=CARTESIAN_POINT('Ctrl Pts',(3.12713920196537,3.51959611807719,398.021803113505));
#40651=CARTESIAN_POINT('Ctrl Pts',(4.42719923245446,1.6020185326593,397.942675238046));
#40652=CARTESIAN_POINT('Ctrl Pts',(4.65528721806493,-0.70346097272927,397.863547362586));
#40653=CARTESIAN_POINT('Ctrl Pts',(3.75617547838133,-2.83860920142977,397.784419487126));
#40654=CARTESIAN_POINT('Ctrl Pts',(1.94756884202228,-4.28643581876784,397.705291611666));
#40655=CARTESIAN_POINT('Ctrl Pts',(-0.332608926446521,-4.69637389108681,
397.626163736207));
#40656=CARTESIAN_POINT('Ctrl Pts',(-2.53225102161336,-3.96916378931016,
397.547035860747));
#40657=CARTESIAN_POINT('Ctrl Pts',(-4.11875100068,-2.28088724342758,397.467907985287));
#40658=CARTESIAN_POINT('Ctrl Pts',(-4.70796450115822,-0.0403321046706491,
397.388780109827));
#40659=CARTESIAN_POINT('Ctrl Pts',(-4.15722335570028,2.20998877681613,397.309652234368));
#40660=CARTESIAN_POINT('Ctrl Pts',(-2.59988029611171,3.92519794006916,397.230524358908));
#40661=CARTESIAN_POINT('Ctrl Pts',(-0.413019825824474,4.6899862522516,397.151396483448));
#40662=CARTESIAN_POINT('Ctrl Pts',(1.87384646846516,4.31917304995456,397.072268607988));
#40663=CARTESIAN_POINT('Ctrl Pts',(3.70699226699225,2.90254453114723,396.993140732528));
#40664=CARTESIAN_POINT('Ctrl Pts',(4.6425520586224,0.783113533157272,396.914012857069));
#40665=CARTESIAN_POINT('Ctrl Pts',(4.45399573023398,-1.52593527316547,396.834884981609));
#40666=CARTESIAN_POINT('Ctrl Pts',(3.18697903443818,-3.46550444479366,396.755757106149));
#40667=CARTESIAN_POINT('Ctrl Pts',(1.14828881478399,-4.56595983563972,396.676629230689));
#40668=CARTESIAN_POINT('Ctrl Pts',(-1.16844028323631,-4.56084462872216,
396.597501355229));
#40669=CARTESIAN_POINT('Ctrl Pts',(-3.20225116276825,-3.45139738560812,
396.51837347977));
#40670=CARTESIAN_POINT('Ctrl Pts',(-4.46069062869795,-1.50625214950199,
396.43924560431));
#40671=CARTESIAN_POINT('Ctrl Pts',(-4.63904866983842,0.803606783012363,
396.36011772885));
#40672=CARTESIAN_POINT('Ctrl Pts',(-3.69413887779848,2.91888581043708,396.28098985339));
#40673=CARTESIAN_POINT('Ctrl Pts',(-1.85475531148862,4.32740559196129,396.201861977931));
#40674=CARTESIAN_POINT('Ctrl Pts',(0.433726147102728,4.68811668499756,396.122734102471));
#40675=CARTESIAN_POINT('Ctrl Pts',(2.61718809326315,3.9136789479101,396.043606227011));
#40676=CARTESIAN_POINT('Ctrl Pts',(4.16694183591648,2.19160949051653,395.964478351551));
#40677=CARTESIAN_POINT('Ctrl Pts',(4.70774049744502,-0.0611214491752849,
395.885350476092));
#40678=CARTESIAN_POINT('Ctrl Pts',(4.10863875177974,-2.29905285502682,395.806222600631));
#40679=CARTESIAN_POINT('Ctrl Pts',(2.5146990390031,-3.98030716981366,395.727094725172));
#40680=CARTESIAN_POINT('Ctrl Pts',(0.311867128348267,-4.69779685779291,
395.647966849712));
#40681=CARTESIAN_POINT('Ctrl Pts',(-1.96647817706303,-4.27779382415375,
395.568838974252));
#40682=CARTESIAN_POINT('Ctrl Pts',(-3.7686737720159,-2.82199475955442,395.489711098792));
#40683=CARTESIAN_POINT('Ctrl Pts',(-4.65834821810063,-0.682896992050643,
395.410583223333));
#40684=CARTESIAN_POINT('Ctrl Pts',(-4.42008176906904,1.62155282910444,395.331455347873));
#40685=CARTESIAN_POINT('Ctrl Pts',(-3.11156664954973,3.53337082801154,395.252327472413));
#40686=CARTESIAN_POINT('Ctrl Pts',(-1.0496378504197,4.58964233963818,395.173199596953));
#40687=CARTESIAN_POINT('Ctrl Pts',(1.2664431505466,4.53460893234099,395.094071721494));
#40688=CARTESIAN_POINT('Ctrl Pts',(3.27587618232697,3.381596022723,395.014943846034));
#40689=CARTESIAN_POINT('Ctrl Pts',(4.49211073679585,1.40978634948583,394.935815970574));
#40690=CARTESIAN_POINT('Ctrl Pts',(4.6206560142512,-0.903379444528889,394.856688095114));
#40691=CARTESIAN_POINT('Ctrl Pts',(3.63038693161045,-2.99780705677087,394.777560219655));
#40692=CARTESIAN_POINT('Ctrl Pts',(1.7610805392752,-4.36636596691336,394.698432344195));
#40693=CARTESIAN_POINT('Ctrl Pts',(-0.534641970284508,-4.6776825871839,
394.619304468735));
#40694=CARTESIAN_POINT('Ctrl Pts',(-2.7009098933051,-3.85637681912437,394.540176593275));
#40695=CARTESIAN_POINT('Ctrl Pts',(-4.21319778305003,-2.1013140802211,394.461048717815));
#40696=CARTESIAN_POINT('Ctrl Pts',(-4.7053304898376,0.162546621736014,394.381920842356));
#40697=CARTESIAN_POINT('Ctrl Pts',(-4.05814633235487,2.38704938533492,394.302792966896));
#40698=CARTESIAN_POINT('Ctrl Pts',(-2.42835010030815,4.03356817385879,394.223665091436));
#40699=CARTESIAN_POINT('Ctrl Pts',(-0.210569617716467,4.70342607669429,
394.144537215976));
#40700=CARTESIAN_POINT('Ctrl Pts',(2.05819676630879,4.23442823696295,394.065409340517));
#40701=CARTESIAN_POINT('Ctrl Pts',(3.82860532171676,2.74013461591856,393.986281465057));
#40702=CARTESIAN_POINT('Ctrl Pts',(4.67198130861809,0.582363352861709,393.907153589597));
#40703=CARTESIAN_POINT('Ctrl Pts',(4.38411537617703,-1.71641742918247,393.828025714137));
#40704=CARTESIAN_POINT('Ctrl Pts',(3.03470943208895,-3.59959651705903,393.748897838677));
#40705=CARTESIAN_POINT('Ctrl Pts',(0.950499494613711,-4.61119367773381,
393.669769963218));
#40706=CARTESIAN_POINT('Ctrl Pts',(-1.36385795450447,-4.50626762440581,
393.590642087758));
#40707=CARTESIAN_POINT('Ctrl Pts',(-3.34798007341745,-3.31022444115695,
393.511514212298));
#40708=CARTESIAN_POINT('Ctrl Pts',(-4.52144496705717,-1.31266592578101,
393.432386336838));
#40709=CARTESIAN_POINT('Ctrl Pts',(-4.60011779179461,1.00273262859438,393.353258461379));
#40710=CARTESIAN_POINT('Ctrl Pts',(-3.56494924255402,3.07533629394358,393.274130585919));
#40711=CARTESIAN_POINT('Ctrl Pts',(-1.6665880225581,4.40329885266706,393.195002710459));
#40712=CARTESIAN_POINT('Ctrl Pts',(0.635309536488234,4.6650764426406,393.115874834999));
#40713=CARTESIAN_POINT('Ctrl Pts',(2.78337754615093,3.79728401076558,393.03674695954));
#40714=CARTESIAN_POINT('Ctrl Pts',(4.25749736347943,2.01004294053605,392.957619084079));
#40715=CARTESIAN_POINT('Ctrl Pts',(4.70073559740488,-0.263896316995348,
392.87849120862));
#40716=CARTESIAN_POINT('Ctrl Pts',(4.00576954320095,-2.47393750721331,392.79936333316));
#40717=CARTESIAN_POINT('Ctrl Pts',(2.3408735755072,-4.08495622085785,392.7202354577));
#40718=CARTESIAN_POINT('Ctrl Pts',(0.109174330666369,-4.70687129507029,
392.64110758224));
#40719=CARTESIAN_POINT('Ctrl Pts',(-2.14895964736531,-4.18909642486643,
392.561979706781));
#40720=CARTESIAN_POINT('Ctrl Pts',(-3.88675908733054,-2.65700211138166,
392.482851831321));
#40721=CARTESIAN_POINT('Ctrl Pts',(-4.68344499975174,-0.481559297629621,
392.403723955861));
#40722=CARTESIAN_POINT('Ctrl Pts',(-4.34611325228191,1.81048502373608,392.324596080401));
#40723=CARTESIAN_POINT('Ctrl Pts',(-2.95644307012664,3.66415076053556,392.245468204942));
#40724=CARTESIAN_POINT('Ctrl Pts',(-0.850919781515802,4.63060384272486,
392.166340329482));
#40725=CARTESIAN_POINT('Ctrl Pts',(1.46063946127848,4.47583386498977,392.087212454022));
#40726=CARTESIAN_POINT('Ctrl Pts',(3.41852935514023,3.23731578176699,392.008084578562));
#40727=CARTESIAN_POINT('Ctrl Pts',(4.54867969835275,1.21493597552573,391.928956703102));
#40728=CARTESIAN_POINT('Ctrl Pts',(4.57744353923776,-1.10162020130516,391.849828827643));
#40729=CARTESIAN_POINT('Ctrl Pts',(3.4978561961279,-3.1514375218371,391.770700952183));
#40730=CARTESIAN_POINT('Ctrl Pts',(1.57132163822667,-4.43818709971468,391.691573076723));
#40731=CARTESIAN_POINT('Ctrl Pts',(-0.735682101486766,-4.65030410493606,
391.612445201263));
#40732=CARTESIAN_POINT('Ctrl Pts',(-2.86455275856638,-3.73642796213481,
391.533317325804));
#40733=CARTESIAN_POINT('Ctrl Pts',(-4.29982000702773,-1.91783845252855,
391.454189450344));
#40734=CARTESIAN_POINT('Ctrl Pts',(-4.6939579537506,0.36512347398464,391.375061574884));
#40735=CARTESIAN_POINT('Ctrl Pts',(-3.95153270508603,2.55967687481616,391.295933699424));
#40736=CARTESIAN_POINT('Ctrl Pts',(-2.25231008366655,4.13444744915776,391.216805823965));
#40737=CARTESIAN_POINT('Ctrl Pts',(-0.00772834933684394,4.70813091315965,
391.137677948505));
#40738=CARTESIAN_POINT('Ctrl Pts',(2.2387246751714,4.14181943735019,391.058550073045));
#40739=CARTESIAN_POINT('Ctrl Pts',(3.94310806559349,2.572635847897,390.979422197585));
#40740=CARTESIAN_POINT('Ctrl Pts',(4.69273396842282,0.380531633959359,390.900294322126));
#40741=CARTESIAN_POINT('Ctrl Pts',(4.30609304338418,-1.90371193318514,390.821166446665));
#40742=CARTESIAN_POINT('Ctrl Pts',(2.87680390605944,-3.72700358316359,390.742038571206));
#40743=CARTESIAN_POINT('Ctrl Pts',(0.750944950216976,-4.64786382164717,
390.662910695746));
#40744=CARTESIAN_POINT('Ctrl Pts',(-1.55674273110369,-4.4433217857802,390.583782820286));
#40745=CARTESIAN_POINT('Ctrl Pts',(-3.48749126846685,-3.16290389914089,
390.504654944827));
#40746=CARTESIAN_POINT('Ctrl Pts',(-4.57380228443991,-1.11664187888751,
390.425527069367));
#40747=CARTESIAN_POINT('Ctrl Pts',(-4.55264378519931,1.19999624496042,390.346399193907));
#40748=CARTESIAN_POINT('Ctrl Pts',(-3.42913894648368,3.22607540341852,390.267271318447));
#40749=CARTESIAN_POINT('Ctrl Pts',(-1.4753256225101,4.47101450796107,390.188143442987));
#40750=CARTESIAN_POINT('Ctrl Pts',(0.835713058034306,4.63337243349421,390.109015567528));
#40751=CARTESIAN_POINT('Ctrl Pts',(2.94439783745191,3.67383693128064,390.029887692068));
#40752=CARTESIAN_POINT('Ctrl Pts',(4.34014606149365,1.8247434306593,389.950759816608));
#40753=CARTESIAN_POINT('Ctrl Pts',(4.68500070602262,-0.466181088634749,
389.871631941148));
#40754=CARTESIAN_POINT('Ctrl Pts',(3.89546100247805,-2.64422767571286,389.792504065689));
#40755=CARTESIAN_POINT('Ctrl Pts',(2.16270074857769,-4.18201887787879,389.713376190229));
#40756=CARTESIAN_POINT('Ctrl Pts',(-0.0937212205934936,-4.70720434606822,
389.634248314769));
#40757=CARTESIAN_POINT('Ctrl Pts',(-2.32745016801145,-4.09261922712786,
389.555120439309));
#40758=CARTESIAN_POINT('Ctrl Pts',(-3.99762609128131,-2.48707500030459,
389.475992563849));
#40759=CARTESIAN_POINT('Ctrl Pts',(-4.69984390136856,-0.279327273286843,
389.39686468839));
#40760=CARTESIAN_POINT('Ctrl Pts',(-4.26407333256687,1.99605486831531,389.31773681293));
#40761=CARTESIAN_POINT('Ctrl Pts',(-2.79582891973421,3.78812579970769,389.23860893747));
#40762=CARTESIAN_POINT('Ctrl Pts',(-0.650621423278113,4.6629655999594,389.159481062011));
#40763=CARTESIAN_POINT('Ctrl Pts',(1.65212313914968,4.40874648351652,389.08035318655));
#40764=CARTESIAN_POINT('Ctrl Pts',(3.55483379145156,3.08702334587661,389.001225311091));
#40765=CARTESIAN_POINT('Ctrl Pts',(4.59680105983476,1.01782927799078,388.922097435631));
#40766=CARTESIAN_POINT('Ctrl Pts',(4.52573004525854,-1.29781507938429,388.842969560171));
#40767=CARTESIAN_POINT('Ctrl Pts',(3.35882940195932,-3.29921528114894,388.763841684711));
#40768=CARTESIAN_POINT('Ctrl Pts',(1.37864455043625,-4.50176583424611,388.684713809252));
#40769=CARTESIAN_POINT('Ctrl Pts',(-0.935355957508586,-4.61428929040934,
388.605585933792));
#40770=CARTESIAN_POINT('Ctrl Pts',(-3.02287570734582,-3.60953998187742,
388.526458058332));
#40771=CARTESIAN_POINT('Ctrl Pts',(-4.37845680177713,-1.73080110290138,
388.447330182872));
#40772=CARTESIAN_POINT('Ctrl Pts',(-4.67386801345155,0.567022235602428,
388.368202307413));
#40773=CARTESIAN_POINT('Ctrl Pts',(-3.83758047185038,2.72755064937495,388.289074431953));
#40774=CARTESIAN_POINT('Ctrl Pts',(-2.07208717966135,4.22764841758585,388.209946556493));
#40775=CARTESIAN_POINT('Ctrl Pts',(0.19512727177995,4.70409202404044,388.130818681033));
#40776=CARTESIAN_POINT('Ctrl Pts',(2.41509492687017,4.04151863994701,388.051690805573));
#40777=CARTESIAN_POINT('Ctrl Pts',(4.0502878493588,2.40035929814049,387.972562930114));
#40778=CARTESIAN_POINT('Ctrl Pts',(4.7047714971451,0.17799320909573,387.893435054654));
#40779=CARTESIAN_POINT('Ctrl Pts',(4.22007363136663,-2.08747095037925,387.814307179194));
#40780=CARTESIAN_POINT('Ctrl Pts',(2.71355571127686,-3.84748902852625,387.735179303735));
#40781=CARTESIAN_POINT('Ctrl Pts',(0.549995785174607,-4.67590216526428,
387.656051428274));
#40782=CARTESIAN_POINT('Ctrl Pts',(-1.74673639624114,-4.37212401298038,
387.576923552815));
#40783=CARTESIAN_POINT('Ctrl Pts',(-3.62052565410023,-3.00970935653847,
387.497795677355));
#40784=CARTESIAN_POINT('Ctrl Pts',(-4.61766534522889,-0.918544055723703,
387.418667801895));
#40785=CARTESIAN_POINT('Ctrl Pts',(-4.49671481660818,1.39503128313651,387.339539926435));
#40786=CARTESIAN_POINT('Ctrl Pts',(-3.28696021026318,3.37082319307611,387.260412050976));
#40787=CARTESIAN_POINT('Ctrl Pts',(-1.28132331513389,4.53042679942271,387.181284175516));
#40788=CARTESIAN_POINT('Ctrl Pts',(1.03456453147854,4.59306353679543,387.102156300057));
#40789=CARTESIAN_POINT('Ctrl Pts',(3.09994992763925,3.54356696973015,387.023028424596));
#40790=CARTESIAN_POINT('Ctrl Pts',(4.414734438574,1.63605509066836,386.943900549137));
#40791=CARTESIAN_POINT('Ctrl Pts',(4.66056504541948,-0.667600090059401,
386.864772673676));
#40792=CARTESIAN_POINT('Ctrl Pts',(3.77791798959212,-2.80960710540626,386.785644798217));
#40793=CARTESIAN_POINT('Ctrl Pts',(1.9805114526468,-4.27131488054533,386.706516922757));
#40794=CARTESIAN_POINT('Ctrl Pts',(-0.29644271708526,-4.69879539225962,
386.627389047298));
#40795=CARTESIAN_POINT('Ctrl Pts',(-2.50161825456297,-3.98854140398097,
386.548261171838));
#40796=CARTESIAN_POINT('Ctrl Pts',(-4.10106888673475,-2.31252900718875,
386.469133296378));
#40797=CARTESIAN_POINT('Ctrl Pts',(-4.70751446766038,-0.0765764950965269,
386.390005420918));
#40798=CARTESIAN_POINT('Ctrl Pts',(-4.1741143707138,2.17791773100677,386.310877545459));
#40799=CARTESIAN_POINT('Ctrl Pts',(-2.63002248363295,3.90506570475047,386.231749669998));
#40800=CARTESIAN_POINT('Ctrl Pts',(-0.449114760664552,4.68666751056509,
386.152621794539));
#40801=CARTESIAN_POINT('Ctrl Pts',(1.84053856942387,4.33347137954045,386.073493919079));
#40802=CARTESIAN_POINT('Ctrl Pts',(3.68453635289055,2.93099783129588,385.994366043619));
#40803=CARTESIAN_POINT('Ctrl Pts',(4.63638545244831,0.818832314432457,385.915238168159));
#40804=CARTESIAN_POINT('Ctrl Pts',(4.46561157225142,-1.49159971460418,385.8361102927));
#40805=CARTESIAN_POINT('Ctrl Pts',(3.21356474331376,-3.44086588860477,385.75698241724));
#40806=CARTESIAN_POINT('Ctrl Pts',(1.18340710698663,-4.55698409498724,385.67785454178));
#40807=CARTESIAN_POINT('Ctrl Pts',(-1.13329271318905,-4.56970502867152,
385.59872666632));
#40808=CARTESIAN_POINT('Ctrl Pts',(-3.17558470949784,-3.47594852891073,
385.519598790861));
#40809=CARTESIAN_POINT('Ctrl Pts',(-4.44896212663648,-1.54054938855827,
385.440470915401));
#40810=CARTESIAN_POINT('Ctrl Pts',(-4.64509797905953,0.767867949435454,
385.361343039941));
#40811=CARTESIAN_POINT('Ctrl Pts',(-3.71650125952819,2.89035894150857,385.282215164481));
#40812=CARTESIAN_POINT('Ctrl Pts',(-1.88801609003413,4.31299799056357,385.203087289022));
#40813=CARTESIAN_POINT('Ctrl Pts',(0.397620511444409,4.69131691017691,385.123959413562));
#40814=CARTESIAN_POINT('Ctrl Pts',(2.58697997463334,3.93371211881083,385.044831538102));
#40815=CARTESIAN_POINT('Ctrl Pts',(4.14994562361626,2.22362491078451,384.965703662642));
#40816=CARTESIAN_POINT('Ctrl Pts',(4.70807153923669,-0.0248757766222604,
384.886575787182));
#40817=CARTESIAN_POINT('Ctrl Pts',(4.12621689144541,-2.26735321191552,384.807447911723));
#40818=CARTESIAN_POINT('Ctrl Pts',(2.54526802482854,-3.96082909308373,384.728320036263));
#40819=CARTESIAN_POINT('Ctrl Pts',(0.348025193093154,-4.69525663705463,
384.649192160803));
#40820=CARTESIAN_POINT('Ctrl Pts',(-1.93348610236405,-4.29280653125647,
384.570064285343));
#40821=CARTESIAN_POINT('Ctrl Pts',(-3.74683616493588,-2.85092531925369,
384.490936409884));
#40822=CARTESIAN_POINT('Ctrl Pts',(-4.65295268895202,-0.718740354514286,
384.411808534423));
#40823=CARTESIAN_POINT('Ctrl Pts',(-4.43243475474589,1.58747553296225,384.332680658964));
#40824=CARTESIAN_POINT('Ctrl Pts',(-3.1386770817443,3.50931084393592,384.253552783504));
#40825=CARTESIAN_POINT('Ctrl Pts',(-1.08494139264941,4.58142538925924,384.174424908044));
#40826=CARTESIAN_POINT('Ctrl Pts',(1.23149465895138,4.54422461238519,384.095297032584));
#40827=CARTESIAN_POINT('Ctrl Pts',(3.24974493247929,3.40671605753374,384.016169157125));
#40828=CARTESIAN_POINT('Ctrl Pts',(4.48112397259501,1.44432834392579,383.937041281665));
#40829=CARTESIAN_POINT('Ctrl Pts',(4.62747399638768,-0.867779255104094,
383.857913406205));
#40830=CARTESIAN_POINT('Ctrl Pts',(3.65335880005533,-2.96976866117404,383.778785530746));
#40831=CARTESIAN_POINT('Ctrl Pts',(1.79464404134943,-4.35267839240186,383.699657655285));
#40832=CARTESIAN_POINT('Ctrl Pts',(-0.498613673709388,-4.68166005036923,
383.620529779826));
#40833=CARTESIAN_POINT('Ctrl Pts',(-2.6711404500085,-3.87705624400286,383.541401904366));
#40834=CARTESIAN_POINT('Ctrl Pts',(-4.19689536445816,-2.13368829087633,
383.462274028906));
#40835=CARTESIAN_POINT('Ctrl Pts',(-4.70644245320202,0.126316497461169,
383.383146153446));
#40836=CARTESIAN_POINT('Ctrl Pts',(-4.07640343439582,2.35573586441245,383.304018277987));
#40837=CARTESIAN_POINT('Ctrl Pts',(-2.45933168995915,4.01475330021607,383.224890402527));
#40838=CARTESIAN_POINT('Ctrl Pts',(-0.246774022640667,4.70166555643666,
383.145762527067));
#40839=CARTESIAN_POINT('Ctrl Pts',(2.02553583557396,4.25014835054481,383.066634651607));
#40840=CARTESIAN_POINT('Ctrl Pts',(3.80739616178709,2.76952900148059,382.987506776148));
#40841=CARTESIAN_POINT('Ctrl Pts',(4.66735936186835,0.618314652917929,382.908378900688));
#40842=CARTESIAN_POINT('Ctrl Pts',(4.39719976949725,-1.68261421899571,382.829251025228));
#40843=CARTESIAN_POINT('Ctrl Pts',(3.06233199907708,-3.57612627716942,382.750123149768));
#40844=CARTESIAN_POINT('Ctrl Pts',(0.985971893936046,-4.60373933310752,
382.670995274309));
#40845=CARTESIAN_POINT('Ctrl Pts',(-1.32912476943063,-4.51663411957612,
382.591867398849));
#40846=CARTESIAN_POINT('Ctrl Pts',(-3.32239616084197,-3.33590170317647,
382.512739523389));
#40847=CARTESIAN_POINT('Ctrl Pts',(-4.51120504233833,-1.34743663628917,
382.433611647929));
#40848=CARTESIAN_POINT('Ctrl Pts',(-4.6077012809677,0.967287614002028,382.354483772469));
#40849=CARTESIAN_POINT('Ctrl Pts',(-3.58851993089967,3.04779939109664,382.27535589701));
#40850=CARTESIAN_POINT('Ctrl Pts',(-1.70043866320114,4.39033766076413,382.19622802155));
#40851=CARTESIAN_POINT('Ctrl Pts',(0.599375308465022,4.66982929692676,382.11710014609));
#40852=CARTESIAN_POINT('Ctrl Pts',(2.75406060140474,3.81860008728635,382.03797227063));
#40853=CARTESIAN_POINT('Ctrl Pts',(4.24189630850143,2.0427609088572,381.95884439517));
#40854=CARTESIAN_POINT('Ctrl Pts',(4.70262796601022,-0.227698564184567,
381.879716519711));
#40855=CARTESIAN_POINT('Ctrl Pts',(4.02469713006905,-2.44302464867774,381.800588644251));
#40856=CARTESIAN_POINT('Ctrl Pts',(2.37225338291554,-4.06681328684744,381.721460768791));
#40857=CARTESIAN_POINT('Ctrl Pts',(0.145408264526719,-4.70589129277765,
381.642332893331));
#40858=CARTESIAN_POINT('Ctrl Pts',(-2.11664502645219,-4.20551664541093,
381.563205017872));
#40859=CARTESIAN_POINT('Ctrl Pts',(-3.86618822286509,-2.68684667374458,
381.484077142412));
#40860=CARTESIAN_POINT('Ctrl Pts',(-4.67959878156707,-0.517601841562701,
381.404949266952));
#40861=CARTESIAN_POINT('Ctrl Pts',(-4.35992297760592,1.77697159577105,381.325821391492));
#40862=CARTESIAN_POINT('Ctrl Pts',(-2.98456494557718,3.6412811630613,381.246693516033));
#40863=CARTESIAN_POINT('Ctrl Pts',(-0.886544566588966,4.62391556522009,
381.167565640573));
#40864=CARTESIAN_POINT('Ctrl Pts',(1.4261377108192,4.48694636168212,381.088437765113));
#40865=CARTESIAN_POINT('Ctrl Pts',(3.39350465953423,3.26353834795189,381.009309889653));
#40866=CARTESIAN_POINT('Ctrl Pts',(4.53919136794792,1.2499192565843,380.930182014193));
#40867=CARTESIAN_POINT('Ctrl Pts',(4.58578901411133,-1.06634682017112,380.851054138734));
#40868=CARTESIAN_POINT('Ctrl Pts',(3.52201475950248,-3.12441489829372,380.771926263274));
#40869=CARTESIAN_POINT('Ctrl Pts',(1.60544369914822,-4.42595830885227,380.692798387814));
#40870=CARTESIAN_POINT('Ctrl Pts',(-0.699858627803908,-4.65583014337095,
380.613670512354));
#40871=CARTESIAN_POINT('Ctrl Pts',(-2.83570192547335,-3.75837079233806,
380.534542636895));
#40872=CARTESIAN_POINT('Ctrl Pts',(-4.28492755989611,-1.95088498617316,
380.455414761435));
#40873=CARTESIAN_POINT('Ctrl Pts',(-4.69662984888973,0.32897490079206,380.376286885975));
#40874=CARTESIAN_POINT('Ctrl Pts',(-3.97112198789876,2.52917903282076,380.297159010515));
#40875=CARTESIAN_POINT('Ctrl Pts',(-2.28407353785474,4.11698487931458,380.218031135056));
#40876=CARTESIAN_POINT('Ctrl Pts',(-0.0439749871787381,4.70793188388869,
380.138903259595));
#40877=CARTESIAN_POINT('Ctrl Pts',(2.20677136913111,4.15893214025144,380.059775384136));
#40878=CARTESIAN_POINT('Ctrl Pts',(3.92318504851847,2.60291672896277,379.980647508676));
#40879=CARTESIAN_POINT('Ctrl Pts',(4.68966526476571,0.416648685685039,379.901519633216));
#40880=CARTESIAN_POINT('Ctrl Pts',(4.32062168826984,-1.8705038491501,379.822391757756));
#40881=CARTESIAN_POINT('Ctrl Pts',(2.90541203179102,-3.70474524743025,379.743263882297));
#40882=CARTESIAN_POINT('Ctrl Pts',(0.786705578939987,-4.64194471691529,
379.664136006837));
#40883=CARTESIAN_POINT('Ctrl Pts',(-1.52248843588733,-4.45517512399035,
379.585008131377));
#40884=CARTESIAN_POINT('Ctrl Pts',(-3.46303740985959,-3.18965959323972,
379.505880255917));
#40885=CARTESIAN_POINT('Ctrl Pts',(-4.56506995418396,-1.15182148627296,
379.426752380458));
#40886=CARTESIAN_POINT('Ctrl Pts',(-4.56174737061485,1.16491087621397,379.347624504998));
#40887=CARTESIAN_POINT('Ctrl Pts',(-3.45387416703998,3.19957960693074,379.268496629538));
#40888=CARTESIAN_POINT('Ctrl Pts',(-1.50970325938777,4.45952379648624,379.189368754078));
#40889=CARTESIAN_POINT('Ctrl Pts',(0.800016973052387,4.63966909010343,379.110240878619));
#40890=CARTESIAN_POINT('Ctrl Pts',(2.91602651267941,3.69639632617822,379.031113003159));
#40891=CARTESIAN_POINT('Ctrl Pts',(4.32596913740423,1.85810318471799,378.951985127699));
#40892=CARTESIAN_POINT('Ctrl Pts',(4.68845088702114,-0.430098480378534,
378.872857252239));
#40893=CARTESIAN_POINT('Ctrl Pts',(3.91570288509923,-2.61415901170123,378.79372937678));
#40894=CARTESIAN_POINT('Ctrl Pts',(2.19483310042462,-4.16524478081583,378.714601501319));
#40895=CARTESIAN_POINT('Ctrl Pts',(-0.0574787096237898,-4.70778638223669,
378.63547362586));
#40896=CARTESIAN_POINT('Ctrl Pts',(-2.29587301412136,-4.11041646623094,
378.5563457504));
#40897=CARTESIAN_POINT('Ctrl Pts',(-3.97836017269986,-2.5177781393738,378.47721787494));
#40898=CARTESIAN_POINT('Ctrl Pts',(-4.69755413716848,-0.315502062123824,
378.398089999481));
#40899=CARTESIAN_POINT('Ctrl Pts',(-4.27931415074721,1.96316754813432,378.318962124021));
#40900=CARTESIAN_POINT('Ctrl Pts',(-2.82491001177881,3.76648906120608,378.239834248561));
#40901=CARTESIAN_POINT('Ctrl Pts',(-0.686501290471962,4.65781841649216,
378.160706373101));
#40902=CARTESIAN_POINT('Ctrl Pts',(1.61813220490064,4.421335159236,378.081578497641));
#40903=CARTESIAN_POINT('Ctrl Pts',(3.5309621248084,3.11429974408401,378.002450622182));
#40904=CARTESIAN_POINT('Ctrl Pts',(4.58882878451957,1.05318887631696,377.923322746722));
#40905=CARTESIAN_POINT('Ctrl Pts',(4.53558751403461,-1.26293401465255,377.844194871262));
#40906=CARTESIAN_POINT('Ctrl Pts',(3.38412979408371,-3.27325861484057,377.765066995802));
#40907=CARTESIAN_POINT('Ctrl Pts',(1.41326180027294,-4.49101853778431,377.685939120342));
#40908=CARTESIAN_POINT('Ctrl Pts',(-0.899803836436171,-4.62135364138776,
377.606811244883));
#40909=CARTESIAN_POINT('Ctrl Pts',(-2.99499706490511,-3.63270546618397,
377.527683369423));
#40910=CARTESIAN_POINT('Ctrl Pts',(-4.36500198367802,-1.76445858702323,
377.448555493963));
#40911=CARTESIAN_POINT('Ctrl Pts',(-4.67809487824384,0.531022346970404,
377.369427618503));
#40912=CARTESIAN_POINT('Ctrl Pts',(-3.858465555114,2.69792512550514,377.290299743043));
#40913=CARTESIAN_POINT('Ctrl Pts',(-2.10457350875104,4.21157058222897,377.211171867584));
#40914=CARTESIAN_POINT('Ctrl Pts',(0.158905716619817,4.70545485538416,377.132043992124));
#40915=CARTESIAN_POINT('Ctrl Pts',(2.38390858774424,4.05999215123785,377.052916116664));
#40916=CARTESIAN_POINT('Ctrl Pts',(4.03168797525527,2.43147043844132,376.973788241204));
#40917=CARTESIAN_POINT('Ctrl Pts',(4.70326173563702,0.21420893755303,376.894660365745));
#40918=CARTESIAN_POINT('Ctrl Pts',(4.23601954588194,-2.0549196650327,376.815532490285));
#40919=CARTESIAN_POINT('Ctrl Pts',(2.74309626604883,-3.82648393411214,376.736404614825));
#40920=CARTESIAN_POINT('Ctrl Pts',(0.585978230290955,-4.67152929311995,
376.657276739365));
#40921=CARTESIAN_POINT('Ctrl Pts',(-1.71302460639056,-4.38544218074737,
376.578148863906));
#40922=CARTESIAN_POINT('Ctrl Pts',(-3.59724726405772,-3.03749379327437,
376.499020988446));
#40923=CARTESIAN_POINT('Ctrl Pts',(-4.61045682670426,-0.954067226005277,
376.419893112986));
#40924=CARTESIAN_POINT('Ctrl Pts',(-4.50732159153776,1.36037071913331,376.340765237526));
#40925=CARTESIAN_POINT('Ctrl Pts',(-3.31281402583599,3.34541770982772,376.261637362067));
#40926=CARTESIAN_POINT('Ctrl Pts',(-1.31616410382415,4.52042790819332,376.182509486607));
#40927=CARTESIAN_POINT('Ctrl Pts',(0.999172883001983,4.60089230230265,376.103381611147));
#40928=CARTESIAN_POINT('Ctrl Pts',(3.07257691207793,3.5673277858007,376.024253735687));
#40929=CARTESIAN_POINT('Ctrl Pts',(4.40200797556968,1.66999467821426,375.945125860228));
#40930=CARTESIAN_POINT('Ctrl Pts',(4.66556662820138,-0.631699641477607,
375.865997984767));
#40931=CARTESIAN_POINT('Ctrl Pts',(3.79943658220811,-2.78043846928895,375.786870109308));
#40932=CARTESIAN_POINT('Ctrl Pts',(2.01333666035538,-4.25594079109181,375.707742233848));
#40933=CARTESIAN_POINT('Ctrl Pts',(-0.260258907652536,-4.70093834665202,
375.628614358388));
#40934=CARTESIAN_POINT('Ctrl Pts',(-2.47083727331916,-4.00768269259632,
375.549486482929));
#40935=CARTESIAN_POINT('Ctrl Pts',(-4.08314356267804,-2.34403352650038,
375.470358607469));
#40936=CARTESIAN_POINT('Ctrl Pts',(-4.70678568739368,-0.112816719080636,
375.391230732009));
#40937=CARTESIAN_POINT('Ctrl Pts',(-4.19075739000426,2.14571838351356,375.312102856549));
#40938=CARTESIAN_POINT('Ctrl Pts',(-2.66001002678919,3.8847003407523,375.232974981089));
#40939=CARTESIAN_POINT('Ctrl Pts',(-0.48518044668226,4.68307451075752,375.153847105629));
#40940=CARTESIAN_POINT('Ctrl Pts',(1.80711601134657,4.34750540330396,375.07471923017));
#40941=CARTESIAN_POINT('Ctrl Pts',(3.66187380043387,2.9592933100083,374.99559135471));
#40942=CARTESIAN_POINT('Ctrl Pts',(4.62991897355734,0.854469882696709,374.91646347925));
#40943=CARTESIAN_POINT('Ctrl Pts',(4.477014386818,-1.45709927207541,374.837335603791));
#40944=CARTESIAN_POINT('Ctrl Pts',(3.23983968516725,-3.41613747848395,374.758207728331));
#40945=CARTESIAN_POINT('Ctrl Pts',(1.8923805371004,-4.17007422695688,374.705455811358));
#40946=CARTESIAN_POINT('Ctrl Pts',(1.16918346556986,-4.36383719750612,374.679079852871));
#40947=CARTESIAN_POINT('Ctrl Pts',(3.57461543774233,3.05624720968358,400.106973382376));
#40948=CARTESIAN_POINT('Ctrl Pts',(4.0811121130032,2.46384394177512,400.08059742389));
#40949=CARTESIAN_POINT('Ctrl Pts',(4.79330604666853,1.02286901533234,400.027845506917));
#40950=CARTESIAN_POINT('Ctrl Pts',(4.70079893715141,-1.38736907251624,399.948717631457));
#40951=CARTESIAN_POINT('Ctrl Pts',(3.47003520682193,-3.46129852254691,399.869589755997));
#40952=CARTESIAN_POINT('Ctrl Pts',(1.39906460383401,-4.69732448980706,399.790461880537));
#40953=CARTESIAN_POINT('Ctrl Pts',(-1.01066992750072,-4.79588345555735,
399.711334005077));
#40954=CARTESIAN_POINT('Ctrl Pts',(-3.17568611614676,-3.73324183578399,
399.632206129617));
#40955=CARTESIAN_POINT('Ctrl Pts',(-4.57176395161188,-1.76663842906183,
399.553078254158));
#40956=CARTESIAN_POINT('Ctrl Pts',(-4.86086545663507,0.627717441216646,
399.473950378698));
#40957=CARTESIAN_POINT('Ctrl Pts',(-3.97299008611081,2.8700865038691,399.394822503238));
#40958=CARTESIAN_POINT('Ctrl Pts',(-2.12312171649347,4.41751015439781,399.315694627778));
#40959=CARTESIAN_POINT('Ctrl Pts',(0.240824931085231,4.89530880016116,399.236566752319));
#40960=CARTESIAN_POINT('Ctrl Pts',(2.54645987869621,4.18779005099161,399.157438876859));
#40961=CARTESIAN_POINT('Ctrl Pts',(4.23551226517086,2.46626839669468,399.078311001399));
#40962=CARTESIAN_POINT('Ctrl Pts',(4.89900639514296,0.147581107578247,398.999183125939));
#40963=CARTESIAN_POINT('Ctrl Pts',(4.37628828662539,-2.20684042213451,398.920055250479));
#40964=CARTESIAN_POINT('Ctrl Pts',(2.79392536583327,-4.02691257828985,398.84092737502));
#40965=CARTESIAN_POINT('Ctrl Pts',(0.53506027464146,-4.87193537854724,398.76179949956));
#40966=CARTESIAN_POINT('Ctrl Pts',(-1.85336068827152,-4.53730074011451,
398.6826716241));
#40967=CARTESIAN_POINT('Ctrl Pts',(-3.7930214436213,-3.10403482078447,398.60354374864));
#40968=CARTESIAN_POINT('Ctrl Pts',(-4.81426566971713,-0.919178929028494,
398.524415873181));
#40969=CARTESIAN_POINT('Ctrl Pts',(-4.6698162047254,1.48824072524753,398.445287997721));
#40970=CARTESIAN_POINT('Ctrl Pts',(-3.39464906397748,3.53530784716552,398.366160122261));
#40971=CARTESIAN_POINT('Ctrl Pts',(-1.29752458459001,4.7263594652241,398.287032246801));
#40972=CARTESIAN_POINT('Ctrl Pts',(1.1137737119676,4.77300240524464,398.207904371341));
#40973=CARTESIAN_POINT('Ctrl Pts',(3.25539038344674,3.66394286164299,398.128776495882));
#40974=CARTESIAN_POINT('Ctrl Pts',(4.60876887024317,1.66772100264832,398.049648620422));
#40975=CARTESIAN_POINT('Ctrl Pts',(4.84621126950363,-0.732311527518088,
397.970520744962));
#40976=CARTESIAN_POINT('Ctrl Pts',(3.91022488643166,-2.95502710301166,397.891392869503));
#40977=CARTESIAN_POINT('Ctrl Pts',(2.02744312611193,-4.46223242473778,397.812264994043));
#40978=CARTESIAN_POINT('Ctrl Pts',(-0.346249984625578,-4.88898300162196,
397.733137118583));
#40979=CARTESIAN_POINT('Ctrl Pts',(-2.63610446859942,-4.13194833857237,
397.654009243123));
#40980=CARTESIAN_POINT('Ctrl Pts',(-4.28767046602801,-2.3744316828985,397.574881367663));
#40981=CARTESIAN_POINT('Ctrl Pts',(-4.90104896930931,-0.0419862171810207,
397.495753492204));
#40982=CARTESIAN_POINT('Ctrl Pts',(-4.3277206609419,2.30062550686931,397.416625616744));
#40983=CARTESIAN_POINT('Ctrl Pts',(-2.70650737541695,4.08617934858649,397.337497741284));
#40984=CARTESIAN_POINT('Ctrl Pts',(-0.429958720199221,4.88233339100534,
397.258369865824));
#40985=CARTESIAN_POINT('Ctrl Pts',(1.95069722820886,4.49631228517985,397.179241990364));
#40986=CARTESIAN_POINT('Ctrl Pts',(3.85902455825875,3.0215845678645,397.100114114904));
#40987=CARTESIAN_POINT('Ctrl Pts',(4.83295381183918,0.815230822914742,397.020986239445));
#40988=CARTESIAN_POINT('Ctrl Pts',(4.63666435411759,-1.58851739343839,396.941858363985));
#40989=CARTESIAN_POINT('Ctrl Pts',(3.31768438527967,-3.60763276424756,396.862730488525));
#40990=CARTESIAN_POINT('Ctrl Pts',(1.19538278395727,-4.75322036537541,396.783602613066));
#40991=CARTESIAN_POINT('Ctrl Pts',(-1.21636071054614,-4.7478953720402,396.704474737606));
#40992=CARTESIAN_POINT('Ctrl Pts',(-3.33358285876919,-3.59294714207171,
396.625346862146));
#40993=CARTESIAN_POINT('Ctrl Pts',(-4.64363382578808,-1.5680270195369,396.546218986686));
#40994=CARTESIAN_POINT('Ctrl Pts',(-4.82930674101173,0.836564548148951,
396.467091111227));
#40995=CARTESIAN_POINT('Ctrl Pts',(-3.84564402196864,3.03859604065724,396.387963235766));
#40996=CARTESIAN_POINT('Ctrl Pts',(-1.93082309891163,4.50488246269648,396.308835360307));
#40997=CARTESIAN_POINT('Ctrl Pts',(0.451514255406424,4.88038714849199,396.229707484847));
#40998=CARTESIAN_POINT('Ctrl Pts',(2.724525005195,4.07418793602703,396.150579609387));
#40999=CARTESIAN_POINT('Ctrl Pts',(4.33783771841656,2.28149244370514,396.071451733927));
#41000=CARTESIAN_POINT('Ctrl Pts',(4.90081577868788,-0.063628180588346,
395.992323858468));
#41001=CARTESIAN_POINT('Ctrl Pts',(4.27714349050859,-2.39334230807068,395.913195983008));
#41002=CARTESIAN_POINT('Ctrl Pts',(2.61783263875445,-4.14354873477711,395.834068107548));
#41003=CARTESIAN_POINT('Ctrl Pts',(0.324657517612272,-4.89046432747023,
395.754940232088));
#41004=CARTESIAN_POINT('Ctrl Pts',(-2.04712797653699,-4.45323600201927,
395.675812356629));
#41005=CARTESIAN_POINT('Ctrl Pts',(-3.92323576387579,-2.93773126460658,
395.596684481169));
#41006=CARTESIAN_POINT('Ctrl Pts',(-4.84939780820125,-0.710904170626361,
395.517556605709));
#41007=CARTESIAN_POINT('Ctrl Pts',(-4.6013595032905,1.68805644558445,395.438428730249));
#41008=CARTESIAN_POINT('Ctrl Pts',(-3.23917916478794,3.67828250415935,395.35930085479));
#41009=CARTESIAN_POINT('Ctrl Pts',(-1.09268591631945,4.77787414341129,395.28017297933));
#41010=CARTESIAN_POINT('Ctrl Pts',(1.31838290117699,4.72058368932118,395.20104510387));
#41011=CARTESIAN_POINT('Ctrl Pts',(3.41022740996214,3.52028306451966,395.12191722841));
#41012=CARTESIAN_POINT('Ctrl Pts',(4.6763425448897,1.46760493487027,395.04278935295));
#41013=CARTESIAN_POINT('Ctrl Pts',(4.81015976025467,-0.940429116322842,
394.963661477491));
#41014=CARTESIAN_POINT('Ctrl Pts',(3.77927746162617,-3.12075402908423,394.884533602031));
#41015=CARTESIAN_POINT('Ctrl Pts',(1.83330650852657,-4.54544069236363,394.805405726571));
#41016=CARTESIAN_POINT('Ctrl Pts',(-0.556568868938532,-4.8695251242939,
394.726277851111));
#41017=CARTESIAN_POINT('Ctrl Pts',(-2.81168042909494,-4.01453571495453,
394.647149975651));
#41018=CARTESIAN_POINT('Ctrl Pts',(-4.3859907284844,-2.18749381065409,394.568022100192));
#41019=CARTESIAN_POINT('Ctrl Pts',(-4.89830693111745,0.169213033090633,
394.488894224732));
#41020=CARTESIAN_POINT('Ctrl Pts',(-4.2245802606628,2.48494777877106,394.409766349272));
#41021=CARTESIAN_POINT('Ctrl Pts',(-2.52794233119419,4.19899409527539,394.330638473813));
#41022=CARTESIAN_POINT('Ctrl Pts',(-0.219205562748669,4.89632441360466,
394.251510598353));
#41023=CARTESIAN_POINT('Ctrl Pts',(2.14260815638517,4.40809189221286,394.172382722893));
#41024=CARTESIAN_POINT('Ctrl Pts',(3.98562524447155,2.85251384792995,394.093254847433));
#41025=CARTESIAN_POINT('Ctrl Pts',(4.86359002316223,0.606247415332937,394.014126971973));
#41026=CARTESIAN_POINT('Ctrl Pts',(4.56391804578379,-1.78681166141541,393.934999096514));
#41027=CARTESIAN_POINT('Ctrl Pts',(3.15916985581216,-3.74722426125376,393.855871221054));
#41028=CARTESIAN_POINT('Ctrl Pts',(0.989481668194294,-4.80030935152189,
393.776743345594));
#41029=CARTESIAN_POINT('Ctrl Pts',(-1.41979291062284,-4.69108003906842,
393.697615470134));
#41030=CARTESIAN_POINT('Ctrl Pts',(-3.48528844770473,-3.44598437000184,
393.618487594675));
#41031=CARTESIAN_POINT('Ctrl Pts',(-4.70687983950021,-1.3665013788897,393.539359719215));
#41032=CARTESIAN_POINT('Ctrl Pts',(-4.788779217989,1.04385700330924,393.460231843755));
#41033=CARTESIAN_POINT('Ctrl Pts',(-3.71115602221747,3.2014629188482,393.381103968295));
#41034=CARTESIAN_POINT('Ctrl Pts',(-1.7349386360522,4.58388828083041,393.301976092836));
#41035=CARTESIAN_POINT('Ctrl Pts',(0.661365043902099,4.85640197272687,393.222848217375));
#41036=CARTESIAN_POINT('Ctrl Pts',(2.89753027033354,3.95301937441519,393.143720341916));
#41037=CARTESIAN_POINT('Ctrl Pts',(4.43210713674341,2.09247943130372,393.064592466456));
#41038=CARTESIAN_POINT('Ctrl Pts',(4.89352359156256,-0.27471931279354,392.985464590996));
#41039=CARTESIAN_POINT('Ctrl Pts',(4.17005537874506,-2.57539938265902,392.906336715536));
#41040=CARTESIAN_POINT('Ctrl Pts',(2.43687819262455,-4.2524896844451,392.827208840076));
#41041=CARTESIAN_POINT('Ctrl Pts',(0.113651821430644,-4.89991092832171,
392.748080964617));
#41042=CARTESIAN_POINT('Ctrl Pts',(-2.23709343224997,-4.3609009180885,392.668953089157));
#41043=CARTESIAN_POINT('Ctrl Pts',(-4.04616402995999,-2.76597188790106,
392.589825213697));
#41044=CARTESIAN_POINT('Ctrl Pts',(-4.87552386667384,-0.501309153611575,
392.510697338238));
#41045=CARTESIAN_POINT('Ctrl Pts',(-4.52435736725662,1.88473718468963,392.431569462777));
#41046=CARTESIAN_POINT('Ctrl Pts',(-3.07769361007314,3.81442602294447,392.352441587318));
#41047=CARTESIAN_POINT('Ctrl Pts',(-0.885817961698088,4.82051557208708,
392.273313711858));
#41048=CARTESIAN_POINT('Ctrl Pts',(1.52054364990864,4.65939812107997,392.194185836399));
#41049=CARTESIAN_POINT('Ctrl Pts',(3.55873111796869,3.37008555855818,392.115057960939));
#41050=CARTESIAN_POINT('Ctrl Pts',(4.73523152985659,1.2647632982709,392.035930085479));
#41051=CARTESIAN_POINT('Ctrl Pts',(4.76517504210868,-1.14680018314682,391.956802210019));
#41052=CARTESIAN_POINT('Ctrl Pts',(3.64131133542052,-3.28068523338327,391.877674334559));
#41053=CARTESIAN_POINT('Ctrl Pts',(1.63576515787017,-4.62020737524832,391.7985464591));
#41054=CARTESIAN_POINT('Ctrl Pts',(-0.765854118981568,-4.84102378742762,
391.71941858364));
#41055=CARTESIAN_POINT('Ctrl Pts',(-2.98203466518281,-3.88966747905899,
391.64029070818));
#41056=CARTESIAN_POINT('Ctrl Pts',(-4.47616552938631,-1.99649342486641,
391.56116283272));
#41057=CARTESIAN_POINT('Ctrl Pts',(-4.88646798113091,0.380098028649711,
391.482034957261));
#41058=CARTESIAN_POINT('Ctrl Pts',(-4.11359416297415,2.66465511921264,391.402907081801));
#41059=CARTESIAN_POINT('Ctrl Pts',(-2.34468250799326,4.30401066201183,391.323779206341));
#41060=CARTESIAN_POINT('Ctrl Pts',(-0.00804530674402572,4.90122220625023,
391.244651330881));
#41061=CARTESIAN_POINT('Ctrl Pts',(2.33053993060416,4.31168499242009,391.165523455421));
#41062=CARTESIAN_POINT('Ctrl Pts',(4.10482400961136,2.67814556962822,391.086395579962));
#41063=CARTESIAN_POINT('Ctrl Pts',(4.88519379734561,0.396138112754947,391.007267704502));
#41064=CARTESIAN_POINT('Ctrl Pts',(4.48269583741255,-1.98178754442679,390.928139829042));
#41065=CARTESIAN_POINT('Ctrl Pts',(2.99478826045289,-3.87985658459878,390.849011953582));
#41066=CARTESIAN_POINT('Ctrl Pts',(0.781742932293461,-4.8384834225003,390.769884078122));
#41067=CARTESIAN_POINT('Ctrl Pts',(-1.62058833618616,-4.62555264661623,
390.690756202663));
#41068=CARTESIAN_POINT('Ctrl Pts',(-3.63052131820232,-3.29262187323105,
390.611628327203));
#41069=CARTESIAN_POINT('Ctrl Pts',(-4.76138445106458,-1.16243793432658,
390.532500451743));
#41070=CARTESIAN_POINT('Ctrl Pts',(-4.7393581930353,1.24921085494409,390.453372576283));
#41071=CARTESIAN_POINT('Ctrl Pts',(-3.56977583309043,3.35838418640342,390.374244700824));
#41072=CARTESIAN_POINT('Ctrl Pts',(-1.53583212443933,4.65438111111899,390.295116825364));
#41073=CARTESIAN_POINT('Ctrl Pts',(0.869987575460632,4.82339770914085,390.215988949904));
#41074=CARTESIAN_POINT('Ctrl Pts',(3.06515437466237,3.82450944586218,390.136861074444));
#41075=CARTESIAN_POINT('Ctrl Pts',(4.51814544822977,1.89958036172247,390.057733198985));
#41076=CARTESIAN_POINT('Ctrl Pts',(4.87714337604219,-0.485300248844855,
389.978605323525));
#41077=CARTESIAN_POINT('Ctrl Pts',(4.05522283069102,-2.75267354320184,389.899477448065));
#41078=CARTESIAN_POINT('Ctrl Pts',(2.25139808767325,-4.35353310459702,389.820349572605));
#41079=CARTESIAN_POINT('Ctrl Pts',(-0.0975649437201896,-4.9002576385082,
389.741221697145));
#41080=CARTESIAN_POINT('Ctrl Pts',(-2.42290426026896,-4.26046696825261,
389.662093821685));
#41081=CARTESIAN_POINT('Ctrl Pts',(-4.16157794510521,-2.58907567460185,
389.582965946226));
#41082=CARTESIAN_POINT('Ctrl Pts',(-4.89259532501792,-0.290783128145012,
389.503838070766));
#41083=CARTESIAN_POINT('Ctrl Pts',(-4.43895280146969,2.07791767602217,389.424710195306));
#41084=CARTESIAN_POINT('Ctrl Pts',(-2.91049230342699,3.9434855640275,389.345582319846));
#41085=CARTESIAN_POINT('Ctrl Pts',(-0.67730490643744,4.85420455952536,389.266454444387));
#41086=CARTESIAN_POINT('Ctrl Pts',(1.71988051445791,4.58955933156866,389.187326568927));
#41087=CARTESIAN_POINT('Ctrl Pts',(3.70062571316616,3.21362928370005,389.108198693467));
#41088=CARTESIAN_POINT('Ctrl Pts',(4.78532645921196,1.05957280106983,389.029070818007));
#41089=CARTESIAN_POINT('Ctrl Pts',(4.71134065862855,-1.35104146507597,388.949942942548));
#41090=CARTESIAN_POINT('Ctrl Pts',(3.49658273219959,-3.43452369898426,388.870815067087));
#41091=CARTESIAN_POINT('Ctrl Pts',(1.43518593891208,-4.68639362012519,388.791687191628));
#41092=CARTESIAN_POINT('Ctrl Pts',(-0.973717059752046,-4.80353192240344,
388.712559316168));
#41093=CARTESIAN_POINT('Ctrl Pts',(-3.14685080276043,-3.75757553046736,
388.633431440709));
#41094=CARTESIAN_POINT('Ctrl Pts',(-4.55802740021425,-1.80178524272377,
388.554303565248));
#41095=CARTESIAN_POINT('Ctrl Pts',(-4.8655541061066,0.590277123519319,388.475175689789));
#41096=CARTESIAN_POINT('Ctrl Pts',(-3.9949684861848,2.83941378393346,388.396047814329));
#41097=CARTESIAN_POINT('Ctrl Pts',(-2.15706824758342,4.401034016827,388.316919938869));
#41098=CARTESIAN_POINT('Ctrl Pts',(0.2031298906366,4.89701767298537,388.237792063409));
#41099=CARTESIAN_POINT('Ctrl Pts',(2.51414353256258,4.20727062829036,388.15866418795));
#41100=CARTESIAN_POINT('Ctrl Pts',(4.21639948317845,2.49880356175781,388.07953631249));
#41101=CARTESIAN_POINT('Ctrl Pts',(4.8977250128471,0.185293120576435,388.00040843703));
#41102=CARTESIAN_POINT('Ctrl Pts',(4.39314857117775,-2.17308294217223,387.92128056157));
#41103=CARTESIAN_POINT('Ctrl Pts',(2.82484488118912,-4.00528341559255,387.842152686111));
#41104=CARTESIAN_POINT('Ctrl Pts',(0.572552379142054,-4.86767168317048,
387.763024810651));
#41105=CARTESIAN_POINT('Ctrl Pts',(-1.8183740791475,-4.55143488916249,387.683896935191));
#41106=CARTESIAN_POINT('Ctrl Pts',(-3.76901175041157,-3.13314446958014,
387.604769059731));
#41107=CARTESIAN_POINT('Ctrl Pts',(-4.80704643700727,-0.956215663151738,
387.525641184272));
#41108=CARTESIAN_POINT('Ctrl Pts',(-4.68113544861982,1.45224472926429,387.446513308812));
#41109=CARTESIAN_POINT('Ctrl Pts',(-3.4217660194141,3.50906841631565,387.367385433352));
#41110=CARTESIAN_POINT('Ctrl Pts',(-1.33387333558782,4.71623003749912,387.288257557892));
#41111=CARTESIAN_POINT('Ctrl Pts',(1.07699440584981,4.78143565174407,387.209129682432));
#41112=CARTESIAN_POINT('Ctrl Pts',(3.22708601435485,3.68889681313483,387.130001806972));
#41113=CARTESIAN_POINT('Ctrl Pts',(4.59579286645524,1.70315347829848,387.050873931513));
#41114=CARTESIAN_POINT('Ctrl Pts',(4.85170555271451,-0.694979907450764,
386.971746056053));
#41115=CARTESIAN_POINT('Ctrl Pts',(3.93285910810722,-2.92483556422906,386.892618180594));
#41116=CARTESIAN_POINT('Ctrl Pts',(2.06173678907561,-4.44649134201037,386.813490305133));
#41117=CARTESIAN_POINT('Ctrl Pts',(-0.308600515715983,-4.89150381413537,
386.734362429674));
#41118=CARTESIAN_POINT('Ctrl Pts',(-2.60421538121517,-4.15212067385372,
386.655234554214));
#41119=CARTESIAN_POINT('Ctrl Pts',(-4.26926316786226,-2.40737114827269,
386.576106678754));
#41120=CARTESIAN_POINT('Ctrl Pts',(-4.90058047890116,-0.0797170735407659,
386.496978803294));
#41121=CARTESIAN_POINT('Ctrl Pts',(-4.34530441538657,2.26723915360136,386.417850927834));
#41122=CARTESIAN_POINT('Ctrl Pts',(-2.7378857634756,4.06522144392636,386.338723052375));
#41123=CARTESIAN_POINT('Ctrl Pts',(-0.46753399145535,4.87887854007813,386.259595176915));
#41124=CARTESIAN_POINT('Ctrl Pts',(1.91602329550907,4.51119702219572,386.180467301455));
#41125=CARTESIAN_POINT('Ctrl Pts',(3.83564767539653,3.05120480338935,386.101339425996));
#41126=CARTESIAN_POINT('Ctrl Pts',(4.82653429894221,0.852414513681883,386.022211550536));
#41127=CARTESIAN_POINT('Ctrl Pts',(4.6487565885712,-1.55277365453466,385.943083675076));
#41128=CARTESIAN_POINT('Ctrl Pts',(3.34536043531169,-3.58198372411883,385.863955799616));
#41129=CARTESIAN_POINT('Ctrl Pts',(1.23194135821188,-4.74387650892475,385.784827924157));
#41130=CARTESIAN_POINT('Ctrl Pts',(-1.17977165769507,-4.75711915739983,
385.705700048696));
#41131=CARTESIAN_POINT('Ctrl Pts',(-3.30582275282872,-3.61850518431036,
385.626572173237));
#41132=CARTESIAN_POINT('Ctrl Pts',(-4.63142431084255,-1.60373086736447,
385.547444297777));
#41133=CARTESIAN_POINT('Ctrl Pts',(-4.8356041463375,0.799359982689007,385.468316422318));
#41134=CARTESIAN_POINT('Ctrl Pts',(-3.86892353648086,3.00889921912741,385.389188546857));
#41135=CARTESIAN_POINT('Ctrl Pts',(-1.96544797859558,4.48988397238009,385.310060671398));
#41136=CARTESIAN_POINT('Ctrl Pts',(0.413927844466849,4.88371862227708,385.230932795938));
#41137=CARTESIAN_POINT('Ctrl Pts',(2.69307798204115,4.09504271340925,385.151804920478));
#41138=CARTESIAN_POINT('Ctrl Pts',(4.32014445230215,2.31482089010014,385.072677045018));
#41139=CARTESIAN_POINT('Ctrl Pts',(4.90116039726593,-0.0258959895184648,
384.993549169559));
#41140=CARTESIAN_POINT('Ctrl Pts',(4.29544255017007,-2.3603425895809,384.914421294099));
#41141=CARTESIAN_POINT('Ctrl Pts',(2.6496553290988,-4.12327181725621,384.835293418639));
#41142=CARTESIAN_POINT('Ctrl Pts',(0.362298507876016,-4.88781992642853,
384.756165543179));
#41143=CARTESIAN_POINT('Ctrl Pts',(-2.01278282086323,-4.46886441481938,
384.67703766772));
#41144=CARTESIAN_POINT('Ctrl Pts',(-3.90050254623037,-2.96784833319553,
384.59790979226));
#41145=CARTESIAN_POINT('Ctrl Pts',(-4.84378099597461,-0.748217551943446,
384.5187819168));
#41146=CARTESIAN_POINT('Ctrl Pts',(-4.61421911336287,1.65258156103648,384.43965404134));
#41147=CARTESIAN_POINT('Ctrl Pts',(-3.26740145825086,3.65323576471889,384.36052616588));
#41148=CARTESIAN_POINT('Ctrl Pts',(-1.12943733813143,4.76932019697102,384.281398290421));
#41149=CARTESIAN_POINT('Ctrl Pts',(1.28200109144381,4.730593730552,384.202270414961));
#41150=CARTESIAN_POINT('Ctrl Pts',(3.38302445736953,3.54643332981752,384.123142539501));
#41151=CARTESIAN_POINT('Ctrl Pts',(4.66490518818293,1.50356357606356,384.044014664042));
#41152=CARTESIAN_POINT('Ctrl Pts',(4.81725736354257,-0.903368881131035,
383.964886788581));
#41153=CARTESIAN_POINT('Ctrl Pts',(3.80319145930759,-3.09156571430251,383.885758913122));
#41154=CARTESIAN_POINT('Ctrl Pts',(1.86824652712842,-4.53119175889452,383.806631037662));
#41155=CARTESIAN_POINT('Ctrl Pts',(-0.519062968936094,-4.87366571240583,
383.727503162202));
#41156=CARTESIAN_POINT('Ctrl Pts',(-2.78069007236013,-4.03606325067867,
383.648375286742));
#41157=CARTESIAN_POINT('Ctrl Pts',(-4.36901971015636,-2.22119576225652,
383.569247411283));
#41158=CARTESIAN_POINT('Ctrl Pts',(-4.89946449866066,0.131497027969629,
383.490119535823));
#41159=CARTESIAN_POINT('Ctrl Pts',(-4.24358612851044,2.45235001823044,383.410991660363));
#41160=CARTESIAN_POINT('Ctrl Pts',(-2.56019454719736,4.17940758032786,383.331863784903));
#41161=CARTESIAN_POINT('Ctrl Pts',(-0.256894793709217,4.89449169035623,
383.252735909444));
#41162=CARTESIAN_POINT('Ctrl Pts',(2.10860772565226,4.4244567238612,383.173608033984));
#41163=CARTESIAN_POINT('Ctrl Pts',(3.96354624804163,2.88311376494861,383.094480158524));
#41164=CARTESIAN_POINT('Ctrl Pts',(4.85877851973045,0.643673161011885,383.015352283064));
#41165=CARTESIAN_POINT('Ctrl Pts',(4.57753906021165,-1.7516221037192,382.936224407605));
#41166=CARTESIAN_POINT('Ctrl Pts',(3.18792528789615,-3.72279145276676,382.857096532144));
#41167=CARTESIAN_POINT('Ctrl Pts',(1.0264088723172,-4.79254928705272,382.777968656685));
#41168=CARTESIAN_POINT('Ctrl Pts',(-1.38363523762741,-4.70187168808304,
382.698840781225));
#41169=CARTESIAN_POINT('Ctrl Pts',(-3.45865527994654,-3.47271471567979,
382.619712905766));
#41170=CARTESIAN_POINT('Ctrl Pts',(-4.69621995188282,-1.40269811632394,
382.540585030305));
#41171=CARTESIAN_POINT('Ctrl Pts',(-4.79667372352029,1.00695830702717,382.461457154846));
#41172=CARTESIAN_POINT('Ctrl Pts',(-3.73569339878306,3.17279666418915,382.382329279386));
#41173=CARTESIAN_POINT('Ctrl Pts',(-1.77017756943694,4.57039552059375,382.303201403927));
#41174=CARTESIAN_POINT('Ctrl Pts',(0.623957070419554,4.86134975251467,382.224073528466));
#41175=CARTESIAN_POINT('Ctrl Pts',(2.86701097015694,3.97520967233186,382.144945653007));
#41176=CARTESIAN_POINT('Ctrl Pts',(4.41586624656651,2.12653923886574,382.065817777547));
#41177=CARTESIAN_POINT('Ctrl Pts',(4.89549357056314,-0.237037006764906,
381.986689902087));
#41178=CARTESIAN_POINT('Ctrl Pts',(4.18975922954695,-2.54321871659263,381.907562026627));
#41179=CARTESIAN_POINT('Ctrl Pts',(2.46954495821251,-4.2336026669219,381.828434151167));
#41180=CARTESIAN_POINT('Ctrl Pts',(0.151371792377024,-4.89889073387779,
381.749306275708));
#41181=CARTESIAN_POINT('Ctrl Pts',(-2.20345351430222,-4.37799456969858,
381.670178400248));
#41182=CARTESIAN_POINT('Ctrl Pts',(-4.0247495069615,-2.79704044450812,381.591050524788));
#41183=CARTESIAN_POINT('Ctrl Pts',(-4.87151990622233,-0.53882988528894,
381.511922649328));
#41184=CARTESIAN_POINT('Ctrl Pts',(-4.53873346122441,1.84984929385154,381.432794773869));
#41185=CARTESIAN_POINT('Ctrl Pts',(-3.10696882840965,3.79061849060175,381.353666898409));
#41186=CARTESIAN_POINT('Ctrl Pts',(-0.922903801262455,4.8135529929166,381.274539022949));
#41187=CARTESIAN_POINT('Ctrl Pts',(1.48462690319438,4.67096636685734,381.195411147489));
#41188=CARTESIAN_POINT('Ctrl Pts',(3.53268010195595,3.39738357258133,381.11628327203));
#41189=CARTESIAN_POINT('Ctrl Pts',(4.72535406116718,1.30118132426344,381.03715539657));
#41190=CARTESIAN_POINT('Ctrl Pts',(4.77386278412913,-1.11008015940651,380.95802752111));
#41191=CARTESIAN_POINT('Ctrl Pts',(3.66646069712405,-3.25255434980657,380.87889964565));
#41192=CARTESIAN_POINT('Ctrl Pts',(1.67128664310421,-4.60747705350581,380.799771770191));
#41193=CARTESIAN_POINT('Ctrl Pts',(-0.728561442129978,-4.84677646142697,
380.72064389473));
#41194=CARTESIAN_POINT('Ctrl Pts',(-2.95200059297187,-3.91251023527028,
380.641516019271));
#41195=CARTESIAN_POINT('Ctrl Pts',(-4.46066230869571,-2.03089527297259,
380.562388143811));
#41196=CARTESIAN_POINT('Ctrl Pts',(-4.88924945684393,0.342466919208695,
380.483260268352));
#41197=CARTESIAN_POINT('Ctrl Pts',(-4.13398684739545,2.63290649047066,380.404132392891));
#41198=CARTESIAN_POINT('Ctrl Pts',(-2.37774865459918,4.28583191195745,380.325004517432));
#41199=CARTESIAN_POINT('Ctrl Pts',(-0.045778502691498,4.90101501433043,
380.245876641972));
#41200=CARTESIAN_POINT('Ctrl Pts',(2.29727614588441,4.32949952668338,380.166748766512));
#41201=CARTESIAN_POINT('Ctrl Pts',(4.08408390371697,2.70966833937311,380.087620891052));
#41202=CARTESIAN_POINT('Ctrl Pts',(4.88199923908331,0.433736407961101,380.008493015593));
#41203=CARTESIAN_POINT('Ctrl Pts',(4.49782033548913,-1.94721752037656,379.929365140133));
#41204=CARTESIAN_POINT('Ctrl Pts',(3.02456967131446,-3.8566853832489,379.850237264673));
#41205=CARTESIAN_POINT('Ctrl Pts',(0.818970186768649,-4.83232156164975,
379.771109389213));
#41206=CARTESIAN_POINT('Ctrl Pts',(-1.5849291934243,-4.63789211752843,379.691981513754));
#41207=CARTESIAN_POINT('Ctrl Pts',(-3.60506455052847,-3.32047487997185,
379.612853638294));
#41208=CARTESIAN_POINT('Ctrl Pts',(-4.75229398783147,-1.19906033844088,
379.533725762834));
#41209=CARTESIAN_POINT('Ctrl Pts',(-4.74883513745721,1.21268655441244,379.454597887374));
#41210=CARTESIAN_POINT('Ctrl Pts',(-3.59552550201493,3.33080173627333,379.375470011914));
#41211=CARTESIAN_POINT('Ctrl Pts',(-1.57161966738812,4.64241913909978,379.296342136455));
#41212=CARTESIAN_POINT('Ctrl Pts',(0.832827511814025,4.82995260614083,379.217214260995));
#41213=CARTESIAN_POINT('Ctrl Pts',(3.03561947651265,3.84799405350607,379.138086385535));
#41214=CARTESIAN_POINT('Ctrl Pts',(4.50338709582942,1.93430827613337,379.058958510075));
#41215=CARTESIAN_POINT('Ctrl Pts',(4.88073505691033,-0.447737809714184,
378.979830634616));
#41216=CARTESIAN_POINT('Ctrl Pts',(4.07629487954206,-2.72137169402128,378.900702759156));
#41217=CARTESIAN_POINT('Ctrl Pts',(2.28484826128058,-4.33607106317736,378.821574883696));
#41218=CARTESIAN_POINT('Ctrl Pts',(-0.0598360438974424,-4.90086354532054,
378.742447008237));
#41219=CARTESIAN_POINT('Ctrl Pts',(-2.39003205456549,-4.27899411312408,
378.663319132776));
#41220=CARTESIAN_POINT('Ctrl Pts',(-4.14152188682712,-2.62103802012351,
378.584191257317));
#41221=CARTESIAN_POINT('Ctrl Pts',(-4.89021165231393,-0.328441528394388,
378.505063381857));
#41222=CARTESIAN_POINT('Ctrl Pts',(-4.45481868070814,2.04368157109047,378.425935506397));
#41223=CARTESIAN_POINT('Ctrl Pts',(-2.94076607803947,3.92096145304356,378.346807630937));
#41224=CARTESIAN_POINT('Ctrl Pts',(-0.714656289627798,4.84884627820851,
378.267679755477));
#41225=CARTESIAN_POINT('Ctrl Pts',(1.68449553370326,4.60266429787517,378.188551880018));
#41226=CARTESIAN_POINT('Ctrl Pts',(3.67577501448982,3.24202434982427,378.109424004558));
#41227=CARTESIAN_POINT('Ctrl Pts',(4.77702722252339,1.09638257796792,378.030296129098));
#41228=CARTESIAN_POINT('Ctrl Pts',(4.72160240490404,-1.31472984753725,377.951168253638));
#41229=CARTESIAN_POINT('Ctrl Pts',(3.52292075167996,-3.40750249000403,377.872040378179));
#41230=CARTESIAN_POINT('Ctrl Pts',(1.47122292189925,-4.67520555228101,377.792912502719));
#41231=CARTESIAN_POINT('Ctrl Pts',(-0.936706864306466,-4.81088599868696,
377.713784627259));
#41232=CARTESIAN_POINT('Ctrl Pts',(-3.11782879297974,-3.78169108464289,
377.634656751799));
#41233=CARTESIAN_POINT('Ctrl Pts',(-4.54402076903412,-1.83682309779347,
377.555528876339));
#41234=CARTESIAN_POINT('Ctrl Pts',(-4.86995432435985,0.552800796535157,
377.47640100088));
#41235=CARTESIAN_POINT('Ctrl Pts',(-4.01671011481814,2.80857324909262,377.39727312542));
#41236=CARTESIAN_POINT('Ctrl Pts',(-2.19088691585556,4.3842967924097,377.31814524996));
#41237=CARTESIAN_POINT('Ctrl Pts',(0.165422806069439,4.89843639718154,377.2390173745));
#41238=CARTESIAN_POINT('Ctrl Pts',(2.48167816983692,4.22650178082969,377.159889499041));
#41239=CARTESIAN_POINT('Ctrl Pts',(4.19703678539643,2.53119064158134,377.080761623581));
#41240=CARTESIAN_POINT('Ctrl Pts',(4.89615333254211,0.222994139474255,377.001633748121));
#41241=CARTESIAN_POINT('Ctrl Pts',(4.40974846437591,-2.13919665363753,376.922505872661));
#41242=CARTESIAN_POINT('Ctrl Pts',(2.85559696215369,-3.98341685387501,376.843377997201));
#41243=CARTESIAN_POINT('Ctrl Pts',(0.610010547211784,-4.86311946946737,
376.764250121742));
#41244=CARTESIAN_POINT('Ctrl Pts',(-1.78327969114604,-4.56529926566563,
376.685122246282));
#41245=CARTESIAN_POINT('Ctrl Pts',(-3.74477865997579,-3.16206841006309,
376.605994370822));
#41246=CARTESIAN_POINT('Ctrl Pts',(-4.79954228053442,-0.99319572046786,
376.526866495362));
#41247=CARTESIAN_POINT('Ctrl Pts',(-4.69217723182007,1.41616265569688,376.447738619902));
#41248=CARTESIAN_POINT('Ctrl Pts',(-3.44868015951322,3.48262099568224,376.368610744443));
#41249=CARTESIAN_POINT('Ctrl Pts',(-1.37014302527182,4.70582106870975,376.289482868983));
#41250=CARTESIAN_POINT('Ctrl Pts',(1.04015126435086,4.78958549295691,376.210354993523));
#41251=CARTESIAN_POINT('Ctrl Pts',(3.1985903683765,3.71363211500125,376.131227118063));
#41252=CARTESIAN_POINT('Ctrl Pts',(4.58254446188996,1.73848500650345,376.052099242604));
#41253=CARTESIAN_POINT('Ctrl Pts',(4.85691226192656,-0.657607098782336,
375.972971367144));
#41254=CARTESIAN_POINT('Ctrl Pts',(3.95526022777064,-2.89447065515981,375.893843491684));
#41255=CARTESIAN_POINT('Ctrl Pts',(2.09590823415934,-4.43048672573689,375.814715616224));
#41256=CARTESIAN_POINT('Ctrl Pts',(-0.270932724915457,-4.89373465602332,
375.735587740765));
#41257=CARTESIAN_POINT('Ctrl Pts',(-2.57217200103202,-4.17204699080374,
375.656459865305));
#41258=CARTESIAN_POINT('Ctrl Pts',(-4.25060268497819,-2.44016774048634,
375.577331989845));
#41259=CARTESIAN_POINT('Ctrl Pts',(-4.8998218096771,-0.117443592583374,
375.498204114385));
#41260=CARTESIAN_POINT('Ctrl Pts',(-4.36263000323237,2.23371923670199,375.419076238926));
#41261=CARTESIAN_POINT('Ctrl Pts',(-2.76910316484765,4.04402084944263,375.339948363465));
#41262=CARTESIAN_POINT('Ctrl Pts',(-0.505078814327535,4.87513818307261,
375.260820488006));
#41263=CARTESIAN_POINT('Ctrl Pts',(1.88123000134211,4.52580661359865,375.181692612546));
#41264=CARTESIAN_POINT('Ctrl Pts',(3.81205567946445,3.08066074485737,375.102564737086));
#41265=CARTESIAN_POINT('Ctrl Pts',(4.81980261485754,0.889513660705449,375.023436861627));
#41266=CARTESIAN_POINT('Ctrl Pts',(4.6606270588275,-1.51685826939215,374.944308986167));
#41267=CARTESIAN_POINT('Ctrl Pts',(3.37271297305025,-3.55624114494146,374.865181110707));
#41268=CARTESIAN_POINT('Ctrl Pts',(1.96999142168877,-4.34109857602843,374.812429193734));
#41269=CARTESIAN_POINT('Ctrl Pts',(1.21713437249897,-4.54280821229842,374.786053235247));
#41270=CARTESIAN_POINT('Ctrl Pts',(3.71544298812251,3.17665283523749,400.213946764753));
#41271=CARTESIAN_POINT('Ctrl Pts',(4.24189388987153,2.56091091663784,400.187570806266));
#41272=CARTESIAN_POINT('Ctrl Pts',(4.98214581433909,1.06316653552657,400.134818889293));
#41273=CARTESIAN_POINT('Ctrl Pts',(4.88599424296224,-1.44202664096201,400.055691013833));
#41274=CARTESIAN_POINT('Ctrl Pts',(3.60674265589465,-3.5976617763163,399.976563138373));
#41275=CARTESIAN_POINT('Ctrl Pts',(1.45418293597717,-4.88238291434578,399.897435262914));
#41276=CARTESIAN_POINT('Ctrl Pts',(-1.05048684560331,-4.98482476427098,
399.818307387454));
#41277=CARTESIAN_POINT('Ctrl Pts',(-3.30079722370572,-3.88031872051941,
399.739179511994));
#41278=CARTESIAN_POINT('Ctrl Pts',(-4.75187572291575,-1.83623790534267,
399.660051636534));
#41279=CARTESIAN_POINT('Ctrl Pts',(-5.05236683263146,0.652447348843657,
399.580923761074));
#41280=CARTESIAN_POINT('Ctrl Pts',(-4.12951222709533,2.98315803806871,399.501795885615));
#41281=CARTESIAN_POINT('Ctrl Pts',(-2.20676540787796,4.59154485677586,399.422668010155));
#41282=CARTESIAN_POINT('Ctrl Pts',(0.250312604852073,5.08816712539591,399.343540134695));
#41283=CARTESIAN_POINT('Ctrl Pts',(2.64678163724731,4.35277457160906,399.264412259235));
#41284=CARTESIAN_POINT('Ctrl Pts',(4.40237687684668,2.5634308867403,399.185284383776));
#41285=CARTESIAN_POINT('Ctrl Pts',(5.09201039289903,0.153395295488701,399.106156508315));
#41286=CARTESIAN_POINT('Ctrl Pts',(4.54869898923014,-2.29378234250105,399.027028632856));
#41287=CARTESIAN_POINT('Ctrl Pts',(2.90399641321393,-4.1855590799549,398.947900757396));
#41288=CARTESIAN_POINT('Ctrl Pts',(0.556139808676901,-5.06387287138275,
398.868772881936));
#41289=CARTESIAN_POINT('Ctrl Pts',(-1.92637672321179,-4.7160547794503,398.789645006477));
#41290=CARTESIAN_POINT('Ctrl Pts',(-3.94245343924376,-3.22632311381047,
398.710517131017));
#41291=CARTESIAN_POINT('Ctrl Pts',(-5.00393117442772,-0.955391416550765,
398.631389255557));
#41292=CARTESIAN_POINT('Ctrl Pts',(-4.85379089746955,1.54687228977885,398.552261380098));
#41293=CARTESIAN_POINT('Ctrl Pts',(-3.52838655837555,3.67458681370817,398.473133504638));
#41294=CARTESIAN_POINT('Ctrl Pts',(-1.34864258930642,4.91256176790427,398.394005629178));
#41295=CARTESIAN_POINT('Ctrl Pts',(1.15765256446685,4.96104227929438,398.314877753718));
#41296=CARTESIAN_POINT('Ctrl Pts',(3.38364156492812,3.80828960520879,398.235749878258));
#41297=CARTESIAN_POINT('Ctrl Pts',(4.79033850803188,1.73342347263734,398.156622002798));
#41298=CARTESIAN_POINT('Ctrl Pts',(5.03713532094231,-0.761162082306909,
398.077494127339));
#41299=CARTESIAN_POINT('Ctrl Pts',(4.064274294482,-3.07144500459355,397.998366251879));
#41300=CARTESIAN_POINT('Ctrl Pts',(2.10731741020158,-4.63802903070772,397.919238376419));
#41301=CARTESIAN_POINT('Ctrl Pts',(-0.359891042804634,-5.08159211215712,
397.840110500959));
#41302=CARTESIAN_POINT('Ctrl Pts',(-2.73995791558548,-4.29473288783458,
397.7609826255));
#41303=CARTESIAN_POINT('Ctrl Pts',(-4.45658993137603,-2.46797612236942,
397.68185475004));
#41304=CARTESIAN_POINT('Ctrl Pts',(-5.0941334374604,-0.0436403296913884,
397.60272687458));
#41305=CARTESIAN_POINT('Ctrl Pts',(-4.49821796618352,2.39126223692249,397.52359899912));
#41306=CARTESIAN_POINT('Ctrl Pts',(-2.81313445472219,4.24716075710381,397.44447112366));
#41307=CARTESIAN_POINT('Ctrl Pts',(-0.446897614573966,5.07468052975907,
397.365343248201));
#41308=CARTESIAN_POINT('Ctrl Pts',(2.02754798795257,4.67345152040515,397.286215372741));
#41309=CARTESIAN_POINT('Ctrl Pts',(4.01105684952524,3.14062460458175,397.207087497281));
#41310=CARTESIAN_POINT('Ctrl Pts',(5.02335556505595,0.847348112672217,397.127959621822));
#41311=CARTESIAN_POINT('Ctrl Pts',(4.8193329780012,-1.65109951371132,397.048831746361));
#41312=CARTESIAN_POINT('Ctrl Pts',(3.44838973612117,-3.74976108370145,396.969703870902));
#41313=CARTESIAN_POINT('Ctrl Pts',(1.24247675313054,-4.94048089511111,396.890575995442));
#41314=CARTESIAN_POINT('Ctrl Pts',(-1.26428113785597,-4.93494611535824,
396.811448119982));
#41315=CARTESIAN_POINT('Ctrl Pts',(-3.46491455477013,-3.73449689853531,
396.732320244522));
#41316=CARTESIAN_POINT('Ctrl Pts',(-4.82657702287821,-1.62980188957181,
396.653192369063));
#41317=CARTESIAN_POINT('Ctrl Pts',(-5.01956481218505,0.869522313285533,
396.574064493603));
#41318=CARTESIAN_POINT('Ctrl Pts',(-3.99714916613881,3.15830627087741,396.494936618143));
#41319=CARTESIAN_POINT('Ctrl Pts',(-2.00689088633465,4.68235933343167,396.415808742683));
#41320=CARTESIAN_POINT('Ctrl Pts',(0.469302363710116,5.07265761198643,396.336680867223));
#41321=CARTESIAN_POINT('Ctrl Pts',(2.83186191712685,4.23469692414397,396.257552991764));
#41322=CARTESIAN_POINT('Ctrl Pts',(4.50873360091663,2.37137539689376,396.178425116304));
#41323=CARTESIAN_POINT('Ctrl Pts',(5.09389105993074,-0.066134912001412,
396.099297240844));
#41324=CARTESIAN_POINT('Ctrl Pts',(4.44564822923743,-2.48763176111453,396.020169365385));
#41325=CARTESIAN_POINT('Ctrl Pts',(2.72096623850579,-4.30679029974057,395.941041489925));
#41326=CARTESIAN_POINT('Ctrl Pts',(0.337447906876279,-5.08313179714755,
395.861913614465));
#41327=CARTESIAN_POINT('Ctrl Pts',(-2.12777777601096,-4.6286781798848,395.782785739005));
#41328=CARTESIAN_POINT('Ctrl Pts',(-4.07779775573568,-3.05346776965875,
395.703657863545));
#41329=CARTESIAN_POINT('Ctrl Pts',(-5.04044739830187,-0.738911349202079,
395.624529988086));
#41330=CARTESIAN_POINT('Ctrl Pts',(-4.78263723751197,1.75456006206446,395.545402112625));
#41331=CARTESIAN_POINT('Ctrl Pts',(-3.36679168002614,3.82319418030715,395.466274237166));
#41332=CARTESIAN_POINT('Ctrl Pts',(-1.13573398221921,4.9661059471844,395.387146361706));
#41333=CARTESIAN_POINT('Ctrl Pts',(1.37032265180738,4.90655844630137,395.308018486247));
#41334=CARTESIAN_POINT('Ctrl Pts',(3.54457863759732,3.65897010631632,395.228890610786));
#41335=CARTESIAN_POINT('Ctrl Pts',(4.86057435298355,1.52542352025471,395.149762735327));
#41336=CARTESIAN_POINT('Ctrl Pts',(4.99966350625814,-0.977478788116796,
395.070634859867));
#41337=CARTESIAN_POINT('Ctrl Pts',(3.9281679916419,-3.24370100139759,394.991506984407));
#41338=CARTESIAN_POINT('Ctrl Pts',(1.90553247777794,-4.72451541781389,394.912379108947));
#41339=CARTESIAN_POINT('Ctrl Pts',(-0.578495767592555,-5.0613676614039,
394.833251233488));
#41340=CARTESIAN_POINT('Ctrl Pts',(-2.92245096488478,-4.17269461078471,
394.754123358028));
#41341=CARTESIAN_POINT('Ctrl Pts',(-4.55878367391877,-2.27367354108707,
394.674995482568));
#41342=CARTESIAN_POINT('Ctrl Pts',(-5.09128337239731,0.175879444445247,
394.595867607109));
#41343=CARTESIAN_POINT('Ctrl Pts',(-4.39101418897073,2.58284617220721,394.516739731648));
#41344=CARTESIAN_POINT('Ctrl Pts',(-2.62753456208024,4.36442001669197,394.437611856189));
#41345=CARTESIAN_POINT('Ctrl Pts',(-0.227841507780872,5.08922275051504,
394.358483980729));
#41346=CARTESIAN_POINT('Ctrl Pts',(2.22701954646155,4.58175554746277,394.279356105269));
#41347=CARTESIAN_POINT('Ctrl Pts',(4.14264516722633,2.96489307994134,394.200228229809));
#41348=CARTESIAN_POINT('Ctrl Pts',(5.05519873770637,0.630131477804167,394.12110035435));
#41349=CARTESIAN_POINT('Ctrl Pts',(4.74372071539057,-1.85720589364835,394.04197247889));
#41350=CARTESIAN_POINT('Ctrl Pts',(3.28363027953537,-3.89485200544849,393.96284460343));
#41351=CARTESIAN_POINT('Ctrl Pts',(1.02846384177488,-4.98942502530997,393.883716727971));
#41352=CARTESIAN_POINT('Ctrl Pts',(-1.47572786674121,-4.87589245373102,
393.80458885251));
#41353=CARTESIAN_POINT('Ctrl Pts',(-3.62259682199201,-3.58174429884674,
393.725460977051));
#41354=CARTESIAN_POINT('Ctrl Pts',(-4.89231471194326,-1.42033683199839,
393.646333101591));
#41355=CARTESIAN_POINT('Ctrl Pts',(-4.97744064418338,1.0849813780241,393.567205226131));
#41356=CARTESIAN_POINT('Ctrl Pts',(-3.85736280188092,3.32758954375282,393.488077350671));
#41357=CARTESIAN_POINT('Ctrl Pts',(-1.8032892495463,4.76447770899377,393.408949475212));
#41358=CARTESIAN_POINT('Ctrl Pts',(0.687420551315965,5.04772750281314,393.329821599752));
#41359=CARTESIAN_POINT('Ctrl Pts',(3.01168299451616,4.1087547380648,393.250693724292));
#41360=CARTESIAN_POINT('Ctrl Pts',(4.60671691000739,2.1749159220714,393.171565848832));
#41361=CARTESIAN_POINT('Ctrl Pts',(5.08631158572023,-0.285542308591735,
393.092437973373));
#41362=CARTESIAN_POINT('Ctrl Pts',(4.33434121428917,-2.67686125810472,393.013310097913));
#41363=CARTESIAN_POINT('Ctrl Pts',(2.5328828097419,-4.42002314803234,392.934182222453));
#41364=CARTESIAN_POINT('Ctrl Pts',(0.118129312194917,-5.09295056157313,
392.855054346993));
#41365=CARTESIAN_POINT('Ctrl Pts',(-2.32522721713463,-4.53270541131057,
392.775926471534));
#41366=CARTESIAN_POINT('Ctrl Pts',(-4.20556897258945,-2.87494166442045,
392.696798596073));
#41367=CARTESIAN_POINT('Ctrl Pts',(-5.06760273359595,-0.521059009593531,
392.617670720614));
#41368=CARTESIAN_POINT('Ctrl Pts',(-4.70260148223132,1.95898934564318,392.538542845154));
#41369=CARTESIAN_POINT('Ctrl Pts',(-3.19894415001964,3.96470128535339,392.459414969695));
#41370=CARTESIAN_POINT('Ctrl Pts',(-0.920716141880372,5.01042730144931,
392.380287094234));
#41371=CARTESIAN_POINT('Ctrl Pts',(1.58044783853879,4.84296237717018,392.301159218775));
#41372=CARTESIAN_POINT('Ctrl Pts',(3.69893288079714,3.50285533534937,392.222031343315));
#41373=CARTESIAN_POINT('Ctrl Pts',(4.92178336136043,1.31459062101607,392.142903467856));
#41374=CARTESIAN_POINT('Ctrl Pts',(4.9529065449796,-1.19198016498848,392.063775592395));
#41375=CARTESIAN_POINT('Ctrl Pts',(3.78476647471314,-3.40993294492945,391.984647716936));
#41376=CARTESIAN_POINT('Ctrl Pts',(1.70020867751367,-4.80222765078197,391.905519841476));
#41377=CARTESIAN_POINT('Ctrl Pts',(-0.796026136476369,-5.03174346991918,
391.826391966016));
#41378=CARTESIAN_POINT('Ctrl Pts',(-3.09951657179924,-4.04290699598317,
391.747264090556));
#41379=CARTESIAN_POINT('Ctrl Pts',(-4.65251105174488,-2.07514839720426,
391.668136215097));
#41380=CARTESIAN_POINT('Ctrl Pts',(-5.07897800851123,0.395072583314779,
391.589008339637));
#41381=CARTESIAN_POINT('Ctrl Pts',(-4.27565562086226,2.76963336360912,391.509880464177));
#41382=CARTESIAN_POINT('Ctrl Pts',(-2.43705493231998,4.47357387486589,391.430752588717));
#41383=CARTESIAN_POINT('Ctrl Pts',(-0.00836226415120685,5.0943134993408,
391.351624713257));
#41384=CARTESIAN_POINT('Ctrl Pts',(2.42235518603692,4.48155054748998,391.272496837798));
#41385=CARTESIAN_POINT('Ctrl Pts',(4.26653995362923,2.78365529135943,391.193368962338));
#41386=CARTESIAN_POINT('Ctrl Pts',(5.0776536262684,0.411744591550536,391.114241086878));
#41387=CARTESIAN_POINT('Ctrl Pts',(4.65929863144093,-2.05986315566845,391.035113211418));
#41388=CARTESIAN_POINT('Ctrl Pts',(3.11277261484635,-4.03270958603397,390.955985335959));
#41389=CARTESIAN_POINT('Ctrl Pts',(0.812540914369942,-5.02910302335342,
390.876857460499));
#41390=CARTESIAN_POINT('Ctrl Pts',(-1.68443394126863,-4.80778350745226,
390.797729585039));
#41391=CARTESIAN_POINT('Ctrl Pts',(-3.7735513679378,-3.42233984732121,390.718601709579));
#41392=CARTESIAN_POINT('Ctrl Pts',(-4.94896661768926,-1.20823398976565,
390.639473834119));
#41393=CARTESIAN_POINT('Ctrl Pts',(-4.92607260087128,1.29842546492777,390.56034595866));
#41394=CARTESIAN_POINT('Ctrl Pts',(-3.71041271969718,3.49069296938833,390.4812180832));
#41395=CARTESIAN_POINT('Ctrl Pts',(-1.59633862636855,4.83774771427692,390.40209020774));
#41396=CARTESIAN_POINT('Ctrl Pts',(0.904262092886961,5.01342298478748,390.32296233228));
#41397=CARTESIAN_POINT('Ctrl Pts',(3.18591091187283,3.97518196044373,390.243834456821));
#41398=CARTESIAN_POINT('Ctrl Pts',(4.69614483496588,1.97441729278565,390.164706581361));
#41399=CARTESIAN_POINT('Ctrl Pts',(5.06928604606176,-0.504419409054961,
390.085578705901));
#41400=CARTESIAN_POINT('Ctrl Pts',(4.21498465890399,-2.86111941069082,390.006450830441));
#41401=CARTESIAN_POINT('Ctrl Pts',(2.34009542676882,-4.52504733131526,389.927322954981));
#41402=CARTESIAN_POINT('Ctrl Pts',(-0.101408666846889,-5.09331093094817,
389.848195079522));
#41403=CARTESIAN_POINT('Ctrl Pts',(-2.51835835252648,-4.42831470937736,
389.769067204062));
#41404=CARTESIAN_POINT('Ctrl Pts',(-4.3255297989291,-2.6910763488991,389.689939328602));
#41405=CARTESIAN_POINT('Ctrl Pts',(-5.08534674866728,-0.302238983003182,
389.610811453142));
#41406=CARTESIAN_POINT('Ctrl Pts',(-4.61383227037253,2.15978048372904,389.531683577683));
#41407=CARTESIAN_POINT('Ctrl Pts',(-3.02515568711978,4.09884532834732,389.452555702223));
#41408=CARTESIAN_POINT('Ctrl Pts',(-0.703988389596766,5.04544351909133,
389.373427826763));
#41409=CARTESIAN_POINT('Ctrl Pts',(1.78763788976615,4.7703721796208,389.294299951303));
#41410=CARTESIAN_POINT('Ctrl Pts',(3.84641763488075,3.34023522152349,389.215172075843));
#41411=CARTESIAN_POINT('Ctrl Pts',(4.97385185858917,1.10131632414888,389.136044200384));
#41412=CARTESIAN_POINT('Ctrl Pts',(4.89695127199855,-1.40426785076764,389.056916324924));
#41413=CARTESIAN_POINT('Ctrl Pts',(3.63433606243988,-3.56983211681959,388.977788449464));
#41414=CARTESIAN_POINT('Ctrl Pts',(1.4917273273879,-4.87102140600428,388.898660574004));
#41415=CARTESIAN_POINT('Ctrl Pts',(-1.0120781619955,-4.99277455439754,388.819532698545));
#41416=CARTESIAN_POINT('Ctrl Pts',(-3.27082589817505,-3.9056110790573,388.740404823085));
#41417=CARTESIAN_POINT('Ctrl Pts',(-4.73759799865136,-1.87276938254615,
388.661276947625));
#41418=CARTESIAN_POINT('Ctrl Pts',(-5.05724019876165,0.613532011436209,
388.582149072166));
#41419=CARTESIAN_POINT('Ctrl Pts',(-4.15235650051922,2.95127691849197,388.503021196705));
#41420=CARTESIAN_POINT('Ctrl Pts',(-2.24204931550549,4.57441961606814,388.423893321246));
#41421=CARTESIAN_POINT('Ctrl Pts',(0.211132509493252,5.0899433219303,388.344765445786));
#41422=CARTESIAN_POINT('Ctrl Pts',(2.613192138255,4.37302261663371,388.265637570326));
#41423=CARTESIAN_POINT('Ctrl Pts',(4.3825111169981,2.59724782537512,388.186509694867));
#41424=CARTESIAN_POINT('Ctrl Pts',(5.09067852854909,0.192593032057139,388.107381819407));
#41425=CARTESIAN_POINT('Ctrl Pts',(4.56622351098889,-2.25869493396522,388.028253943947));
#41426=CARTESIAN_POINT('Ctrl Pts',(2.93613405110136,-4.16307780265885,387.949126068487));
#41427=CARTESIAN_POINT('Ctrl Pts',(0.595108973109503,-5.05944120107668,
387.869998193027));
#41428=CARTESIAN_POINT('Ctrl Pts',(-1.89001176205386,-4.73074576534459,
387.790870317568));
#41429=CARTESIAN_POINT('Ctrl Pts',(-3.91749784672291,-3.2565795826218,387.711742442108));
#41430=CARTESIAN_POINT('Ctrl Pts',(-4.99642752878567,-0.993887270579772,
387.632614566648));
#41431=CARTESIAN_POINT('Ctrl Pts',(-4.86555608063145,1.50945817539208,387.553486691188));
#41432=CARTESIAN_POINT('Ctrl Pts',(-3.55657182856503,3.6473136395552,387.474358815728));
#41433=CARTESIAN_POINT('Ctrl Pts',(-1.38642335604174,4.90203327557553,387.395230940269));
#41434=CARTESIAN_POINT('Ctrl Pts',(1.11942428022107,4.96980776669272,387.316103064809));
#41435=CARTESIAN_POINT('Ctrl Pts',(3.35422210107046,3.83422665653951,387.236975189349));
#41436=CARTESIAN_POINT('Ctrl Pts',(4.77685129433647,1.77025186592861,387.157847313889));
#41437=CARTESIAN_POINT('Ctrl Pts',(5.04284606000954,-0.72235972484213,387.07871943843));
#41438=CARTESIAN_POINT('Ctrl Pts',(4.08780022662232,-3.04006402305186,386.99959156297));
#41439=CARTESIAN_POINT('Ctrl Pts',(2.14296212550442,-4.62166780347541,386.92046368751));
#41440=CARTESIAN_POINT('Ctrl Pts',(-0.320758314346703,-5.08421223601112,
386.84133581205));
#41441=CARTESIAN_POINT('Ctrl Pts',(-2.70681250786736,-4.31569994372646,
386.76220793659));
#41442=CARTESIAN_POINT('Ctrl Pts',(-4.43745744898977,-2.50221328935662,
386.683080061131));
#41443=CARTESIAN_POINT('Ctrl Pts',(-5.09364649014193,-0.082857651985011,
386.603952185671));
#41444=CARTESIAN_POINT('Ctrl Pts',(-4.51649446005934,2.35656057619595,386.524824310211));
#41445=CARTESIAN_POINT('Ctrl Pts',(-2.84574904331825,4.22537718310224,386.445696434751));
#41446=CARTESIAN_POINT('Ctrl Pts',(-0.485953222246148,5.07108956959117,
386.366568559292));
#41447=CARTESIAN_POINT('Ctrl Pts',(1.99150802159427,4.68892266485099,386.287440683832));
#41448=CARTESIAN_POINT('Ctrl Pts',(3.98675899790251,3.17141177548282,386.208312808372));
#41449=CARTESIAN_POINT('Ctrl Pts',(5.01668314543611,0.885996712931309,386.129184932912));
#41450=CARTESIAN_POINT('Ctrl Pts',(4.83190160489097,-1.61394759446514,386.050057057452));
#41451=CARTESIAN_POINT('Ctrl Pts',(3.47715612730962,-3.72310155963289,385.970929181992));
#41452=CARTESIAN_POINT('Ctrl Pts',(1.28047560943712,-4.93076892286227,385.891801306533));
#41453=CARTESIAN_POINT('Ctrl Pts',(-1.22625060220108,-4.94453328612815,
385.812673431073));
#41454=CARTESIAN_POINT('Ctrl Pts',(-3.43606079615961,-3.76106183970999,
385.733545555613));
#41455=CARTESIAN_POINT('Ctrl Pts',(-4.81388649504862,-1.66691234617067,
385.654417680153));
#41456=CARTESIAN_POINT('Ctrl Pts',(-5.02611031361548,0.830852015942555,
385.575289804694));
#41457=CARTESIAN_POINT('Ctrl Pts',(-4.02134581343353,3.12743949674625,385.496161929234));
#41458=CARTESIAN_POINT('Ctrl Pts',(-2.04287986715703,4.66676995419661,385.417034053774));
#41459=CARTESIAN_POINT('Ctrl Pts',(0.430235177489289,5.07612033437727,385.337906178314));
#41460=CARTESIAN_POINT('Ctrl Pts',(2.79917598944896,4.25637330800767,385.258778302855));
#41461=CARTESIAN_POINT('Ctrl Pts',(4.49034328098805,2.40601686941577,385.179650427394));
#41462=CARTESIAN_POINT('Ctrl Pts',(5.09424925529516,-0.0269162024146704,
385.100522551935));
#41463=CARTESIAN_POINT('Ctrl Pts',(4.46466820889472,-2.45333196724627,385.021394676475));
#41464=CARTESIAN_POINT('Ctrl Pts',(2.75404263336906,-4.28571454142868,384.942266801016));
#41465=CARTESIAN_POINT('Ctrl Pts',(0.376571822658881,-5.08038321580243,
384.863138925555));
#41466=CARTESIAN_POINT('Ctrl Pts',(-2.09207953936242,-4.64492229838228,
384.784011050096));
#41467=CARTESIAN_POINT('Ctrl Pts',(-4.05416892752487,-3.08477134713736,
384.704883174636));
#41468=CARTESIAN_POINT('Ctrl Pts',(-5.03460930299721,-0.777694749372607,
384.625755299176));
#41469=CARTESIAN_POINT('Ctrl Pts',(-4.79600347197984,1.71768758911072,384.546627423717));
#41470=CARTESIAN_POINT('Ctrl Pts',(-3.39612583475742,3.79716068550186,384.467499548257));
#41471=CARTESIAN_POINT('Ctrl Pts',(-1.17393328361345,4.9572150046828,384.388371672797));
#41472=CARTESIAN_POINT('Ctrl Pts',(1.33250752393625,4.91696284871881,384.309243797337));
#41473=CARTESIAN_POINT('Ctrl Pts',(3.51630398225976,3.6861506021013,384.230115921877));
#41474=CARTESIAN_POINT('Ctrl Pts',(4.84868640377085,1.56279880820132,384.150988046418));
#41475=CARTESIAN_POINT('Ctrl Pts',(5.00704073069747,-0.938958507157973,
384.071860170958));
#41476=CARTESIAN_POINT('Ctrl Pts',(3.95302411855986,-3.213362767431,383.992732295498));
#41477=CARTESIAN_POINT('Ctrl Pts',(1.94184901290741,-4.70970512538717,383.913604420038));
#41478=CARTESIAN_POINT('Ctrl Pts',(-0.539512264162803,-5.06567137444245,
383.834476544579));
#41479=CARTESIAN_POINT('Ctrl Pts',(-2.89023969471176,-4.19507025735449,
383.755348669118));
#41480=CARTESIAN_POINT('Ctrl Pts',(-4.54114405585455,-2.30870323363671,
383.676220793659));
#41481=CARTESIAN_POINT('Ctrl Pts',(-5.0924865441193,0.136677558478088,383.597092918199));
#41482=CARTESIAN_POINT('Ctrl Pts',(-4.41076882262505,2.54896417204843,383.51796504274));
#41483=CARTESIAN_POINT('Ctrl Pts',(-2.66105740443557,4.34406186043965,383.43883716728));
#41484=CARTESIAN_POINT('Ctrl Pts',(-0.267015564777766,5.08731782427579,
383.35970929182));
#41485=CARTESIAN_POINT('Ctrl Pts',(2.19167961573057,4.59876509717759,383.28058141636));
#41486=CARTESIAN_POINT('Ctrl Pts',(4.11969633429617,2.99669852841663,383.201453540901));
#41487=CARTESIAN_POINT('Ctrl Pts',(5.05019767759256,0.669031669105843,383.12232566544));
#41488=CARTESIAN_POINT('Ctrl Pts',(4.75787835092606,-1.8206299884427,383.043197789981));
#41489=CARTESIAN_POINT('Ctrl Pts',(3.31351857671521,-3.8694566283641,382.964069914521));
#41490=CARTESIAN_POINT('Ctrl Pts',(1.06684585069835,-4.98135924099793,382.884942039061));
#41491=CARTESIAN_POINT('Ctrl Pts',(-1.43814570582419,-4.88710925658996,
382.805814163602));
#41492=CARTESIAN_POINT('Ctrl Pts',(-3.59491439905111,-3.60952772818311,
382.726686288142));
#41493=CARTESIAN_POINT('Ctrl Pts',(-4.8812348614273,-1.45795959635872,382.647558412682));
#41494=CARTESIAN_POINT('Ctrl Pts',(-4.98564616607288,1.04662900005231,382.568430537222));
#41495=CARTESIAN_POINT('Ctrl Pts',(-3.88286686666645,3.29779393728166,382.489302661762));
#41496=CARTESIAN_POINT('Ctrl Pts',(-1.83991647567274,4.75045338042336,382.410174786303));
#41497=CARTESIAN_POINT('Ctrl Pts',(0.648538832374088,5.05287020810257,382.331046910843));
#41498=CARTESIAN_POINT('Ctrl Pts',(2.97996133890915,4.13181925737738,382.251919035383));
#41499=CARTESIAN_POINT('Ctrl Pts',(4.58983618463159,2.21031756887428,382.172791159923));
#41500=CARTESIAN_POINT('Ctrl Pts',(5.08835917511605,-0.246375449345246,
382.093663284464));
#41501=CARTESIAN_POINT('Ctrl Pts',(4.35482132902486,-2.64341278450753,382.014535409004));
#41502=CARTESIAN_POINT('Ctrl Pts',(2.56683653350947,-4.40039204699635,381.935407533544));
#41503=CARTESIAN_POINT('Ctrl Pts',(0.157335320227334,-5.09189017497793,
381.856279658084));
#41504=CARTESIAN_POINT('Ctrl Pts',(-2.29026200215225,-4.55047249398623,
381.777151782624));
#41505=CARTESIAN_POINT('Ctrl Pts',(-4.1833107910579,-2.90723421527166,381.698023907165));
#41506=CARTESIAN_POINT('Ctrl Pts',(-5.06344103087761,-0.560057929015174,
381.618896031705));
#41507=CARTESIAN_POINT('Ctrl Pts',(-4.71754394484289,1.92272699193202,381.539768156245));
#41508=CARTESIAN_POINT('Ctrl Pts',(-3.22937271124211,3.9399558181422,381.460640280785));
#41509=CARTESIAN_POINT('Ctrl Pts',(-0.959263035935946,5.0031904206131,381.381512405325));
#41510=CARTESIAN_POINT('Ctrl Pts',(1.54311609556955,4.85498637203256,381.302384529866));
#41511=CARTESIAN_POINT('Ctrl Pts',(3.67185554437766,3.53122879721078,381.223256654406));
#41512=CARTESIAN_POINT('Ctrl Pts',(4.91151675438643,1.35244339194259,381.144128778947));
#41513=CARTESIAN_POINT('Ctrl Pts',(4.96193655414693,-1.15381349864191,381.065000903486));
#41514=CARTESIAN_POINT('Ctrl Pts',(3.81090663474561,-3.38069380131942,380.985873028027));
#41515=CARTESIAN_POINT('Ctrl Pts',(1.73712958706021,-4.78899579815935,380.906745152567));
#41516=CARTESIAN_POINT('Ctrl Pts',(-0.757264256456047,-5.03772277948299,
380.827617277107));
#41517=CARTESIAN_POINT('Ctrl Pts',(-3.06829926047039,-4.0666496782025,380.748489401647));
#41518=CARTESIAN_POINT('Ctrl Pts',(-4.63639705749532,-2.11090555977201,
380.669361526187));
#41519=CARTESIAN_POINT('Ctrl Pts',(-5.08186906479814,0.355958937625331,
380.590233650728));
#41520=CARTESIAN_POINT('Ctrl Pts',(-4.29685170689215,2.73663394812055,380.511105775268));
#41521=CARTESIAN_POINT('Ctrl Pts',(-2.47142377134362,4.45467894460033,380.431977899808));
#41522=CARTESIAN_POINT('Ctrl Pts',(-0.0475820182042561,5.09409814477217,
380.352850024348));
#41523=CARTESIAN_POINT('Ctrl Pts',(2.38778092263769,4.50006691311533,380.273722148889));
#41524=CARTESIAN_POINT('Ctrl Pts',(4.24498275891546,2.81641994978345,380.194594273428));
#41525=CARTESIAN_POINT('Ctrl Pts',(5.07433321340091,0.450824130237162,380.115466397969));
#41526=CARTESIAN_POINT('Ctrl Pts',(4.67501898270842,-2.02393119160303,380.036338522509));
#41527=CARTESIAN_POINT('Ctrl Pts',(3.14372731083789,-4.00862551906755,379.957210647049));
#41528=CARTESIAN_POINT('Ctrl Pts',(0.851234794597309,-5.02269840638422,
379.87808277159));
#41529=CARTESIAN_POINT('Ctrl Pts',(-1.64736995096127,-4.82060911106652,
379.79895489613));
#41530=CARTESIAN_POINT('Ctrl Pts',(-3.74709169119734,-3.45129016670399,
379.71982702067));
#41531=CARTESIAN_POINT('Ctrl Pts',(-4.93951802147898,-1.2462991906088,379.64069914521));
#41532=CARTESIAN_POINT('Ctrl Pts',(-4.93592290429957,1.26046223261093,379.56157126975));
#41533=CARTESIAN_POINT('Ctrl Pts',(-3.73717683698987,3.46202386561592,379.482443394291));
#41534=CARTESIAN_POINT('Ctrl Pts',(-1.63353607538846,4.82531448171332,379.403315518831));
#41535=CARTESIAN_POINT('Ctrl Pts',(0.865638050575662,5.02023612217824,379.324187643371));
#41536=CARTESIAN_POINT('Ctrl Pts',(3.15521244034589,3.99959178083392,379.245059767911));
#41537=CARTESIAN_POINT('Ctrl Pts',(4.6808050542546,2.01051336754875,379.165931892452));
#41538=CARTESIAN_POINT('Ctrl Pts',(5.07301922679952,-0.465377139049836,
379.086804016992));
#41539=CARTESIAN_POINT('Ctrl Pts',(4.23688687398491,-2.82858437634132,379.007676141532));
#41540=CARTESIAN_POINT('Ctrl Pts',(2.37486342213654,-4.5068973455389,378.928548266072));
#41541=CARTESIAN_POINT('Ctrl Pts',(-0.0621933781710937,-5.0939407084044,
378.849420390613));
#41542=CARTESIAN_POINT('Ctrl Pts',(-2.48419109500962,-4.44757176001722,
378.770292515152));
#41543=CARTESIAN_POINT('Ctrl Pts',(-4.30468360095437,-2.72429790087321,
378.691164639693));
#41544=CARTESIAN_POINT('Ctrl Pts',(-5.08286916745938,-0.341380994664952,
378.612036764233));
#41545=CARTESIAN_POINT('Ctrl Pts',(-4.63032321066906,2.12419559404662,378.532908888774));
#41546=CARTESIAN_POINT('Ctrl Pts',(-3.05662214430013,4.07543384488105,378.453781013314));
#41547=CARTESIAN_POINT('Ctrl Pts',(-0.742811288783636,5.03987413992486,
378.374653137854));
#41548=CARTESIAN_POINT('Ctrl Pts',(1.75085886250587,4.78399343651434,378.295525262394));
#41549=CARTESIAN_POINT('Ctrl Pts',(3.82058790417125,3.36974895556452,378.216397386935));
#41550=CARTESIAN_POINT('Ctrl Pts',(4.9652256605272,1.13957627961887,378.137269511474));
#41551=CARTESIAN_POINT('Ctrl Pts',(4.90761729577347,-1.36652568042196,378.058141636015));
#41552=CARTESIAN_POINT('Ctrl Pts',(3.66171170927622,-3.54174636516749,377.979013760555));
#41553=CARTESIAN_POINT('Ctrl Pts',(1.52918404352555,-4.85939256677772,377.899885885095));
#41554=CARTESIAN_POINT('Ctrl Pts',(-0.973609892176757,-5.00041835598616,
377.820758009635));
#41555=CARTESIAN_POINT('Ctrl Pts',(-3.24066052105438,-3.93067670310182,
377.741630134176));
#41556=CARTESIAN_POINT('Ctrl Pts',(-4.72303955439021,-1.90918760856372,
377.662502258716));
#41557=CARTESIAN_POINT('Ctrl Pts',(-5.06181377047586,0.574579246099912,
377.583374383256));
#41558=CARTESIAN_POINT('Ctrl Pts',(-4.17495467452228,2.91922137268011,377.504246507796));
#41559=CARTESIAN_POINT('Ctrl Pts',(-2.27720032296007,4.55702300259043,377.425118632336));
#41560=CARTESIAN_POINT('Ctrl Pts',(0.171939895519064,5.09141793897891,377.345990756877));
#41561=CARTESIAN_POINT('Ctrl Pts',(2.5794477519296,4.39301141042152,377.266862881417));
#41562=CARTESIAN_POINT('Ctrl Pts',(4.36238559553759,2.63091084472138,377.187735005957));
#41563=CARTESIAN_POINT('Ctrl Pts',(5.08904492944719,0.231779341395482,377.108607130498));
#41564=CARTESIAN_POINT('Ctrl Pts',(4.58347738286989,-2.22347364224237,377.029479255037));
#41565=CARTESIAN_POINT('Ctrl Pts',(2.96809765825856,-4.14034977363789,376.950351379578));
#41566=CARTESIAN_POINT('Ctrl Pts',(0.634042864132613,-5.0547096458148,376.871223504118));
#41567=CARTESIAN_POINT('Ctrl Pts',(-1.85353477590152,-4.7451563505839,376.792095628658));
#41568=CARTESIAN_POINT('Ctrl Pts',(-3.89231005589385,-3.28664302685179,
376.712967753199));
#41569=CARTESIAN_POINT('Ctrl Pts',(-4.98862773436458,-1.03232421493045,
376.633839877739));
#41570=CARTESIAN_POINT('Ctrl Pts',(-4.87703287210239,1.47195459226046,376.554712002279));
#41571=CARTESIAN_POINT('Ctrl Pts',(-3.58454629319045,3.61982428153675,376.475584126819));
#41572=CARTESIAN_POINT('Ctrl Pts',(-1.42412194671949,4.89121422922617,376.39645625136));
#41573=CARTESIAN_POINT('Ctrl Pts',(1.08112964569973,4.97827868361118,376.3173283759));
#41574=CARTESIAN_POINT('Ctrl Pts',(3.32460382467506,3.85993644420179,376.23820050044));
#41575=CARTESIAN_POINT('Ctrl Pts',(4.76308094821025,1.80697533479263,376.15907262498));
#41576=CARTESIAN_POINT('Ctrl Pts',(5.04825789565173,-0.683514556087066,
376.07994474952));
#41577=CARTESIAN_POINT('Ctrl Pts',(4.11108387333318,-3.00850284103068,376.000816874061));
#41578=CARTESIAN_POINT('Ctrl Pts',(2.1784798079633,-4.60503266038196,375.921688998601));
#41579=CARTESIAN_POINT('Ctrl Pts',(-0.281606542178375,-5.08653096539461,
375.842561123141));
#41580=CARTESIAN_POINT('Ctrl Pts',(-2.67350672874489,-4.33641128901115,
375.763433247681));
#41581=CARTESIAN_POINT('Ctrl Pts',(-4.41806180727835,-2.5363019544723,375.684305372222));
#41582=CARTESIAN_POINT('Ctrl Pts',(-5.09285793196053,-0.12207046608611,
375.605177496761));
#41583=CARTESIAN_POINT('Ctrl Pts',(-4.53450261646048,2.32172008989041,375.526049621302));
#41584=CARTESIAN_POINT('Ctrl Pts',(-2.8781963029061,4.20334135813296,375.446921745842));
#41585=CARTESIAN_POINT('Ctrl Pts',(-0.524977181972811,5.06720185538771,
375.367793870382));
#41586=CARTESIAN_POINT('Ctrl Pts',(1.95534399133764,4.70410782389334,375.288665994923));
#41587=CARTESIAN_POINT('Ctrl Pts',(3.96223755849503,3.20202817970643,375.209538119463));
#41588=CARTESIAN_POINT('Ctrl Pts',(5.00968625615773,0.924557438714191,375.130410244003));
#41589=CARTESIAN_POINT('Ctrl Pts',(4.84423973083701,-1.5766172667089,375.051282368543));
#41590=CARTESIAN_POINT('Ctrl Pts',(3.50558626093324,-3.69634481139898,374.972154493084));
#41591=CARTESIAN_POINT('Ctrl Pts',(2.04760230627713,-4.51212292509998,374.91940257611));
#41592=CARTESIAN_POINT('Ctrl Pts',(1.26508527942809,-4.72177922709072,374.893026617624));
#41593=CARTESIAN_POINT('Ctrl Pts',(3.8562705385027,3.2970584607914,400.320920147129));
#41594=CARTESIAN_POINT('Ctrl Pts',(4.40267566673985,2.65797789150057,400.294544188642));
#41595=CARTESIAN_POINT('Ctrl Pts',(5.17098558200965,1.10346405572081,400.241792271669));
#41596=CARTESIAN_POINT('Ctrl Pts',(5.07118954877308,-1.49668420940778,400.162664396209));
#41597=CARTESIAN_POINT('Ctrl Pts',(3.74345010496737,-3.73402503008569,400.08353652075));
#41598=CARTESIAN_POINT('Ctrl Pts',(1.50930126812034,-5.0674413388845,400.00440864529));
#41599=CARTESIAN_POINT('Ctrl Pts',(-1.09030376370591,-5.17376607298461,
399.925280769831));
#41600=CARTESIAN_POINT('Ctrl Pts',(-3.42590833126468,-4.02739560525483,
399.84615289437));
#41601=CARTESIAN_POINT('Ctrl Pts',(-4.93198749421962,-1.90583738162352,
399.767025018911));
#41602=CARTESIAN_POINT('Ctrl Pts',(-5.24386820862784,0.677177256470671,
399.68789714345));
#41603=CARTESIAN_POINT('Ctrl Pts',(-4.28603436807985,3.09622957226831,399.608769267991));
#41604=CARTESIAN_POINT('Ctrl Pts',(-2.29040909926245,4.7655795591539,399.529641392531));
#41605=CARTESIAN_POINT('Ctrl Pts',(0.259800278618912,5.28102545063066,399.450513517072));
#41606=CARTESIAN_POINT('Ctrl Pts',(2.7471033957984,4.51775909222651,399.371385641611));
#41607=CARTESIAN_POINT('Ctrl Pts',(4.56924148852249,2.66059337678593,399.292257766152));
#41608=CARTESIAN_POINT('Ctrl Pts',(5.2850143906551,0.159209483399153,399.213129890692));
#41609=CARTESIAN_POINT('Ctrl Pts',(4.7211096918349,-2.38072426286758,399.134002015232));
#41610=CARTESIAN_POINT('Ctrl Pts',(3.01406746059458,-4.34420558161996,399.054874139772));
#41611=CARTESIAN_POINT('Ctrl Pts',(0.577219342712345,-5.25581036421826,
398.975746264313));
#41612=CARTESIAN_POINT('Ctrl Pts',(-1.99939275815206,-4.89480881878609,
398.896618388853));
#41613=CARTESIAN_POINT('Ctrl Pts',(-4.09188543486623,-3.34861140683646,
398.817490513394));
#41614=CARTESIAN_POINT('Ctrl Pts',(-5.19359667913832,-0.991603904073038,
398.738362637933));
#41615=CARTESIAN_POINT('Ctrl Pts',(-5.03776559021372,1.60550385431017,398.659234762474));
#41616=CARTESIAN_POINT('Ctrl Pts',(-3.66212405277363,3.81386578025083,398.580106887014));
#41617=CARTESIAN_POINT('Ctrl Pts',(-1.39976059402284,5.09876407058445,398.500979011554));
#41618=CARTESIAN_POINT('Ctrl Pts',(1.2015314169661,5.14908215334412,398.421851136094));
#41619=CARTESIAN_POINT('Ctrl Pts',(3.51189274640949,3.9526363487746,398.342723260634));
#41620=CARTESIAN_POINT('Ctrl Pts',(4.97190814582059,1.79912594262636,398.263595385175));
#41621=CARTESIAN_POINT('Ctrl Pts',(5.22805937238099,-0.790012637095727,
398.184467509715));
#41622=CARTESIAN_POINT('Ctrl Pts',(4.21832370253235,-3.18786290617544,398.105339634255));
#41623=CARTESIAN_POINT('Ctrl Pts',(2.18719169429123,-4.81382563667766,398.026211758795));
#41624=CARTESIAN_POINT('Ctrl Pts',(-0.37353210098369,-5.27420122269227,
397.947083883336));
#41625=CARTESIAN_POINT('Ctrl Pts',(-2.84381136257153,-4.45751743709679,
397.867956007876));
#41626=CARTESIAN_POINT('Ctrl Pts',(-4.62550939672404,-2.56152056184034,
397.788828132416));
#41627=CARTESIAN_POINT('Ctrl Pts',(-5.2872179056115,-0.0452944422017613,
397.709700256956));
#41628=CARTESIAN_POINT('Ctrl Pts',(-4.66871527142514,2.48189896697567,397.630572381496));
#41629=CARTESIAN_POINT('Ctrl Pts',(-2.91976153402742,4.40814216562114,397.551444506037));
#41630=CARTESIAN_POINT('Ctrl Pts',(-0.463836508948714,5.26702766851281,
397.472316630577));
#41631=CARTESIAN_POINT('Ctrl Pts',(2.10439874769627,4.85059075563045,397.393188755117));
#41632=CARTESIAN_POINT('Ctrl Pts',(4.16308914079174,3.25966464129901,397.314060879657));
#41633=CARTESIAN_POINT('Ctrl Pts',(5.21375731827273,0.87946540242969,397.234933004198));
#41634=CARTESIAN_POINT('Ctrl Pts',(5.00200160188481,-1.71368163398425,397.155805128738));
#41635=CARTESIAN_POINT('Ctrl Pts',(3.57909508696266,-3.89188940315535,397.076677253278));
#41636=CARTESIAN_POINT('Ctrl Pts',(1.28957072230382,-5.12774142484681,396.997549377819));
#41637=CARTESIAN_POINT('Ctrl Pts',(-1.31220156516579,-5.12199685867627,
396.918421502358));
#41638=CARTESIAN_POINT('Ctrl Pts',(-3.59624625077107,-3.87604665499891,
396.839293626899));
#41639=CARTESIAN_POINT('Ctrl Pts',(-5.00952021996834,-1.69157675960673,
396.760165751439));
#41640=CARTESIAN_POINT('Ctrl Pts',(-5.20982288335836,0.90248007842212,396.681037875979));
#41641=CARTESIAN_POINT('Ctrl Pts',(-4.14865431030898,3.27801650109757,396.601910000519));
#41642=CARTESIAN_POINT('Ctrl Pts',(-2.08295867375766,4.85983620416686,396.52278212506));
#41643=CARTESIAN_POINT('Ctrl Pts',(0.487090472013812,5.26492807548086,396.4436542496));
#41644=CARTESIAN_POINT('Ctrl Pts',(2.93919882905869,4.3952059122609,396.36452637414));
#41645=CARTESIAN_POINT('Ctrl Pts',(4.67962948341671,2.46125835008237,396.28539849868));
#41646=CARTESIAN_POINT('Ctrl Pts',(5.2869663411736,-0.0686416434144708,
396.206270623221));
#41647=CARTESIAN_POINT('Ctrl Pts',(4.61415296796628,-2.58192121415839,396.127142747761));
#41648=CARTESIAN_POINT('Ctrl Pts',(2.82409983825713,-4.47003186470401,396.048014872301));
#41649=CARTESIAN_POINT('Ctrl Pts',(0.350238296140284,-5.27579926682488,
395.968886996841));
#41650=CARTESIAN_POINT('Ctrl Pts',(-2.20842757548492,-4.80412035775031,
395.889759121382));
#41651=CARTESIAN_POINT('Ctrl Pts',(-4.23235974759556,-3.16920427471092,
395.810631245921));
#41652=CARTESIAN_POINT('Ctrl Pts',(-5.23149698840249,-0.766918527777797,
395.731503370462));
#41653=CARTESIAN_POINT('Ctrl Pts',(-4.96391497173342,1.82106367854447,395.652375495002));
#41654=CARTESIAN_POINT('Ctrl Pts',(-3.49440419526435,3.96810585645496,395.573247619542));
#41655=CARTESIAN_POINT('Ctrl Pts',(-1.17878204811896,5.1543377509575,395.494119744082));
#41656=CARTESIAN_POINT('Ctrl Pts',(1.42226240243777,5.09253320328156,395.414991868623));
#41657=CARTESIAN_POINT('Ctrl Pts',(3.67892986523249,3.79765714811298,395.335863993163));
#41658=CARTESIAN_POINT('Ctrl Pts',(5.0448061610774,1.58324210563915,395.256736117703));
#41659=CARTESIAN_POINT('Ctrl Pts',(5.18916725226161,-1.01452845991075,395.177608242243));
#41660=CARTESIAN_POINT('Ctrl Pts',(4.07705852165763,-3.36664797371096,395.098480366784));
#41661=CARTESIAN_POINT('Ctrl Pts',(1.97775844702931,-4.90359014326416,395.019352491324));
#41662=CARTESIAN_POINT('Ctrl Pts',(-0.60042266624658,-5.25321019851391,
394.940224615864));
#41663=CARTESIAN_POINT('Ctrl Pts',(-3.03322150067462,-4.33085350661488,
394.861096740404));
#41664=CARTESIAN_POINT('Ctrl Pts',(-4.73157661935314,-2.35985327152006,
394.781968864945));
#41665=CARTESIAN_POINT('Ctrl Pts',(-5.28425981367717,0.182545855799866,
394.702840989484));
#41666=CARTESIAN_POINT('Ctrl Pts',(-4.55744811727866,2.68074456564335,394.623713114025));
#41667=CARTESIAN_POINT('Ctrl Pts',(-2.72712679296628,4.52984593810856,394.544585238565));
#41668=CARTESIAN_POINT('Ctrl Pts',(-0.236477452813074,5.28212108742541,
394.465457363106));
#41669=CARTESIAN_POINT('Ctrl Pts',(2.31143093653793,4.75541920271268,394.386329487645));
#41670=CARTESIAN_POINT('Ctrl Pts',(4.29966508998112,3.07727231195273,394.307201612186));
#41671=CARTESIAN_POINT('Ctrl Pts',(5.2468074522505,0.654015540275394,394.228073736726));
#41672=CARTESIAN_POINT('Ctrl Pts',(4.92352338499734,-1.92760012588128,394.148945861266));
#41673=CARTESIAN_POINT('Ctrl Pts',(3.40809070325859,-4.04247974964323,394.069817985806));
#41674=CARTESIAN_POINT('Ctrl Pts',(1.06744601535546,-5.17854069909805,393.990690110347));
#41675=CARTESIAN_POINT('Ctrl Pts',(-1.53166282285958,-5.06070486839363,
393.911562234887));
#41676=CARTESIAN_POINT('Ctrl Pts',(-3.75990519627929,-3.71750422769163,
393.832434359427));
#41677=CARTESIAN_POINT('Ctrl Pts',(-5.07774958438631,-1.47417228510708,
393.753306483967));
#41678=CARTESIAN_POINT('Ctrl Pts',(-5.16610207037776,1.12610575273896,393.674178608508));
#41679=CARTESIAN_POINT('Ctrl Pts',(-4.00356958154437,3.45371616865744,393.595050733048));
#41680=CARTESIAN_POINT('Ctrl Pts',(-1.8716398630404,4.94506713715712,393.515922857588));
#41681=CARTESIAN_POINT('Ctrl Pts',(0.713476058729831,5.23905303289941,393.436794982128));
#41682=CARTESIAN_POINT('Ctrl Pts',(3.12583571869877,4.26449010171441,393.357667106669));
#41683=CARTESIAN_POINT('Ctrl Pts',(4.78132668327137,2.25735241283907,393.278539231209));
#41684=CARTESIAN_POINT('Ctrl Pts',(5.2790995798779,-0.296365304389928,393.199411355749));
#41685=CARTESIAN_POINT('Ctrl Pts',(4.49862704983328,-2.77832313355043,393.120283480289));
#41686=CARTESIAN_POINT('Ctrl Pts',(2.62888742685924,-4.58755661161959,393.041155604829));
#41687=CARTESIAN_POINT('Ctrl Pts',(0.122606802959192,-5.28599019482455,
392.96202772937));
#41688=CARTESIAN_POINT('Ctrl Pts',(-2.41336100201929,-4.70450990453263,
392.88289985391));
#41689=CARTESIAN_POINT('Ctrl Pts',(-4.3649739152189,-2.98391144093985,392.80377197845));
#41690=CARTESIAN_POINT('Ctrl Pts',(-5.25968160051806,-0.540808865575483,
392.724644102991));
#41691=CARTESIAN_POINT('Ctrl Pts',(-4.88084559720602,2.03324150659673,392.64551622753));
#41692=CARTESIAN_POINT('Ctrl Pts',(-3.32019468996614,4.11497654776232,392.566388352071));
#41693=CARTESIAN_POINT('Ctrl Pts',(-0.955614322062658,5.20033903081154,
392.487260476611));
#41694=CARTESIAN_POINT('Ctrl Pts',(1.64035202716895,5.02652663326038,392.408132601151));
#41695=CARTESIAN_POINT('Ctrl Pts',(3.83913464362559,3.63562511214056,392.329004725691));
#41696=CARTESIAN_POINT('Ctrl Pts',(5.10833519286426,1.36441794376124,392.249876850232));
#41697=CARTESIAN_POINT('Ctrl Pts',(5.14063804785052,-1.23716014683014,392.170748974772));
#41698=CARTESIAN_POINT('Ctrl Pts',(3.92822161400576,-3.53918065647562,392.091621099312));
#41699=CARTESIAN_POINT('Ctrl Pts',(1.76465219715718,-4.98424792631562,392.012493223852));
#41700=CARTESIAN_POINT('Ctrl Pts',(-0.826198153971171,-5.22246315241074,
391.933365348392));
#41701=CARTESIAN_POINT('Ctrl Pts',(-3.21699847841567,-4.19614651290735,
391.854237472933));
#41702=CARTESIAN_POINT('Ctrl Pts',(-4.82885657410346,-2.15380336954211,
391.775109597473));
#41703=CARTESIAN_POINT('Ctrl Pts',(-5.27148803589155,0.41004713797985,391.695981722013));
#41704=CARTESIAN_POINT('Ctrl Pts',(-4.43771707875037,2.8746116080056,391.616853846554));
#41705=CARTESIAN_POINT('Ctrl Pts',(-2.52942735664669,4.64313708771996,391.537725971094));
#41706=CARTESIAN_POINT('Ctrl Pts',(-0.00867922155838994,5.28740479243137,
391.458598095634));
#41707=CARTESIAN_POINT('Ctrl Pts',(2.51417044146968,4.65141610255989,391.379470220174));
#41708=CARTESIAN_POINT('Ctrl Pts',(4.42825589764708,2.88916501309064,391.300342344714));
#41709=CARTESIAN_POINT('Ctrl Pts',(5.27011345519119,0.427351070346123,391.221214469255));
#41710=CARTESIAN_POINT('Ctrl Pts',(4.8359014254693,-2.1379387669101,391.142086593795));
#41711=CARTESIAN_POINT('Ctrl Pts',(3.23075696923981,-4.18556258746916,391.062958718335));
#41712=CARTESIAN_POINT('Ctrl Pts',(0.843338896446427,-5.21972262420654,
390.983830842875));
#41713=CARTESIAN_POINT('Ctrl Pts',(-1.7482795463511,-4.99001436828829,390.904702967415));
#41714=CARTESIAN_POINT('Ctrl Pts',(-3.91658141767327,-3.55205782141137,
390.825575091956));
#41715=CARTESIAN_POINT('Ctrl Pts',(-5.13654878431394,-1.25403004520473,
390.746447216496));
#41716=CARTESIAN_POINT('Ctrl Pts',(-5.11278700870727,1.34764007491144,390.667319341036));
#41717=CARTESIAN_POINT('Ctrl Pts',(-3.85104960630393,3.62300175237324,390.588191465576));
#41718=CARTESIAN_POINT('Ctrl Pts',(-1.65684512829777,5.02111431743484,390.509063590116));
#41719=CARTESIAN_POINT('Ctrl Pts',(0.938536610313288,5.20344826043412,390.429935714657));
#41720=CARTESIAN_POINT('Ctrl Pts',(3.30666744908329,4.12585447502528,390.350807839197));
#41721=CARTESIAN_POINT('Ctrl Pts',(4.874144221702,2.04925422384882,390.271679963737));
#41722=CARTESIAN_POINT('Ctrl Pts',(5.26142871608132,-0.523538569265068,
390.192552088277));
#41723=CARTESIAN_POINT('Ctrl Pts',(4.37474648711696,-2.96956527817979,390.113424212818));
#41724=CARTESIAN_POINT('Ctrl Pts',(2.42879276586438,-4.69656155803349,390.034296337358));
#41725=CARTESIAN_POINT('Ctrl Pts',(-0.105252389973582,-5.28636422338813,
389.955168461898));
#41726=CARTESIAN_POINT('Ctrl Pts',(-2.61381244478399,-4.59616245050211,
389.876040586438));
#41727=CARTESIAN_POINT('Ctrl Pts',(-4.48948165275299,-2.79307702319636,
389.796912710979));
#41728=CARTESIAN_POINT('Ctrl Pts',(-5.27809817231664,-0.313694837861352,
389.717784835519));
#41729=CARTESIAN_POINT('Ctrl Pts',(-4.78871173927535,2.2416432914359,389.638656960059));
#41730=CARTESIAN_POINT('Ctrl Pts',(-3.13981907081257,4.25420509266713,389.559529084599));
#41731=CARTESIAN_POINT('Ctrl Pts',(-0.730671872756092,5.23668247865729,
389.48040120914));
#41732=CARTESIAN_POINT('Ctrl Pts',(1.85539526507438,4.95118502767294,389.401273333679));
#41733=CARTESIAN_POINT('Ctrl Pts',(3.99220955659535,3.46684115934693,389.32214545822));
#41734=CARTESIAN_POINT('Ctrl Pts',(5.16237725796638,1.14305984722794,389.24301758276));
#41735=CARTESIAN_POINT('Ctrl Pts',(5.08256188536855,-1.45749423645932,389.1638897073));
#41736=CARTESIAN_POINT('Ctrl Pts',(3.77208939268016,-3.70514053465492,389.08476183184));
#41737=CARTESIAN_POINT('Ctrl Pts',(1.54826871586373,-5.05564919188336,389.005633956381));
#41738=CARTESIAN_POINT('Ctrl Pts',(-1.05043926423896,-5.18201718639165,
388.926506080921));
#41739=CARTESIAN_POINT('Ctrl Pts',(-3.39480099358967,-4.05364662764723,
388.847378205461));
#41740=CARTESIAN_POINT('Ctrl Pts',(-4.91716859708847,-1.94375352236854,
388.768250330001));
#41741=CARTESIAN_POINT('Ctrl Pts',(-5.2489262914167,0.636786899353102,388.689122454542));
#41742=CARTESIAN_POINT('Ctrl Pts',(-4.30974451485365,3.06314005305047,388.609994579082));
#41743=CARTESIAN_POINT('Ctrl Pts',(-2.32703038342756,4.74780521530929,388.530866703622));
#41744=CARTESIAN_POINT('Ctrl Pts',(0.2191351283499,5.28286897087523,388.451738828163));
#41745=CARTESIAN_POINT('Ctrl Pts',(2.71224074394742,4.53877460497707,388.372610952702));
#41746=CARTESIAN_POINT('Ctrl Pts',(4.54862275081774,2.69569208899244,388.293483077243));
#41747=CARTESIAN_POINT('Ctrl Pts',(5.28363204425109,0.199892943537846,388.214355201783));
#41748=CARTESIAN_POINT('Ctrl Pts',(4.73929845080001,-2.34430692575821,388.135227326323));
#41749=CARTESIAN_POINT('Ctrl Pts',(3.04742322101362,-4.32087218972514,388.056099450863));
#41750=CARTESIAN_POINT('Ctrl Pts',(0.617665567076949,-5.25121071898288,
387.976971575404));
#41751=CARTESIAN_POINT('Ctrl Pts',(-1.96164944496022,-4.9100566415267,387.897843699944));
#41752=CARTESIAN_POINT('Ctrl Pts',(-4.06598394303424,-3.38001469566346,
387.818715824484));
#41753=CARTESIAN_POINT('Ctrl Pts',(-5.18580862056406,-1.03155887800781,
387.739587949024));
#41754=CARTESIAN_POINT('Ctrl Pts',(-5.04997671264308,1.56667162151986,387.660460073564));
#41755=CARTESIAN_POINT('Ctrl Pts',(-3.69137763771595,3.78555886279474,387.581332198105));
#41756=CARTESIAN_POINT('Ctrl Pts',(-1.43897337649567,5.08783651365194,387.502204322645));
#41757=CARTESIAN_POINT('Ctrl Pts',(1.16185415459233,5.15817988164137,387.423076447186));
#41758=CARTESIAN_POINT('Ctrl Pts',(3.48135818778607,3.97955649994419,387.343948571725));
#41759=CARTESIAN_POINT('Ctrl Pts',(4.95790972221771,1.83735025355874,387.264820696266));
#41760=CARTESIAN_POINT('Ctrl Pts',(5.23398656730458,-0.749739542233496,
387.185692820806));
#41761=CARTESIAN_POINT('Ctrl Pts',(4.24274134513742,-3.15529248187465,387.106564945346));
#41762=CARTESIAN_POINT('Ctrl Pts',(2.22418746193322,-4.79684426494046,387.027437069886));
#41763=CARTESIAN_POINT('Ctrl Pts',(-0.332916112977428,-5.27692065788687,
386.948309194427));
#41764=CARTESIAN_POINT('Ctrl Pts',(-2.80940963451955,-4.47927921359921,
386.869181318967));
#41765=CARTESIAN_POINT('Ctrl Pts',(-4.6056517301173,-2.59705543044056,386.790053443507));
#41766=CARTESIAN_POINT('Ctrl Pts',(-5.2867125013827,-0.0859982304292488,
386.710925568047));
#41767=CARTESIAN_POINT('Ctrl Pts',(-4.68768450473212,2.44588199879054,386.631797692588));
#41768=CARTESIAN_POINT('Ctrl Pts',(-2.95361232316089,4.38553292227813,386.552669817127));
#41769=CARTESIAN_POINT('Ctrl Pts',(-0.504372453036948,5.26330059910421,
386.473541941668));
#41770=CARTESIAN_POINT('Ctrl Pts',(2.06699274767947,4.86664830750627,386.394414066208));
#41771=CARTESIAN_POINT('Ctrl Pts',(4.1378703204085,3.29161874757629,386.315286190749));
#41772=CARTESIAN_POINT('Ctrl Pts',(5.20683199193,0.919578912180737,386.236158315288));
#41773=CARTESIAN_POINT('Ctrl Pts',(5.01504662121074,-1.67512153439562,386.157030439829));
#41774=CARTESIAN_POINT('Ctrl Pts',(3.60895181930755,-3.86421939514695,386.077902564369));
#41775=CARTESIAN_POINT('Ctrl Pts',(1.32900986066236,-5.11766133679979,385.998774688909));
#41776=CARTESIAN_POINT('Ctrl Pts',(-1.2727295467071,-5.13194741485647,385.91964681345));
#41777=CARTESIAN_POINT('Ctrl Pts',(-3.5662988394905,-3.90361849510962,385.84051893799));
#41778=CARTESIAN_POINT('Ctrl Pts',(-4.99634867925468,-1.73009382497687,
385.76139106253));
#41779=CARTESIAN_POINT('Ctrl Pts',(-5.21661648089346,0.862344049196109,
385.68226318707));
#41780=CARTESIAN_POINT('Ctrl Pts',(-4.1737680903862,3.24597977436508,385.60313531161));
#41781=CARTESIAN_POINT('Ctrl Pts',(-2.12031175571847,4.84365593601313,385.524007436151));
#41782=CARTESIAN_POINT('Ctrl Pts',(0.446542510511727,5.26852204647746,385.44487956069));
#41783=CARTESIAN_POINT('Ctrl Pts',(2.90527399685678,4.41770390260608,385.365751685231));
#41784=CARTESIAN_POINT('Ctrl Pts',(4.66054210967394,2.4972128487314,385.286623809771));
#41785=CARTESIAN_POINT('Ctrl Pts',(5.2873381133244,-0.0279364153108744,
385.207495934311));
#41786=CARTESIAN_POINT('Ctrl Pts',(4.63389386761938,-2.54632134491165,385.128368058852));
#41787=CARTESIAN_POINT('Ctrl Pts',(2.85842993763932,-4.44815726560116,385.049240183392));
#41788=CARTESIAN_POINT('Ctrl Pts',(0.390845137441743,-5.27294650517633,
384.970112307932));
#41789=CARTESIAN_POINT('Ctrl Pts',(-2.1713762578616,-4.82098018194518,384.890984432472));
#41790=CARTESIAN_POINT('Ctrl Pts',(-4.20783530881936,-3.2016943610792,384.811856557012));
#41791=CARTESIAN_POINT('Ctrl Pts',(-5.2254376100198,-0.807171946801767,
384.732728681553));
#41792=CARTESIAN_POINT('Ctrl Pts',(-4.97778783059681,1.78279361718495,384.653600806093));
#41793=CARTESIAN_POINT('Ctrl Pts',(-3.52485021126398,3.94108560628483,384.574472930633));
#41794=CARTESIAN_POINT('Ctrl Pts',(-1.21842922909547,5.14510981239459,384.495345055173));
#41795=CARTESIAN_POINT('Ctrl Pts',(1.38301395642869,5.10333196688562,384.416217179714));
#41796=CARTESIAN_POINT('Ctrl Pts',(3.64958350715001,3.82586787438508,384.337089304254));
#41797=CARTESIAN_POINT('Ctrl Pts',(5.03246761935876,1.62203404033908,384.257961428794));
#41798=CARTESIAN_POINT('Ctrl Pts',(5.19682409785237,-0.974548133184912,
384.178833553334));
#41799=CARTESIAN_POINT('Ctrl Pts',(4.10285677781212,-3.33515982055948,384.099705677875));
#41800=CARTESIAN_POINT('Ctrl Pts',(2.0154514986864,-4.88821849187982,384.020577802414));
#41801=CARTESIAN_POINT('Ctrl Pts',(-0.559961559389509,-5.25767703647906,
383.941449926955));
#41802=CARTESIAN_POINT('Ctrl Pts',(-2.99978931706339,-4.3540772640303,383.862322051495));
#41803=CARTESIAN_POINT('Ctrl Pts',(-4.71326840155275,-2.39621070501691,
383.783194176035));
#41804=CARTESIAN_POINT('Ctrl Pts',(-5.28550858957794,0.14185808898655,383.704066300575));
#41805=CARTESIAN_POINT('Ctrl Pts',(-4.57795151673967,2.64557832586642,383.624938425116));
#41806=CARTESIAN_POINT('Ctrl Pts',(-2.76192026167378,4.50871614055144,383.545810549656));
#41807=CARTESIAN_POINT('Ctrl Pts',(-0.277136335846315,5.28014395819535,
383.466682674197));
#41808=CARTESIAN_POINT('Ctrl Pts',(2.27475150580887,4.77307347049397,383.387554798736));
#41809=CARTESIAN_POINT('Ctrl Pts',(4.27584642055071,3.11028329188466,383.308426923277));
#41810=CARTESIAN_POINT('Ctrl Pts',(5.24161683545466,0.6943901771998,383.229299047817));
#41811=CARTESIAN_POINT('Ctrl Pts',(4.93821764164047,-1.8896378731662,383.150171172357));
#41812=CARTESIAN_POINT('Ctrl Pts',(3.43911186553428,-4.01612180396144,383.071043296897));
#41813=CARTESIAN_POINT('Ctrl Pts',(1.1072828290795,-5.17016919494313,382.991915421438));
#41814=CARTESIAN_POINT('Ctrl Pts',(-1.49265617402097,-5.07234682509687,
382.912787545978));
#41815=CARTESIAN_POINT('Ctrl Pts',(-3.73117351815568,-3.74634074068643,
382.833659670518));
#41816=CARTESIAN_POINT('Ctrl Pts',(-5.06624977097178,-1.5132210763935,382.754531795058));
#41817=CARTESIAN_POINT('Ctrl Pts',(-5.17461860862547,1.08629969307746,382.675403919598));
#41818=CARTESIAN_POINT('Ctrl Pts',(-4.03004033454984,3.42279121037416,382.596276044139));
#41819=CARTESIAN_POINT('Ctrl Pts',(-1.90965538190854,4.93051124025298,382.517148168679));
#41820=CARTESIAN_POINT('Ctrl Pts',(0.673120594328623,5.24439066369047,382.438020293219));
#41821=CARTESIAN_POINT('Ctrl Pts',(3.09291170766135,4.28842884242289,382.35889241776));
#41822=CARTESIAN_POINT('Ctrl Pts',(4.76380612269667,2.29409589888282,382.2797645423));
#41823=CARTESIAN_POINT('Ctrl Pts',(5.28122477966896,-0.255713891925586,
382.20063666684));
#41824=CARTESIAN_POINT('Ctrl Pts',(4.51988342850276,-2.74360685242242,382.12150879138));
#41825=CARTESIAN_POINT('Ctrl Pts',(2.66412810880644,-4.56718142707082,382.04238091592));
#41826=CARTESIAN_POINT('Ctrl Pts',(0.16329884807764,-5.28488961607806,381.96325304046));
#41827=CARTESIAN_POINT('Ctrl Pts',(-2.37707049000228,-4.72295041827389,
381.884125165001));
#41828=CARTESIAN_POINT('Ctrl Pts',(-4.3418720751543,-3.0174279860352,381.804997289541));
#41829=CARTESIAN_POINT('Ctrl Pts',(-5.25536215553288,-0.581285972741413,
381.725869414081));
#41830=CARTESIAN_POINT('Ctrl Pts',(-4.89635442846138,1.99560469001251,381.646741538622));
#41831=CARTESIAN_POINT('Ctrl Pts',(-3.35177659407457,4.08929314568265,381.567613663161));
#41832=CARTESIAN_POINT('Ctrl Pts',(-0.995622270609436,5.1928278483096,381.488485787702));
#41833=CARTESIAN_POINT('Ctrl Pts',(1.60160528794473,5.03900637720777,381.409357912242));
#41834=CARTESIAN_POINT('Ctrl Pts',(3.81103098679937,3.66507402184023,381.330230036782));
#41835=CARTESIAN_POINT('Ctrl Pts',(5.09767944760569,1.40370545962173,381.251102161322));
#41836=CARTESIAN_POINT('Ctrl Pts',(5.15001032416474,-1.1975468378773,381.171974285863));
#41837=CARTESIAN_POINT('Ctrl Pts',(3.95535257236717,-3.50883325283227,381.092846410403));
#41838=CARTESIAN_POINT('Ctrl Pts',(1.8029725310162,-4.97051454281288,381.013718534943));
#41839=CARTESIAN_POINT('Ctrl Pts',(-0.785967070782117,-5.22866909753901,
380.934590659483));
#41840=CARTESIAN_POINT('Ctrl Pts',(-3.18459792796892,-4.22078912113472,
380.855462784024));
#41841=CARTESIAN_POINT('Ctrl Pts',(-4.81213180629493,-2.19091584657144,
380.776334908564));
#41842=CARTESIAN_POINT('Ctrl Pts',(-5.27448867275235,0.369450956041967,
380.697207033104));
#41843=CARTESIAN_POINT('Ctrl Pts',(-4.45971656638884,2.84036140577044,380.618079157644));
#41844=CARTESIAN_POINT('Ctrl Pts',(-2.56509888808806,4.6235259772432,380.538951282184));
#41845=CARTESIAN_POINT('Ctrl Pts',(-0.0493855337170155,5.28718127521391,
380.459823406725));
#41846=CARTESIAN_POINT('Ctrl Pts',(2.47828569939099,4.67063429954727,380.380695531265));
#41847=CARTESIAN_POINT('Ctrl Pts',(4.40588161411396,2.92317156019379,380.301567655805));
#41848=CARTESIAN_POINT('Ctrl Pts',(5.26666718771851,0.467911852513223,380.222439780345));
#41849=CARTESIAN_POINT('Ctrl Pts',(4.8522176299277,-2.10064486282949,380.143311904886));
#41850=CARTESIAN_POINT('Ctrl Pts',(3.26288495036134,-4.1605656548862,380.064184029426));
#41851=CARTESIAN_POINT('Ctrl Pts',(0.883499402425967,-5.21307525111868,
379.985056153966));
#41852=CARTESIAN_POINT('Ctrl Pts',(-1.70981070849824,-5.0033261046046,379.905928278506));
#41853=CARTESIAN_POINT('Ctrl Pts',(-3.88911883186622,-3.58210545343612,
379.826800403046));
#41854=CARTESIAN_POINT('Ctrl Pts',(-5.1267420551265,-1.29353804277671,379.747672527587));
#41855=CARTESIAN_POINT('Ctrl Pts',(-5.12301067114194,1.3082379108094,379.668544652126));
#41856=CARTESIAN_POINT('Ctrl Pts',(-3.87882817196482,3.59324599495851,379.589416776668));
#41857=CARTESIAN_POINT('Ctrl Pts',(-1.69545248338881,5.00820982432685,379.510288901207));
#41858=CARTESIAN_POINT('Ctrl Pts',(0.898448589337301,5.21051963821565,379.431161025747));
#41859=CARTESIAN_POINT('Ctrl Pts',(3.27480540417913,4.15118950816177,379.352033150288));
#41860=CARTESIAN_POINT('Ctrl Pts',(4.85822301267979,2.08671845896413,379.272905274828));
#41861=CARTESIAN_POINT('Ctrl Pts',(5.26530339668872,-0.483016468385486,
379.193777399368));
#41862=CARTESIAN_POINT('Ctrl Pts',(4.39747886842774,-2.93579705866137,379.114649523908));
#41863=CARTESIAN_POINT('Ctrl Pts',(2.4648785829925,-4.67772362790043,379.035521648449));
#41864=CARTESIAN_POINT('Ctrl Pts',(-0.0645507124447473,-5.28701787148826,
378.956393772989));
#41865=CARTESIAN_POINT('Ctrl Pts',(-2.57835013545374,-4.61614940691036,
378.877265897529));
#41866=CARTESIAN_POINT('Ctrl Pts',(-4.46784531508162,-2.82755778162292,
378.798138022069));
#41867=CARTESIAN_POINT('Ctrl Pts',(-5.27552668260484,-0.354320460935515,
378.719010146609));
#41868=CARTESIAN_POINT('Ctrl Pts',(-4.80582774062997,2.20470961700277,378.63988227115));
#41869=CARTESIAN_POINT('Ctrl Pts',(-3.17247821056078,4.22990623671853,378.56075439569));
#41870=CARTESIAN_POINT('Ctrl Pts',(-0.770966287939471,5.23090200164121,
378.48162652023));
#41871=CARTESIAN_POINT('Ctrl Pts',(1.81722219130848,4.96532257515351,378.40249864477));
#41872=CARTESIAN_POINT('Ctrl Pts',(3.96540079385267,3.49747356130477,378.323370769311));
#41873=CARTESIAN_POINT('Ctrl Pts',(5.15342409853101,1.18276998126983,378.244242893851));
#41874=CARTESIAN_POINT('Ctrl Pts',(5.09363218664291,-1.41832151330666,378.165115018391));
#41875=CARTESIAN_POINT('Ctrl Pts',(3.80050266687247,-3.67599024033094,378.085987142931));
#41876=CARTESIAN_POINT('Ctrl Pts',(1.58714516515185,-5.04357958127442,378.006859267472));
#41877=CARTESIAN_POINT('Ctrl Pts',(-1.01051292004705,-5.18995071328536,
377.927731392012));
#41878=CARTESIAN_POINT('Ctrl Pts',(-3.36349224912901,-4.07966232156074,
377.848603516552));
#41879=CARTESIAN_POINT('Ctrl Pts',(-4.90205833974629,-1.98155211933397,
377.769475641092));
#41880=CARTESIAN_POINT('Ctrl Pts',(-5.25367321659188,0.596357695664665,
377.690347765633));
#41881=CARTESIAN_POINT('Ctrl Pts',(-4.33319923422642,3.02986949626759,377.611219890172));
#41882=CARTESIAN_POINT('Ctrl Pts',(-2.36351373006459,4.72974921277116,377.532092014713));
#41883=CARTESIAN_POINT('Ctrl Pts',(0.178456984968689,5.28439948077629,377.452964139253));
#41884=CARTESIAN_POINT('Ctrl Pts',(2.67721733402229,4.55952104001336,377.373836263793));
#41885=CARTESIAN_POINT('Ctrl Pts',(4.52773440567874,2.73063104786141,377.294708388334));
#41886=CARTESIAN_POINT('Ctrl Pts',(5.28193652635228,0.240564543316707,377.215580512874));
#41887=CARTESIAN_POINT('Ctrl Pts',(4.75720630136386,-2.3077506308472,377.136452637414));
#41888=CARTESIAN_POINT('Ctrl Pts',(3.08059835436342,-4.29728269340077,377.057324761954));
#41889=CARTESIAN_POINT('Ctrl Pts',(0.658075181053442,-5.24629982216222,
376.978196886494));
#41890=CARTESIAN_POINT('Ctrl Pts',(-1.923789860657,-4.92501343550216,376.899069011035));
#41891=CARTESIAN_POINT('Ctrl Pts',(-4.03984145181191,-3.4112176436405,376.819941135575));
#41892=CARTESIAN_POINT('Ctrl Pts',(-5.17771318819473,-1.07145270939303,
376.740813260115));
#41893=CARTESIAN_POINT('Ctrl Pts',(-5.0618885123847,1.52774652882403,376.661685384655));
#41894=CARTESIAN_POINT('Ctrl Pts',(-3.72041242686768,3.75702756739127,376.582557509196));
#41895=CARTESIAN_POINT('Ctrl Pts',(-1.47810086816716,5.0766073897426,376.503429633736));
#41896=CARTESIAN_POINT('Ctrl Pts',(1.12210802704861,5.16697187426544,376.424301758276));
#41897=CARTESIAN_POINT('Ctrl Pts',(3.45061728097363,4.00624077340234,376.345173882816));
#41898=CARTESIAN_POINT('Ctrl Pts',(4.94361743453053,1.87546566308182,376.266046007357));
#41899=CARTESIAN_POINT('Ctrl Pts',(5.23960352937691,-0.709422013391795,
376.186918131896));
#41900=CARTESIAN_POINT('Ctrl Pts',(4.2669075188957,-3.12253502690154,376.107790256437));
#41901=CARTESIAN_POINT('Ctrl Pts',(2.26105138176727,-4.77957859502704,376.028662380977));
#41902=CARTESIAN_POINT('Ctrl Pts',(-0.292280359441297,-5.27932727476591,
375.949534505517));
#41903=CARTESIAN_POINT('Ctrl Pts',(-2.77484145645776,-4.50077558721857,
375.870406630058));
#41904=CARTESIAN_POINT('Ctrl Pts',(-4.58552092957851,-2.63243616845826,
375.791278754598));
#41905=CARTESIAN_POINT('Ctrl Pts',(-5.28589405424394,-0.126697339588848,
375.712150879138));
#41906=CARTESIAN_POINT('Ctrl Pts',(-4.70637522968859,2.40972094307884,375.633023003678));
#41907=CARTESIAN_POINT('Ctrl Pts',(-2.98728944096456,4.36266186682328,375.553895128218));
#41908=CARTESIAN_POINT('Ctrl Pts',(-0.544875549618088,5.2592655277028,375.474767252759));
#41909=CARTESIAN_POINT('Ctrl Pts',(2.02945798133318,4.88240903418803,375.395639377299));
#41910=CARTESIAN_POINT('Ctrl Pts',(4.1124194375256,3.3233956145555,375.316511501839));
#41911=CARTESIAN_POINT('Ctrl Pts',(5.19956989745793,0.959601216722932,375.237383626379));
#41912=CARTESIAN_POINT('Ctrl Pts',(5.02785240284651,-1.63637626402564,375.15825575092));
#41913=CARTESIAN_POINT('Ctrl Pts',(3.63845954881624,-3.83644847785649,375.07912787546));
#41914=CARTESIAN_POINT('Ctrl Pts',(2.1252131908655,-4.68314727417153,375.026375958487));
#41915=CARTESIAN_POINT('Ctrl Pts',(1.3130361863572,-4.90075024188303,375.));
#41916=CARTESIAN_POINT('Ctrl Pts',(3.43378788736214,2.93584158412968,400.));
#41917=CARTESIAN_POINT('Ctrl Pts',(3.5274081047691,2.83896859117363,400.));
#41918=CARTESIAN_POINT('Ctrl Pts',(3.61639766139016,2.73803801067182,400.));
#41919=CARTESIAN_POINT('Ctrl Pts',(3.70064392711817,2.63347462098305,400.));
#41920=CARTESIAN_POINT('Ctrl Pts',(3.7863602040819,2.52708670700993,400.));
#41921=CARTESIAN_POINT('Ctrl Pts',(3.86716669541736,2.4169376104458,400.));
#41922=CARTESIAN_POINT('Ctrl Pts',(3.94291532865978,2.30342952486372,400.));
#41923=CARTESIAN_POINT('Ctrl Pts',(4.0194785589048,2.18870077902246,400.));
#41924=CARTESIAN_POINT('Ctrl Pts',(4.09087506217895,2.07053982333204,400.));
#41925=CARTESIAN_POINT('Ctrl Pts',(4.15691470252894,1.94932444936402,400.));
#41926=CARTESIAN_POINT('Ctrl Pts',(4.22265038067262,1.82866699624951,400.));
#41927=CARTESIAN_POINT('Ctrl Pts',(4.28307881326963,1.70498249960347,400.));
#41928=CARTESIAN_POINT('Ctrl Pts',(4.33796903578875,1.57861622186133,400.));
#41929=CARTESIAN_POINT('Ctrl Pts',(4.35514545623615,1.53907329021963,400.));
#41930=CARTESIAN_POINT('Ctrl Pts',(4.37177922400871,1.4992675947038,400.));
#41931=CARTESIAN_POINT('Ctrl Pts',(4.38786228046478,1.45920932342454,400.));
#41932=CARTESIAN_POINT('Ctrl Pts',(4.39466658849891,1.44226174770453,400.));
#41933=CARTESIAN_POINT('Ctrl Pts',(4.40137035215038,1.4252737748662,400.));
#41934=CARTESIAN_POINT('Ctrl Pts',(4.40797035684919,1.40825358562441,400.));
#41935=CARTESIAN_POINT('Ctrl Pts',(4.45876403554847,1.27726609952389,400.));
#41936=CARTESIAN_POINT('Ctrl Pts',(4.50346815482664,1.14424239282724,400.));
#41937=CARTESIAN_POINT('Ctrl Pts',(4.54192438339399,1.0095915875114,400.));
#41938=CARTESIAN_POINT('Ctrl Pts',(4.54556160496616,0.996856204140475,400.));
#41939=CARTESIAN_POINT('Ctrl Pts',(4.54914290628383,0.984106240915922,400.));
#41940=CARTESIAN_POINT('Ctrl Pts',(4.55266813447105,0.971342029205324,400.));
#41941=CARTESIAN_POINT('Ctrl Pts',(4.58957020263633,0.837726335240427,400.));
#41942=CARTESIAN_POINT('Ctrl Pts',(4.62033177525015,0.702551284224113,400.));
#41943=CARTESIAN_POINT('Ctrl Pts',(4.64501953741251,0.566245432199611,400.));
#41944=CARTESIAN_POINT('Ctrl Pts',(4.66997011124341,0.428488546737278,400.));
#41945=CARTESIAN_POINT('Ctrl Pts',(4.68871702492031,0.289575922051531,400.));
#41946=CARTESIAN_POINT('Ctrl Pts',(4.70127911966368,0.149931994443125,400.));
#41947=CARTESIAN_POINT('Ctrl Pts',(4.71259060845871,0.0241901691579915,
400.));
#41948=CARTESIAN_POINT('Ctrl Pts',(4.71888682786237,-0.102145233205809,
400.));
#41949=CARTESIAN_POINT('Ctrl Pts',(4.72014590598849,-0.228768981279396,
400.));
#41950=CARTESIAN_POINT('Ctrl Pts',(4.72038025896983,-0.252337536919386,
400.));
#41951=CARTESIAN_POINT('Ctrl Pts',(4.72044000678068,-0.275916082362071,
400.));
#41952=CARTESIAN_POINT('Ctrl Pts',(4.72032487691908,-0.299502644881673,
400.));
#41953=CARTESIAN_POINT('Ctrl Pts',(4.7202295663887,-0.319028836890583,400.));
#41954=CARTESIAN_POINT('Ctrl Pts',(4.72001432373552,-0.338562445738198,
400.));
#41955=CARTESIAN_POINT('Ctrl Pts',(4.71967941555818,-0.358084898519809,
400.));
#41956=CARTESIAN_POINT('Ctrl Pts',(4.71723826258667,-0.50038448044343,400.));
#41957=CARTESIAN_POINT('Ctrl Pts',(4.70844382065583,-0.642283037525432,
400.));
#41958=CARTESIAN_POINT('Ctrl Pts',(4.69336920270997,-0.783339178745919,
400.));
#41959=CARTESIAN_POINT('Ctrl Pts',(4.6781762779915,-0.925502339519639,400.));
#41960=CARTESIAN_POINT('Ctrl Pts',(4.65660432919034,-1.06681060067863,400.));
#41961=CARTESIAN_POINT('Ctrl Pts',(4.62867689090467,-1.20682343753469,400.));
#41962=CARTESIAN_POINT('Ctrl Pts',(4.61869343839589,-1.25687498515869,400.));
#41963=CARTESIAN_POINT('Ctrl Pts',(4.6078973313099,-1.30676103650428,400.));
#41964=CARTESIAN_POINT('Ctrl Pts',(4.59628802798414,-1.35646151489045,400.));
#41965=CARTESIAN_POINT('Ctrl Pts',(4.56393613692852,-1.49496288892161,400.));
#41966=CARTESIAN_POINT('Ctrl Pts',(4.5252728763513,-1.63202392528166,400.));
#41967=CARTESIAN_POINT('Ctrl Pts',(4.48051876179014,-1.76728613860278,400.));
#41968=CARTESIAN_POINT('Ctrl Pts',(4.45444111221125,-1.84610169857621,400.));
#41969=CARTESIAN_POINT('Ctrl Pts',(4.42629449108343,-1.92430635496666,400.));
#41970=CARTESIAN_POINT('Ctrl Pts',(4.3961147432142,-2.00182684735068,400.));
#41971=CARTESIAN_POINT('Ctrl Pts',(4.37905752655991,-2.04564046168142,400.));
#41972=CARTESIAN_POINT('Ctrl Pts',(4.36135075314648,-2.08923549081769,400.));
#41973=CARTESIAN_POINT('Ctrl Pts',(4.34300012999985,-2.13259835388101,400.));
#41974=CARTESIAN_POINT('Ctrl Pts',(4.33569114983399,-2.14986960965973,400.));
#41975=CARTESIAN_POINT('Ctrl Pts',(4.32828379731778,-2.1670950989908,400.));
#41976=CARTESIAN_POINT('Ctrl Pts',(4.32077934892109,-2.18427268326289,400.));
#41977=CARTESIAN_POINT('Ctrl Pts',(4.26291559960507,-2.31672204897711,400.));
#41978=CARTESIAN_POINT('Ctrl Pts',(4.19927220468674,-2.44635051906979,400.));
#41979=CARTESIAN_POINT('Ctrl Pts',(4.13013682131626,-2.57280699644751,400.));
#41980=CARTESIAN_POINT('Ctrl Pts',(4.06045781537672,-2.70025782131784,400.));
#41981=CARTESIAN_POINT('Ctrl Pts',(3.98519984558575,-2.82448729912954,400.));
#41982=CARTESIAN_POINT('Ctrl Pts',(3.90460511771477,-2.94512595263581,400.));
#41983=CARTESIAN_POINT('Ctrl Pts',(3.82424500701874,-3.06541341815719,400.));
#41984=CARTESIAN_POINT('Ctrl Pts',(3.73857881602801,-3.18213164834041,400.));
#41985=CARTESIAN_POINT('Ctrl Pts',(3.6477996177404,-3.29489368172134,400.));
#41986=CARTESIAN_POINT('Ctrl Pts',(3.5967838663573,-3.35826326383848,400.));
#41987=CARTESIAN_POINT('Ctrl Pts',(3.54415252096129,-3.42038297838046,400.));
#41988=CARTESIAN_POINT('Ctrl Pts',(3.48993392052895,-3.48117996717138,400.));
#41989=CARTESIAN_POINT('Ctrl Pts',(3.44896085489101,-3.52712432929906,400.));
#41990=CARTESIAN_POINT('Ctrl Pts',(3.40708123835602,-3.57231323683387,400.));
#41991=CARTESIAN_POINT('Ctrl Pts',(3.36432098798037,-3.61672891625407,400.));
#41992=CARTESIAN_POINT('Ctrl Pts',(3.33855500174508,-3.64349241212974,400.));
#41993=CARTESIAN_POINT('Ctrl Pts',(3.31246924398559,-3.66997513430726,400.));
#41994=CARTESIAN_POINT('Ctrl Pts',(3.28606918882681,-3.69617297251379,400.));
#41995=CARTESIAN_POINT('Ctrl Pts',(3.27036247014898,-3.71175938217099,400.));
#41996=CARTESIAN_POINT('Ctrl Pts',(3.25455092639766,-3.72723854435311,400.));
#41997=CARTESIAN_POINT('Ctrl Pts',(3.23863897351742,-3.74260697959096,400.));
#41998=CARTESIAN_POINT('Ctrl Pts',(3.1336340986207,-3.84402511673945,400.));
#41999=CARTESIAN_POINT('Ctrl Pts',(3.02421929001433,-3.94066423251855,400.));
#42000=CARTESIAN_POINT('Ctrl Pts',(2.9108005879282,-4.03233943093569,400.));
#42001=CARTESIAN_POINT('Ctrl Pts',(2.80145832608402,-4.12071968362393,400.));
#42002=CARTESIAN_POINT('Ctrl Pts',(2.6883940765038,-4.20448664484191,400.));
#42003=CARTESIAN_POINT('Ctrl Pts',(2.57193725133249,-4.28344581179871,400.));
#42004=CARTESIAN_POINT('Ctrl Pts',(2.52394060920348,-4.31598812843542,400.));
#42005=CARTESIAN_POINT('Ctrl Pts',(2.47536734937678,-4.34771342641671,400.));
#42006=CARTESIAN_POINT('Ctrl Pts',(2.4262391678432,-4.37860645542617,400.));
#42007=CARTESIAN_POINT('Ctrl Pts',(2.4057205129273,-4.39150909871084,400.));
#42008=CARTESIAN_POINT('Ctrl Pts',(2.38510290902907,-4.40426785187222,400.));
#42009=CARTESIAN_POINT('Ctrl Pts',(2.36439500508045,-4.41687723791363,400.));
#42010=CARTESIAN_POINT('Ctrl Pts',(2.23718127032588,-4.49433979014823,400.));
#42011=CARTESIAN_POINT('Ctrl Pts',(2.10670807231056,-4.56608151115334,400.));
#42012=CARTESIAN_POINT('Ctrl Pts',(1.97337536799814,-4.63189274468176,400.));
#42013=CARTESIAN_POINT('Ctrl Pts',(1.84010399988323,-4.69767370348621,400.));
#42014=CARTESIAN_POINT('Ctrl Pts',(1.70397511685538,-4.75753010362705,400.));
#42015=CARTESIAN_POINT('Ctrl Pts',(1.56535633801641,-4.81121182598771,400.));
#42016=CARTESIAN_POINT('Ctrl Pts',(1.52584133805609,-4.82651446589492,400.));
#42017=CARTESIAN_POINT('Ctrl Pts',(1.48612384295406,-4.84131506971587,400.));
#42018=CARTESIAN_POINT('Ctrl Pts',(1.44621200692229,-4.85560715259022,400.));
#42019=CARTESIAN_POINT('Ctrl Pts',(1.4021027224054,-4.87140230542011,400.));
#42020=CARTESIAN_POINT('Ctrl Pts',(1.35775607141996,-4.88657636029028,400.));
#42021=CARTESIAN_POINT('Ctrl Pts',(1.31318543090145,-4.90112867346808,400.));
#42022=CARTESIAN_POINT('Ctrl Pts',(-4.51746064445937,-7.62825515632226E-5,
398.387416697508));
#42023=CARTESIAN_POINT('Ctrl Pts',(-4.51763289072636,-0.284226777710601,
398.397425295273));
#42024=CARTESIAN_POINT('Ctrl Pts',(-4.49123863994107,-0.568345670691312,
398.407433893039));
#42025=CARTESIAN_POINT('Ctrl Pts',(-4.4379719366677,-0.847333855511198,
398.417442490804));
#42026=CARTESIAN_POINT('Ctrl Pts',(-4.29759659267063,-1.58255980359031,
398.443818449291));
#42027=CARTESIAN_POINT('Ctrl Pts',(-3.97059302033473,-2.2821531656744,398.470194407778));
#42028=CARTESIAN_POINT('Ctrl Pts',(-3.49655043505552,-2.86141654221982,
398.496570366264));
#42029=CARTESIAN_POINT('Ctrl Pts',(-3.0225078497763,-3.44067991876523,398.522946324751));
#42030=CARTESIAN_POINT('Ctrl Pts',(-2.40142625155378,-3.89961330977197,
398.549322283237));
#42031=CARTESIAN_POINT('Ctrl Pts',(-1.70849788678631,-4.18265520276417,
398.575698241724));
#42032=CARTESIAN_POINT('Ctrl Pts',(-1.01556952201883,-4.46569709575638,
398.60207420021));
#42033=CARTESIAN_POINT('Ctrl Pts',(-0.250794390706405,-4.57284749073406,
398.628450158697));
#42034=CARTESIAN_POINT('Ctrl Pts',(0.493238771257572,-4.49113405337507,
398.654826117184));
#42035=CARTESIAN_POINT('Ctrl Pts',(1.23727193322155,-4.40942061601609,398.68120207567));
#42036=CARTESIAN_POINT('Ctrl Pts',(1.96056312583708,-4.13884334632044,398.707578034157));
#42037=CARTESIAN_POINT('Ctrl Pts',(2.57554593307285,-3.71216011566315,398.733953992643));
#42038=CARTESIAN_POINT('Ctrl Pts',(3.19052874030862,-3.28547688500585,398.76032995113));
#42039=CARTESIAN_POINT('Ctrl Pts',(3.69720316216463,-2.70268769338692,398.786705909617));
#42040=CARTESIAN_POINT('Ctrl Pts',(4.03422784198701,-2.03434886067149,398.813081868103));
#42041=CARTESIAN_POINT('Ctrl Pts',(4.37125252180939,-1.36601002795605,398.83945782659));
#42042=CARTESIAN_POINT('Ctrl Pts',(4.53862745959814,-0.612121554144129,
398.865833785076));
#42043=CARTESIAN_POINT('Ctrl Pts',(4.51608913784387,0.136045847258709,398.892209743563));
#42044=CARTESIAN_POINT('Ctrl Pts',(4.49355081608961,0.884213248661547,398.91858570205));
#42045=CARTESIAN_POINT('Ctrl Pts',(4.28109923479233,1.6266595776553,398.944961660536));
#42046=CARTESIAN_POINT('Ctrl Pts',(3.90445518858537,2.27349934610636,398.971337619023));
#42047=CARTESIAN_POINT('Ctrl Pts',(3.5278111423784,2.92033911455742,398.997713577509));
#42048=CARTESIAN_POINT('Ctrl Pts',(2.98697463126176,3.47157232246578,399.024089535996));
#42049=CARTESIAN_POINT('Ctrl Pts',(2.34742289856565,3.86046308384535,399.050465494483));
#42050=CARTESIAN_POINT('Ctrl Pts',(1.70787116586954,4.24935384522491,399.076841452969));
#42051=CARTESIAN_POINT('Ctrl Pts',(0.969604211593966,4.47590216007566,399.103217411456));
#42052=CARTESIAN_POINT('Ctrl Pts',(0.222001520718283,4.51268048034993,399.129593369942));
#42053=CARTESIAN_POINT('Ctrl Pts',(-0.525601170157399,4.5494588006242,399.155969328429));
#42054=CARTESIAN_POINT('Ctrl Pts',(-1.28253959763319,4.39646712632199,399.182345286915));
#42055=CARTESIAN_POINT('Ctrl Pts',(-1.95717379804064,4.07222787544583,399.208721245402));
#42056=CARTESIAN_POINT('Ctrl Pts',(-2.63180799844808,3.74798862456968,399.235097203889));
#42057=CARTESIAN_POINT('Ctrl Pts',(-3.22413797178719,3.25250179711959,399.261473162375));
#42058=CARTESIAN_POINT('Ctrl Pts',(-3.66245231437547,2.64575381071457,399.287849120862));
#42059=CARTESIAN_POINT('Ctrl Pts',(-4.10076665696376,2.03900582430954,399.314225079348));
#42060=CARTESIAN_POINT('Ctrl Pts',(-4.38506536880122,1.32099667894959,399.340601037835));
#42061=CARTESIAN_POINT('Ctrl Pts',(-4.48092940799817,0.578654358541173,
399.366976996322));
#42062=CARTESIAN_POINT('Ctrl Pts',(-4.50569226564232,0.386898228114258,
399.37379023005));
#42063=CARTESIAN_POINT('Ctrl Pts',(-4.51788177656568,0.193518461005119,
399.380603463779));
#42064=CARTESIAN_POINT('Ctrl Pts',(-4.51769110620511,0.00011483889287206,
399.387416697508));
#42065=CARTESIAN_POINT('Ctrl Pts',(-1.31303618635555,-4.90075024188347,
400.));
#42066=CARTESIAN_POINT('Ctrl Pts',(-2.12521319086393,-4.68314727417224,
399.973624041513));
#42067=CARTESIAN_POINT('Ctrl Pts',(-3.63845957255092,-3.83644859241818,
399.92087212454));
#42068=CARTESIAN_POINT('Ctrl Pts',(-5.02785239518849,-1.63637624738159,
399.84174424908));
#42069=CARTESIAN_POINT('Ctrl Pts',(-5.19956989353463,0.959601198026513,
399.76261637362));
#42070=CARTESIAN_POINT('Ctrl Pts',(-4.11241943286933,3.32339561801255,399.683488498161));
#42071=CARTESIAN_POINT('Ctrl Pts',(-2.02945797892606,4.8824090247121,399.604360622701));
#42072=CARTESIAN_POINT('Ctrl Pts',(0.54487554882432,5.2592655238007,399.525232747241));
#42073=CARTESIAN_POINT('Ctrl Pts',(2.98728943775363,4.36266186092565,399.446104871781));
#42074=CARTESIAN_POINT('Ctrl Pts',(4.70637522433117,2.40972094089285,399.366976996322));
#42075=CARTESIAN_POINT('Ctrl Pts',(5.28589404837916,-0.126697339701679,
399.287849120862));
#42076=CARTESIAN_POINT('Ctrl Pts',(4.58552092441564,-2.6324361653814,399.208721245402));
#42077=CARTESIAN_POINT('Ctrl Pts',(2.77484145336967,-4.50077558224301,399.129593369943));
#42078=CARTESIAN_POINT('Ctrl Pts',(0.292280359106768,-5.27932726882375,
399.050465494482));
#42079=CARTESIAN_POINT('Ctrl Pts',(-2.26105137922953,-4.77957858969287,
398.971337619023));
#42080=CARTESIAN_POINT('Ctrl Pts',(-4.26690751412045,-3.12253502339944,
398.892209743563));
#42081=CARTESIAN_POINT('Ctrl Pts',(-5.23960352350959,-0.709422012603199,
398.813081868103));
#42082=CARTESIAN_POINT('Ctrl Pts',(-4.94361742899746,1.87546566098248,398.733953992643));
#42083=CARTESIAN_POINT('Ctrl Pts',(-3.45061727711166,4.00624076891526,398.654826117184));
#42084=CARTESIAN_POINT('Ctrl Pts',(-1.12210802579434,5.16697186848109,398.575698241724));
#42085=CARTESIAN_POINT('Ctrl Pts',(1.47810086651078,5.07660738405961,398.496570366264));
#42086=CARTESIAN_POINT('Ctrl Pts',(3.72041242270134,3.75702756318667,398.417442490805));
#42087=CARTESIAN_POINT('Ctrl Pts',(5.06188850671742,1.52774652711538,398.338314615344));
#42088=CARTESIAN_POINT('Ctrl Pts',(5.17771318239863,-1.0714527081918,398.259186739885));
#42089=CARTESIAN_POINT('Ctrl Pts',(4.03984144729043,-3.41121763982034,398.180058864425));
#42090=CARTESIAN_POINT('Ctrl Pts',(1.92378985850489,-4.92501342998799,398.100930988965));
#42091=CARTESIAN_POINT('Ctrl Pts',(-0.658075180315041,-5.24629981628919,
398.021803113506));
#42092=CARTESIAN_POINT('Ctrl Pts',(-3.08059835091328,-4.29728268859095,
397.942675238046));
#42093=CARTESIAN_POINT('Ctrl Pts',(-4.75720629603741,-2.30775062826524,
397.863547362586));
#42094=CARTESIAN_POINT('Ctrl Pts',(-5.28193652043922,0.240564543045645,
397.784419487126));
#42095=CARTESIAN_POINT('Ctrl Pts',(-4.52773440061085,2.73063104480294,397.705291611666));
#42096=CARTESIAN_POINT('Ctrl Pts',(-2.67721733102668,4.55952103490808,397.626163736206));
#42097=CARTESIAN_POINT('Ctrl Pts',(-0.178456984770649,5.28439947486034,
397.547035860747));
#42098=CARTESIAN_POINT('Ctrl Pts',(2.36351372741711,4.72974920747697,397.467907985287));
#42099=CARTESIAN_POINT('Ctrl Pts',(4.33319922937441,3.02986949287705,397.388780109827));
#42100=CARTESIAN_POINT('Ctrl Pts',(5.25367321071018,0.596357694998765,397.309652234368));
#42101=CARTESIAN_POINT('Ctrl Pts',(4.90205833425909,-1.98155211711401,397.230524358907));
#42102=CARTESIAN_POINT('Ctrl Pts',(3.36349224536493,-4.07966231699243,397.151396483448));
#42103=CARTESIAN_POINT('Ctrl Pts',(1.01051291891753,-5.18995070747486,397.072268607988));
#42104=CARTESIAN_POINT('Ctrl Pts',(-1.58714516337332,-5.04357957562867,
396.993140732529));
#42105=CARTESIAN_POINT('Ctrl Pts',(-3.80050266261658,-3.67599023621695,
396.914012857068));
#42106=CARTESIAN_POINT('Ctrl Pts',(-5.09363218094012,-1.41832151172053,
396.834884981609));
#42107=CARTESIAN_POINT('Ctrl Pts',(-5.15342409276215,1.182769979944,396.755757106149));
#42108=CARTESIAN_POINT('Ctrl Pts',(-3.96540078941456,3.49747355738801,396.676629230689));
#42109=CARTESIAN_POINT('Ctrl Pts',(-1.81722218927578,4.96532256959422,396.597501355229));
#42110=CARTESIAN_POINT('Ctrl Pts',(0.770966287074601,5.23090199578547,396.51837347977));
#42111=CARTESIAN_POINT('Ctrl Pts',(3.17247820700774,4.22990623198423,396.43924560431));
#42112=CARTESIAN_POINT('Ctrl Pts',(4.8058277352491,2.20470961453625,396.36011772885));
#42113=CARTESIAN_POINT('Ctrl Pts',(5.275526676699,-0.354320460537079,396.28098985339));
#42114=CARTESIAN_POINT('Ctrl Pts',(4.46784531008081,-2.82755777845599,396.201861977931));
#42115=CARTESIAN_POINT('Ctrl Pts',(2.57835013256881,-4.61614940174172,396.122734102471));
#42116=CARTESIAN_POINT('Ctrl Pts',(0.0645507123742531,-5.2870178655694,
396.043606227011));
#42117=CARTESIAN_POINT('Ctrl Pts',(-2.46487858023149,-4.67772362266456,
395.964478351551));
#42118=CARTESIAN_POINT('Ctrl Pts',(-4.39747886350376,-2.93579705537622,
395.885350476092));
#42119=CARTESIAN_POINT('Ctrl Pts',(-5.26530339079403,-0.48301646784655,
395.806222600631));
#42120=CARTESIAN_POINT('Ctrl Pts',(-4.85822300724173,2.08671845662638,395.727094725172));
#42121=CARTESIAN_POINT('Ctrl Pts',(-3.27480540051438,4.15118950351341,395.647966849712));
#42122=CARTESIAN_POINT('Ctrl Pts',(-0.898448588333209,5.21051963238218,
395.568838974252));
#42123=CARTESIAN_POINT('Ctrl Pts',(1.69545248148909,5.00820981872071,395.489711098793));
#42124=CARTESIAN_POINT('Ctrl Pts',(3.87882816762124,3.59324599093717,395.410583223333));
#42125=CARTESIAN_POINT('Ctrl Pts',(5.12301066540628,1.30823790934658,395.331455347873));
#42126=CARTESIAN_POINT('Ctrl Pts',(5.12674204938754,-1.29353804132683,395.252327472413));
#42127=CARTESIAN_POINT('Ctrl Pts',(3.88911882751359,-3.58210544942458,395.173199596953));
#42128=CARTESIAN_POINT('Ctrl Pts',(1.70981070658587,-5.00332609900278,395.094071721494));
#42129=CARTESIAN_POINT('Ctrl Pts',(-0.883499401435098,-5.21307524528295,
395.014943846034));
#42130=CARTESIAN_POINT('Ctrl Pts',(-3.26288494670713,-4.16056565022955,
394.935815970574));
#42131=CARTESIAN_POINT('Ctrl Pts',(-4.85221762449495,-2.10064486047942,
394.856688095114));
#42132=CARTESIAN_POINT('Ctrl Pts',(-5.26666718182262,0.467911851987696,
394.777560219655));
#42133=CARTESIAN_POINT('Ctrl Pts',(-4.40588160918252,2.92317155691987,394.698432344195));
#42134=CARTESIAN_POINT('Ctrl Pts',(-2.47828569661807,4.67063429431767,394.619304468735));
#42135=CARTESIAN_POINT('Ctrl Pts',(0.0493855336599835,5.28718126929493,
394.540176593275));
#42136=CARTESIAN_POINT('Ctrl Pts',(2.56509888521489,4.623525972068,394.461048717816));
#42137=CARTESIAN_POINT('Ctrl Pts',(4.45971656139522,2.84036140259214,394.381920842355));
#42138=CARTESIAN_POINT('Ctrl Pts',(5.27448866684743,0.369450955630144,394.302792966896));
#42139=CARTESIAN_POINT('Ctrl Pts',(4.81213180090847,-2.19091584411711,394.223665091436));
#42140=CARTESIAN_POINT('Ctrl Pts',(3.18459792440514,-4.2207891164085,394.144537215977));
#42141=CARTESIAN_POINT('Ctrl Pts',(0.785967069903959,-5.22866909168525,
394.065409340517));
#42142=CARTESIAN_POINT('Ctrl Pts',(-1.8029725289961,-4.97051453724898,393.986281465057));
#42143=CARTESIAN_POINT('Ctrl Pts',(-3.95535256793798,-3.50883324890547,
393.907153589597));
#42144=CARTESIAN_POINT('Ctrl Pts',(-5.15001031839888,-1.19754683653839,
393.828025714137));
#42145=CARTESIAN_POINT('Ctrl Pts',(-5.0976794418993,1.40370545804854,393.748897838677));
#42146=CARTESIAN_POINT('Ctrl Pts',(-3.81103098253419,3.66507401773587,393.669769963218));
#42147=CARTESIAN_POINT('Ctrl Pts',(-1.60160528615343,5.03900637156607,393.590642087758));
#42148=CARTESIAN_POINT('Ctrl Pts',(0.995622269493122,5.19282784249655,393.511514212298));
#42149=CARTESIAN_POINT('Ctrl Pts',(3.3517765903209,4.08929314110579,393.432386336838));
#42150=CARTESIAN_POINT('Ctrl Pts',(4.89635442297923,1.99560468778007,393.353258461378));
#42151=CARTESIAN_POINT('Ctrl Pts',(5.2553621496497,-0.581285972088894,393.274130585919));
#42152=CARTESIAN_POINT('Ctrl Pts',(4.34187207029457,-3.01742798265574,393.195002710459));
#42153=CARTESIAN_POINT('Ctrl Pts',(2.37707048734272,-4.72295041298575,393.115874834999));
#42154=CARTESIAN_POINT('Ctrl Pts',(-0.163298847893048,-5.28488961016167,
393.03674695954));
#42155=CARTESIAN_POINT('Ctrl Pts',(-2.66412810582239,-4.56718142195876,
392.957619084079));
#42156=CARTESIAN_POINT('Ctrl Pts',(-4.51988342344183,-2.74360684935247,
392.87849120862));
#42157=CARTESIAN_POINT('Ctrl Pts',(-5.28122477375654,-0.255713891641081,
392.79936333316));
#42158=CARTESIAN_POINT('Ctrl Pts',(-4.76380611736435,2.29409589631297,392.7202354577));
#42159=CARTESIAN_POINT('Ctrl Pts',(-3.09291170420029,4.28842883762094,392.64110758224));
#42160=CARTESIAN_POINT('Ctrl Pts',(-0.67312059357683,5.24439065781915,392.561979706781));
#42161=CARTESIAN_POINT('Ctrl Pts',(1.90965537976903,4.9305112347339,392.482851831321));
#42162=CARTESIAN_POINT('Ctrl Pts',(4.03004033003705,3.4227912065437,392.403723955861));
#42163=CARTESIAN_POINT('Ctrl Pts',(5.17461860283211,1.0862996918631,392.324596080401));
#42164=CARTESIAN_POINT('Ctrl Pts',(5.06624976530063,-1.51322107469774,392.245468204942));
#42165=CARTESIAN_POINT('Ctrl Pts',(3.73117351397988,-3.74634073649114,392.166340329482));
#42166=CARTESIAN_POINT('Ctrl Pts',(1.49265617235166,-5.07234681941786,392.087212454022));
#42167=CARTESIAN_POINT('Ctrl Pts',(-1.10728282783815,-5.1701691891555,392.008084578562));
#42168=CARTESIAN_POINT('Ctrl Pts',(-3.43911186168285,-4.01612179946654,
391.928956703103));
#42169=CARTESIAN_POINT('Ctrl Pts',(-4.93821763611149,-1.8896378710524,391.849828827643));
#42170=CARTESIAN_POINT('Ctrl Pts',(-5.24161682958689,0.694390176420624,
391.770700952183));
#42171=CARTESIAN_POINT('Ctrl Pts',(-4.27584641576499,3.1102832884012,391.691573076723));
#42172=CARTESIAN_POINT('Ctrl Pts',(-2.27475150326393,4.77307346514974,391.612445201264));
#42173=CARTESIAN_POINT('Ctrl Pts',(0.277136335534271,5.28014395228432,391.533317325804));
#42174=CARTESIAN_POINT('Ctrl Pts',(2.76192025858026,4.50871613550486,391.454189450344));
#42175=CARTESIAN_POINT('Ctrl Pts',(4.57795151161372,2.64557832290629,391.375061574885));
#42176=CARTESIAN_POINT('Ctrl Pts',(5.28550858366077,0.141858088829558,391.295933699424));
#42177=CARTESIAN_POINT('Ctrl Pts',(4.71326839627705,-2.39621070233275,391.216805823965));
#42178=CARTESIAN_POINT('Ctrl Pts',(2.99978931370662,-4.35407725915487,391.137677948505));
#42179=CARTESIAN_POINT('Ctrl Pts',(0.559961558764467,-5.2576770305929,391.058550073045));
#42180=CARTESIAN_POINT('Ctrl Pts',(-2.01545149642842,-4.88821848640817,
390.979422197585));
#42181=CARTESIAN_POINT('Ctrl Pts',(-4.10285677321784,-3.33515981682715,
390.900294322126));
#42182=CARTESIAN_POINT('Ctrl Pts',(-5.19682409203417,-0.974548132095691,
390.821166446665));
#42183=CARTESIAN_POINT('Ctrl Pts',(-5.03246761372548,1.62203403852146,390.742038571206));
#42184=CARTESIAN_POINT('Ctrl Pts',(-3.64958350306562,3.82586787010077,390.662910695746));
#42185=CARTESIAN_POINT('Ctrl Pts',(-1.38301395488213,5.10333196117197,390.583782820286));
#42186=CARTESIAN_POINT('Ctrl Pts',(1.21842922772966,5.14510980663504,390.504654944826));
#42187=CARTESIAN_POINT('Ctrl Pts',(3.52485020731651,3.94108560187402,390.425527069367));
#42188=CARTESIAN_POINT('Ctrl Pts',(4.97778782502355,1.78279361519087,390.346399193907));
#42189=CARTESIAN_POINT('Ctrl Pts',(5.2254376041702,-0.807171945896316,390.267271318447));
#42190=CARTESIAN_POINT('Ctrl Pts',(4.2078353041098,-3.20169435749343,390.188143442988));
#42191=CARTESIAN_POINT('Ctrl Pts',(2.17137625543244,-4.82098017654731,390.109015567527));
#42192=CARTESIAN_POINT('Ctrl Pts',(-0.390845137002325,-5.27294649927341,
390.029887692068));
#42193=CARTESIAN_POINT('Ctrl Pts',(-2.85842993443779,-4.44815726062243,
389.950759816608));
#42194=CARTESIAN_POINT('Ctrl Pts',(-4.63389386243089,-2.54632134206259,
389.871631941148));
#42195=CARTESIAN_POINT('Ctrl Pts',(-5.2873381074052,-0.0279364152813674,
389.792504065688));
#42196=CARTESIAN_POINT('Ctrl Pts',(-4.66054210445731,2.49721284593419,389.713376190229));
#42197=CARTESIAN_POINT('Ctrl Pts',(-2.90527399360582,4.41770389765948,389.634248314769));
#42198=CARTESIAN_POINT('Ctrl Pts',(-0.446542510013585,5.2685220405792,389.55512043931));
#42199=CARTESIAN_POINT('Ctrl Pts',(2.12031175334316,4.84365593059135,389.475992563849));
#42200=CARTESIAN_POINT('Ctrl Pts',(4.17376808571255,3.24597977073262,389.39686468839));
#42201=CARTESIAN_POINT('Ctrl Pts',(5.21661647505316,0.862344048232485,389.31773681293));
#42202=CARTESIAN_POINT('Ctrl Pts',(4.99634867366186,-1.73009382303836,389.23860893747));
#42203=CARTESIAN_POINT('Ctrl Pts',(3.56629883549932,-3.90361849073832,389.15948106201));
#42204=CARTESIAN_POINT('Ctrl Pts',(1.27272954528402,-5.13194740911081,389.08035318655));
#42205=CARTESIAN_POINT('Ctrl Pts',(-1.3290098591728,-5.11766133107102,389.001225311091));
#42206=CARTESIAN_POINT('Ctrl Pts',(-3.60895181526604,-3.86421939082217,
388.922097435631));
#42207=CARTESIAN_POINT('Ctrl Pts',(-5.01504661559582,-1.67512153252199,
388.842969560171));
#42208=CARTESIAN_POINT('Ctrl Pts',(-5.20683198610126,0.919578911149497,
388.763841684712));
#42209=CARTESIAN_POINT('Ctrl Pts',(-4.13787031577727,3.29161874388992,388.684713809251));
#42210=CARTESIAN_POINT('Ctrl Pts',(-2.0669927453671,4.86664830205737,388.605585933792));
#42211=CARTESIAN_POINT('Ctrl Pts',(0.504372452470541,5.2633005932121,388.526458058332));
#42212=CARTESIAN_POINT('Ctrl Pts',(2.95361231985281,4.38553291736953,388.447330182872));
#42213=CARTESIAN_POINT('Ctrl Pts',(4.68768449948338,2.44588199605403,388.368202307412));
#42214=CARTESIAN_POINT('Ctrl Pts',(5.28671249546426,-0.0859982303311033,
388.289074431953));
#42215=CARTESIAN_POINT('Ctrl Pts',(4.60565172496217,-2.59705542753155,388.209946556493));
#42216=CARTESIAN_POINT('Ctrl Pts',(2.80940963137597,-4.47927920858367,388.130818681033));
#42217=CARTESIAN_POINT('Ctrl Pts',(0.332916112606594,-5.27692065197923,
388.051690805573));
#42218=CARTESIAN_POINT('Ctrl Pts',(-2.22418745944155,-4.79684425957118,
387.972562930114));
#42219=CARTESIAN_POINT('Ctrl Pts',(-4.24274134038657,-3.15529247834378,
387.893435054654));
#42220=CARTESIAN_POINT('Ctrl Pts',(-5.23398656144486,-0.749739541395986,
387.814307179194));
#42221=CARTESIAN_POINT('Ctrl Pts',(-4.95790971666796,1.83735025150007,387.735179303734));
#42222=CARTESIAN_POINT('Ctrl Pts',(-3.48135818389009,3.97955649548785,387.656051428275));
#42223=CARTESIAN_POINT('Ctrl Pts',(-1.16185415329344,5.15817987586638,387.576923552815));
#42224=CARTESIAN_POINT('Ctrl Pts',(1.43897337488296,5.0878365079566,387.497795677355));
#42225=CARTESIAN_POINT('Ctrl Pts',(3.69137763358211,3.7855588585581,387.418667801895));
#42226=CARTESIAN_POINT('Ctrl Pts',(5.04997670698908,1.56667161976776,387.339539926436));
#42227=CARTESIAN_POINT('Ctrl Pts',(5.1858086147589,-1.03155887685117,387.260412050976));
#42228=CARTESIAN_POINT('Ctrl Pts',(4.06598393848355,-3.38001469187811,387.181284175516));
#42229=CARTESIAN_POINT('Ctrl Pts',(1.96164944276588,-4.91005663602919,387.102156300056));
#42230=CARTESIAN_POINT('Ctrl Pts',(-0.617665566383616,-5.25121071310437,
387.023028424596));
#42231=CARTESIAN_POINT('Ctrl Pts',(-3.04742321760052,-4.32087218488899,
386.943900549136));
#42232=CARTESIAN_POINT('Ctrl Pts',(-4.73929844549354,-2.34430692313541,
386.864772673677));
#42233=CARTESIAN_POINT('Ctrl Pts',(-5.28363203833613,0.199892943312196,
386.785644798217));
#42234=CARTESIAN_POINT('Ctrl Pts',(-4.54862274572651,2.695692085973,386.706516922757));
#42235=CARTESIAN_POINT('Ctrl Pts',(-2.71224074091265,4.53877459989496,386.627389047297));
#42236=CARTESIAN_POINT('Ctrl Pts',(-0.219135128106394,5.28286896496098,
386.548261171838));
#42237=CARTESIAN_POINT('Ctrl Pts',(2.32703038082081,4.74780520999492,386.469133296378));
#42238=CARTESIAN_POINT('Ctrl Pts',(4.30974451002784,3.06314004962277,386.390005420918));
#42239=CARTESIAN_POINT('Ctrl Pts',(5.24892628554031,0.636786898642001,386.310877545458));
#42240=CARTESIAN_POINT('Ctrl Pts',(4.91716859158436,-1.94375352019086,386.231749669999));
#42241=CARTESIAN_POINT('Ctrl Pts',(3.39480098979053,-4.05364662310803,386.152621794539));
#42242=CARTESIAN_POINT('Ctrl Pts',(1.05043926306477,-5.18201718059,386.073493919079));
#42243=CARTESIAN_POINT('Ctrl Pts',(-1.54826871412865,-5.0556491862241,385.994366043619));
#42244=CARTESIAN_POINT('Ctrl Pts',(-3.772089388456,-3.70514053050835,385.91523816816));
#42245=CARTESIAN_POINT('Ctrl Pts',(-5.08256187967811,-1.45749423482943,
385.836110292699));
#42246=CARTESIAN_POINT('Ctrl Pts',(-5.16237725218749,1.14305984594648,385.75698241724));
#42247=CARTESIAN_POINT('Ctrl Pts',(-3.99220955212729,3.46684115546438,385.67785454178));
#42248=CARTESIAN_POINT('Ctrl Pts',(-1.85539526299902,4.95118502212943,385.59872666632));
#42249=CARTESIAN_POINT('Ctrl Pts',(0.73067187193628,5.23668247279509,385.51959879086));
#42250=CARTESIAN_POINT('Ctrl Pts',(3.13981906729605,4.25420508790564,385.440470915401));
#42251=CARTESIAN_POINT('Ctrl Pts',(4.78871173391359,2.24164328892807,385.361343039941));
#42252=CARTESIAN_POINT('Ctrl Pts',(5.27809816640793,-0.313694837508304,
385.282215164481));
#42253=CARTESIAN_POINT('Ctrl Pts',(4.48948164772799,-2.79307702006795,385.203087289022));
#42254=CARTESIAN_POINT('Ctrl Pts',(2.61381244185943,-4.59616244535579,385.123959413562));
#42255=CARTESIAN_POINT('Ctrl Pts',(0.105252389857621,-5.28636421747,385.044831538102));
#42256=CARTESIAN_POINT('Ctrl Pts',(-2.42879276314368,-4.69656155277656,
384.965703662642));
#42257=CARTESIAN_POINT('Ctrl Pts',(-4.3747464822184,-2.96956527485689,384.886575787182));
#42258=CARTESIAN_POINT('Ctrl Pts',(-5.26142871019096,-0.5235385686808,384.807447911723));
#42259=CARTESIAN_POINT('Ctrl Pts',(-4.87414421624611,2.04925422155296,384.728320036263));
#42260=CARTESIAN_POINT('Ctrl Pts',(-3.30666744538294,4.12585447040522,384.649192160803));
#42261=CARTESIAN_POINT('Ctrl Pts',(-0.93853660926441,5.20344825460853,384.570064285343));
#42262=CARTESIAN_POINT('Ctrl Pts',(1.65684512644118,5.02111431181428,384.490936409884));
#42263=CARTESIAN_POINT('Ctrl Pts',(3.85104960199139,3.62300174831864,384.411808534424));
#42264=CARTESIAN_POINT('Ctrl Pts',(5.11278700298303,1.34764007340457,384.332680658964));
#42265=CARTESIAN_POINT('Ctrl Pts',(5.13654877856401,-1.25403004379905,384.253552783504));
#42266=CARTESIAN_POINT('Ctrl Pts',(3.91658141328989,-3.55205781743347,384.174424908044));
#42267=CARTESIAN_POINT('Ctrl Pts',(1.74827954439566,-4.99001436270134,384.095297032584));
#42268=CARTESIAN_POINT('Ctrl Pts',(-0.843338895500463,-5.21972261836337,
384.016169157125));
#42269=CARTESIAN_POINT('Ctrl Pts',(-3.23075696562154,-4.18556258278454,
383.937041281665));
#42270=CARTESIAN_POINT('Ctrl Pts',(-4.8359014200548,-2.1379387645183,383.857913406205));
#42271=CARTESIAN_POINT('Ctrl Pts',(-5.27011344929143,0.427351069865941,
383.778785530745));
#42272=CARTESIAN_POINT('Ctrl Pts',(-4.42825589269063,2.88916500985471,383.699657655286));
#42273=CARTESIAN_POINT('Ctrl Pts',(-2.51417043865664,4.65141609735177,383.620529779826));
#42274=CARTESIAN_POINT('Ctrl Pts',(0.00867922154690349,5.28740478651213,
383.541401904366));
#42275=CARTESIAN_POINT('Ctrl Pts',(2.52942735381344,4.6431370825228,383.462274028906));
#42276=CARTESIAN_POINT('Ctrl Pts',(4.43771707378134,2.87461160478899,383.383146153446));
#42277=CARTESIAN_POINT('Ctrl Pts',(5.27148802998996,0.410047137522666,383.304018277987));
#42278=CARTESIAN_POINT('Ctrl Pts',(4.82885656869832,-2.15380336712922,383.224890402527));
#42279=CARTESIAN_POINT('Ctrl Pts',(3.2169984748157,-4.19614650820864,383.145762527067));
#42280=CARTESIAN_POINT('Ctrl Pts',(0.82619815304806,-5.22246314656389,383.066634651607));
#42281=CARTESIAN_POINT('Ctrl Pts',(-1.76465219517988,-4.98424792073636,
382.987506776148));
#42282=CARTESIAN_POINT('Ctrl Pts',(-3.92822160960685,-3.5391806525149,382.908378900688));
#42283=CARTESIAN_POINT('Ctrl Pts',(-5.14063804209515,-1.23716014544694,
382.829251025228));
#42284=CARTESIAN_POINT('Ctrl Pts',(-5.10833518714595,1.36441794223199,382.750123149768));
#42285=CARTESIAN_POINT('Ctrl Pts',(-3.83913463932894,3.63562510806912,382.670995274309));
#42286=CARTESIAN_POINT('Ctrl Pts',(-1.64035202533435,5.0265266276326,382.591867398849));
#42287=CARTESIAN_POINT('Ctrl Pts',(0.955614320991023,5.2003390249901,382.512739523389));
#42288=CARTESIAN_POINT('Ctrl Pts',(3.32019468624774,4.11497654315675,382.433611647929));
#42289=CARTESIAN_POINT('Ctrl Pts',(4.8808455917412,2.03324150432223,382.354483772469));
#42290=CARTESIAN_POINT('Ctrl Pts',(5.25968159463003,-0.540808864968189,
382.27535589701));
#42291=CARTESIAN_POINT('Ctrl Pts',(4.36497391033337,-2.98391143759783,382.19622802155));
#42292=CARTESIAN_POINT('Ctrl Pts',(2.41336099931917,-4.70450989926509,382.11710014609));
#42293=CARTESIAN_POINT('Ctrl Pts',(-0.122606802820077,-5.28599018890692,
382.03797227063));
#42294=CARTESIAN_POINT('Ctrl Pts',(-2.6288874239146,-4.58755660648474,381.958844395171));
#42295=CARTESIAN_POINT('Ctrl Pts',(-4.49862704479611,-2.77832313044165,
381.879716519711));
#42296=CARTESIAN_POINT('Ctrl Pts',(-5.27909957396784,-0.296365304059962,
381.800588644251));
#42297=CARTESIAN_POINT('Ctrl Pts',(-4.78132667791946,2.25735241031028,381.721460768791));
#42298=CARTESIAN_POINT('Ctrl Pts',(-3.12583571520092,4.26449009693918,381.642332893332));
#42299=CARTESIAN_POINT('Ctrl Pts',(-0.713476057932961,5.23905302703404,
381.563205017871));
#42300=CARTESIAN_POINT('Ctrl Pts',(1.87163986094335,4.94506713162178,381.484077142412));
#42301=CARTESIAN_POINT('Ctrl Pts',(4.00356957706116,3.45371616479241,381.404949266952));
#42302=CARTESIAN_POINT('Ctrl Pts',(5.16610206459392,1.12610575148009,381.325821391492));
#42303=CARTESIAN_POINT('Ctrl Pts',(5.07774957870228,-1.47417228345499,381.246693516033));
#42304=CARTESIAN_POINT('Ctrl Pts',(3.75990519207135,-3.71750422352859,381.167565640573));
#42305=CARTESIAN_POINT('Ctrl Pts',(1.53166282114666,-5.06070486272762,381.088437765113));
#42306=CARTESIAN_POINT('Ctrl Pts',(-1.0674460141586,-5.17854069330105,381.009309889653));
#42307=CARTESIAN_POINT('Ctrl Pts',(-3.40809069944175,-4.04247974511891,
380.930182014193));
#42308=CARTESIAN_POINT('Ctrl Pts',(-4.92352337948473,-1.92760012372517,
380.851054138734));
#42309=CARTESIAN_POINT('Ctrl Pts',(-5.24680744637695,0.654015539541282,
380.771926263274));
#42310=CARTESIAN_POINT('Ctrl Pts',(-4.29966508516876,3.07727230850615,380.692798387814));
#42311=CARTESIAN_POINT('Ctrl Pts',(-2.31143093395199,4.75541919738815,380.613670512354));
#42312=CARTESIAN_POINT('Ctrl Pts',(0.236477452546483,5.28212108151216,380.534542636895));
#42313=CARTESIAN_POINT('Ctrl Pts',(2.7271267899117,4.52984593303835,380.455414761435));
#42314=CARTESIAN_POINT('Ctrl Pts',(4.55744811217567,2.68074456264382,380.376286885975));
#42315=CARTESIAN_POINT('Ctrl Pts',(5.28425980776137,0.182545855597361,380.297159010515));
#42316=CARTESIAN_POINT('Ctrl Pts',(4.73157661405697,-2.35985326887651,380.218031135055));
#42317=CARTESIAN_POINT('Ctrl Pts',(3.03322149728047,-4.33085350176541,380.138903259596));
#42318=CARTESIAN_POINT('Ctrl Pts',(0.600422665576261,-5.25321019263273,
380.059775384136));
#42319=CARTESIAN_POINT('Ctrl Pts',(-1.97775844481349,-4.90359013777528,
379.980647508676));
#42320=CARTESIAN_POINT('Ctrl Pts',(-4.07705851709219,-3.36664796994342,
379.901519633216));
#42321=CARTESIAN_POINT('Ctrl Pts',(-5.18916724645199,-1.01452845877678,
379.822391757756));
#42322=CARTESIAN_POINT('Ctrl Pts',(-5.04480615543027,1.58324210386498,379.743263882297));
#42323=CARTESIAN_POINT('Ctrl Pts',(-3.67892986111526,3.7976571438602,379.664136006837));
#42324=CARTESIAN_POINT('Ctrl Pts',(-1.42226240084736,5.09253319757995,379.585008131377));
#42325=CARTESIAN_POINT('Ctrl Pts',(1.17878204679748,5.15433774518764,379.505880255918));
#42326=CARTESIAN_POINT('Ctrl Pts',(3.49440419135096,3.9681058520139,379.426752380457));
#42327=CARTESIAN_POINT('Ctrl Pts',(4.96391496617568,1.82106367650753,379.347624504998));
#42328=CARTESIAN_POINT('Ctrl Pts',(5.2314969825461,-0.766918526917405,379.268496629538));
#42329=CARTESIAN_POINT('Ctrl Pts',(4.23235974285854,-3.16920427116154,379.189368754078));
#42330=CARTESIAN_POINT('Ctrl Pts',(2.20842757301423,-4.80412035237133,379.110240878619));
#42331=CARTESIAN_POINT('Ctrl Pts',(-0.350238295746339,-5.27579926091873,
379.031113003158));
#42332=CARTESIAN_POINT('Ctrl Pts',(-2.82409983509395,-4.47003185970082,
378.951985127699));
#42333=CARTESIAN_POINT('Ctrl Pts',(-4.61415296279982,-2.58192121126957,
378.872857252239));
#42334=CARTESIAN_POINT('Ctrl Pts',(-5.28696633525482,-0.0686416433394937,
378.793729376779));
#42335=CARTESIAN_POINT('Ctrl Pts',(-4.67962947817872,2.46125834732535,378.71460150132));
#42336=CARTESIAN_POINT('Ctrl Pts',(-2.9391988257698,4.39520590733944,378.63547362586));
#42337=CARTESIAN_POINT('Ctrl Pts',(-0.487090471470337,5.2649280695866,378.5563457504));
#42338=CARTESIAN_POINT('Ctrl Pts',(2.08295867142411,4.85983619872698,378.47721787494));
#42339=CARTESIAN_POINT('Ctrl Pts',(4.1486543056634,3.27801649742928,378.398089999481));
#42340=CARTESIAN_POINT('Ctrl Pts',(5.20982287752563,0.902480077413658,378.318962124021));
#42341=CARTESIAN_POINT('Ctrl Pts',(5.00952021436078,-1.69157675771122,378.239834248561));
#42342=CARTESIAN_POINT('Ctrl Pts',(3.59624624674644,-3.8760466506584,378.160706373101));
#42343=CARTESIAN_POINT('Ctrl Pts',(1.31220156369858,-5.12199685294173,378.081578497641));
#42344=CARTESIAN_POINT('Ctrl Pts',(-1.28957072085835,-5.12774141910675,
378.002450622182));
#42345=CARTESIAN_POINT('Ctrl Pts',(-3.57909508295452,-3.89188939879962,
377.923322746722));
#42346=CARTESIAN_POINT('Ctrl Pts',(-5.00200159628448,-1.71368163206748,
377.844194871262));
#42347=CARTESIAN_POINT('Ctrl Pts',(-5.21375731243622,0.879465401443313,
377.765066995802));
#42348=CARTESIAN_POINT('Ctrl Pts',(-4.16308913613231,3.25966463764834,377.685939120343));
#42349=CARTESIAN_POINT('Ctrl Pts',(-2.1043987453421,4.85059075019948,377.606811244883));
#42350=CARTESIAN_POINT('Ctrl Pts',(0.463836508427624,5.26702766261653,377.527683369423));
#42351=CARTESIAN_POINT('Ctrl Pts',(2.91976153075723,4.40814216068722,377.448555493963));
#42352=CARTESIAN_POINT('Ctrl Pts',(4.66871526619766,2.48189896419878,377.369427618503));
#42353=CARTESIAN_POINT('Ctrl Pts',(5.28721789969248,-0.0452944421492617,
377.290299743044));
#42354=CARTESIAN_POINT('Ctrl Pts',(4.62550939154664,-2.56152055897115,377.211171867584));
#42355=CARTESIAN_POINT('Ctrl Pts',(2.84381135938942,-4.45751743210561,377.132043992124));
#42356=CARTESIAN_POINT('Ctrl Pts',(0.373532100567371,-5.27420121678766,
377.052916116664));
#42357=CARTESIAN_POINT('Ctrl Pts',(-2.18719169184094,-4.81382563128935,
376.973788241204));
#42358=CARTESIAN_POINT('Ctrl Pts',(-4.21832369780876,-3.18786290260816,
376.894660365745));
#42359=CARTESIAN_POINT('Ctrl Pts',(-5.2280593665279,-0.790012636213206,
376.815532490285));
#42360=CARTESIAN_POINT('Ctrl Pts',(-4.97190814025518,1.79912594061044,376.736404614825));
#42361=CARTESIAN_POINT('Ctrl Pts',(-3.51189274247934,3.95263634434836,376.657276739365));
#42362=CARTESIAN_POINT('Ctrl Pts',(-1.20153141562281,5.1490821475793,376.578148863906));
#42363=CARTESIAN_POINT('Ctrl Pts',(1.39976059245402,5.09876406487689,376.499020988446));
#42364=CARTESIAN_POINT('Ctrl Pts',(3.66212404867255,3.81386577598244,376.419893112986));
#42365=CARTESIAN_POINT('Ctrl Pts',(5.03776558457334,1.60550385251465,376.340765237526));
#42366=CARTESIAN_POINT('Ctrl Pts',(5.19359667332446,-0.99160390296118,376.261637362067));
#42367=CARTESIAN_POINT('Ctrl Pts',(4.09188543028651,-3.34861140308599,376.182509486607));
#42368=CARTESIAN_POINT('Ctrl Pts',(1.99939275591558,-4.89480881330613,376.103381611147));
#42369=CARTESIAN_POINT('Ctrl Pts',(-0.577219342064538,-5.2558103583336,
376.024253735687));
#42370=CARTESIAN_POINT('Ctrl Pts',(-3.01406745721832,-4.34420557675964,
375.945125860227));
#42371=CARTESIAN_POINT('Ctrl Pts',(-4.72110968654987,-2.38072426020005,
375.865997984768));
#42372=CARTESIAN_POINT('Ctrl Pts',(-5.28501438473626,0.159209483211192,
375.786870109308));
#42373=CARTESIAN_POINT('Ctrl Pts',(-4.56924148341307,2.66059337382158,375.707742233848));
#42374=CARTESIAN_POINT('Ctrl Pts',(-2.74710339271414,4.51775908713646,375.628614358388));
#42375=CARTESIAN_POINT('Ctrl Pts',(-0.25980027835232,5.28102544478076,375.549486482929));
#42376=CARTESIAN_POINT('Ctrl Pts',(2.29040909674433,4.76557955369675,375.470358607468));
#42377=CARTESIAN_POINT('Ctrl Pts',(4.28603436317887,3.09622956904483,375.391230732009));
#42378=CARTESIAN_POINT('Ctrl Pts',(5.24386820297344,0.677177255244125,375.312102856549));
#42379=CARTESIAN_POINT('Ctrl Pts',(4.93198748823577,-1.90583737857549,375.232974981089));
#42380=CARTESIAN_POINT('Ctrl Pts',(3.42590832840442,-4.02739560248487,375.153847105629));
#42381=CARTESIAN_POINT('Ctrl Pts',(1.09030376033057,-5.1737660638094,375.07471923017));
#42382=CARTESIAN_POINT('Ctrl Pts',(-1.50930126232148,-5.06744133910014,
374.99559135471));
#42383=CARTESIAN_POINT('Ctrl Pts',(-3.74345011231245,-3.7340250124542,374.91646347925));
#42384=CARTESIAN_POINT('Ctrl Pts',(-5.07118953303831,-1.49668421879837,
374.83733560379));
#42385=CARTESIAN_POINT('Ctrl Pts',(-5.17098566641861,1.10346413672945,374.758207728331));
#42386=CARTESIAN_POINT('Ctrl Pts',(-4.40267566674078,2.65797789149901,374.705455811358));
#42387=CARTESIAN_POINT('Ctrl Pts',(-3.85627053850387,3.29705846079003,374.679079852871));
#42388=CARTESIAN_POINT('Ctrl Pts',(-1.2650852794265,-4.72177922709115,400.106973382376));
#42389=CARTESIAN_POINT('Ctrl Pts',(-2.04760230627562,-4.51212292510067,
400.08059742389));
#42390=CARTESIAN_POINT('Ctrl Pts',(-3.50558628380115,-3.69634492177698,
400.027845506916));
#42391=CARTESIAN_POINT('Ctrl Pts',(-4.84423972345866,-1.57661725067267,
399.948717631457));
#42392=CARTESIAN_POINT('Ctrl Pts',(-5.0096862523777,0.92455742070055,399.869589755997));
#42393=CARTESIAN_POINT('Ctrl Pts',(-3.9622375540088,3.20202818303723,399.790461880537));
#42394=CARTESIAN_POINT('Ctrl Pts',(-1.95534398901843,4.70410781476347,399.711334005077));
#42395=CARTESIAN_POINT('Ctrl Pts',(0.524977181208032,5.06720185162811,399.632206129618));
#42396=CARTESIAN_POINT('Ctrl Pts',(2.87819629981243,4.2033413524507,399.553078254158));
#42397=CARTESIAN_POINT('Ctrl Pts',(4.53450261129871,2.32172008778426,399.473950378698));
#42398=CARTESIAN_POINT('Ctrl Pts',(5.09285792630992,-0.122070466194823,
399.394822503238));
#42399=CARTESIAN_POINT('Ctrl Pts',(4.41806180230403,-2.5363019515078,399.315694627778));
#42400=CARTESIAN_POINT('Ctrl Pts',(2.67350672576957,-4.3364112842173,399.236566752319));
#42401=CARTESIAN_POINT('Ctrl Pts',(0.281606541856066,-5.08653095966945,
399.157438876859));
#42402=CARTESIAN_POINT('Ctrl Pts',(-2.17847980551824,-4.60503265524259,
399.078311001399));
#42403=CARTESIAN_POINT('Ctrl Pts',(-4.1110838687323,-3.00850283765647,398.999183125939));
#42404=CARTESIAN_POINT('Ctrl Pts',(-5.04825788999868,-0.683514555327269,
398.920055250479));
#42405=CARTESIAN_POINT('Ctrl Pts',(-4.76308094287924,1.80697533276996,398.84092737502));
#42406=CARTESIAN_POINT('Ctrl Pts',(-3.32460382095413,3.85993643987858,398.76179949956));
#42407=CARTESIAN_POINT('Ctrl Pts',(-1.08112964449127,4.97827867803806,398.6826716241));
#42408=CARTESIAN_POINT('Ctrl Pts',(1.4241219451236,4.89121422375072,398.603543748641));
#42409=CARTESIAN_POINT('Ctrl Pts',(3.58454628917626,3.6198242774857,398.52441587318));
#42410=CARTESIAN_POINT('Ctrl Pts',(4.87703286664207,1.4719545906142,398.445287997721));
#42411=CARTESIAN_POINT('Ctrl Pts',(4.98862772878014,-1.03232421377308,398.366160122261));
#42412=CARTESIAN_POINT('Ctrl Pts',(3.89231005153748,-3.28664302317114,398.287032246801));
#42413=CARTESIAN_POINT('Ctrl Pts',(1.853534773828,-4.7451563452711,398.207904371342));
#42414=CARTESIAN_POINT('Ctrl Pts',(-0.634042863421179,-5.05470964015625,
398.128776495882));
#42415=CARTESIAN_POINT('Ctrl Pts',(-2.96809765493441,-4.14034976900372,
398.049648620422));
#42416=CARTESIAN_POINT('Ctrl Pts',(-4.58347737773795,-2.22347363975469,
397.970520744962));
#42417=CARTESIAN_POINT('Ctrl Pts',(-5.08904492375008,0.231779341134317,
397.891392869503));
#42418=CARTESIAN_POINT('Ctrl Pts',(-4.36238559065476,2.6309108417746,397.812264994043));
#42419=CARTESIAN_POINT('Ctrl Pts',(-2.57944774904339,4.39301140550268,397.733137118583));
#42420=CARTESIAN_POINT('Ctrl Pts',(-0.171939895328258,5.09141793327901,
397.654009243123));
#42421=CARTESIAN_POINT('Ctrl Pts',(2.27720032040928,4.55702299748958,397.574881367663));
#42422=CARTESIAN_POINT('Ctrl Pts',(4.17495466984747,2.91922136941339,397.495753492203));
#42423=CARTESIAN_POINT('Ctrl Pts',(5.06181376480896,0.574579245458329,397.416625616744));
#42424=CARTESIAN_POINT('Ctrl Pts',(4.72303954910339,-1.90918760642483,397.337497741284));
#42425=CARTESIAN_POINT('Ctrl Pts',(3.24066051742776,-3.93067669870034,397.258369865824));
#42426=CARTESIAN_POINT('Ctrl Pts',(0.973609891088484,-5.00041835038785,
397.179241990364));
#42427=CARTESIAN_POINT('Ctrl Pts',(-1.52918404181197,-4.85939256133815,
397.100114114905));
#42428=CARTESIAN_POINT('Ctrl Pts',(-3.66171170517574,-3.54174636120374,
397.020986239445));
#42429=CARTESIAN_POINT('Ctrl Pts',(-4.90761729027895,-1.36652567889375,
396.941858363985));
#42430=CARTESIAN_POINT('Ctrl Pts',(-4.965225654969,1.13957627834147,396.862730488525));
#42431=CARTESIAN_POINT('Ctrl Pts',(-3.82058789989522,3.3697489517908,396.783602613066));
#42432=CARTESIAN_POINT('Ctrl Pts',(-1.7508588605474,4.78399343115808,396.704474737606));
#42433=CARTESIAN_POINT('Ctrl Pts',(0.742811287950349,5.03987413428296,396.625346862146));
#42434=CARTESIAN_POINT('Ctrl Pts',(3.05662214087683,4.07543384031964,396.546218986686));
#42435=CARTESIAN_POINT('Ctrl Pts',(4.63032320548468,2.12419559167018,396.467091111227));
#42436=CARTESIAN_POINT('Ctrl Pts',(5.08286916176923,-0.341380994281065,
396.387963235767));
#42437=CARTESIAN_POINT('Ctrl Pts',(4.30468359613617,-2.72429789782194,396.308835360307));
#42438=CARTESIAN_POINT('Ctrl Pts',(2.48419109223004,-4.44757175503734,396.229707484847));
#42439=CARTESIAN_POINT('Ctrl Pts',(0.0621933781031742,-5.09394070270169,
396.150579609387));
#42440=CARTESIAN_POINT('Ctrl Pts',(-2.37486341947636,-4.50689734049423,
396.071451733928));
#42441=CARTESIAN_POINT('Ctrl Pts',(-4.23688686924074,-2.82858437317615,
395.992323858468));
#42442=CARTESIAN_POINT('Ctrl Pts',(-5.07301922112011,-0.46537713853058,
395.913195983008));
#42443=CARTESIAN_POINT('Ctrl Pts',(-4.68080504901513,2.01051336529637,395.834068107548));
#42444=CARTESIAN_POINT('Ctrl Pts',(-3.15521243681498,3.99959177635531,395.754940232089));
#42445=CARTESIAN_POINT('Ctrl Pts',(-0.865638049608238,5.0202361165578,395.675812356629));
#42446=CARTESIAN_POINT('Ctrl Pts',(1.63353607355812,4.82531447631191,395.596684481169));
#42447=CARTESIAN_POINT('Ctrl Pts',(3.73717683280492,3.46202386174144,395.517556605709));
#42448=CARTESIAN_POINT('Ctrl Pts',(4.93592289877338,1.26046223120153,395.43842873025));
#42449=CARTESIAN_POINT('Ctrl Pts',(4.93951801594962,-1.24629918921186,395.35930085479));
#42450=CARTESIAN_POINT('Ctrl Pts',(3.74709168700367,-3.45129016283895,395.28017297933));
#42451=CARTESIAN_POINT('Ctrl Pts',(1.64736994911874,-4.82060910566927,395.20104510387));
#42452=CARTESIAN_POINT('Ctrl Pts',(-0.851234793642623,-5.0226984007616,
395.12191722841));
#42453=CARTESIAN_POINT('Ctrl Pts',(-3.14372730731715,-4.00862551458096,
395.04278935295));
#42454=CARTESIAN_POINT('Ctrl Pts',(-4.67501897747406,-2.02393118933878,
394.963661477491));
#42455=CARTESIAN_POINT('Ctrl Pts',(-5.07433320772034,0.450824129730827,
394.884533602031));
#42456=CARTESIAN_POINT('Ctrl Pts',(-4.24498275416411,2.81641994662909,394.805405726571));
#42457=CARTESIAN_POINT('Ctrl Pts',(-2.38778091996604,4.50006690807671,394.726277851111));
#42458=CARTESIAN_POINT('Ctrl Pts',(0.0475820181493076,5.09409813906934,
394.647149975652));
#42459=CARTESIAN_POINT('Ctrl Pts',(2.47142376857538,4.45467893961412,394.568022100192));
#42460=CARTESIAN_POINT('Ctrl Pts',(4.29685170208089,2.73663394505832,394.488894224732));
#42461=CARTESIAN_POINT('Ctrl Pts',(5.08186905910887,0.355958937228547,394.409766349272));
#42462=CARTESIAN_POINT('Ctrl Pts',(4.63639705230557,-2.11090555740732,394.330638473812));
#42463=CARTESIAN_POINT('Ctrl Pts',(3.06829925703676,-4.06664967364888,394.251510598353));
#42464=CARTESIAN_POINT('Ctrl Pts',(0.757264255609957,-5.037722773843,394.172382722893));
#42465=CARTESIAN_POINT('Ctrl Pts',(-1.73712958511388,-4.78899579279863,
394.093254847433));
#42466=CARTESIAN_POINT('Ctrl Pts',(-3.81090663047816,-3.38069379753602,
394.014126971973));
#42467=CARTESIAN_POINT('Ctrl Pts',(-4.96193654859164,-1.15381349735189,
393.934999096513));
#42468=CARTESIAN_POINT('Ctrl Pts',(-4.91151674888844,1.35244339042685,393.855871221054));
#42469=CARTESIAN_POINT('Ctrl Pts',(-3.67185554026823,3.53122879325631,393.776743345594));
#42470=CARTESIAN_POINT('Ctrl Pts',(-1.54311609384367,4.85498636659688,393.697615470134));
#42471=CARTESIAN_POINT('Ctrl Pts',(0.959263034860399,5.00319041501234,393.618487594674));
#42472=CARTESIAN_POINT('Ctrl Pts',(3.22937270762551,3.93995581373248,393.539359719215));
#42473=CARTESIAN_POINT('Ctrl Pts',(4.71754393956094,1.92272698978111,393.460231843755));
#42474=CARTESIAN_POINT('Ctrl Pts',(5.06344102520928,-0.560057928386485,
393.381103968295));
#42475=CARTESIAN_POINT('Ctrl Pts',(4.18331078637565,-2.90723421201562,393.301976092835));
#42476=CARTESIAN_POINT('Ctrl Pts',(2.29026199958981,-4.55047248889121,393.222848217376));
#42477=CARTESIAN_POINT('Ctrl Pts',(-0.157335320049481,-5.0918901692776,
393.143720341916));
#42478=CARTESIAN_POINT('Ctrl Pts',(-2.5668365306344,-4.40039204207098,393.064592466456));
#42479=CARTESIAN_POINT('Ctrl Pts',(-4.35482132414875,-2.6434127815497,392.985464590996));
#42480=CARTESIAN_POINT('Ctrl Pts',(-5.08835916941954,-0.24637544907113,
392.906336715536));
#42481=CARTESIAN_POINT('Ctrl Pts',(-4.58983617949401,2.21031756639828,392.827208840077));
#42482=CARTESIAN_POINT('Ctrl Pts',(-2.97996133557448,4.13181925275079,392.748080964617));
#42483=CARTESIAN_POINT('Ctrl Pts',(-0.648538831649752,5.05287020244567,
392.668953089157));
#42484=CARTESIAN_POINT('Ctrl Pts',(1.83991647361136,4.75045337510584,392.589825213697));
#42485=CARTESIAN_POINT('Ctrl Pts',(3.88286686231846,3.29779393359108,392.510697338238));
#42486=CARTESIAN_POINT('Ctrl Pts',(4.98564616049109,1.04662899888231,392.431569462778));
#42487=CARTESIAN_POINT('Ctrl Pts',(4.88123485596325,-1.45795959472489,392.352441587318));
#42488=CARTESIAN_POINT('Ctrl Pts',(3.59491439502781,-3.60952772414103,392.273313711858));
#42489=CARTESIAN_POINT('Ctrl Pts',(1.43814570421584,-4.88710925111834,392.194185836399));
#42490=CARTESIAN_POINT('Ctrl Pts',(-1.06684584950233,-4.98135923542166,
392.115057960939));
#42491=CARTESIAN_POINT('Ctrl Pts',(-3.31351857300444,-3.86945662403335,
392.035930085479));
#42492=CARTESIAN_POINT('Ctrl Pts',(-4.75787834559899,-1.82062998640609,
391.956802210019));
#42493=CARTESIAN_POINT('Ctrl Pts',(-5.05019767193907,0.669031668355122,
391.877674334559));
#42494=CARTESIAN_POINT('Ctrl Pts',(-4.11969632968522,2.99669852506039,391.7985464591));
#42495=CARTESIAN_POINT('Ctrl Pts',(-2.19167961327856,4.59876509202852,391.71941858364));
#42496=CARTESIAN_POINT('Ctrl Pts',(0.267015564477117,5.08731781858062,391.64029070818));
#42497=CARTESIAN_POINT('Ctrl Pts',(2.66105740145502,4.34406185557737,391.56116283272));
#42498=CARTESIAN_POINT('Ctrl Pts',(4.4107688176863,2.54896416919641,391.48203495726));
#42499=CARTESIAN_POINT('Ctrl Pts',(5.09248653841822,0.136677558326831,391.402907081801));
#42500=CARTESIAN_POINT('Ctrl Pts',(4.54114405077152,-2.30870323105058,391.323779206341));
#42501=CARTESIAN_POINT('Ctrl Pts',(2.89023969147757,-4.1950702526571,391.244651330881));
#42502=CARTESIAN_POINT('Ctrl Pts',(0.539512263560586,-5.06567136877124,
391.165523455421));
#42503=CARTESIAN_POINT('Ctrl Pts',(-1.94184901073189,-4.70970512011533,
391.086395579962));
#42504=CARTESIAN_POINT('Ctrl Pts',(-3.95302411413336,-3.21336276383497,
391.007267704502));
#42505=CARTESIAN_POINT('Ctrl Pts',(-5.00704072509175,-0.93895850610853,
390.928139829042));
#42506=CARTESIAN_POINT('Ctrl Pts',(-4.84868639834328,1.56279880645007,390.849011953582));
#42507=CARTESIAN_POINT('Ctrl Pts',(-3.51630397832454,3.68615059797345,390.769884078122));
#42508=CARTESIAN_POINT('Ctrl Pts',(-1.33250752244617,4.91696284321382,390.690756202663));
#42509=CARTESIAN_POINT('Ctrl Pts',(1.17393328229752,4.95721499913359,390.611628327203));
#42510=CARTESIAN_POINT('Ctrl Pts',(3.39612583095411,3.79716068125213,390.532500451743));
#42511=CARTESIAN_POINT('Ctrl Pts',(4.79600346661011,1.71768758718946,390.453372576283));
#42512=CARTESIAN_POINT('Ctrl Pts',(5.03460929736123,-0.777694748500222,
390.374244700824));
#42513=CARTESIAN_POINT('Ctrl Pts',(4.05416892298729,-3.08477134368254,390.295116825364));
#42514=CARTESIAN_POINT('Ctrl Pts',(2.09207953702197,-4.64492229318153,390.215988949904));
#42515=CARTESIAN_POINT('Ctrl Pts',(-0.376571822235509,-5.08038321011508,
390.136861074444));
#42516=CARTESIAN_POINT('Ctrl Pts',(-2.75404263028444,-4.28571453663178,
390.057733198984));
#42517=CARTESIAN_POINT('Ctrl Pts',(-4.46466820389571,-2.45333196450126,
389.978605323525));
#42518=CARTESIAN_POINT('Ctrl Pts',(-5.09424924959213,-0.0269162023862396,
389.899477448065));
#42519=CARTESIAN_POINT('Ctrl Pts',(-4.49034327596192,2.40601686672071,389.820349572605));
#42520=CARTESIAN_POINT('Ctrl Pts',(-2.79917598631673,4.25637330324171,389.741221697145));
#42521=CARTESIAN_POINT('Ctrl Pts',(-0.430235177009337,5.07612032869441,
389.662093821686));
#42522=CARTESIAN_POINT('Ctrl Pts',(2.04287986486846,4.66676994897283,389.582965946226));
#42523=CARTESIAN_POINT('Ctrl Pts',(4.02134580893056,3.12743949324644,389.503838070766));
#42524=CARTESIAN_POINT('Ctrl Pts',(5.02611030798847,0.830852015014124,389.424710195306));
#42525=CARTESIAN_POINT('Ctrl Pts',(4.81388648966003,-1.66691234430295,389.345582319847));
#42526=CARTESIAN_POINT('Ctrl Pts',(3.43606079231419,-3.76106183549833,389.266454444386));
#42527=CARTESIAN_POINT('Ctrl Pts',(1.22625060082997,-4.94453328059232,389.187326568927));
#42528=CARTESIAN_POINT('Ctrl Pts',(-1.28047560800195,-4.93076891734271,
389.108198693467));
#42529=CARTESIAN_POINT('Ctrl Pts',(-3.4771561234157,-3.72310155546604,389.029070818007));
#42530=CARTESIAN_POINT('Ctrl Pts',(-4.8319015994811,-1.61394759265993,388.949942942547));
#42531=CARTESIAN_POINT('Ctrl Pts',(-5.01668313982022,0.88599671193773,388.870815067088));
#42532=CARTESIAN_POINT('Ctrl Pts',(-3.98675899344041,3.17141177193107,388.791687191628));
#42533=CARTESIAN_POINT('Ctrl Pts',(-1.99150801936634,4.68892265960108,388.712559316169));
#42534=CARTESIAN_POINT('Ctrl Pts',(0.485953221700427,5.07108956391423,388.633431440708));
#42535=CARTESIAN_POINT('Ctrl Pts',(2.84574904013097,4.2253771783729,388.554303565249));
#42536=CARTESIAN_POINT('Ctrl Pts',(4.51649445500228,2.35656057355938,388.475175689789));
#42537=CARTESIAN_POINT('Ctrl Pts',(5.09364648443963,-0.0828576518904476,
388.396047814329));
#42538=CARTESIAN_POINT('Ctrl Pts',(4.43745744402291,-2.50221328655385,388.316919938869));
#42539=CARTESIAN_POINT('Ctrl Pts',(2.70681250483858,-4.31569993889408,388.23779206341));
#42540=CARTESIAN_POINT('Ctrl Pts',(0.320758313989414,-5.08421223031922,
388.15866418795));
#42541=CARTESIAN_POINT('Ctrl Pts',(-2.14296212310374,-4.62166779830222,
388.07953631249));
#42542=CARTESIAN_POINT('Ctrl Pts',(-4.08780022204497,-3.04006401964993,
388.00040843703));
#42543=CARTESIAN_POINT('Ctrl Pts',(-5.04284605436382,-0.722359724035205,
387.921280561571));
#42544=CARTESIAN_POINT('Ctrl Pts',(-4.7768512889894,1.77025186394512,387.842152686111));
#42545=CARTESIAN_POINT('Ctrl Pts',(-3.35422209731677,3.83422665224591,387.763024810651));
#42546=CARTESIAN_POINT('Ctrl Pts',(-1.11942427896961,4.96980776112863,387.683896935191));
#42547=CARTESIAN_POINT('Ctrl Pts',(1.38642335448793,4.90203327008818,387.604769059731));
#42548=CARTESIAN_POINT('Ctrl Pts',(3.55657182458215,3.64731363547327,387.525641184271));
#42549=CARTESIAN_POINT('Ctrl Pts',(4.86555607518393,1.50945817370396,387.446513308812));
#42550=CARTESIAN_POINT('Ctrl Pts',(4.99642752319251,-0.993887269465375,
387.367385433352));
#42551=CARTESIAN_POINT('Ctrl Pts',(3.9174978423384,-3.25657957897469,387.288257557892));
#42552=CARTESIAN_POINT('Ctrl Pts',(1.89001175993966,-4.73074576004784,387.209129682432));
#42553=CARTESIAN_POINT('Ctrl Pts',(-0.595108972441489,-5.05944119541285,
387.130001806973));
#42554=CARTESIAN_POINT('Ctrl Pts',(-2.93613404781291,-4.1630777979993,387.050873931513));
#42555=CARTESIAN_POINT('Ctrl Pts',(-4.5662235058762,-2.2586949314382,386.971746056053));
#42556=CARTESIAN_POINT('Ctrl Pts',(-5.09067852285014,0.192593031839733,
386.892618180593));
#42557=CARTESIAN_POINT('Ctrl Pts',(-4.38251111209279,2.59724782246595,386.813490305134));
#42558=CARTESIAN_POINT('Ctrl Pts',(-2.61319213533106,4.37302261173721,386.734362429674));
#42559=CARTESIAN_POINT('Ctrl Pts',(-0.211132509258637,5.08994331623203,
386.655234554214));
#42560=CARTESIAN_POINT('Ctrl Pts',(2.24204931299394,4.57441961094785,386.576106678754));
#42561=CARTESIAN_POINT('Ctrl Pts',(4.15235649586965,2.95127691518944,386.496978803295));
#42562=CARTESIAN_POINT('Ctrl Pts',(5.05724019309986,0.613532010751077,386.417850927834));
#42563=CARTESIAN_POINT('Ctrl Pts',(4.73759799334825,-1.872769380448,386.338723052375));
#42564=CARTESIAN_POINT('Ctrl Pts',(3.27082589451466,-3.90561107468386,386.259595176915));
#42565=CARTESIAN_POINT('Ctrl Pts',(1.01207816086419,-4.99277454880777,386.180467301455));
#42566=CARTESIAN_POINT('Ctrl Pts',(-1.49172732571618,-4.87102140055169,
386.101339425996));
#42567=CARTESIAN_POINT('Ctrl Pts',(-3.63433605836998,-3.56983211282445,
386.022211550536));
#42568=CARTESIAN_POINT('Ctrl Pts',(-4.89695126651592,-1.40426784919727,
385.943083675076));
#42569=CARTESIAN_POINT('Ctrl Pts',(-4.97385185302132,1.10131632291422,385.863955799616));
#42570=CARTESIAN_POINT('Ctrl Pts',(-3.84641763057586,3.34023521778273,385.784827924157));
#42571=CARTESIAN_POINT('Ctrl Pts',(-1.78763788776658,4.77037217427974,385.705700048697));
#42572=CARTESIAN_POINT('Ctrl Pts',(0.703988388806892,5.0454435134432,385.626572173237));
#42573=CARTESIAN_POINT('Ctrl Pts',(3.02515568373168,4.09884532375971,385.547444297777));
#42574=CARTESIAN_POINT('Ctrl Pts',(4.61383226520657,2.15978048131279,385.468316422317));
#42575=CARTESIAN_POINT('Ctrl Pts',(5.08534674297434,-0.302238982663029,
385.389188546858));
#42576=CARTESIAN_POINT('Ctrl Pts',(4.32552979408761,-2.69107634588493,385.310060671397));
#42577=CARTESIAN_POINT('Ctrl Pts',(2.51835834970871,-4.42831470441898,385.230932795938));
#42578=CARTESIAN_POINT('Ctrl Pts',(0.10140866673516,-5.09331092524616,385.151804920478));
#42579=CARTESIAN_POINT('Ctrl Pts',(-2.34009542414748,-4.5250473262503,385.072677045019));
#42580=CARTESIAN_POINT('Ctrl Pts',(-4.21498465418432,-2.86111940748926,
384.993549169558));
#42581=CARTESIAN_POINT('Ctrl Pts',(-5.06928604038651,-0.504419408492031,
384.914421294099));
#42582=CARTESIAN_POINT('Ctrl Pts',(-4.69614482970923,1.97441729057362,384.835293418639));
#42583=CARTESIAN_POINT('Ctrl Pts',(-3.18591090830761,3.97518195599239,384.756165543179));
#42584=CARTESIAN_POINT('Ctrl Pts',(-0.904262091876385,5.01342297917464,
384.677037667719));
#42585=CARTESIAN_POINT('Ctrl Pts',(1.59633862457976,4.83774770886161,384.59790979226));
#42586=CARTESIAN_POINT('Ctrl Pts',(3.71041271554213,3.4906929654818,384.5187819168));
#42587=CARTESIAN_POINT('Ctrl Pts',(4.92607259535609,1.29842546347592,384.43965404134));
#42588=CARTESIAN_POINT('Ctrl Pts',(4.94896661214932,-1.20823398841131,384.360526165881));
#42589=CARTESIAN_POINT('Ctrl Pts',(3.77355136371449,-3.42233984348858,384.281398290421));
#42590=CARTESIAN_POINT('Ctrl Pts',(1.6844339393846,-4.80778350206934,384.202270414961));
#42591=CARTESIAN_POINT('Ctrl Pts',(-0.812540913458525,-5.02910301772363,
384.123142539501));
#42592=CARTESIAN_POINT('Ctrl Pts',(-3.11277261136022,-4.03270958152043,
384.044014664041));
#42593=CARTESIAN_POINT('Ctrl Pts',(-4.65929862622416,-2.05986315336399,
383.964886788582));
#42594=CARTESIAN_POINT('Ctrl Pts',(-5.07765362058409,0.411744591087888,
383.885758913121));
#42595=CARTESIAN_POINT('Ctrl Pts',(-4.26653994885377,2.78365528824167,383.806631037662));
#42596=CARTESIAN_POINT('Ctrl Pts',(-2.42235518332661,4.48155054247207,383.727503162202));
#42597=CARTESIAN_POINT('Ctrl Pts',(0.00836226414014005,5.09431349363773,
383.648375286742));
#42598=CARTESIAN_POINT('Ctrl Pts',(2.43705492959019,4.47357386985853,383.569247411283));
#42599=CARTESIAN_POINT('Ctrl Pts',(4.27565561607469,2.76963336050998,383.490119535823));
#42600=CARTESIAN_POINT('Ctrl Pts',(5.07897800282517,0.39507258287429,383.410991660363));
#42601=CARTESIAN_POINT('Ctrl Pts',(4.65251104653713,-2.07514839487948,383.331863784903));
#42602=CARTESIAN_POINT('Ctrl Pts',(3.09951656833074,-4.04290699145606,383.252735909444));
#42603=CARTESIAN_POINT('Ctrl Pts',(0.79602613558697,-5.03174346428585,383.173608033984));
#42604=CARTESIAN_POINT('Ctrl Pts',(-1.70020867560859,-4.80222764540647,
383.094480158524));
#42605=CARTESIAN_POINT('Ctrl Pts',(-3.78476647047488,-3.40993294111337,
383.015352283064));
#42606=CARTESIAN_POINT('Ctrl Pts',(-4.9529065394344,-1.1919801636558,382.936224407604));
#42607=CARTESIAN_POINT('Ctrl Pts',(-4.92178335585094,1.31459061954267,382.857096532145));
#42608=CARTESIAN_POINT('Ctrl Pts',(-3.6989328766574,3.50285533142662,382.777968656685));
#42609=CARTESIAN_POINT('Ctrl Pts',(-1.58044783677119,4.84296237174792,382.698840781225));
#42610=CARTESIAN_POINT('Ctrl Pts',(0.920716140847871,5.01042729584046,382.619712905765));
#42611=CARTESIAN_POINT('Ctrl Pts',(3.19894414643704,3.96470128091602,382.540585030306));
#42612=CARTESIAN_POINT('Ctrl Pts',(4.70260147696606,1.95898934345174,382.461457154846));
#42613=CARTESIAN_POINT('Ctrl Pts',(5.06760272792295,-0.521059009008414,
382.382329279386));
#42614=CARTESIAN_POINT('Ctrl Pts',(4.20556896788232,-2.87494166120048,382.303201403926));
#42615=CARTESIAN_POINT('Ctrl Pts',(2.32522721453312,-4.53270540623539,382.224073528466));
#42616=CARTESIAN_POINT('Ctrl Pts',(-0.118129312060885,-5.0929505558716,
382.144945653006));
#42617=CARTESIAN_POINT('Ctrl Pts',(-2.53288280690479,-4.42002314308501,
382.065817777547));
#42618=CARTESIAN_POINT('Ctrl Pts',(-4.33434120943595,-2.67686125510947,
381.986689902087));
#42619=CARTESIAN_POINT('Ctrl Pts',(-5.08631158002599,-0.285542308273818,
381.907562026627));
#42620=CARTESIAN_POINT('Ctrl Pts',(-4.60671690485093,2.17491591963496,381.828434151168));
#42621=CARTESIAN_POINT('Ctrl Pts',(-3.01168299114604,4.10875473346396,381.749306275708));
#42622=CARTESIAN_POINT('Ctrl Pts',(-0.687420550548197,5.04772749716196,
381.670178400248));
#42623=CARTESIAN_POINT('Ctrl Pts',(1.80328924752583,4.76447770366057,381.591050524788));
#42624=CARTESIAN_POINT('Ctrl Pts',(3.85736279756143,3.32758954002893,381.511922649328));
#42625=CARTESIAN_POINT('Ctrl Pts',(4.97744063861076,1.0849813768112,381.432794773869));
#42626=CARTESIAN_POINT('Ctrl Pts',(4.89231470646681,-1.42033683040663,381.353666898409));
#42627=CARTESIAN_POINT('Ctrl Pts',(3.62259681793774,-3.58174429483572,381.274539022949));
#42628=CARTESIAN_POINT('Ctrl Pts',(1.47572786509085,-4.87589244827193,381.195411147489));
#42629=CARTESIAN_POINT('Ctrl Pts',(-1.02846384062172,-4.98942501972467,
381.11628327203));
#42630=CARTESIAN_POINT('Ctrl Pts',(-3.28363027585792,-3.89485200108939,
381.03715539657));
#42631=CARTESIAN_POINT('Ctrl Pts',(-4.74372071007927,-1.85720589157097,
380.95802752111));
#42632=CARTESIAN_POINT('Ctrl Pts',(-5.05519873204731,0.630131477096863,
380.87889964565));
#42633=CARTESIAN_POINT('Ctrl Pts',(-4.14264516258972,2.96489307662063,380.79977177019));
#42634=CARTESIAN_POINT('Ctrl Pts',(-2.22701954397005,4.58175554233269,380.720643894731));
#42635=CARTESIAN_POINT('Ctrl Pts',(0.227841507524015,5.08922274481773,380.641516019271));
#42636=CARTESIAN_POINT('Ctrl Pts',(2.6275345591372,4.36442001180692,380.562388143811));
#42637=CARTESIAN_POINT('Ctrl Pts',(4.39101418405409,2.58284616931722,380.483260268351));
#42638=CARTESIAN_POINT('Ctrl Pts',(5.09128336669755,0.175879444250141,380.404132392892));
#42639=CARTESIAN_POINT('Ctrl Pts',(4.55878366881602,-2.27367353854006,380.325004517432));
#42640=CARTESIAN_POINT('Ctrl Pts',(2.92245096161458,-4.17269460611234,380.245876641972));
#42641=CARTESIAN_POINT('Ctrl Pts',(0.578495766946718,-5.0613676557375,380.166748766512));
#42642=CARTESIAN_POINT('Ctrl Pts',(-1.90553247564304,-4.72451541252546,
380.087620891052));
#42643=CARTESIAN_POINT('Ctrl Pts',(-3.92816798724318,-3.24370099776764,
380.008493015593));
#42644=CARTESIAN_POINT('Ctrl Pts',(-4.99966350066068,-0.977478787024238,
379.929365140133));
#42645=CARTESIAN_POINT('Ctrl Pts',(-4.86057434754265,1.52542351854533,379.850237264673));
#42646=CARTESIAN_POINT('Ctrl Pts',(-3.54457863363044,3.65897010221885,379.771109389213));
#42647=CARTESIAN_POINT('Ctrl Pts',(-1.37032265027505,4.90655844080798,379.691981513754));
#42648=CARTESIAN_POINT('Ctrl Pts',(1.13573398094598,4.96610594162524,379.612853638294));
#42649=CARTESIAN_POINT('Ctrl Pts',(3.36679167625567,3.82319417602828,379.533725762834));
#42650=CARTESIAN_POINT('Ctrl Pts',(4.78263723215717,1.75456006010191,379.454597887374));
#42651=CARTESIAN_POINT('Ctrl Pts',(5.04044739265935,-0.738911348373108,
379.375470011914));
#42652=CARTESIAN_POINT('Ctrl Pts',(4.07779775117163,-3.05346776623899,379.296342136454));
#42653=CARTESIAN_POINT('Ctrl Pts',(2.1277777736305,-4.62867817470224,379.217214260995));
#42654=CARTESIAN_POINT('Ctrl Pts',(-0.337447906496721,-5.0831317914571,
379.138086385535));
#42655=CARTESIAN_POINT('Ctrl Pts',(-2.72096623545812,-4.30679029492008,
379.058958510076));
#42656=CARTESIAN_POINT('Ctrl Pts',(-4.44564822425965,-2.48763175833121,
378.979830634615));
#42657=CARTESIAN_POINT('Ctrl Pts',(-5.09389105422811,-0.0661349119291711,
378.900702759156));
#42658=CARTESIAN_POINT('Ctrl Pts',(-4.50873359586993,2.37137539423742,378.821574883696));
#42659=CARTESIAN_POINT('Ctrl Pts',(-2.83186191395806,4.23469691940223,378.742447008236));
#42660=CARTESIAN_POINT('Ctrl Pts',(-0.469302363186489,5.07265760630743,
378.663319132776));
#42661=CARTESIAN_POINT('Ctrl Pts',(2.00689088408632,4.68235932819045,378.584191257317));
#42662=CARTESIAN_POINT('Ctrl Pts',(3.99714916166288,3.15830626734308,378.505063381856));
#42663=CARTESIAN_POINT('Ctrl Pts',(5.01956480656533,0.869522312313901,378.425935506397));
#42664=CARTESIAN_POINT('Ctrl Pts',(4.82657701747544,-1.62980188774553,378.346807630937));
#42665=CARTESIAN_POINT('Ctrl Pts',(3.46491455089248,-3.73449689435332,378.267679755478));
#42666=CARTESIAN_POINT('Ctrl Pts',(1.26428113644233,-4.93494610983311,378.188551880018));
#42667=CARTESIAN_POINT('Ctrl Pts',(-1.24247675173787,-4.94048088958068,
378.109424004558));
#42668=CARTESIAN_POINT('Ctrl Pts',(-3.4483897322594,-3.74976107950479,378.030296129098));
#42669=CARTESIAN_POINT('Ctrl Pts',(-4.81933297260539,-1.65109951186456,
377.951168253638));
#42670=CARTESIAN_POINT('Ctrl Pts',(-5.02335555943258,0.847348111721862,
377.872040378178));
#42671=CARTESIAN_POINT('Ctrl Pts',(-4.01105684503597,3.1406246010644,377.792912502719));
#42672=CARTESIAN_POINT('Ctrl Pts',(-2.02754798568437,4.67345151517251,377.713784627259));
#42673=CARTESIAN_POINT('Ctrl Pts',(0.44689761407191,5.07468052407812,377.634656751799));
#42674=CARTESIAN_POINT('Ctrl Pts',(2.81313445157142,4.24716075235008,377.555528876339));
#42675=CARTESIAN_POINT('Ctrl Pts',(4.49821796114695,2.39126223424701,377.47640100088));
#42676=CARTESIAN_POINT('Ctrl Pts',(5.09413343175754,-0.043640329640808,
377.39727312542));
#42677=CARTESIAN_POINT('Ctrl Pts',(4.4565899263877,-2.46797611960502,377.31814524996));
#42678=CARTESIAN_POINT('Ctrl Pts',(2.73995791251956,-4.29473288302567,377.2390173745));
#42679=CARTESIAN_POINT('Ctrl Pts',(0.35989104240352,-5.08159210646814,377.159889499041));
#42680=CARTESIAN_POINT('Ctrl Pts',(-2.10731740784078,-4.63802902551619,
377.080761623581));
#42681=CARTESIAN_POINT('Ctrl Pts',(-4.06427428993092,-3.07144500115654,
377.001633748121));
#42682=CARTESIAN_POINT('Ctrl Pts',(-5.03713531530297,-0.761162081456616,
376.922505872661));
#42683=CARTESIAN_POINT('Ctrl Pts',(-4.79033850266972,1.73342347069504,376.843377997201));
#42684=CARTESIAN_POINT('Ctrl Pts',(-3.38364156114149,3.8082896009442,376.764250121742));
#42685=CARTESIAN_POINT('Ctrl Pts',(-1.15765256317261,4.96104227374008,376.685122246282));
#42686=CARTESIAN_POINT('Ctrl Pts',(1.3486425877949,4.91256176240515,376.605994370822));
#42687=CARTESIAN_POINT('Ctrl Pts',(3.52838655442424,3.67458680959566,376.526866495362));
#42688=CARTESIAN_POINT('Ctrl Pts',(4.85379089203517,1.5468722880489,376.447738619903));
#42689=CARTESIAN_POINT('Ctrl Pts',(5.00393116882618,-0.955391415479512,
376.368610744443));
#42690=CARTESIAN_POINT('Ctrl Pts',(3.94245343483129,-3.22632311019696,376.289482868983));
#42691=CARTESIAN_POINT('Ctrl Pts',(1.92637672105698,-4.71605477417046,376.210354993523));
#42692=CARTESIAN_POINT('Ctrl Pts',(-0.556139808052753,-5.06387286571299,
376.131227118063));
#42693=CARTESIAN_POINT('Ctrl Pts',(-2.90399640996096,-4.18555907527208,
376.052099242604));
#42694=CARTESIAN_POINT('Ctrl Pts',(-4.54869898413812,-2.29378233993093,
375.972971367144));
#42695=CARTESIAN_POINT('Ctrl Pts',(-5.09201038719634,0.153395295307603,
375.893843491684));
#42696=CARTESIAN_POINT('Ctrl Pts',(-4.40237687192385,2.56343088388421,375.814715616224));
#42697=CARTESIAN_POINT('Ctrl Pts',(-2.64678163427568,4.35277456670489,375.735587740765));
#42698=CARTESIAN_POINT('Ctrl Pts',(-0.250312604595216,5.08816711975964,
375.656459865305));
#42699=CARTESIAN_POINT('Ctrl Pts',(2.2067654054518,4.59154485151799,375.577331989845));
#42700=CARTESIAN_POINT('Ctrl Pts',(4.12951222237333,2.98315803496294,375.498204114385));
#42701=CARTESIAN_POINT('Ctrl Pts',(5.05236682718355,0.652447347661906,375.419076238925));
#42702=CARTESIAN_POINT('Ctrl Pts',(4.75187571715042,-1.83623790240596,375.339948363465));
#42703=CARTESIAN_POINT('Ctrl Pts',(3.30079722094991,-3.88031871785061,375.260820488006));
#42704=CARTESIAN_POINT('Ctrl Pts',(1.05048684235124,-4.98482475543083,375.181692612546));
#42705=CARTESIAN_POINT('Ctrl Pts',(-1.45418293039009,-4.88238291455355,
375.102564737087));
#42706=CARTESIAN_POINT('Ctrl Pts',(-3.60674266297149,-3.59766175932869,
375.023436861626));
#42707=CARTESIAN_POINT('Ctrl Pts',(-4.8859942278021,-1.44202665000967,374.944308986167));
#42708=CARTESIAN_POINT('Ctrl Pts',(-4.98214589566551,1.06316661357685,374.865181110707));
#42709=CARTESIAN_POINT('Ctrl Pts',(-4.24189388987242,2.56091091663634,374.812429193734));
#42710=CARTESIAN_POINT('Ctrl Pts',(-3.71544298812364,3.17665283523617,374.786053235247));
#42711=CARTESIAN_POINT('Ctrl Pts',(-1.21713437249744,-4.54280821229883,
400.213946764753));
#42712=CARTESIAN_POINT('Ctrl Pts',(-1.96999142168732,-4.34109857602909,
400.187570806266));
#42713=CARTESIAN_POINT('Ctrl Pts',(-3.37271299505139,-3.55624125113577,
400.134818889293));
#42714=CARTESIAN_POINT('Ctrl Pts',(-4.66062705172882,-1.51685825396376,
400.055691013833));
#42715=CARTESIAN_POINT('Ctrl Pts',(-4.81980261122079,0.889513643374588,
399.976563138373));
#42716=CARTESIAN_POINT('Ctrl Pts',(-3.81205567514826,3.08066074806192,399.897435262913));
#42717=CARTESIAN_POINT('Ctrl Pts',(-1.8812299991108,4.52580660481483,399.818307387454));
#42718=CARTESIAN_POINT('Ctrl Pts',(0.505078813591743,4.87513817945551,399.739179511994));
#42719=CARTESIAN_POINT('Ctrl Pts',(2.76910316187124,4.04402084397575,399.660051636534));
#42720=CARTESIAN_POINT('Ctrl Pts',(4.36262999826625,2.23371923467566,399.580923761074));
#42721=CARTESIAN_POINT('Ctrl Pts',(4.89982180424067,-0.117443592687962,
399.501795885615));
#42722=CARTESIAN_POINT('Ctrl Pts',(4.25060268019241,-2.44016773763421,399.422668010155));
#42723=CARTESIAN_POINT('Ctrl Pts',(2.57217199816948,-4.17204698619159,399.343540134695));
#42724=CARTESIAN_POINT('Ctrl Pts',(0.270932724605363,-4.89373465051516,
399.264412259235));
#42725=CARTESIAN_POINT('Ctrl Pts',(-2.09590823180696,-4.43048672079232,
399.185284383776));
#42726=CARTESIAN_POINT('Ctrl Pts',(-3.95526022334416,-2.89447065191351,
399.106156508316));
#42727=CARTESIAN_POINT('Ctrl Pts',(-4.85691225648777,-0.657607098051338,
399.027028632856));
#42728=CARTESIAN_POINT('Ctrl Pts',(-4.58254445676102,1.73848500455744,398.947900757396));
#42729=CARTESIAN_POINT('Ctrl Pts',(-3.1985903647966,3.71363211084189,398.868772881936));
#42730=CARTESIAN_POINT('Ctrl Pts',(-1.0401512631882,4.78958548759503,398.789645006477));
#42731=CARTESIAN_POINT('Ctrl Pts',(1.37014302373642,4.70582106344184,398.710517131017));
#42732=CARTESIAN_POINT('Ctrl Pts',(3.44868015565118,3.48262099178473,398.631389255557));
#42733=CARTESIAN_POINT('Ctrl Pts',(4.69217722656672,1.41616265411303,398.552261380097));
#42734=CARTESIAN_POINT('Ctrl Pts',(4.79954227516165,-0.993195719354361,
398.473133504638));
#42735=CARTESIAN_POINT('Ctrl Pts',(3.74477865578454,-3.16206840652194,398.394005629178));
#42736=CARTESIAN_POINT('Ctrl Pts',(1.78327968915111,-4.56529926055421,398.314877753718));
#42737=CARTESIAN_POINT('Ctrl Pts',(-0.610010546527312,-4.8631194640233,
398.235749878258));
#42738=CARTESIAN_POINT('Ctrl Pts',(-2.85559695895555,-3.9834168494165,398.156622002799));
#42739=CARTESIAN_POINT('Ctrl Pts',(-4.40974845943849,-2.13919665124415,
398.077494127339));
#42740=CARTESIAN_POINT('Ctrl Pts',(-4.89615332706093,0.22299413922299,397.998366251879));
#42741=CARTESIAN_POINT('Ctrl Pts',(-4.19703678069868,2.53119063874627,397.919238376419));
#42742=CARTESIAN_POINT('Ctrl Pts',(-2.48167816706011,4.22650177609728,397.840110500959));
#42743=CARTESIAN_POINT('Ctrl Pts',(-0.165422805885864,4.89843639169769,
397.7609826255));
#42744=CARTESIAN_POINT('Ctrl Pts',(2.19088691340144,4.38429678750219,397.68185475004));
#42745=CARTESIAN_POINT('Ctrl Pts',(4.01671011032052,2.80857324594973,397.60272687458));
#42746=CARTESIAN_POINT('Ctrl Pts',(4.86995431890775,0.55280079591789,397.52359899912));
#42747=CARTESIAN_POINT('Ctrl Pts',(4.54402076394769,-1.83682309573565,397.444471123661));
#42748=CARTESIAN_POINT('Ctrl Pts',(3.11782878949058,-3.78169108040825,397.365343248201));
#42749=CARTESIAN_POINT('Ctrl Pts',(0.93670686325944,-4.81088599330085,397.286215372741));
#42750=CARTESIAN_POINT('Ctrl Pts',(-1.47122292025061,-4.67520554704762,
397.207087497281));
#42751=CARTESIAN_POINT('Ctrl Pts',(-3.52292074773491,-3.40750248619052,
397.127959621821));
#42752=CARTESIAN_POINT('Ctrl Pts',(-4.72160239961778,-1.31472984606697,
397.048831746362));
#42753=CARTESIAN_POINT('Ctrl Pts',(-4.77702721717586,1.09638257673893,396.969703870902));
#42754=CARTESIAN_POINT('Ctrl Pts',(-3.67577501037587,3.24202434619358,396.890575995442));
#42755=CARTESIAN_POINT('Ctrl Pts',(-1.68449553181902,4.60266429272193,396.811448119982));
#42756=CARTESIAN_POINT('Ctrl Pts',(0.714656288826095,4.84884627278046,396.732320244522));
#42757=CARTESIAN_POINT('Ctrl Pts',(2.94076607474594,3.92096144865504,396.653192369063));
#42758=CARTESIAN_POINT('Ctrl Pts',(4.45481867572026,2.0436815688041,396.574064493603));
#42759=CARTESIAN_POINT('Ctrl Pts',(4.89021164683945,-0.328441528025053,
396.494936618143));
#42760=CARTESIAN_POINT('Ctrl Pts',(4.14152188219155,-2.62103801718789,396.415808742683));
#42761=CARTESIAN_POINT('Ctrl Pts',(2.39003205189126,-4.27899410833295,396.336680867224));
#42762=CARTESIAN_POINT('Ctrl Pts',(0.0598360438320979,-4.90086353983399,
396.257552991764));
#42763=CARTESIAN_POINT('Ctrl Pts',(-2.28484825872123,-4.33607105832391,
396.178425116304));
#42764=CARTESIAN_POINT('Ctrl Pts',(-4.07629487497772,-2.72137169097608,
396.099297240844));
#42765=CARTESIAN_POINT('Ctrl Pts',(-4.88073505144618,-0.447737809214611,
396.020169365385));
#42766=CARTESIAN_POINT('Ctrl Pts',(-4.50338709078854,1.93430827396637,395.941041489924));
#42767=CARTESIAN_POINT('Ctrl Pts',(-3.03561947311557,3.84799404919722,395.861913614465));
#42768=CARTESIAN_POINT('Ctrl Pts',(-0.832827510883269,4.82995260073343,
395.782785739005));
#42769=CARTESIAN_POINT('Ctrl Pts',(1.57161966562715,4.64241913390311,395.703657863545));
#42770=CARTESIAN_POINT('Ctrl Pts',(3.5955254979886,3.3308017325457,395.624529988085));
#42771=CARTESIAN_POINT('Ctrl Pts',(4.74883513214048,1.21268655305647,395.545402112626));
#42772=CARTESIAN_POINT('Ctrl Pts',(4.75229398251168,-1.19906033709689,395.466274237166));
#42773=CARTESIAN_POINT('Ctrl Pts',(3.60506454649375,-3.32047487625331,395.387146361706));
#42774=CARTESIAN_POINT('Ctrl Pts',(1.5849291916516,-4.63789211233576,395.308018486247));
#42775=CARTESIAN_POINT('Ctrl Pts',(-0.818970185850148,-4.83232155624025,
395.228890610786));
#42776=CARTESIAN_POINT('Ctrl Pts',(-3.02456966792716,-3.85668537893236,
395.149762735327));
#42777=CARTESIAN_POINT('Ctrl Pts',(-4.49782033045318,-1.94721751819814,
395.070634859867));
#42778=CARTESIAN_POINT('Ctrl Pts',(-4.88199923361805,0.433736407473957,
394.991506984407));
#42779=CARTESIAN_POINT('Ctrl Pts',(-4.08408389914571,2.70966833633831,394.912379108948));
#42780=CARTESIAN_POINT('Ctrl Pts',(-2.29727614331402,4.32949952183574,394.833251233488));
#42781=CARTESIAN_POINT('Ctrl Pts',(0.04577850263863,4.90101500884376,394.754123358028));
#42782=CARTESIAN_POINT('Ctrl Pts',(2.37774865193587,4.28583190716024,394.674995482568));
#42783=CARTESIAN_POINT('Ctrl Pts',(4.13398684276656,2.63290648752449,394.595867607109));
#42784=CARTESIAN_POINT('Ctrl Pts',(4.8892494513703,0.34246691882695,394.516739731649));
#42785=CARTESIAN_POINT('Ctrl Pts',(4.46066230370267,-2.03089527069752,394.437611856189));
#42786=CARTESIAN_POINT('Ctrl Pts',(2.95200058966839,-3.91251023088926,394.358483980729));
#42787=CARTESIAN_POINT('Ctrl Pts',(0.728561441315958,-4.84677645600076,
394.279356105269));
#42788=CARTESIAN_POINT('Ctrl Pts',(-1.67128664123166,-4.60747704834829,
394.200228229809));
#42789=CARTESIAN_POINT('Ctrl Pts',(-3.66646069301835,-3.25255434616657,
394.12110035435));
#42790=CARTESIAN_POINT('Ctrl Pts',(-4.7738627787844,-1.11008015816539,394.04197247889));
#42791=CARTESIAN_POINT('Ctrl Pts',(-4.72535405587758,1.30118132280515,393.96284460343));
#42792=CARTESIAN_POINT('Ctrl Pts',(-3.53268009800228,3.39738356877675,393.88371672797));
#42793=CARTESIAN_POINT('Ctrl Pts',(-1.48462690153391,4.6709663616277,393.804588852511));
#42794=CARTESIAN_POINT('Ctrl Pts',(0.922903800227676,4.81355298752812,393.725460977051));
#42795=CARTESIAN_POINT('Ctrl Pts',(3.10696882493013,3.79061848635918,393.646333101591));
#42796=CARTESIAN_POINT('Ctrl Pts',(4.53873345614266,1.84984929178215,393.567205226131));
#42797=CARTESIAN_POINT('Ctrl Pts',(4.87151990076886,-0.538829884684078,
393.488077350672));
#42798=CARTESIAN_POINT('Ctrl Pts',(4.02474950245672,-2.79704044137549,393.408949475212));
#42799=CARTESIAN_POINT('Ctrl Pts',(2.2034535118369,-4.37799456479668,393.329821599752));
#42800=CARTESIAN_POINT('Ctrl Pts',(-0.151371792205916,-4.89889072839352,
393.250693724292));
#42801=CARTESIAN_POINT('Ctrl Pts',(-2.46954495544641,-4.23360266218321,
393.171565848832));
#42802=CARTESIAN_POINT('Ctrl Pts',(-4.18975922485567,-2.54321871374691,
393.092437973373));
#42803=CARTESIAN_POINT('Ctrl Pts',(-4.89549356508254,-0.23703700650118,
393.013310097913));
#42804=CARTESIAN_POINT('Ctrl Pts',(-4.41586624162366,2.12653923648359,392.934182222453));
#42805=CARTESIAN_POINT('Ctrl Pts',(-2.86701096694867,3.97520966788064,392.855054346993));
#42806=CARTESIAN_POINT('Ctrl Pts',(-0.623957069722673,4.86134974707218,
392.775926471534));
#42807=CARTESIAN_POINT('Ctrl Pts',(1.7701775674537,4.57039551547777,392.696798596074));
#42808=CARTESIAN_POINT('Ctrl Pts',(3.73569339459987,3.17279666063845,392.617670720614));
#42809=CARTESIAN_POINT('Ctrl Pts',(4.79667371815007,1.00695830590151,392.538542845154));
#42810=CARTESIAN_POINT('Ctrl Pts',(4.69621994662587,-1.40269811475204,392.459414969694));
#42811=CARTESIAN_POINT('Ctrl Pts',(3.45865527607574,-3.47271471179091,392.380287094234));
#42812=CARTESIAN_POINT('Ctrl Pts',(1.38363523608003,-4.70187168281881,392.301159218775));
#42813=CARTESIAN_POINT('Ctrl Pts',(-1.02640887116651,-4.79254928168782,
392.222031343315));
#42814=CARTESIAN_POINT('Ctrl Pts',(-3.18792528432602,-3.72279144860016,
392.142903467855));
#42815=CARTESIAN_POINT('Ctrl Pts',(-4.5775390550865,-1.75162210175979,392.063775592395));
#42816=CARTESIAN_POINT('Ctrl Pts',(-4.85877851429126,0.64367316028962,391.984647716936));
#42817=CARTESIAN_POINT('Ctrl Pts',(-3.96354624360545,2.88311376171958,391.905519841476));
#42818=CARTESIAN_POINT('Ctrl Pts',(-2.1086077232932,4.4244567189073,391.826391966016));
#42819=CARTESIAN_POINT('Ctrl Pts',(0.256894793419963,4.89449168487693,391.747264090557));
#42820=CARTESIAN_POINT('Ctrl Pts',(2.56019454432978,4.17940757564988,391.668136215096));
#42821=CARTESIAN_POINT('Ctrl Pts',(4.24358612375888,2.45235001548652,391.589008339637));
#42822=CARTESIAN_POINT('Ctrl Pts',(4.89946449317567,0.131497027824103,391.509880464177));
#42823=CARTESIAN_POINT('Ctrl Pts',(4.36901970526599,-2.22119575976841,391.430752588718));
#42824=CARTESIAN_POINT('Ctrl Pts',(2.78069006924853,-4.03606324615933,391.351624713257));
#42825=CARTESIAN_POINT('Ctrl Pts',(0.519062968356706,-4.87366570694958,
391.272496837798));
#42826=CARTESIAN_POINT('Ctrl Pts',(-1.86824652503536,-4.5311917538225,391.193368962338));
#42827=CARTESIAN_POINT('Ctrl Pts',(-3.80319145504887,-3.09156571084279,
391.114241086878));
#42828=CARTESIAN_POINT('Ctrl Pts',(-4.81725735814933,-0.903368880121367,
391.035113211418));
#42829=CARTESIAN_POINT('Ctrl Pts',(-4.66490518296109,1.50356357437869,390.955985335959));
#42830=CARTESIAN_POINT('Ctrl Pts',(-3.38302445358346,3.54643332584613,390.876857460499));
#42831=CARTESIAN_POINT('Ctrl Pts',(-1.28200109001022,4.73059372525567,390.797729585039));
#42832=CARTESIAN_POINT('Ctrl Pts',(1.12943733686538,4.76932019163214,390.718601709579));
#42833=CARTESIAN_POINT('Ctrl Pts',(3.2674014545917,3.65323576063024,390.639473834119));
#42834=CARTESIAN_POINT('Ctrl Pts',(4.61421910819667,1.65258155918805,390.56034595866));
#42835=CARTESIAN_POINT('Ctrl Pts',(4.84378099055226,-0.74821755110413,390.4812180832));
#42836=CARTESIAN_POINT('Ctrl Pts',(3.90050254186479,-2.96784832987165,390.40209020774));
#42837=CARTESIAN_POINT('Ctrl Pts',(2.01278281861149,-4.46886440981576,390.32296233228));
#42838=CARTESIAN_POINT('Ctrl Pts',(-0.362298507468694,-4.88781992095675,
390.243834456821));
#42839=CARTESIAN_POINT('Ctrl Pts',(-2.6496553261311,-4.12327181264112,390.164706581361));
#42840=CARTESIAN_POINT('Ctrl Pts',(-4.29544254536053,-2.36034258693993,
390.085578705901));
#42841=CARTESIAN_POINT('Ctrl Pts',(-4.90116039177906,-0.0258959894911138,
390.006450830441));
#42842=CARTESIAN_POINT('Ctrl Pts',(-4.32014444746653,2.31482088750723,389.927322954982));
#42843=CARTESIAN_POINT('Ctrl Pts',(-2.69307797902764,4.09504270882394,389.848195079522));
#42844=CARTESIAN_POINT('Ctrl Pts',(-0.41392784400509,4.88371861680963,389.769067204062));
#42845=CARTESIAN_POINT('Ctrl Pts',(1.96544797639375,4.48988396735431,389.689939328602));
#42846=CARTESIAN_POINT('Ctrl Pts',(3.86892353214857,3.00889921576025,389.610811453142));
#42847=CARTESIAN_POINT('Ctrl Pts',(4.83560414092378,0.799359981795764,389.531683577683));
#42848=CARTESIAN_POINT('Ctrl Pts',(4.63142430565821,-1.60373086556754,389.452555702223));
#42849=CARTESIAN_POINT('Ctrl Pts',(3.30582274912905,-3.61850518025834,389.373427826763));
#42850=CARTESIAN_POINT('Ctrl Pts',(1.17977165637593,-4.75711915207383,389.294299951303));
#42851=CARTESIAN_POINT('Ctrl Pts',(-1.23194135683111,-4.74387650361441,
389.215172075843));
#42852=CARTESIAN_POINT('Ctrl Pts',(-3.34536043156536,-3.58198372010992,
389.136044200384));
#42853=CARTESIAN_POINT('Ctrl Pts',(-4.64875658336638,-1.55277365279788,
389.056916324924));
#42854=CARTESIAN_POINT('Ctrl Pts',(-4.82653429353919,0.852414512725966,
388.977788449464));
#42855=CARTESIAN_POINT('Ctrl Pts',(-3.83564767110356,3.05120479997222,388.898660574004));
#42856=CARTESIAN_POINT('Ctrl Pts',(-1.91602329336559,4.5111970171448,388.819532698545));
#42857=CARTESIAN_POINT('Ctrl Pts',(0.467533990930312,4.87887853461636,388.740404823085));
#42858=CARTESIAN_POINT('Ctrl Pts',(2.73788576040913,4.06522143937628,388.661276947625));
#42859=CARTESIAN_POINT('Ctrl Pts',(4.34530441052119,2.26723915106472,388.582149072165));
#42860=CARTESIAN_POINT('Ctrl Pts',(4.90058047341499,-0.0797170734497908,
388.503021196706));
#42861=CARTESIAN_POINT('Ctrl Pts',(4.26926316308366,-2.40737114557615,388.423893321245));
#42862=CARTESIAN_POINT('Ctrl Pts',(2.60421537830119,-4.1521206692045,388.344765445786));
#42863=CARTESIAN_POINT('Ctrl Pts',(0.308600515372232,-4.89150380865921,
388.265637570326));
#42864=CARTESIAN_POINT('Ctrl Pts',(-2.06173678676592,-4.44649133703325,
388.186509694866));
#42865=CARTESIAN_POINT('Ctrl Pts',(-3.93285910370337,-2.92483556095608,
388.107381819407));
#42866=CARTESIAN_POINT('Ctrl Pts',(-4.85170554728278,-0.694979906674425,
388.028253943947));
#42867=CARTESIAN_POINT('Ctrl Pts',(-4.59579286131083,1.70315347639018,387.949126068487));
#42868=CARTESIAN_POINT('Ctrl Pts',(-3.22708601074344,3.68889680900396,387.869998193027));
#42869=CARTESIAN_POINT('Ctrl Pts',(-1.07699440464578,4.78143564639088,387.790870317567));
#42870=CARTESIAN_POINT('Ctrl Pts',(1.3338733340929,4.71623003221975,387.711742442108));
#42871=CARTESIAN_POINT('Ctrl Pts',(3.42176601558219,3.50906841238845,387.632614566648));
#42872=CARTESIAN_POINT('Ctrl Pts',(4.68113544337878,1.45224472764016,387.553486691188));
#42873=CARTESIAN_POINT('Ctrl Pts',(4.80704643162612,-0.956215662079578,
387.474358815728));
#42874=CARTESIAN_POINT('Ctrl Pts',(3.76901174619325,-3.13314446607126,387.395230940269));
#42875=CARTESIAN_POINT('Ctrl Pts',(1.81837407711343,-4.5514348840665,387.316103064809));
#42876=CARTESIAN_POINT('Ctrl Pts',(-0.572552378499359,-4.86767167772133,
387.236975189349));
#42877=CARTESIAN_POINT('Ctrl Pts',(-2.82484487802531,-4.00528341110962,
387.157847313889));
#42878=CARTESIAN_POINT('Ctrl Pts',(-4.39314856625886,-2.173082939741,387.07871943843));
#42879=CARTESIAN_POINT('Ctrl Pts',(-4.89772500736415,0.185293120367267,
386.99959156297));
#42880=CARTESIAN_POINT('Ctrl Pts',(-4.21639947845907,2.4988035589589,386.92046368751));
#42881=CARTESIAN_POINT('Ctrl Pts',(-2.51414352974947,4.20727062357945,386.84133581205));
#42882=CARTESIAN_POINT('Ctrl Pts',(-0.203129890410879,4.89701766750308,
386.762207936591));
#42883=CARTESIAN_POINT('Ctrl Pts',(2.15706824516707,4.40103401190078,386.68308006113));
#42884=CARTESIAN_POINT('Ctrl Pts',(3.99496848171146,2.83941378075611,386.603952185671));
#42885=CARTESIAN_POINT('Ctrl Pts',(4.86555410065941,0.590277122860157,386.524824310211));
#42886=CARTESIAN_POINT('Ctrl Pts',(4.55802739511214,-1.80178524070515,386.445696434751));
#42887=CARTESIAN_POINT('Ctrl Pts',(3.14685079923878,-3.75757552625969,386.366568559291));
#42888=CARTESIAN_POINT('Ctrl Pts',(0.973717058663619,-4.80353191702554,
386.287440683832));
#42889=CARTESIAN_POINT('Ctrl Pts',(-1.43518593730373,-4.68639361487927,
386.208312808372));
#42890=CARTESIAN_POINT('Ctrl Pts',(-3.49658272828396,-3.43452369514056,
386.129184932912));
#42891=CARTESIAN_POINT('Ctrl Pts',(-4.71134065335373,-1.35104146356512,
386.050057057452));
#42892=CARTESIAN_POINT('Ctrl Pts',(-4.78532645385515,1.05957279988197,385.970929181993));
#42893=CARTESIAN_POINT('Ctrl Pts',(-3.70062570902444,3.21362928010108,385.891801306533));
#42894=CARTESIAN_POINT('Ctrl Pts',(-1.71988051253413,4.58955932643004,385.812673431073));
#42895=CARTESIAN_POINT('Ctrl Pts',(0.677304905677504,4.85420455409132,385.733545555613));
#42896=CARTESIAN_POINT('Ctrl Pts',(2.91049230016732,3.94348555961378,385.654417680154));
#42897=CARTESIAN_POINT('Ctrl Pts',(4.43895279649954,2.07791767369751,385.575289804694));
#42898=CARTESIAN_POINT('Ctrl Pts',(4.89259531954076,-0.29078312781775,385.496161929234));
#42899=CARTESIAN_POINT('Ctrl Pts',(4.16157794044722,-2.58907567170192,385.417034053774));
#42900=CARTESIAN_POINT('Ctrl Pts',(2.42290425755801,-4.26046696348217,385.337906178315));
#42901=CARTESIAN_POINT('Ctrl Pts',(0.0975649436126985,-4.90025763302231,
385.258778302854));
#42902=CARTESIAN_POINT('Ctrl Pts',(-2.25139808515128,-4.35353309972404,
385.179650427395));
#42903=CARTESIAN_POINT('Ctrl Pts',(-4.05522282615024,-2.75267354012164,
385.100522551935));
#42904=CARTESIAN_POINT('Ctrl Pts',(-4.87714337058205,-0.485300248303261,
385.021394676475));
#42905=CARTESIAN_POINT('Ctrl Pts',(-4.51814544317236,1.89958035959429,384.942266801015));
#42906=CARTESIAN_POINT('Ctrl Pts',(-3.06515437123229,3.82450944157957,384.863138925556));
#42907=CARTESIAN_POINT('Ctrl Pts',(-0.869987574488363,4.82339770374075,
384.784011050096));
#42908=CARTESIAN_POINT('Ctrl Pts',(1.53583212271834,4.65438110590894,384.704883174636));
#42909=CARTESIAN_POINT('Ctrl Pts',(3.56977582909287,3.35838418264497,384.625755299176));
#42910=CARTESIAN_POINT('Ctrl Pts',(4.73935818772915,1.24921085354728,384.546627423716));
#42911=CARTESIAN_POINT('Ctrl Pts',(4.76138444573462,-1.16243793302357,384.467499548257));
#42912=CARTESIAN_POINT('Ctrl Pts',(3.6305213141391,-3.29262186954369,384.388371672797));
#42913=CARTESIAN_POINT('Ctrl Pts',(1.62058833437354,-4.62555264143734,384.309243797337));
#42914=CARTESIAN_POINT('Ctrl Pts',(-0.781742931416587,-4.83848341708389,
384.230115921878));
#42915=CARTESIAN_POINT('Ctrl Pts',(-2.9947882570989,-3.87985658025632,384.150988046417));
#42916=CARTESIAN_POINT('Ctrl Pts',(-4.48269583239351,-1.98178754220968,
384.071860170958));
#42917=CARTESIAN_POINT('Ctrl Pts',(-4.88519379187676,0.396138112309837,
383.992732295498));
#42918=CARTESIAN_POINT('Ctrl Pts',(-4.10482400501691,2.67814556662863,383.913604420039));
#42919=CARTESIAN_POINT('Ctrl Pts',(-2.33053992799659,4.31168498759236,383.834476544578));
#42920=CARTESIAN_POINT('Ctrl Pts',(0.00804530673338092,4.90122220076332,
383.755348669119));
#42921=CARTESIAN_POINT('Ctrl Pts',(2.34468250536694,4.30401065719426,383.676220793659));
#42922=CARTESIAN_POINT('Ctrl Pts',(4.11359415836805,2.66465511623097,383.5970929182));
#42923=CARTESIAN_POINT('Ctrl Pts',(4.88646797566037,0.380098028225917,383.517965042739));
#42924=CARTESIAN_POINT('Ctrl Pts',(4.47616552437595,-1.99649342262975,383.43883716728));
#42925=CARTESIAN_POINT('Ctrl Pts',(2.98203466184577,-3.88966747470347,383.35970929182));
#42926=CARTESIAN_POINT('Ctrl Pts',(0.765854118125881,-4.84102378200782,
383.28058141636));
#42927=CARTESIAN_POINT('Ctrl Pts',(-1.6357651560373,-4.62020737007657,383.2014535409));
#42928=CARTESIAN_POINT('Ctrl Pts',(-3.6413113313429,-3.28068522971184,383.122325665441));
#42929=CARTESIAN_POINT('Ctrl Pts',(-4.76517503677366,-1.14680018186465,
383.043197789981));
#42930=CARTESIAN_POINT('Ctrl Pts',(-4.73523152455593,1.26476329685335,382.964069914521));
#42931=CARTESIAN_POINT('Ctrl Pts',(-3.55873111398586,3.37008555478411,382.884942039061));
#42932=CARTESIAN_POINT('Ctrl Pts',(-1.52054364820804,4.65939811586324,382.805814163601));
#42933=CARTESIAN_POINT('Ctrl Pts',(0.885817960704724,4.82051556669083,382.726686288142));
#42934=CARTESIAN_POINT('Ctrl Pts',(3.07769360662633,3.8144260186753,382.647558412682));
#42935=CARTESIAN_POINT('Ctrl Pts',(4.52435736219093,1.88473718258125,382.568430537222));
#42936=CARTESIAN_POINT('Ctrl Pts',(4.87552386121587,-0.501309153048634,
382.489302661763));
#42937=CARTESIAN_POINT('Ctrl Pts',(4.04616402543129,-2.76597188480314,382.410174786302));
#42938=CARTESIAN_POINT('Ctrl Pts',(2.23709342974706,-4.36090091320568,382.331046910843));
#42939=CARTESIAN_POINT('Ctrl Pts',(-0.113651821301689,-4.89991092283629,
382.251919035383));
#42940=CARTESIAN_POINT('Ctrl Pts',(-2.43687818989498,-4.25248967968529,
382.172791159923));
#42941=CARTESIAN_POINT('Ctrl Pts',(-4.17005537407579,-2.5753993797773,382.093663284464));
#42942=CARTESIAN_POINT('Ctrl Pts',(-4.89352358608415,-0.274719312487676,
382.014535409004));
#42943=CARTESIAN_POINT('Ctrl Pts',(-4.43210713178239,2.09247942895964,381.935407533544));
#42944=CARTESIAN_POINT('Ctrl Pts',(-2.89753026709117,3.95301936998874,381.856279658084));
#42945=CARTESIAN_POINT('Ctrl Pts',(-0.661365043163431,4.85640196728989,
381.777151782624));
#42946=CARTESIAN_POINT('Ctrl Pts',(1.73493863410831,4.58388827569936,381.698023907165));
#42947=CARTESIAN_POINT('Ctrl Pts',(3.7111560180617,3.20146291526546,381.618896031705));
#42948=CARTESIAN_POINT('Ctrl Pts',(4.78877921262759,1.04385700214232,381.539768156245));
#42949=CARTESIAN_POINT('Ctrl Pts',(4.70687983423134,-1.36650137735827,381.460640280785));
#42950=CARTESIAN_POINT('Ctrl Pts',(3.48528844380413,-3.44598436614286,381.381512405325));
#42951=CARTESIAN_POINT('Ctrl Pts',(1.41979290903503,-4.69108003381625,381.302384529866));
#42952=CARTESIAN_POINT('Ctrl Pts',(-0.989481667084847,-4.80030934614829,
381.223256654406));
#42953=CARTESIAN_POINT('Ctrl Pts',(-3.1591698522741,-3.74722425705989,381.144128778946));
#42954=CARTESIAN_POINT('Ctrl Pts',(-4.56391804067381,-1.78681165941677,
381.065000903487));
#42955=CARTESIAN_POINT('Ctrl Pts',(-4.86359001771767,0.606247414652442,
380.985873028026));
#42956=CARTESIAN_POINT('Ctrl Pts',(-3.98562524001068,2.85251384473511,380.906745152567));
#42957=CARTESIAN_POINT('Ctrl Pts',(-2.1426081539881,4.40809188727722,380.827617277107));
#42958=CARTESIAN_POINT('Ctrl Pts',(0.219205562501549,4.89632440812331,380.748489401647));
#42959=CARTESIAN_POINT('Ctrl Pts',(2.52794232836271,4.19899409057548,380.669361526187));
#42960=CARTESIAN_POINT('Ctrl Pts',(4.22458025593252,2.48494777599062,380.590233650728));
#42961=CARTESIAN_POINT('Ctrl Pts',(4.89830692563373,0.169213032902914,380.511105775268));
#42962=CARTESIAN_POINT('Ctrl Pts',(4.38599072357506,-2.18749380820361,380.431977899808));
#42963=CARTESIAN_POINT('Ctrl Pts',(2.81168042594869,-4.01453571045926,380.352850024348));
#42964=CARTESIAN_POINT('Ctrl Pts',(0.556568868317172,-4.86952511884227,
380.273722148889));
#42965=CARTESIAN_POINT('Ctrl Pts',(-1.83330650647258,-4.54544068727564,
380.194594273429));
#42966=CARTESIAN_POINT('Ctrl Pts',(-3.77927745739419,-3.12075402559187,
380.115466397969));
#42967=CARTESIAN_POINT('Ctrl Pts',(-4.81015975486937,-0.940429115271696,
380.036338522509));
#42968=CARTESIAN_POINT('Ctrl Pts',(-4.67634253965503,1.46760493322567,379.95721064705));
#42969=CARTESIAN_POINT('Ctrl Pts',(-3.41022740614562,3.5202830605775,379.878082771589));
#42970=CARTESIAN_POINT('Ctrl Pts',(-1.31838289970275,4.72058368403601,379.79895489613));
#42971=CARTESIAN_POINT('Ctrl Pts',(1.09268591509449,4.77787413806285,379.71982702067));
#42972=CARTESIAN_POINT('Ctrl Pts',(3.23917916116038,3.67828250004266,379.64069914521));
#42973=CARTESIAN_POINT('Ctrl Pts',(4.60135949813868,1.68805644369628,379.56157126975));
#42974=CARTESIAN_POINT('Ctrl Pts',(4.8493978027726,-0.71090416982881,379.482443394291));
#42975=CARTESIAN_POINT('Ctrl Pts',(3.92323575948474,-2.93773126131644,379.403315518831));
#42976=CARTESIAN_POINT('Ctrl Pts',(2.04712797424676,-4.45323599703316,379.324187643371));
#42977=CARTESIAN_POINT('Ctrl Pts',(-0.324657517247101,-4.89046432199546,
379.245059767911));
#42978=CARTESIAN_POINT('Ctrl Pts',(-2.61783263582229,-4.14354873013934,
379.165931892452));
#42979=CARTESIAN_POINT('Ctrl Pts',(-4.27714348571947,-2.39334230539285,
379.086804016992));
#42980=CARTESIAN_POINT('Ctrl Pts',(-4.90081577320139,-0.0636281805188475,
379.007676141532));
#42981=CARTESIAN_POINT('Ctrl Pts',(-4.33783771356114,2.28149244114949,378.928548266072));
#42982=CARTESIAN_POINT('Ctrl Pts',(-2.72452500214632,4.07418793146503,378.849420390613));
#42983=CARTESIAN_POINT('Ctrl Pts',(-0.451514254902642,4.88038714302825,
378.770292515153));
#42984=CARTESIAN_POINT('Ctrl Pts',(1.93082309674852,4.50488245765392,378.691164639693));
#42985=CARTESIAN_POINT('Ctrl Pts',(3.84564401766237,3.03859603725688,378.612036764233));
#42986=CARTESIAN_POINT('Ctrl Pts',(4.82930673560502,0.836564547214143,378.532908888774));
#42987=CARTESIAN_POINT('Ctrl Pts',(4.64363382059009,-1.56802701777984,378.453781013314));
#42988=CARTESIAN_POINT('Ctrl Pts',(3.33358285503851,-3.59294713804823,378.374653137854));
#42989=CARTESIAN_POINT('Ctrl Pts',(1.21636070918609,-4.74789536672449,378.295525262394));
#42990=CARTESIAN_POINT('Ctrl Pts',(-1.19538278261738,-4.7532203600546,378.216397386934));
#42991=CARTESIAN_POINT('Ctrl Pts',(-3.31768438156428,-3.60763276020996,
378.137269511475));
#42992=CARTESIAN_POINT('Ctrl Pts',(-4.6366643489263,-1.58851739166163,378.058141636015));
#42993=CARTESIAN_POINT('Ctrl Pts',(-4.83295380642895,0.815230822000412,
377.979013760555));
#42994=CARTESIAN_POINT('Ctrl Pts',(-3.85902455393964,3.02158456448046,377.899885885095));
#42995=CARTESIAN_POINT('Ctrl Pts',(-1.95069722602663,4.49631228014555,377.820758009635));
#42996=CARTESIAN_POINT('Ctrl Pts',(0.429958719716191,4.88233338553971,377.741630134176));
#42997=CARTESIAN_POINT('Ctrl Pts',(2.70650737238561,4.08617934401293,377.662502258716));
#42998=CARTESIAN_POINT('Ctrl Pts',(4.32772065609622,2.30062550429524,377.583374383256));
#42999=CARTESIAN_POINT('Ctrl Pts',(4.9010489638226,-0.0419862171323538,
377.504246507796));
#43000=CARTESIAN_POINT('Ctrl Pts',(4.28767046122876,-2.37443168023888,377.425118632336));
#43001=CARTESIAN_POINT('Ctrl Pts',(2.63610446564972,-4.13194833394574,377.345990756877));
#43002=CARTESIAN_POINT('Ctrl Pts',(0.346249984239667,-4.88898299614862,
377.266862881417));
#43003=CARTESIAN_POINT('Ctrl Pts',(-2.0274431238406,-4.46223241974302,377.187735005957));
#43004=CARTESIAN_POINT('Ctrl Pts',(-3.91022488205308,-2.95502709970493,
377.108607130498));
#43005=CARTESIAN_POINT('Ctrl Pts',(-4.84621126407803,-0.732311526700024,
377.029479255038));
#43006=CARTESIAN_POINT('Ctrl Pts',(-4.60876886508425,1.66772100077964,376.950351379578));
#43007=CARTESIAN_POINT('Ctrl Pts',(-3.25539037980364,3.66394285754004,376.871223504118));
#43008=CARTESIAN_POINT('Ctrl Pts',(-1.11377371072242,4.77300239990086,376.792095628659));
#43009=CARTESIAN_POINT('Ctrl Pts',(1.29752458313577,4.72635945993341,376.712967753198));
#43010=CARTESIAN_POINT('Ctrl Pts',(3.39464906017594,3.53530784320889,376.633839877739));
#43011=CARTESIAN_POINT('Ctrl Pts',(4.66981619949699,1.48824072358315,376.554712002279));
#43012=CARTESIAN_POINT('Ctrl Pts',(4.8142656643279,-0.919178927997845,376.475584126819));
#43013=CARTESIAN_POINT('Ctrl Pts',(3.79302143937608,-3.10403481730793,376.396456251359));
#43014=CARTESIAN_POINT('Ctrl Pts',(1.85336068619839,-4.53730073503479,376.3173283759));
#43015=CARTESIAN_POINT('Ctrl Pts',(-0.535060274040971,-4.87193537309239,
376.23820050044));
#43016=CARTESIAN_POINT('Ctrl Pts',(-2.7939253627036,-4.02691257378452,376.15907262498));
#43017=CARTESIAN_POINT('Ctrl Pts',(-4.37628828172638,-2.20684041966181,
376.07994474952));
#43018=CARTESIAN_POINT('Ctrl Pts',(-4.89900638965642,0.147581107404016,
376.000816874061));
#43019=CARTESIAN_POINT('Ctrl Pts',(-4.23551226043463,2.46626839394683,375.921688998601));
#43020=CARTESIAN_POINT('Ctrl Pts',(-2.54645987583722,4.18779004627332,375.842561123141));
#43021=CARTESIAN_POINT('Ctrl Pts',(-0.24082493083811,4.89530879473852,375.763433247681));
#43022=CARTESIAN_POINT('Ctrl Pts',(2.12312171415927,4.41751014933925,375.684305372222));
#43023=CARTESIAN_POINT('Ctrl Pts',(3.97299008156779,2.87008650088106,375.605177496762));
#43024=CARTESIAN_POINT('Ctrl Pts',(4.86086545139366,0.627717440079687,375.526049621302));
#43025=CARTESIAN_POINT('Ctrl Pts',(4.57176394606508,-1.76663842623643,375.446921745842));
#43026=CARTESIAN_POINT('Ctrl Pts',(3.1756861134954,-3.73324183321634,375.367793870382));
#43027=CARTESIAN_POINT('Ctrl Pts',(1.01066992437191,-4.79588344705227,375.288665994922));
#43028=CARTESIAN_POINT('Ctrl Pts',(-1.39906459845869,-4.69732449000695,
375.209538119463));
#43029=CARTESIAN_POINT('Ctrl Pts',(-3.47003521363053,-3.46129850620319,
375.130410244003));
#43030=CARTESIAN_POINT('Ctrl Pts',(-4.70079892256589,-1.38736908122097,
375.051282368543));
#43031=CARTESIAN_POINT('Ctrl Pts',(-4.79330612491241,1.02286909042425,374.972154493083));
#43032=CARTESIAN_POINT('Ctrl Pts',(-4.08111211300407,2.46384394177367,374.91940257611));
#43033=CARTESIAN_POINT('Ctrl Pts',(-3.57461543774341,3.05624720968232,374.893026617624));
#43034=CARTESIAN_POINT('Ctrl Pts',(-1.16918346556839,-4.36383719750651,
400.320920147129));
#43035=CARTESIAN_POINT('Ctrl Pts',(-1.89238053709901,-4.17007422695751,
400.294544188642));
#43036=CARTESIAN_POINT('Ctrl Pts',(-3.23983970630162,-3.41613758049457,
400.241792271669));
#43037=CARTESIAN_POINT('Ctrl Pts',(-4.47701437999898,-1.45709925725484,
400.162664396209));
#43038=CARTESIAN_POINT('Ctrl Pts',(-4.62991897006387,0.854469866048622,
400.08353652075));
#43039=CARTESIAN_POINT('Ctrl Pts',(-3.66187379628773,2.9592933130866,400.00440864529));
#43040=CARTESIAN_POINT('Ctrl Pts',(-1.80711600920317,4.34750539486619,399.92528076983));
#43041=CARTESIAN_POINT('Ctrl Pts',(0.485180445975455,4.68307450728292,399.84615289437));
#43042=CARTESIAN_POINT('Ctrl Pts',(2.66001002393004,3.8847003355008,399.767025018911));
#43043=CARTESIAN_POINT('Ctrl Pts',(4.19075738523379,2.14571838156707,399.687897143451));
#43044=CARTESIAN_POINT('Ctrl Pts',(4.70678568217143,-0.112816719181106,
399.608769267991));
#43045=CARTESIAN_POINT('Ctrl Pts',(4.0831435580808,-2.34403352376061,399.529641392531));
#43046=CARTESIAN_POINT('Ctrl Pts',(2.47083727056938,-4.00768268816587,399.450513517072));
#43047=CARTESIAN_POINT('Ctrl Pts',(0.26025890735466,-4.70093834136087,399.371385641611));
#43048=CARTESIAN_POINT('Ctrl Pts',(-2.01333665809567,-4.25594078634204,
399.292257766152));
#43049=CARTESIAN_POINT('Ctrl Pts',(-3.79943657795602,-2.78043846617054,
399.213129890692));
#43050=CARTESIAN_POINT('Ctrl Pts',(-4.66556662297687,-0.631699640775407,
399.134002015232));
#43051=CARTESIAN_POINT('Ctrl Pts',(-4.40200797064279,1.66999467634492,399.054874139773));
#43052=CARTESIAN_POINT('Ctrl Pts',(-3.07257690863908,3.56732778180521,398.975746264313));
#43053=CARTESIAN_POINT('Ctrl Pts',(-0.999172881885126,4.60089229715201,
398.896618388853));
#43054=CARTESIAN_POINT('Ctrl Pts',(1.31616410234924,4.52042790313295,398.817490513393));
#43055=CARTESIAN_POINT('Ctrl Pts',(3.3128140221261,3.34541770608376,398.738362637933));
#43056=CARTESIAN_POINT('Ctrl Pts',(4.50732158649137,1.36037071761185,398.659234762474));
#43057=CARTESIAN_POINT('Ctrl Pts',(4.61045682154316,-0.954067224935643,
398.580106887014));
#43058=CARTESIAN_POINT('Ctrl Pts',(3.5972472600316,-3.03749378987274,398.500979011554));
#43059=CARTESIAN_POINT('Ctrl Pts',(1.71302460447423,-4.38544217583732,398.421851136094));
#43060=CARTESIAN_POINT('Ctrl Pts',(-0.58597822963345,-4.67152928789035,
398.342723260635));
#43061=CARTESIAN_POINT('Ctrl Pts',(-2.74309626297668,-3.82648392982927,
398.263595385175));
#43062=CARTESIAN_POINT('Ctrl Pts',(-4.23601954113904,-2.05491966273361,
398.184467509715));
#43063=CARTESIAN_POINT('Ctrl Pts',(-4.70326173037178,0.214208937311664,
398.105339634255));
#43064=CARTESIAN_POINT('Ctrl Pts',(-4.0316879707426,2.43147043571793,398.026211758796));
#43065=CARTESIAN_POINT('Ctrl Pts',(-2.38390858507682,4.05999214669189,397.947083883336));
#43066=CARTESIAN_POINT('Ctrl Pts',(-0.158905716443472,4.70545485011635,
397.867956007876));
#43067=CARTESIAN_POINT('Ctrl Pts',(2.10457350639361,4.2115705775148,397.788828132416));
#43068=CARTESIAN_POINT('Ctrl Pts',(3.85846555079357,2.69792512248606,397.709700256956));
#43069=CARTESIAN_POINT('Ctrl Pts',(4.67809487300653,0.531022346377457,397.630572381497));
#43070=CARTESIAN_POINT('Ctrl Pts',(4.36500197879199,-1.76445858504648,397.551444506037));
#43071=CARTESIAN_POINT('Ctrl Pts',(2.99499706155341,-3.63270546211616,397.472316630577));
#43072=CARTESIAN_POINT('Ctrl Pts',(0.899803835430396,-4.62135363621384,
397.393188755117));
#43073=CARTESIAN_POINT('Ctrl Pts',(-1.41326179868926,-4.4910185327571,397.314060879658));
#43074=CARTESIAN_POINT('Ctrl Pts',(-3.38412979029408,-3.2732586111773,397.234933004198));
#43075=CARTESIAN_POINT('Ctrl Pts',(-4.53558750895661,-1.26293401324019,
397.155805128738));
#43076=CARTESIAN_POINT('Ctrl Pts',(-4.58882877938272,1.0531888751364,397.076677253278));
#43077=CARTESIAN_POINT('Ctrl Pts',(-3.53096212085652,3.11429974059636,396.997549377818));
#43078=CARTESIAN_POINT('Ctrl Pts',(-1.61813220309064,4.42133515428577,396.918421502359));
#43079=CARTESIAN_POINT('Ctrl Pts',(0.686501289701844,4.65781841127795,396.839293626899));
#43080=CARTESIAN_POINT('Ctrl Pts',(2.82491000861503,3.76648905699045,396.760165751439));
#43081=CARTESIAN_POINT('Ctrl Pts',(4.27931414595585,1.96316754593802,396.681037875979));
#43082=CARTESIAN_POINT('Ctrl Pts',(4.69755413190968,-0.315502061769038,
396.601910000519));
#43083=CARTESIAN_POINT('Ctrl Pts',(3.97836016824692,-2.51777813655384,396.52278212506));
#43084=CARTESIAN_POINT('Ctrl Pts',(2.29587301155249,-4.11041646162856,396.4436542496));
#43085=CARTESIAN_POINT('Ctrl Pts',(0.0574787095610184,-4.70778637696628,
396.36452637414));
#43086=CARTESIAN_POINT('Ctrl Pts',(-2.1948330979661,-4.16524477615358,396.28539849868));
#43087=CARTESIAN_POINT('Ctrl Pts',(-3.9157028807147,-2.614159008776,396.206270623221));
#43088=CARTESIAN_POINT('Ctrl Pts',(-4.68845088177226,-0.430098479898641,
396.127142747761));
#43089=CARTESIAN_POINT('Ctrl Pts',(-4.32596913256195,1.85810318263636,396.048014872301));
#43090=CARTESIAN_POINT('Ctrl Pts',(-2.91602650941616,3.69639632203913,395.968886996841));
#43091=CARTESIAN_POINT('Ctrl Pts',(-0.8000169721583,4.63966908490906,395.889759121381));
#43092=CARTESIAN_POINT('Ctrl Pts',(1.50970325769618,4.4595237914943,395.810631245922));
#43093=CARTESIAN_POINT('Ctrl Pts',(3.45387416317228,3.19957960334997,395.731503370462));
#43094=CARTESIAN_POINT('Ctrl Pts',(4.56174736550757,1.16491087491141,395.652375495002));
#43095=CARTESIAN_POINT('Ctrl Pts',(4.56506994907375,-1.15182148498192,395.573247619542));
#43096=CARTESIAN_POINT('Ctrl Pts',(3.46303740598383,-3.18965958966768,395.494119744083));
#43097=CARTESIAN_POINT('Ctrl Pts',(1.52248843418447,-4.45517511900225,395.414991868623));
#43098=CARTESIAN_POINT('Ctrl Pts',(-0.786705578057672,-4.64194471171891,
395.335863993163));
#43099=CARTESIAN_POINT('Ctrl Pts',(-2.90541202853717,-3.70474524328377,
395.256736117703));
#43100=CARTESIAN_POINT('Ctrl Pts',(-4.32062168343229,-1.87050384705749,
395.177608242243));
#43101=CARTESIAN_POINT('Ctrl Pts',(-4.68966525951576,0.416648685217087,
395.098480366784));
#43102=CARTESIAN_POINT('Ctrl Pts',(-3.92318504412731,2.60291672604753,395.019352491324));
#43103=CARTESIAN_POINT('Ctrl Pts',(-2.20677136666199,4.15893213559478,394.940224615864));
#43104=CARTESIAN_POINT('Ctrl Pts',(0.0439749871279553,4.70793187861818,
394.861096740404));
#43105=CARTESIAN_POINT('Ctrl Pts',(2.28407353529635,4.11698487470637,394.781968864944));
#43106=CARTESIAN_POINT('Ctrl Pts',(3.97112198345224,2.52917902999067,394.702840989485));
#43107=CARTESIAN_POINT('Ctrl Pts',(4.69662984363174,0.328974900425354,394.623713114025));
#43108=CARTESIAN_POINT('Ctrl Pts',(4.28492755509978,-1.95088498398772,394.544585238566));
#43109=CARTESIAN_POINT('Ctrl Pts',(2.83570192230001,-3.75837078812964,394.465457363105));
#43110=CARTESIAN_POINT('Ctrl Pts',(0.699858627021958,-4.65583013815851,
394.386329487646));
#43111=CARTESIAN_POINT('Ctrl Pts',(-1.60544369734944,-4.42595830389794,
394.307201612186));
#43112=CARTESIAN_POINT('Ctrl Pts',(-3.52201475555854,-3.12441489479712,
394.228073736726));
#43113=CARTESIAN_POINT('Ctrl Pts',(-4.58578900897716,-1.06634681897889,
394.148945861266));
#43114=CARTESIAN_POINT('Ctrl Pts',(-4.53919136286672,1.24991925518346,394.069817985807));
#43115=CARTESIAN_POINT('Ctrl Pts',(-3.39350465573632,3.26353834429719,393.990690110347));
#43116=CARTESIAN_POINT('Ctrl Pts',(-1.42613770922415,4.48694635665851,393.911562234887));
#43117=CARTESIAN_POINT('Ctrl Pts',(0.886544565594953,4.62391556004391,393.832434359427));
#43118=CARTESIAN_POINT('Ctrl Pts',(2.98456494223475,3.64128115898587,393.753306483967));
#43119=CARTESIAN_POINT('Ctrl Pts',(4.35992297272438,1.77697159378319,393.674178608508));
#43120=CARTESIAN_POINT('Ctrl Pts',(4.67959877632843,-0.51760184098167,393.595050733048));
#43121=CARTESIAN_POINT('Ctrl Pts',(3.86618821853779,-2.68684667073537,393.515922857588));
#43122=CARTESIAN_POINT('Ctrl Pts',(2.116645024084,-4.20551664070214,393.436794982129));
#43123=CARTESIAN_POINT('Ctrl Pts',(-0.14540826436235,-4.70589128750945,
393.357667106668));
#43124=CARTESIAN_POINT('Ctrl Pts',(-2.37225338025842,-4.06681328229544,
393.278539231209));
#43125=CARTESIAN_POINT('Ctrl Pts',(-4.02469712556258,-2.44302464594413,
393.199411355749));
#43126=CARTESIAN_POINT('Ctrl Pts',(-4.70262796074555,-0.227698563931231,
393.120283480289));
#43127=CARTESIAN_POINT('Ctrl Pts',(-4.24189630375331,2.04276090656889,393.04115560483));
#43128=CARTESIAN_POINT('Ctrl Pts',(-2.75406059832286,3.81860008301049,392.962027729369));
#43129=CARTESIAN_POINT('Ctrl Pts',(-0.599375307795595,4.66982929169869,
392.88289985391));
#43130=CARTESIAN_POINT('Ctrl Pts',(1.70043866129603,4.39033765584971,392.80377197845));
#43131=CARTESIAN_POINT('Ctrl Pts',(3.58851992688128,3.04779938768583,392.72464410299));
#43132=CARTESIAN_POINT('Ctrl Pts',(4.60770127580904,0.967287612920714,392.64551622753));
#43133=CARTESIAN_POINT('Ctrl Pts',(4.51120503728849,-1.34743663477919,392.566388352071));
#43134=CARTESIAN_POINT('Ctrl Pts',(3.32239615712367,-3.3359016994408,392.487260476611));
#43135=CARTESIAN_POINT('Ctrl Pts',(1.32912476794421,-4.51663411451929,392.408132601151));
#43136=CARTESIAN_POINT('Ctrl Pts',(-0.985971892830688,-4.60373932795397,
392.329004725692));
#43137=CARTESIAN_POINT('Ctrl Pts',(-3.06233199564761,-3.57612627316698,
392.249876850231));
#43138=CARTESIAN_POINT('Ctrl Pts',(-4.397199764574,-1.68261421711348,392.170748974772));
#43139=CARTESIAN_POINT('Ctrl Pts',(-4.66735935664344,0.618314652224117,
392.091621099312));
#43140=CARTESIAN_POINT('Ctrl Pts',(-3.80739615752567,2.76952899837877,392.012493223852));
#43141=CARTESIAN_POINT('Ctrl Pts',(-2.02553583330784,4.25014834578608,391.933365348393));
#43142=CARTESIAN_POINT('Ctrl Pts',(0.24677402236281,4.70166555117323,391.854237472933));
#43143=CARTESIAN_POINT('Ctrl Pts',(2.45933168720454,4.01475329572239,391.775109597473));
#43144=CARTESIAN_POINT('Ctrl Pts',(4.07640342983146,2.35573586177663,391.695981722014));
#43145=CARTESIAN_POINT('Ctrl Pts',(4.70644244793312,0.126316497321376,391.616853846553));
#43146=CARTESIAN_POINT('Ctrl Pts',(4.19689535976046,-2.13368828848624,391.537725971094));
#43147=CARTESIAN_POINT('Ctrl Pts',(2.67114044701949,-3.87705623966156,391.458598095634));
#43148=CARTESIAN_POINT('Ctrl Pts',(0.498613673152825,-4.68166004512793,
391.379470220174));
#43149=CARTESIAN_POINT('Ctrl Pts',(-1.79464403933883,-4.35267838752966,
391.300342344714));
#43150=CARTESIAN_POINT('Ctrl Pts',(-3.65335879596438,-2.96976865785062,
391.221214469255));
#43151=CARTESIAN_POINT('Ctrl Pts',(-4.62747399120691,-0.867779254134205,
391.142086593794));
#43152=CARTESIAN_POINT('Ctrl Pts',(-4.4811239675789,1.4443283423073,391.062958718335));
#43153=CARTESIAN_POINT('Ctrl Pts',(-3.24974492884238,3.40671605371881,390.983830842875));
#43154=CARTESIAN_POINT('Ctrl Pts',(-1.23149465757426,4.54422460729751,390.904702967416));
#43155=CARTESIAN_POINT('Ctrl Pts',(1.08494139143324,4.58142538413069,390.825575091955));
#43156=CARTESIAN_POINT('Ctrl Pts',(3.1386770782293,3.50931084000835,390.746447216496));
#43157=CARTESIAN_POINT('Ctrl Pts',(4.43243474978322,1.58747553118664,390.667319341036));
#43158=CARTESIAN_POINT('Ctrl Pts',(4.65295268374329,-0.718740353708034,
390.588191465577));
#43159=CARTESIAN_POINT('Ctrl Pts',(3.74683616074228,-2.85092531606077,390.509063590117));
#43160=CARTESIAN_POINT('Ctrl Pts',(1.93348610020102,-4.29280652644998,390.429935714657));
#43161=CARTESIAN_POINT('Ctrl Pts',(-0.348025192701879,-4.69525663179842,
390.350807839197));
#43162=CARTESIAN_POINT('Ctrl Pts',(-2.54526802197775,-3.96082908865047,
390.271679963737));
#43163=CARTESIAN_POINT('Ctrl Pts',(-4.12621688682536,-2.2673532093786,390.192552088278));
#43164=CARTESIAN_POINT('Ctrl Pts',(-4.70807153396599,-0.0248757765959869,
390.113424212818));
#43165=CARTESIAN_POINT('Ctrl Pts',(-4.14994561897114,2.22362490829375,390.034296337358));
#43166=CARTESIAN_POINT('Ctrl Pts',(-2.58697997173855,3.93371211440616,389.955168461898));
#43167=CARTESIAN_POINT('Ctrl Pts',(-0.397620511000842,4.69131690492484,
389.876040586439));
#43168=CARTESIAN_POINT('Ctrl Pts',(1.88801608791904,4.31299798573579,389.796912710978));
#43169=CARTESIAN_POINT('Ctrl Pts',(3.71650125536658,2.89035893827407,389.717784835519));
#43170=CARTESIAN_POINT('Ctrl Pts',(4.64509797385908,0.767867948577403,389.638656960059));
#43171=CARTESIAN_POINT('Ctrl Pts',(4.44896212165639,-1.54054938683214,389.559529084599));
#43172=CARTESIAN_POINT('Ctrl Pts',(3.17558470594392,-3.47594852501834,389.480401209139));
#43173=CARTESIAN_POINT('Ctrl Pts',(1.13329271192188,-4.56970502355534,389.40127333368));
#43174=CARTESIAN_POINT('Ctrl Pts',(-1.18340710566026,-4.55698408988609,
389.32214545822));
#43175=CARTESIAN_POINT('Ctrl Pts',(-3.21356473971502,-3.44086588475379,
389.24301758276));
#43176=CARTESIAN_POINT('Ctrl Pts',(-4.46561156725167,-1.49159971293583,
389.1638897073));
#43177=CARTESIAN_POINT('Ctrl Pts',(-4.63638544725815,0.818832313514199,
389.084761831841));
#43178=CARTESIAN_POINT('Ctrl Pts',(-3.6845363487667,2.93099782801338,389.00563395638));
#43179=CARTESIAN_POINT('Ctrl Pts',(-1.84053856736483,4.33347137468852,388.926506080921));
#43180=CARTESIAN_POINT('Ctrl Pts',(0.449114760160199,4.6866675053185,388.847378205461));
#43181=CARTESIAN_POINT('Ctrl Pts',(2.63002248068729,3.90506570037965,388.768250330001));
#43182=CARTESIAN_POINT('Ctrl Pts',(4.1741143660401,2.17791772857007,388.689122454542));
#43183=CARTESIAN_POINT('Ctrl Pts',(4.70751446239035,-0.0765764950091339,
388.609994579082));
#43184=CARTESIAN_POINT('Ctrl Pts',(4.10106888214441,-2.31252900459844,388.530866703622));
#43185=CARTESIAN_POINT('Ctrl Pts',(2.5016182517638,-3.98854139951492,388.451738828162));
#43186=CARTESIAN_POINT('Ctrl Pts',(0.296442716755053,-4.6987953869992,388.372610952703));
#43187=CARTESIAN_POINT('Ctrl Pts',(-1.98051145042811,-4.27131487576429,
388.293483077243));
#43188=CARTESIAN_POINT('Ctrl Pts',(-3.77791798536176,-2.80960710226223,
388.214355201783));
#43189=CARTESIAN_POINT('Ctrl Pts',(-4.66056504020173,-0.667600089313645,
388.135227326323));
#43190=CARTESIAN_POINT('Ctrl Pts',(-4.41473443363227,1.63605508883523,388.056099450863));
#43191=CARTESIAN_POINT('Ctrl Pts',(-3.09994992417011,3.54356696576203,387.976971575404));
#43192=CARTESIAN_POINT('Ctrl Pts',(-1.03456453032195,4.59306353165313,387.897843699944));
#43193=CARTESIAN_POINT('Ctrl Pts',(1.28132331369787,4.53042679435133,387.818715824484));
#43194=CARTESIAN_POINT('Ctrl Pts',(3.28696020658222,3.37082318930362,387.739587949024));
#43195=CARTESIAN_POINT('Ctrl Pts',(4.49671481157362,1.39503128157636,387.660460073565));
#43196=CARTESIAN_POINT('Ctrl Pts',(4.61766534005973,-0.918544054693783,
387.581332198105));
#43197=CARTESIAN_POINT('Ctrl Pts',(3.6205256500481,-3.00970935316784,387.502204322645));
#43198=CARTESIAN_POINT('Ctrl Pts',(1.74673639428721,-4.37212400808516,387.423076447185));
#43199=CARTESIAN_POINT('Ctrl Pts',(-0.549995784557234,-4.67590216002981,
387.343948571725));
#43200=CARTESIAN_POINT('Ctrl Pts',(-2.71355570823769,-3.84748902421993,
387.264820696266));
#43201=CARTESIAN_POINT('Ctrl Pts',(-4.22007362664152,-2.08747094804379,
387.185692820806));
#43202=CARTESIAN_POINT('Ctrl Pts',(-4.70477149187816,0.177993208894804,
387.106564945346));
#43203=CARTESIAN_POINT('Ctrl Pts',(-4.05028784482536,2.40035929545185,387.027437069887));
#43204=CARTESIAN_POINT('Ctrl Pts',(-2.41509492416788,4.04151863542169,386.948309194426));
#43205=CARTESIAN_POINT('Ctrl Pts',(-0.195127271563123,4.70409201877413,
386.869181318967));
#43206=CARTESIAN_POINT('Ctrl Pts',(2.0720871773402,4.22764841285371,386.790053443507));
#43207=CARTESIAN_POINT('Ctrl Pts',(3.83758046755327,2.72755064632278,386.710925568048));
#43208=CARTESIAN_POINT('Ctrl Pts',(4.67386800821896,0.567022234969233,386.631797692587));
#43209=CARTESIAN_POINT('Ctrl Pts',(4.37845679687603,-1.73080110096229,386.552669817128));
#43210=CARTESIAN_POINT('Ctrl Pts',(3.02287570396291,-3.60953997783552,386.473541941668));
#43211=CARTESIAN_POINT('Ctrl Pts',(0.935355956463039,-4.61428928524331,
386.394414066208));
#43212=CARTESIAN_POINT('Ctrl Pts',(-1.37864454889126,-4.50176582920686,
386.315286190748));
#43213=CARTESIAN_POINT('Ctrl Pts',(-3.35882939819794,-3.29921527745666,
386.236158315289));
#43214=CARTESIAN_POINT('Ctrl Pts',(-4.52573004019154,-1.29781507793296,
386.157030439828));
#43215=CARTESIAN_POINT('Ctrl Pts',(-4.59680105468898,1.01782927684972,386.077902564369));
#43216=CARTESIAN_POINT('Ctrl Pts',(-3.55483378747301,3.08702334241943,385.998774688909));
#43217=CARTESIAN_POINT('Ctrl Pts',(-1.65212313730168,4.40874647858035,385.91964681345));
#43218=CARTESIAN_POINT('Ctrl Pts',(0.650621422548117,4.66296559473944,385.84051893799));
#43219=CARTESIAN_POINT('Ctrl Pts',(2.79582891660295,3.78812579546785,385.76139106253));
#43220=CARTESIAN_POINT('Ctrl Pts',(4.26407332779252,1.99605486608223,385.68226318707));
#43221=CARTESIAN_POINT('Ctrl Pts',(4.69984389610718,-0.279327272972474,
385.603135311611));
#43222=CARTESIAN_POINT('Ctrl Pts',(3.99762608680683,-2.48707499751891,385.52400743615));
#43223=CARTESIAN_POINT('Ctrl Pts',(2.32745016540729,-4.09261922254535,385.444879560691));
#43224=CARTESIAN_POINT('Ctrl Pts',(0.0937212204902381,-4.70720434079847,
385.365751685231));
#43225=CARTESIAN_POINT('Ctrl Pts',(-2.16270074615507,-4.18201887319778,
385.286623809771));
#43226=CARTESIAN_POINT('Ctrl Pts',(-3.89546099811616,-2.64422767275401,
385.207495934311));
#43227=CARTESIAN_POINT('Ctrl Pts',(-4.6850007007776,-0.466181088114491,
385.128368058852));
#43228=CARTESIAN_POINT('Ctrl Pts',(-4.34014605663549,1.82474342861496,385.049240183392));
#43229=CARTESIAN_POINT('Ctrl Pts',(-2.94439783415696,3.67383692716674,384.970112307932));
#43230=CARTESIAN_POINT('Ctrl Pts',(-0.83571305710034,4.63337242830686,384.890984432472));
#43231=CARTESIAN_POINT('Ctrl Pts',(1.47532562085691,4.47101450295627,384.811856557013));
#43232=CARTESIAN_POINT('Ctrl Pts',(3.42913894264361,3.22607539980813,384.732728681553));
#43233=CARTESIAN_POINT('Ctrl Pts',(4.55264378010221,1.19999624361863,384.653600806093));
#43234=CARTESIAN_POINT('Ctrl Pts',(4.57380227931992,-1.11664187763583,384.574472930633));
#43235=CARTESIAN_POINT('Ctrl Pts',(3.4874912645637,-3.1629038955988,384.495345055174));
#43236=CARTESIAN_POINT('Ctrl Pts',(1.55674272936248,-4.44332178080534,384.416217179713));
#43237=CARTESIAN_POINT('Ctrl Pts',(-0.750944949374648,-4.64786381644416,
384.337089304254));
#43238=CARTESIAN_POINT('Ctrl Pts',(-2.87680390283758,-3.72700357899221,
384.257961428794));
#43239=CARTESIAN_POINT('Ctrl Pts',(-4.30609303856287,-1.90371193105537,
384.178833553335));
#43240=CARTESIAN_POINT('Ctrl Pts',(-4.69273396316942,0.380531633531783,
384.099705677874));
#43241=CARTESIAN_POINT('Ctrl Pts',(-3.94310806118005,2.5726358450156,384.020577802415));
#43242=CARTESIAN_POINT('Ctrl Pts',(-2.23872467266656,4.14181943271266,383.941449926955));
#43243=CARTESIAN_POINT('Ctrl Pts',(0.00772834932661786,4.70813090788891,
383.862322051495));
#43244=CARTESIAN_POINT('Ctrl Pts',(2.2523100811437,4.13444744452999,383.783194176035));
#43245=CARTESIAN_POINT('Ctrl Pts',(3.9515327006614,2.55967687195196,383.704066300576));
#43246=CARTESIAN_POINT('Ctrl Pts',(4.69395794849557,0.365123473577542,383.624938425116));
#43247=CARTESIAN_POINT('Ctrl Pts',(4.29982000221476,-1.91783845038001,383.545810549656));
#43248=CARTESIAN_POINT('Ctrl Pts',(2.86455275536081,-3.73642795795088,383.466682674196));
#43249=CARTESIAN_POINT('Ctrl Pts',(0.735682100664791,-4.65030409972978,
383.387554798737));
#43250=CARTESIAN_POINT('Ctrl Pts',(-1.571321636466,-4.43818709474668,383.308426923276));
#43251=CARTESIAN_POINT('Ctrl Pts',(-3.49785619221092,-3.15143751831031,
383.229299047817));
#43252=CARTESIAN_POINT('Ctrl Pts',(-4.57744353411293,-1.10162020007351,
383.150171172357));
#43253=CARTESIAN_POINT('Ctrl Pts',(-4.54867969326092,1.21493597416402,383.071043296898));
#43254=CARTESIAN_POINT('Ctrl Pts',(-3.41852935131432,3.23731577814161,382.991915421438));
#43255=CARTESIAN_POINT('Ctrl Pts',(-1.46063945964488,4.47583385997855,382.912787545978));
#43256=CARTESIAN_POINT('Ctrl Pts',(0.850919780561573,4.6306038375412,382.833659670518));
#43257=CARTESIAN_POINT('Ctrl Pts',(2.95644306681562,3.66415075643457,382.754531795058));
#43258=CARTESIAN_POINT('Ctrl Pts',(4.3461132474158,1.81048502171076,382.675403919598));
#43259=CARTESIAN_POINT('Ctrl Pts',(4.68344499450879,-0.481559297088858,
382.596276044139));
#43260=CARTESIAN_POINT('Ctrl Pts',(3.88675908298024,-2.65700210840579,382.517148168679));
#43261=CARTESIAN_POINT('Ctrl Pts',(2.14895964496101,-4.18909642017598,382.438020293219));
#43262=CARTESIAN_POINT('Ctrl Pts',(-0.109174330542496,-4.70687128980098,
382.358892417759));
#43263=CARTESIAN_POINT('Ctrl Pts',(-2.34087357288517,-4.08495621628556,
382.2797645423));
#43264=CARTESIAN_POINT('Ctrl Pts',(-4.00576953871563,-2.47393750444512,
382.20063666684));
#43265=CARTESIAN_POINT('Ctrl Pts',(-4.7007355921423,-0.263896316701532,
382.12150879138));
#43266=CARTESIAN_POINT('Ctrl Pts',(-4.25749735871386,2.01004293828431,382.04238091592));
#43267=CARTESIAN_POINT('Ctrl Pts',(-2.78337754303629,3.79728400651352,381.963253040461));
#43268=CARTESIAN_POINT('Ctrl Pts',(-0.635309535778666,4.66507643741782,
381.884125165001));
#43269=CARTESIAN_POINT('Ctrl Pts',(1.6665880206908,4.40329884773815,381.804997289541));
#43270=CARTESIAN_POINT('Ctrl Pts',(3.56494923856197,3.07533629050199,381.725869414081));
#43271=CARTESIAN_POINT('Ctrl Pts',(4.60011778664443,1.00273262747343,381.646741538621));
#43272=CARTESIAN_POINT('Ctrl Pts',(4.52144496199587,-1.31266592430991,381.567613663161));
#43273=CARTESIAN_POINT('Ctrl Pts',(3.34798006967052,-3.31022443744999,381.488485787702));
#43274=CARTESIAN_POINT('Ctrl Pts',(1.36385795297921,-4.50626761936056,381.409357912242));
#43275=CARTESIAN_POINT('Ctrl Pts',(-0.950499493547971,-4.6111936725719,
381.330230036783));
#43276=CARTESIAN_POINT('Ctrl Pts',(-3.03470942869027,-3.59959651303038,
381.251102161322));
#43277=CARTESIAN_POINT('Ctrl Pts',(-4.38411537126835,-1.71641742726257,
381.171974285863));
#43278=CARTESIAN_POINT('Ctrl Pts',(-4.67198130338802,0.582363352208024,
381.092846410403));
#43279=CARTESIAN_POINT('Ctrl Pts',(-3.82860531743164,2.74013461284959,381.013718534943));
#43280=CARTESIAN_POINT('Ctrl Pts',(-2.05819676400615,4.23442823222176,380.934590659483));
#43281=CARTESIAN_POINT('Ctrl Pts',(0.210569617479083,4.70342607142888,380.855462784024));
#43282=CARTESIAN_POINT('Ctrl Pts',(2.42835009758821,4.03356816934405,380.776334908564));
#43283=CARTESIAN_POINT('Ctrl Pts',(4.05814632781095,2.38704938266401,380.697207033104));
#43284=CARTESIAN_POINT('Ctrl Pts',(4.70533048456991,0.162546621555695,380.618079157644));
#43285=CARTESIAN_POINT('Ctrl Pts',(4.2131977783341,-2.10131407786716,380.538951282185));
#43286=CARTESIAN_POINT('Ctrl Pts',(2.7009098902828,-3.85637681480619,380.459823406725));
#43287=CARTESIAN_POINT('Ctrl Pts',(0.53464196968763,-4.67768258194704,380.380695531265));
#43288=CARTESIAN_POINT('Ctrl Pts',(-1.76108053730214,-4.36636596202583,
380.301567655805));
#43289=CARTESIAN_POINT('Ctrl Pts',(-3.63038692754518,-2.99780705341609,
380.222439780345));
#43290=CARTESIAN_POINT('Ctrl Pts',(-4.62065600907807,-0.903379443519156,
380.143311904886));
#43291=CARTESIAN_POINT('Ctrl Pts',(-4.49211073176741,1.40978634790602,380.064184029426));
#43292=CARTESIAN_POINT('Ctrl Pts',(-3.27587617866081,3.38159601893615,379.985056153966));
#43293=CARTESIAN_POINT('Ctrl Pts',(-1.26644314913044,4.53460892726404,379.905928278506));
#43294=CARTESIAN_POINT('Ctrl Pts',(1.049637849243,4.58964233450045,379.826800403046));
#43295=CARTESIAN_POINT('Ctrl Pts',(3.11156664606508,3.53337082405704,379.747672527587));
#43296=CARTESIAN_POINT('Ctrl Pts',(4.42008176412018,1.62155282729066,379.668544652127));
#43297=CARTESIAN_POINT('Ctrl Pts',(4.65834821288585,-0.682896991284513,
379.589416776667));
#43298=CARTESIAN_POINT('Ctrl Pts',(3.76867376779785,-2.82199475639389,379.510288901207));
#43299=CARTESIAN_POINT('Ctrl Pts',(1.96647817486303,-4.27779381936408,379.431161025748));
#43300=CARTESIAN_POINT('Ctrl Pts',(-0.311867127997482,-4.69779685253383,
379.352033150288));
#43301=CARTESIAN_POINT('Ctrl Pts',(-2.51469903618647,-3.9803071653586,379.272905274828));
#43302=CARTESIAN_POINT('Ctrl Pts',(-4.1086387471793,-2.29905285245449,379.193777399368));
#43303=CARTESIAN_POINT('Ctrl Pts',(-4.70774049217468,-0.0611214491085228,
379.114649523908));
#43304=CARTESIAN_POINT('Ctrl Pts',(-4.16694183125235,2.19160948806155,379.035521648449));
#43305=CARTESIAN_POINT('Ctrl Pts',(-2.61718809033458,3.91367894352783,378.956393772989));
#43306=CARTESIAN_POINT('Ctrl Pts',(-0.433726146618794,4.68811667974907,
378.877265897529));
#43307=CARTESIAN_POINT('Ctrl Pts',(1.85475530941073,4.32740558711739,378.798138022069));
#43308=CARTESIAN_POINT('Ctrl Pts',(3.69413887366186,2.91888580717067,378.71901014661));
#43309=CARTESIAN_POINT('Ctrl Pts',(4.63904866464471,0.803606782114387,378.63988227115));
#43310=CARTESIAN_POINT('Ctrl Pts',(4.46069062370475,-1.50625214781415,378.56075439569));
#43311=CARTESIAN_POINT('Ctrl Pts',(3.20225115918455,-3.45139738174314,378.48162652023));
#43312=CARTESIAN_POINT('Ctrl Pts',(1.16844028192984,-4.56084462361588,378.40249864477));
#43313=CARTESIAN_POINT('Ctrl Pts',(-1.14828881349689,-4.56595983052853,
378.323370769311));
#43314=CARTESIAN_POINT('Ctrl Pts',(-3.18697903086916,-3.46550444091513,
378.244242893851));
#43315=CARTESIAN_POINT('Ctrl Pts',(-4.45399572524721,-1.5259352714587,378.165115018391));
#43316=CARTESIAN_POINT('Ctrl Pts',(-4.64255205342532,0.783113532278959,
378.085987142931));
#43317=CARTESIAN_POINT('Ctrl Pts',(-3.7069922628433,2.90254452789652,378.006859267472));
#43318=CARTESIAN_POINT('Ctrl Pts',(-1.8738464663689,4.31917304511859,377.927731392012));
#43319=CARTESIAN_POINT('Ctrl Pts',(0.413019825360475,4.68998624700131,377.848603516552));
#43320=CARTESIAN_POINT('Ctrl Pts',(2.59988029319979,3.92519793567579,377.769475641092));
#43321=CARTESIAN_POINT('Ctrl Pts',(4.15722335104551,2.20998877434347,377.690347765632));
#43322=CARTESIAN_POINT('Ctrl Pts',(4.70796449588766,-0.0403321046239016,
377.611219890173));
#43323=CARTESIAN_POINT('Ctrl Pts',(4.11875099606982,-2.28088724087274,377.532092014713));
#43324=CARTESIAN_POINT('Ctrl Pts',(2.53225101877986,-3.9691637848658,377.452964139253));
#43325=CARTESIAN_POINT('Ctrl Pts',(0.332608926075814,-4.69637388582909,
377.373836263793));
#43326=CARTESIAN_POINT('Ctrl Pts',(-1.94756883984043,-4.28643581396986,
377.294708388333));
#43327=CARTESIAN_POINT('Ctrl Pts',(-3.75617547417524,-2.83860919825332,
377.215580512874));
#43328=CARTESIAN_POINT('Ctrl Pts',(-4.65528721285309,-0.703460971943434,
377.136452637414));
#43329=CARTESIAN_POINT('Ctrl Pts',(-4.42719922749879,1.60201853086424,377.057324761954));
#43330=CARTESIAN_POINT('Ctrl Pts',(-3.12713919846579,3.51959611413589,376.978196886494));
#43331=CARTESIAN_POINT('Ctrl Pts',(-1.06989485827222,4.58496252606164,376.899069011035));
#43332=CARTESIAN_POINT('Ctrl Pts',(1.24640657847665,4.54015715746168,376.819941135575));
#43333=CARTESIAN_POINT('Ctrl Pts',(3.26091156592763,3.39602887682211,376.740813260115));
#43334=CARTESIAN_POINT('Ctrl Pts',(4.48584150695881,1.4296091591174,376.661685384655));
#43335=CARTESIAN_POINT('Ctrl Pts',(4.62460015982963,-0.882966440516176,
376.582557509196));
#43336=CARTESIAN_POINT('Ctrl Pts',(3.64358944392086,-2.9817465244189,376.503429633736));
#43337=CARTESIAN_POINT('Ctrl Pts',(1.7803446513398,-4.35854669589912,376.424301758276));
#43338=CARTESIAN_POINT('Ctrl Pts',(-0.513980740029185,-4.67999788047178,
376.345173882816));
#43339=CARTESIAN_POINT('Ctrl Pts',(-2.68385431544624,-3.86826607229696,
376.266046007356));
#43340=CARTESIAN_POINT('Ctrl Pts',(-4.20387757931463,-2.11989849939269,
376.186918131897));
#43341=CARTESIAN_POINT('Ctrl Pts',(-4.7060023921165,0.141766919500427,376.107790256437));
#43342=CARTESIAN_POINT('Ctrl Pts',(-4.0686476489454,2.36910590400946,376.028662380977));
#43343=CARTESIAN_POINT('Ctrl Pts',(-2.44613811739875,4.02280552584175,375.949534505517));
#43344=CARTESIAN_POINT('Ctrl Pts',(-0.231337257081005,4.70245046971741,
375.870406630058));
#43345=CARTESIAN_POINT('Ctrl Pts',(2.03947802286674,4.24347544716049,375.791278754597));
#43346=CARTESIAN_POINT('Ctrl Pts',(3.81646794076225,2.75701496679917,375.712150879138));
#43347=CARTESIAN_POINT('Ctrl Pts',(4.66936407560377,0.602987532497468,375.633023003678));
#43348=CARTESIAN_POINT('Ctrl Pts',(4.39165217497973,-1.6970389500669,375.553895128218));
#43349=CARTESIAN_POINT('Ctrl Pts',(3.05057500604089,-3.58616494858208,375.474767252759));
#43350=CARTESIAN_POINT('Ctrl Pts',(0.970853006392586,-4.60694213867371,
375.395639377299));
#43351=CARTESIAN_POINT('Ctrl Pts',(-1.34394626652729,-4.51226606546036,
375.316511501839));
#43352=CARTESIAN_POINT('Ctrl Pts',(-3.33332776428957,-3.32493525307769,
375.23738362638));
#43353=CARTESIAN_POINT('Ctrl Pts',(-4.51560361732968,-1.33271151243227,
375.158255750919));
#43354=CARTESIAN_POINT('Ctrl Pts',(-4.60446635415931,0.982571567271653,
375.07912787546));
#43355=CARTESIAN_POINT('Ctrl Pts',(-3.92033033613572,2.36677696691101,375.026375958487));
#43356=CARTESIAN_POINT('Ctrl Pts',(-3.43378788736318,2.93584158412846,375.));
#43357=CARTESIAN_POINT('Ctrl Pts',(-4.51766328535307,-0.00011344722995056,
399.112583302492));
#43358=CARTESIAN_POINT('Ctrl Pts',(-4.51713673458649,0.545949625983492,
399.093346914919));
#43359=CARTESIAN_POINT('Ctrl Pts',(-4.41799450573444,1.09219871675483,399.074110527346));
#43360=CARTESIAN_POINT('Ctrl Pts',(-4.22436256903118,1.60260114106826,399.054874139773));
#43361=CARTESIAN_POINT('Ctrl Pts',(-3.95886428330821,2.3024390448317,399.028498181286));
#43362=CARTESIAN_POINT('Ctrl Pts',(-3.51572059597365,2.93488341331845,399.002122222799));
#43363=CARTESIAN_POINT('Ctrl Pts',(-2.94858141451404,3.42336635011963,398.975746264313));
#43364=CARTESIAN_POINT('Ctrl Pts',(-2.38144223305443,3.91184928692081,398.949370305826));
#43365=CARTESIAN_POINT('Ctrl Pts',(-1.69030755746978,4.25637079203641,398.92299434734));
#43366=CARTESIAN_POINT('Ctrl Pts',(-0.958850722305057,4.4152208122577,398.896618388853));
#43367=CARTESIAN_POINT('Ctrl Pts',(-0.227393887140339,4.57407083247899,
398.870242430366));
#43368=CARTESIAN_POINT('Ctrl Pts',(0.544385107604448,4.54724936780597,398.84386647188));
#43369=CARTESIAN_POINT('Ctrl Pts',(1.26304959160632,4.33800360262792,398.817490513393));
#43370=CARTESIAN_POINT('Ctrl Pts',(1.98171407560819,4.12875783744988,398.791114554907));
#43371=CARTESIAN_POINT('Ctrl Pts',(2.64726404886714,3.73708777176682,398.76473859642));
#43372=CARTESIAN_POINT('Ctrl Pts',(3.1791236295575,3.21041157417997,398.738362637933));
#43373=CARTESIAN_POINT('Ctrl Pts',(3.71098321024786,2.68373537659312,398.711986679447));
#43374=CARTESIAN_POINT('Ctrl Pts',(4.10915239836962,2.02205304710248,398.68561072096));
#43375=CARTESIAN_POINT('Ctrl Pts',(4.32542619827246,1.30547222526591,398.659234762474));
#43376=CARTESIAN_POINT('Ctrl Pts',(4.5416999981753,0.588891403429356,398.632858803987));
#43377=CARTESIAN_POINT('Ctrl Pts',(4.57607840985923,-0.182587910753133,
398.6064828455));
#43378=CARTESIAN_POINT('Ctrl Pts',(4.42439935544928,-0.915565328667223,
398.580106887014));
#43379=CARTESIAN_POINT('Ctrl Pts',(4.27272030103931,-1.64854274658133,398.553730928527));
#43380=CARTESIAN_POINT('Ctrl Pts',(3.93498378053545,-2.34301826822704,398.527354970041));
#43381=CARTESIAN_POINT('Ctrl Pts',(3.45207841102396,-2.91491409337733,398.500979011554));
#43382=CARTESIAN_POINT('Ctrl Pts',(2.96917304151247,-3.48680991852761,398.474603053068));
#43383=CARTESIAN_POINT('Ctrl Pts',(2.34109882299336,-3.93612604718246,398.448227094581));
#43384=CARTESIAN_POINT('Ctrl Pts',(1.64389457471586,-4.20846529685206,398.421851136094));
#43385=CARTESIAN_POINT('Ctrl Pts',(0.946690326438348,-4.48080454652167,
398.395475177608));
#43386=CARTESIAN_POINT('Ctrl Pts',(0.180356048402448,-4.57616691720601,
398.369099219121));
#43387=CARTESIAN_POINT('Ctrl Pts',(-0.562330762839376,-4.483007209538,398.342723260635));
#43388=CARTESIAN_POINT('Ctrl Pts',(-1.3050175740812,-4.38984750186999,398.316347302148));
#43389=CARTESIAN_POINT('Ctrl Pts',(-2.02405691852894,-4.10816571584963,
398.289971343661));
#43390=CARTESIAN_POINT('Ctrl Pts',(-2.63239713711321,-3.67206411165684,
398.263595385175));
#43391=CARTESIAN_POINT('Ctrl Pts',(-3.24073735569747,-3.23596250746405,
398.237219426688));
#43392=CARTESIAN_POINT('Ctrl Pts',(-3.73837844841825,-2.64544108509883,
398.210843468202));
#43393=CARTESIAN_POINT('Ctrl Pts',(-4.0650726929841,-1.97199227390868,398.184467509715));
#43394=CARTESIAN_POINT('Ctrl Pts',(-4.36186009740405,-1.36019354158502,
398.160506107307));
#43395=CARTESIAN_POINT('Ctrl Pts',(-4.51756632872819,-0.679955446831048,
398.1365447049));
#43396=CARTESIAN_POINT('Ctrl Pts',(-4.51805439081064,6.66898104614677E-5,
398.112583302492));
#43397=CARTESIAN_POINT('Ctrl Pts',(-1.31303618635555,-4.90075024188347,
400.));
#43398=CARTESIAN_POINT('Ctrl Pts',(-1.45291589482402,-4.85500689927294,
400.));
#43399=CARTESIAN_POINT('Ctrl Pts',(-1.59044602699472,-4.80315746369625,
400.));
#43400=CARTESIAN_POINT('Ctrl Pts',(-1.72529743087534,-4.74548509357023,
400.));
#43401=CARTESIAN_POINT('Ctrl Pts',(-1.86151474898354,-4.68722855814354,
400.));
#43402=CARTESIAN_POINT('Ctrl Pts',(-1.99499946782598,-4.62303013629637,
400.));
#43403=CARTESIAN_POINT('Ctrl Pts',(-2.12539163452376,-4.55313283560557,
400.));
#43404=CARTESIAN_POINT('Ctrl Pts',(-2.25520494367751,-4.48354583407488,
400.));
#43405=CARTESIAN_POINT('Ctrl Pts',(-2.38195370500541,-4.40830995570903,
400.));
#43406=CARTESIAN_POINT('Ctrl Pts',(-2.50525282411489,-4.32762357969483,
400.));
#43407=CARTESIAN_POINT('Ctrl Pts',(-2.6270809920476,-4.24789978736008,400.));
#43408=CARTESIAN_POINT('Ctrl Pts',(-2.74554186145885,-4.1628542844716,400.));
#43409=CARTESIAN_POINT('Ctrl Pts',(-2.86022634881304,-4.07264517835143,
400.));
#43410=CARTESIAN_POINT('Ctrl Pts',(-2.90206457395326,-4.03973585487948,
400.));
#43411=CARTESIAN_POINT('Ctrl Pts',(-2.94339980617641,-4.00613903342865,
400.));
#43412=CARTESIAN_POINT('Ctrl Pts',(-2.98421070502804,-3.97186145992605,
400.));
#43413=CARTESIAN_POINT('Ctrl Pts',(-3.00176471409307,-3.95711763283762,
400.));
#43414=CARTESIAN_POINT('Ctrl Pts',(-3.01922333710064,-3.94224634426854,
400.));
#43415=CARTESIAN_POINT('Ctrl Pts',(-3.0365678292172,-3.92726308267954,400.));
#43416=CARTESIAN_POINT('Ctrl Pts',(-3.14698675201001,-3.83187628245151,
400.));
#43417=CARTESIAN_POINT('Ctrl Pts',(-3.25293553514171,-3.73182827889012,
400.));
#43418=CARTESIAN_POINT('Ctrl Pts',(-3.35406834590596,-3.62734196551097,
400.));
#43419=CARTESIAN_POINT('Ctrl Pts',(-3.36860939901959,-3.61231873990287,
400.));
#43420=CARTESIAN_POINT('Ctrl Pts',(-3.3830508320319,-3.59720369462607,400.));
#43421=CARTESIAN_POINT('Ctrl Pts',(-3.3973915556082,-3.58199742790278,400.));
#43422=CARTESIAN_POINT('Ctrl Pts',(-3.49724054898418,-3.4761219874308,400.));
#43423=CARTESIAN_POINT('Ctrl Pts',(-3.59221081092533,-3.36582685075802,
400.));
#43424=CARTESIAN_POINT('Ctrl Pts',(-3.68210185106465,-3.25150412359693,
400.));
#43425=CARTESIAN_POINT('Ctrl Pts',(-3.77205159485829,-3.13710673758391,
400.));
#43426=CARTESIAN_POINT('Ctrl Pts',(-3.85691583765602,-3.01867577562728,
400.));
#43427=CARTESIAN_POINT('Ctrl Pts',(-3.93644802914845,-2.89657936297904,
400.));
#43428=CARTESIAN_POINT('Ctrl Pts',(-4.00696577927717,-2.78832176115549,
400.));
#43429=CARTESIAN_POINT('Ctrl Pts',(-4.07329120966267,-2.67718185514111,
400.));
#43430=CARTESIAN_POINT('Ctrl Pts',(-4.13521902572865,-2.56340683612714,
400.));
#43431=CARTESIAN_POINT('Ctrl Pts',(-4.14927174249539,-2.53758890455934,
400.));
#43432=CARTESIAN_POINT('Ctrl Pts',(-4.16309787710306,-2.511635261477,400.));
#43433=CARTESIAN_POINT('Ctrl Pts',(-4.17669478808166,-2.48554876582588,
400.));
#43434=CARTESIAN_POINT('Ctrl Pts',(-4.18567658693009,-2.46831664178184,
400.));
#43435=CARTESIAN_POINT('Ctrl Pts',(-4.19455855900594,-2.45102602806576,
400.));
#43436=CARTESIAN_POINT('Ctrl Pts',(-4.20333295387386,-2.43369188245622,
400.));
#43437=CARTESIAN_POINT('Ctrl Pts',(-4.26826574456287,-2.30541472311025,
400.));
#43438=CARTESIAN_POINT('Ctrl Pts',(-4.32740788322074,-2.17457173953832,
400.));
#43439=CARTESIAN_POINT('Ctrl Pts',(-4.38057216155237,-2.04153956135574,
400.));
#43440=CARTESIAN_POINT('Ctrl Pts',(-4.43343069026291,-1.90927245587513,
400.));
#43441=CARTESIAN_POINT('Ctrl Pts',(-4.48038018757078,-1.77484054207341,
400.));
#43442=CARTESIAN_POINT('Ctrl Pts',(-4.52118875294636,-1.63859604986007,
400.));
#43443=CARTESIAN_POINT('Ctrl Pts',(-4.53639547739945,-1.58782650105892,
400.));
#43444=CARTESIAN_POINT('Ctrl Pts',(-4.55074898869301,-1.53680513764063,
400.));
#43445=CARTESIAN_POINT('Ctrl Pts',(-4.56423545493657,-1.48554984951531,
400.));
#43446=CARTESIAN_POINT('Ctrl Pts',(-4.60065397684761,-1.34714132945246,
400.));
#43447=CARTESIAN_POINT('Ctrl Pts',(-4.63075368245775,-1.20702677925683,
400.));
#43448=CARTESIAN_POINT('Ctrl Pts',(-4.65449674508562,-1.06564398750406,
400.));
#43449=CARTESIAN_POINT('Ctrl Pts',(-4.6677938749007,-0.986463581630512,
400.));
#43450=CARTESIAN_POINT('Ctrl Pts',(-4.67909632529634,-0.906885415400295,
400.));
#43451=CARTESIAN_POINT('Ctrl Pts',(-4.68839036132626,-0.826987472477294,
400.));
#43452=CARTESIAN_POINT('Ctrl Pts',(-4.69350021378828,-0.783059656936131,
400.));
#43453=CARTESIAN_POINT('Ctrl Pts',(-4.69800287543295,-0.73903519996531,
400.));
#43454=CARTESIAN_POINT('Ctrl Pts',(-4.70189541038099,-0.69492725727482,
400.));
#43455=CARTESIAN_POINT('Ctrl Pts',(-4.70335699391325,-0.678365442534775,
400.));
#43456=CARTESIAN_POINT('Ctrl Pts',(-4.70473233460286,-0.661793969471143,
400.));
#43457=CARTESIAN_POINT('Ctrl Pts',(-4.70602072340745,-0.645222510455179,
400.));
#43458=CARTESIAN_POINT('Ctrl Pts',(-4.71697947907218,-0.504269275129255,
400.));
#43459=CARTESIAN_POINT('Ctrl Pts',(-4.72166837458957,-0.363132695636631,
400.));
#43460=CARTESIAN_POINT('Ctrl Pts',(-4.7201177742283,-0.222235244668839,
400.));
#43461=CARTESIAN_POINT('Ctrl Pts',(-4.71856870881553,-0.0814772689241232,
400.));
#43462=CARTESIAN_POINT('Ctrl Pts',(-4.71079242396856,0.0590428483946887,
400.));
#43463=CARTESIAN_POINT('Ctrl Pts',(-4.69676735600276,0.19890200600945,400.));
#43464=CARTESIAN_POINT('Ctrl Pts',(-4.68295624998761,0.33662751705272,400.));
#43465=CARTESIAN_POINT('Ctrl Pts',(-4.66308539592085,0.473712790055481,
400.));
#43466=CARTESIAN_POINT('Ctrl Pts',(-4.63708587274883,0.609740845579473,
400.));
#43467=CARTESIAN_POINT('Ctrl Pts',(-4.62194193613231,0.6889730775437,400.));
#43468=CARTESIAN_POINT('Ctrl Pts',(-4.60471782759541,0.767846329349665,
400.));
#43469=CARTESIAN_POINT('Ctrl Pts',(-4.58539250818854,0.846274698465189,
400.));
#43470=CARTESIAN_POINT('Ctrl Pts',(-4.57105296447468,0.904469184344614,
400.));
#43471=CARTESIAN_POINT('Ctrl Pts',(-4.55555640760633,0.962418671522469,
400.));
#43472=CARTESIAN_POINT('Ctrl Pts',(-4.53891410477628,1.02009082935325,400.));
#43473=CARTESIAN_POINT('Ctrl Pts',(-4.53055828962656,1.04904703181158,400.));
#43474=CARTESIAN_POINT('Ctrl Pts',(-4.52191362534324,1.07793330641511,400.));
#43475=CARTESIAN_POINT('Ctrl Pts',(-4.51298141319226,1.1067454537709,400.));
#43476=CARTESIAN_POINT('Ctrl Pts',(-4.50751626468392,1.12437408388872,400.));
#43477=CARTESIAN_POINT('Ctrl Pts',(-4.50194375351087,1.14197390912326,400.));
#43478=CARTESIAN_POINT('Ctrl Pts',(-4.49626740324529,1.15953444897625,400.));
#43479=CARTESIAN_POINT('Ctrl Pts',(-4.45341464273149,1.29210512795207,400.));
#43480=CARTESIAN_POINT('Ctrl Pts',(-4.4046021744809,1.42258699257377,400.));
#43481=CARTESIAN_POINT('Ctrl Pts',(-4.35004408840361,1.55060321390413,400.));
#43482=CARTESIAN_POINT('Ctrl Pts',(-4.29958883856276,1.66899245545036,400.));
#43483=CARTESIAN_POINT('Ctrl Pts',(-4.24421884943669,1.7852731960868,400.));
#43484=CARTESIAN_POINT('Ctrl Pts',(-4.18406982393872,1.89912668839153,400.));
#43485=CARTESIAN_POINT('Ctrl Pts',(-4.15968128005935,1.94529070966877,400.));
#43486=CARTESIAN_POINT('Ctrl Pts',(-4.13450669520302,1.99105541062324,400.));
#43487=CARTESIAN_POINT('Ctrl Pts',(-4.10855377241811,2.03639833327113,400.));
#43488=CARTESIAN_POINT('Ctrl Pts',(-4.09598731345164,2.05835347033207,400.));
#43489=CARTESIAN_POINT('Ctrl Pts',(-4.08323760980602,2.0802109712186,400.));
#43490=CARTESIAN_POINT('Ctrl Pts',(-4.07030781226104,2.10196429342508,400.));
#43491=CARTESIAN_POINT('Ctrl Pts',(-3.9998914613058,2.22043401931249,400.));
#43492=CARTESIAN_POINT('Ctrl Pts',(-3.92427608656828,2.33558378339706,400.));
#43493=CARTESIAN_POINT('Ctrl Pts',(-3.84364635340467,2.44703278518893,400.));
#43494=CARTESIAN_POINT('Ctrl Pts',(-3.76407407271829,2.55702014226977,400.));
#43495=CARTESIAN_POINT('Ctrl Pts',(-3.67961761227173,2.66340373121656,400.));
#43496=CARTESIAN_POINT('Ctrl Pts',(-3.59041821150276,2.76578232711007,400.));
#43497=CARTESIAN_POINT('Ctrl Pts',(-3.56727357293573,2.79234658178586,400.));
#43498=CARTESIAN_POINT('Ctrl Pts',(-3.5438094445685,2.81864098904491,400.));
#43499=CARTESIAN_POINT('Ctrl Pts',(-3.52002794801113,2.84465807439287,400.));
#43500=CARTESIAN_POINT('Ctrl Pts',(-3.49182454546321,2.87551274871592,400.));
#43501=CARTESIAN_POINT('Ctrl Pts',(-3.46317478144493,2.90597739162215,400.));
#43502=CARTESIAN_POINT('Ctrl Pts',(-3.43408816619831,2.93604416807489,400.));
#43503=CARTESIAN_POINT('Origin',(0.,0.,387.));
#43504=CARTESIAN_POINT('Origin',(0.,0.,374.));
#43505=CARTESIAN_POINT('',(-4.,-4.89858719658941E-16,374.));
#43506=CARTESIAN_POINT('Origin',(0.,0.,374.));
#43507=CARTESIAN_POINT('Origin',(-17.,5.,0.));
#43508=CARTESIAN_POINT('',(-16.,5.,400.));
#43509=CARTESIAN_POINT('',(-17.,4.,400.));
#43510=CARTESIAN_POINT('Origin',(-17.,5.,400.));
#43511=CARTESIAN_POINT('',(-17.,4.,0.));
#43512=CARTESIAN_POINT('',(-17.,4.,0.));
#43513=CARTESIAN_POINT('',(-16.,5.,0.));
#43514=CARTESIAN_POINT('Origin',(-17.,5.,0.));
#43515=CARTESIAN_POINT('',(-16.,5.,0.));
#43516=CARTESIAN_POINT('Origin',(-20.,4.,0.));
#43517=CARTESIAN_POINT('',(-19.,4.,400.));
#43518=CARTESIAN_POINT('',(-16.,4.,400.));
#43519=CARTESIAN_POINT('',(-19.,4.,0.));
#43520=CARTESIAN_POINT('',(-19.,4.,0.));
#43521=CARTESIAN_POINT('',(-16.,4.,0.));
#43522=CARTESIAN_POINT('Origin',(0.,0.,400.));
#43523=CARTESIAN_POINT('',(-16.,6.,400.));
#43524=CARTESIAN_POINT('',(-16.,7.,400.));
#43525=CARTESIAN_POINT('',(-15.,7.,400.));
#43526=CARTESIAN_POINT('Origin',(-15.,6.,400.));
#43527=CARTESIAN_POINT('',(-9.,7.,400.));
#43528=CARTESIAN_POINT('',(-8.,7.,400.));
#43529=CARTESIAN_POINT('',(-8.,6.,400.));
#43530=CARTESIAN_POINT('Origin',(-9.,6.,400.));
#43531=CARTESIAN_POINT('',(-8.,-6.,400.));
#43532=CARTESIAN_POINT('',(-8.,-7.,400.));
#43533=CARTESIAN_POINT('',(-9.,-7.,400.));
#43534=CARTESIAN_POINT('Origin',(-9.,-6.,400.));
#43535=CARTESIAN_POINT('',(-15.,-7.,400.));
#43536=CARTESIAN_POINT('',(-16.,-7.,400.));
#43537=CARTESIAN_POINT('',(-16.,-6.,400.));
#43538=CARTESIAN_POINT('Origin',(-15.,-6.,400.));
#43539=CARTESIAN_POINT('',(-16.,-5.,400.));
#43540=CARTESIAN_POINT('',(-16.,-4.,400.));
#43541=CARTESIAN_POINT('',(-17.,-4.,400.));
#43542=CARTESIAN_POINT('Origin',(-17.,-5.,400.));
#43543=CARTESIAN_POINT('',(-19.,-4.,400.));
#43544=CARTESIAN_POINT('',(-20.,-4.,400.));
#43545=CARTESIAN_POINT('',(-20.,-5.,400.));
#43546=CARTESIAN_POINT('Origin',(-19.,-5.,400.));
#43547=CARTESIAN_POINT('',(-20.,-19.,400.));
#43548=CARTESIAN_POINT('',(-20.,-20.,400.));
#43549=CARTESIAN_POINT('',(-19.,-20.,400.));
#43550=CARTESIAN_POINT('Origin',(-19.,-19.,400.));
#43551=CARTESIAN_POINT('',(-5.,-20.,400.));
#43552=CARTESIAN_POINT('',(-4.,-20.,400.));
#43553=CARTESIAN_POINT('',(-4.,-19.,400.));
#43554=CARTESIAN_POINT('Origin',(-5.,-19.,400.));
#43555=CARTESIAN_POINT('',(-4.,-17.,400.));
#43556=CARTESIAN_POINT('',(-4.,-16.,400.));
#43557=CARTESIAN_POINT('',(-5.,-16.,400.));
#43558=CARTESIAN_POINT('Origin',(-5.,-17.,400.));
#43559=CARTESIAN_POINT('',(-6.,-16.,400.));
#43560=CARTESIAN_POINT('',(-7.,-16.,400.));
#43561=CARTESIAN_POINT('',(-7.,-15.,400.));
#43562=CARTESIAN_POINT('Origin',(-6.,-15.,400.));
#43563=CARTESIAN_POINT('',(-7.,-9.,400.));
#43564=CARTESIAN_POINT('',(-7.,-8.,400.));
#43565=CARTESIAN_POINT('',(-6.,-8.,400.));
#43566=CARTESIAN_POINT('Origin',(-6.,-9.,400.));
#43567=CARTESIAN_POINT('',(6.,-8.,400.));
#43568=CARTESIAN_POINT('',(7.,-8.,400.));
#43569=CARTESIAN_POINT('',(7.,-9.,400.));
#43570=CARTESIAN_POINT('Origin',(6.,-9.,400.));
#43571=CARTESIAN_POINT('',(7.,-15.,400.));
#43572=CARTESIAN_POINT('',(7.,-16.,400.));
#43573=CARTESIAN_POINT('',(6.,-16.,400.));
#43574=CARTESIAN_POINT('Origin',(6.,-15.,400.));
#43575=CARTESIAN_POINT('',(5.,-16.,400.));
#43576=CARTESIAN_POINT('',(4.,-16.,400.));
#43577=CARTESIAN_POINT('',(4.,-17.,400.));
#43578=CARTESIAN_POINT('Origin',(5.,-17.,400.));
#43579=CARTESIAN_POINT('',(4.,-19.,400.));
#43580=CARTESIAN_POINT('',(4.,-20.,400.));
#43581=CARTESIAN_POINT('',(5.,-20.,400.));
#43582=CARTESIAN_POINT('Origin',(5.,-19.,400.));
#43583=CARTESIAN_POINT('',(19.,-20.,400.));
#43584=CARTESIAN_POINT('',(20.,-20.,400.));
#43585=CARTESIAN_POINT('',(20.,-19.,400.));
#43586=CARTESIAN_POINT('Origin',(19.,-19.,400.));
#43587=CARTESIAN_POINT('',(20.,-5.,400.));
#43588=CARTESIAN_POINT('',(20.,-4.,400.));
#43589=CARTESIAN_POINT('',(19.,-4.,400.));
#43590=CARTESIAN_POINT('Origin',(19.,-5.,400.));
#43591=CARTESIAN_POINT('',(17.,-4.,400.));
#43592=CARTESIAN_POINT('',(16.,-4.,400.));
#43593=CARTESIAN_POINT('',(16.,-5.,400.));
#43594=CARTESIAN_POINT('Origin',(17.,-5.,400.));
#43595=CARTESIAN_POINT('',(16.,-6.,400.));
#43596=CARTESIAN_POINT('',(16.,-7.,400.));
#43597=CARTESIAN_POINT('',(15.,-7.,400.));
#43598=CARTESIAN_POINT('Origin',(15.,-6.,400.));
#43599=CARTESIAN_POINT('',(9.,-7.,400.));
#43600=CARTESIAN_POINT('',(8.,-7.,400.));
#43601=CARTESIAN_POINT('',(8.,-6.,400.));
#43602=CARTESIAN_POINT('Origin',(9.,-6.,400.));
#43603=CARTESIAN_POINT('',(8.,6.,400.));
#43604=CARTESIAN_POINT('',(8.,7.,400.));
#43605=CARTESIAN_POINT('',(9.,7.,400.));
#43606=CARTESIAN_POINT('Origin',(9.,6.,400.));
#43607=CARTESIAN_POINT('',(15.,7.,400.));
#43608=CARTESIAN_POINT('',(16.,7.,400.));
#43609=CARTESIAN_POINT('',(16.,6.,400.));
#43610=CARTESIAN_POINT('Origin',(15.,6.,400.));
#43611=CARTESIAN_POINT('',(16.,5.,400.));
#43612=CARTESIAN_POINT('',(16.,4.,400.));
#43613=CARTESIAN_POINT('',(17.,4.,400.));
#43614=CARTESIAN_POINT('Origin',(17.,5.,400.));
#43615=CARTESIAN_POINT('',(19.,4.,400.));
#43616=CARTESIAN_POINT('',(20.,4.,400.));
#43617=CARTESIAN_POINT('',(20.,5.,400.));
#43618=CARTESIAN_POINT('Origin',(19.,5.,400.));
#43619=CARTESIAN_POINT('',(20.,19.,400.));
#43620=CARTESIAN_POINT('',(20.,20.,400.));
#43621=CARTESIAN_POINT('',(19.,20.,400.));
#43622=CARTESIAN_POINT('Origin',(19.,19.,400.));
#43623=CARTESIAN_POINT('',(5.,20.,400.));
#43624=CARTESIAN_POINT('',(4.,20.,400.));
#43625=CARTESIAN_POINT('',(4.,19.,400.));
#43626=CARTESIAN_POINT('Origin',(5.,19.,400.));
#43627=CARTESIAN_POINT('',(4.,17.,400.));
#43628=CARTESIAN_POINT('',(4.,16.,400.));
#43629=CARTESIAN_POINT('',(5.,16.,400.));
#43630=CARTESIAN_POINT('Origin',(5.,17.,400.));
#43631=CARTESIAN_POINT('',(6.,16.,400.));
#43632=CARTESIAN_POINT('',(7.,16.,400.));
#43633=CARTESIAN_POINT('',(7.,15.,400.));
#43634=CARTESIAN_POINT('Origin',(6.,15.,400.));
#43635=CARTESIAN_POINT('',(7.,9.,400.));
#43636=CARTESIAN_POINT('',(7.,8.,400.));
#43637=CARTESIAN_POINT('',(6.,8.,400.));
#43638=CARTESIAN_POINT('Origin',(6.,9.,400.));
#43639=CARTESIAN_POINT('',(-6.,8.,400.));
#43640=CARTESIAN_POINT('',(-7.,8.,400.));
#43641=CARTESIAN_POINT('',(-7.,9.,400.));
#43642=CARTESIAN_POINT('Origin',(-6.,9.,400.));
#43643=CARTESIAN_POINT('',(-7.,15.,400.));
#43644=CARTESIAN_POINT('',(-7.,16.,400.));
#43645=CARTESIAN_POINT('',(-6.,16.,400.));
#43646=CARTESIAN_POINT('Origin',(-6.,15.,400.));
#43647=CARTESIAN_POINT('',(-5.,16.,400.));
#43648=CARTESIAN_POINT('',(-4.,16.,400.));
#43649=CARTESIAN_POINT('',(-4.,17.,400.));
#43650=CARTESIAN_POINT('Origin',(-5.,17.,400.));
#43651=CARTESIAN_POINT('',(-4.,19.,400.));
#43652=CARTESIAN_POINT('',(-4.,20.,400.));
#43653=CARTESIAN_POINT('',(-5.,20.,400.));
#43654=CARTESIAN_POINT('Origin',(-5.,19.,400.));
#43655=CARTESIAN_POINT('',(-19.,20.,400.));
#43656=CARTESIAN_POINT('',(-20.,20.,400.));
#43657=CARTESIAN_POINT('',(-20.,19.,400.));
#43658=CARTESIAN_POINT('Origin',(-19.,19.,400.));
#43659=CARTESIAN_POINT('',(-20.,5.,400.));
#43660=CARTESIAN_POINT('',(-20.,4.,400.));
#43661=CARTESIAN_POINT('Origin',(-19.,5.,400.));
#43662=CARTESIAN_POINT('',(-15.,-12.,400.));
#43663=CARTESIAN_POINT('Origin',(-12.,-12.,400.));
#43664=CARTESIAN_POINT('',(9.,12.,400.));
#43665=CARTESIAN_POINT('Origin',(12.,12.,400.));
#43666=CARTESIAN_POINT('',(-15.,12.,400.));
#43667=CARTESIAN_POINT('Origin',(-12.,12.,400.));
#43668=CARTESIAN_POINT('',(9.,-12.,400.));
#43669=CARTESIAN_POINT('Origin',(12.,-12.,400.));
#43670=CARTESIAN_POINT('Origin',(-15.,6.,0.));
#43671=CARTESIAN_POINT('',(-16.,6.,0.));
#43672=CARTESIAN_POINT('',(-15.,7.,0.));
#43673=CARTESIAN_POINT('Origin',(-15.,6.,0.));
#43674=CARTESIAN_POINT('',(-15.,7.,0.));
#43675=CARTESIAN_POINT('',(-16.,6.,0.));
#43676=CARTESIAN_POINT('Origin',(-16.,7.,0.));
#43677=CARTESIAN_POINT('',(-9.,7.,0.));
#43678=CARTESIAN_POINT('',(-8.,7.,0.));
#43679=CARTESIAN_POINT('',(-9.,7.,0.));
#43680=CARTESIAN_POINT('Origin',(-9.,6.,0.));
#43681=CARTESIAN_POINT('',(-8.,6.,0.));
#43682=CARTESIAN_POINT('Origin',(-9.,6.,0.));
#43683=CARTESIAN_POINT('',(-8.,6.,0.));
#43684=CARTESIAN_POINT('Origin',(-8.,7.,0.));
#43685=CARTESIAN_POINT('',(-8.,-6.,0.));
#43686=CARTESIAN_POINT('',(-8.,-7.,0.));
#43687=CARTESIAN_POINT('',(-8.,-6.,0.));
#43688=CARTESIAN_POINT('Origin',(-9.,-6.,0.));
#43689=CARTESIAN_POINT('',(-9.,-7.,0.));
#43690=CARTESIAN_POINT('Origin',(-9.,-6.,0.));
#43691=CARTESIAN_POINT('',(-9.,-7.,0.));
#43692=CARTESIAN_POINT('Origin',(-8.,-7.,0.));
#43693=CARTESIAN_POINT('',(-15.,-7.,0.));
#43694=CARTESIAN_POINT('',(-16.,-7.,0.));
#43695=CARTESIAN_POINT('',(-15.,-7.,0.));
#43696=CARTESIAN_POINT('Origin',(-15.,-6.,0.));
#43697=CARTESIAN_POINT('',(-16.,-6.,0.));
#43698=CARTESIAN_POINT('Origin',(-15.,-6.,0.));
#43699=CARTESIAN_POINT('',(-16.,-6.,0.));
#43700=CARTESIAN_POINT('Origin',(-16.,-7.,0.));
#43701=CARTESIAN_POINT('',(-16.,-5.,0.));
#43702=CARTESIAN_POINT('',(-16.,-4.,0.));
#43703=CARTESIAN_POINT('',(-16.,-5.,0.));
#43704=CARTESIAN_POINT('Origin',(-17.,-5.,0.));
#43705=CARTESIAN_POINT('',(-17.,-4.,0.));
#43706=CARTESIAN_POINT('Origin',(-17.,-5.,0.));
#43707=CARTESIAN_POINT('',(-17.,-4.,0.));
#43708=CARTESIAN_POINT('Origin',(-19.,-5.,0.));
#43709=CARTESIAN_POINT('',(-19.,-4.,0.));
#43710=CARTESIAN_POINT('',(-19.,-4.,0.));
#43711=CARTESIAN_POINT('',(-20.,-5.,0.));
#43712=CARTESIAN_POINT('Origin',(-19.,-5.,0.));
#43713=CARTESIAN_POINT('',(-20.,-5.,0.));
#43714=CARTESIAN_POINT('Origin',(-20.,-4.,0.));
#43715=CARTESIAN_POINT('',(-20.,-19.,0.));
#43716=CARTESIAN_POINT('',(-20.,-20.,0.));
#43717=CARTESIAN_POINT('',(-20.,-19.,0.));
#43718=CARTESIAN_POINT('Origin',(-19.,-19.,0.));
#43719=CARTESIAN_POINT('',(-19.,-20.,0.));
#43720=CARTESIAN_POINT('Origin',(-19.,-19.,0.));
#43721=CARTESIAN_POINT('',(-19.,-20.,0.));
#43722=CARTESIAN_POINT('Origin',(-5.,-19.,0.));
#43723=CARTESIAN_POINT('',(-5.,-20.,0.));
#43724=CARTESIAN_POINT('',(-5.,-20.,0.));
#43725=CARTESIAN_POINT('',(-4.,-19.,0.));
#43726=CARTESIAN_POINT('Origin',(-5.,-19.,0.));
#43727=CARTESIAN_POINT('',(-4.,-19.,0.));
#43728=CARTESIAN_POINT('Origin',(-4.,-20.,0.));
#43729=CARTESIAN_POINT('',(-4.,-17.,0.));
#43730=CARTESIAN_POINT('',(-4.,-16.,0.));
#43731=CARTESIAN_POINT('',(-4.,-17.,0.));
#43732=CARTESIAN_POINT('Origin',(-5.,-17.,0.));
#43733=CARTESIAN_POINT('',(-5.,-16.,0.));
#43734=CARTESIAN_POINT('Origin',(-5.,-17.,0.));
#43735=CARTESIAN_POINT('',(-5.,-16.,0.));
#43736=CARTESIAN_POINT('Origin',(-6.,-15.,0.));
#43737=CARTESIAN_POINT('',(-6.,-16.,0.));
#43738=CARTESIAN_POINT('',(-7.,-15.,0.));
#43739=CARTESIAN_POINT('Origin',(-6.,-15.,0.));
#43740=CARTESIAN_POINT('',(-7.,-15.,0.));
#43741=CARTESIAN_POINT('',(-6.,-16.,0.));
#43742=CARTESIAN_POINT('Origin',(-7.,-16.,0.));
#43743=CARTESIAN_POINT('',(-7.,-9.,0.));
#43744=CARTESIAN_POINT('',(-7.,-8.,0.));
#43745=CARTESIAN_POINT('',(-7.,-9.,0.));
#43746=CARTESIAN_POINT('Origin',(-6.,-9.,0.));
#43747=CARTESIAN_POINT('',(-6.,-8.,0.));
#43748=CARTESIAN_POINT('Origin',(-6.,-9.,0.));
#43749=CARTESIAN_POINT('',(-6.,-8.,0.));
#43750=CARTESIAN_POINT('Origin',(-7.,-8.,0.));
#43751=CARTESIAN_POINT('',(6.,-8.,0.));
#43752=CARTESIAN_POINT('',(7.,-8.,0.));
#43753=CARTESIAN_POINT('',(6.,-8.,0.));
#43754=CARTESIAN_POINT('Origin',(6.,-9.,0.));
#43755=CARTESIAN_POINT('',(7.,-9.,0.));
#43756=CARTESIAN_POINT('Origin',(6.,-9.,0.));
#43757=CARTESIAN_POINT('',(7.,-9.,0.));
#43758=CARTESIAN_POINT('Origin',(7.,-8.,0.));
#43759=CARTESIAN_POINT('',(7.,-15.,0.));
#43760=CARTESIAN_POINT('',(7.,-16.,0.));
#43761=CARTESIAN_POINT('',(7.,-15.,0.));
#43762=CARTESIAN_POINT('Origin',(6.,-15.,0.));
#43763=CARTESIAN_POINT('',(6.,-16.,0.));
#43764=CARTESIAN_POINT('Origin',(6.,-15.,0.));
#43765=CARTESIAN_POINT('',(6.,-16.,0.));
#43766=CARTESIAN_POINT('Origin',(7.,-16.,0.));
#43767=CARTESIAN_POINT('',(5.,-16.,0.));
#43768=CARTESIAN_POINT('',(4.,-16.,0.));
#43769=CARTESIAN_POINT('',(5.,-16.,0.));
#43770=CARTESIAN_POINT('Origin',(5.,-17.,0.));
#43771=CARTESIAN_POINT('',(4.,-17.,0.));
#43772=CARTESIAN_POINT('Origin',(5.,-17.,0.));
#43773=CARTESIAN_POINT('',(4.,-17.,0.));
#43774=CARTESIAN_POINT('Origin',(5.,-19.,0.));
#43775=CARTESIAN_POINT('',(4.,-19.,0.));
#43776=CARTESIAN_POINT('',(4.,-19.,0.));
#43777=CARTESIAN_POINT('',(5.,-20.,0.));
#43778=CARTESIAN_POINT('Origin',(5.,-19.,0.));
#43779=CARTESIAN_POINT('',(5.,-20.,0.));
#43780=CARTESIAN_POINT('Origin',(4.,-20.,0.));
#43781=CARTESIAN_POINT('',(19.,-20.,0.));
#43782=CARTESIAN_POINT('',(20.,-20.,0.));
#43783=CARTESIAN_POINT('',(19.,-20.,0.));
#43784=CARTESIAN_POINT('Origin',(19.,-19.,0.));
#43785=CARTESIAN_POINT('',(20.,-19.,0.));
#43786=CARTESIAN_POINT('Origin',(19.,-19.,0.));
#43787=CARTESIAN_POINT('',(20.,-19.,0.));
#43788=CARTESIAN_POINT('Origin',(19.,-5.,0.));
#43789=CARTESIAN_POINT('',(20.,-5.,0.));
#43790=CARTESIAN_POINT('',(20.,-5.,0.));
#43791=CARTESIAN_POINT('',(19.,-4.,0.));
#43792=CARTESIAN_POINT('Origin',(19.,-5.,0.));
#43793=CARTESIAN_POINT('',(19.,-4.,0.));
#43794=CARTESIAN_POINT('Origin',(20.,-4.,0.));
#43795=CARTESIAN_POINT('',(17.,-4.,0.));
#43796=CARTESIAN_POINT('',(16.,-4.,0.));
#43797=CARTESIAN_POINT('',(17.,-4.,0.));
#43798=CARTESIAN_POINT('Origin',(17.,-5.,0.));
#43799=CARTESIAN_POINT('',(16.,-5.,0.));
#43800=CARTESIAN_POINT('Origin',(17.,-5.,0.));
#43801=CARTESIAN_POINT('',(16.,-5.,0.));
#43802=CARTESIAN_POINT('Origin',(15.,-6.,0.));
#43803=CARTESIAN_POINT('',(16.,-6.,0.));
#43804=CARTESIAN_POINT('',(15.,-7.,0.));
#43805=CARTESIAN_POINT('Origin',(15.,-6.,0.));
#43806=CARTESIAN_POINT('',(15.,-7.,0.));
#43807=CARTESIAN_POINT('',(16.,-6.,0.));
#43808=CARTESIAN_POINT('Origin',(16.,-7.,0.));
#43809=CARTESIAN_POINT('',(9.,-7.,0.));
#43810=CARTESIAN_POINT('',(8.,-7.,0.));
#43811=CARTESIAN_POINT('',(9.,-7.,0.));
#43812=CARTESIAN_POINT('Origin',(9.,-6.,0.));
#43813=CARTESIAN_POINT('',(8.,-6.,0.));
#43814=CARTESIAN_POINT('Origin',(9.,-6.,0.));
#43815=CARTESIAN_POINT('',(8.,-6.,0.));
#43816=CARTESIAN_POINT('Origin',(8.,-7.,0.));
#43817=CARTESIAN_POINT('',(8.,6.,0.));
#43818=CARTESIAN_POINT('',(8.,7.,0.));
#43819=CARTESIAN_POINT('',(8.,6.,0.));
#43820=CARTESIAN_POINT('Origin',(9.,6.,0.));
#43821=CARTESIAN_POINT('',(9.,7.,0.));
#43822=CARTESIAN_POINT('Origin',(9.,6.,0.));
#43823=CARTESIAN_POINT('',(9.,7.,0.));
#43824=CARTESIAN_POINT('Origin',(8.,7.,0.));
#43825=CARTESIAN_POINT('',(15.,7.,0.));
#43826=CARTESIAN_POINT('',(16.,7.,0.));
#43827=CARTESIAN_POINT('',(15.,7.,0.));
#43828=CARTESIAN_POINT('Origin',(15.,6.,0.));
#43829=CARTESIAN_POINT('',(16.,6.,0.));
#43830=CARTESIAN_POINT('Origin',(15.,6.,0.));
#43831=CARTESIAN_POINT('',(16.,6.,0.));
#43832=CARTESIAN_POINT('Origin',(16.,7.,0.));
#43833=CARTESIAN_POINT('',(16.,5.,0.));
#43834=CARTESIAN_POINT('',(16.,4.,0.));
#43835=CARTESIAN_POINT('',(16.,5.,0.));
#43836=CARTESIAN_POINT('Origin',(17.,5.,0.));
#43837=CARTESIAN_POINT('',(17.,4.,0.));
#43838=CARTESIAN_POINT('Origin',(17.,5.,0.));
#43839=CARTESIAN_POINT('',(17.,4.,0.));
#43840=CARTESIAN_POINT('Origin',(19.,5.,0.));
#43841=CARTESIAN_POINT('',(19.,4.,0.));
#43842=CARTESIAN_POINT('',(19.,4.,0.));
#43843=CARTESIAN_POINT('',(20.,5.,0.));
#43844=CARTESIAN_POINT('Origin',(19.,5.,0.));
#43845=CARTESIAN_POINT('',(20.,5.,0.));
#43846=CARTESIAN_POINT('Origin',(20.,4.,0.));
#43847=CARTESIAN_POINT('',(20.,19.,0.));
#43848=CARTESIAN_POINT('',(20.,20.,0.));
#43849=CARTESIAN_POINT('',(20.,19.,0.));
#43850=CARTESIAN_POINT('Origin',(19.,19.,0.));
#43851=CARTESIAN_POINT('',(19.,20.,0.));
#43852=CARTESIAN_POINT('Origin',(19.,19.,0.));
#43853=CARTESIAN_POINT('',(19.,20.,0.));
#43854=CARTESIAN_POINT('Origin',(5.,19.,0.));
#43855=CARTESIAN_POINT('',(5.,20.,0.));
#43856=CARTESIAN_POINT('',(5.,20.,0.));
#43857=CARTESIAN_POINT('',(4.,19.,0.));
#43858=CARTESIAN_POINT('Origin',(5.,19.,0.));
#43859=CARTESIAN_POINT('',(4.,19.,0.));
#43860=CARTESIAN_POINT('Origin',(4.,20.,0.));
#43861=CARTESIAN_POINT('',(4.,17.,0.));
#43862=CARTESIAN_POINT('',(4.,16.,0.));
#43863=CARTESIAN_POINT('',(4.,17.,0.));
#43864=CARTESIAN_POINT('Origin',(5.,17.,0.));
#43865=CARTESIAN_POINT('',(5.,16.,0.));
#43866=CARTESIAN_POINT('Origin',(5.,17.,0.));
#43867=CARTESIAN_POINT('',(5.,16.,0.));
#43868=CARTESIAN_POINT('Origin',(6.,15.,0.));
#43869=CARTESIAN_POINT('',(6.,16.,0.));
#43870=CARTESIAN_POINT('',(7.,15.,0.));
#43871=CARTESIAN_POINT('Origin',(6.,15.,0.));
#43872=CARTESIAN_POINT('',(7.,15.,0.));
#43873=CARTESIAN_POINT('',(6.,16.,0.));
#43874=CARTESIAN_POINT('Origin',(7.,16.,0.));
#43875=CARTESIAN_POINT('',(7.,9.,0.));
#43876=CARTESIAN_POINT('',(7.,8.,0.));
#43877=CARTESIAN_POINT('',(7.,9.,0.));
#43878=CARTESIAN_POINT('Origin',(6.,9.,0.));
#43879=CARTESIAN_POINT('',(6.,8.,0.));
#43880=CARTESIAN_POINT('Origin',(6.,9.,0.));
#43881=CARTESIAN_POINT('',(6.,8.,0.));
#43882=CARTESIAN_POINT('Origin',(7.,8.,0.));
#43883=CARTESIAN_POINT('',(-6.,8.,0.));
#43884=CARTESIAN_POINT('',(-7.,8.,0.));
#43885=CARTESIAN_POINT('',(-6.,8.,0.));
#43886=CARTESIAN_POINT('Origin',(-6.,9.,0.));
#43887=CARTESIAN_POINT('',(-7.,9.,0.));
#43888=CARTESIAN_POINT('Origin',(-6.,9.,0.));
#43889=CARTESIAN_POINT('',(-7.,9.,0.));
#43890=CARTESIAN_POINT('Origin',(-7.,8.,0.));
#43891=CARTESIAN_POINT('',(-7.,15.,0.));
#43892=CARTESIAN_POINT('',(-7.,16.,0.));
#43893=CARTESIAN_POINT('',(-7.,15.,0.));
#43894=CARTESIAN_POINT('Origin',(-6.,15.,0.));
#43895=CARTESIAN_POINT('',(-6.,16.,0.));
#43896=CARTESIAN_POINT('Origin',(-6.,15.,0.));
#43897=CARTESIAN_POINT('',(-6.,16.,0.));
#43898=CARTESIAN_POINT('Origin',(-7.,16.,0.));
#43899=CARTESIAN_POINT('',(-5.,16.,0.));
#43900=CARTESIAN_POINT('',(-4.,16.,0.));
#43901=CARTESIAN_POINT('',(-5.,16.,0.));
#43902=CARTESIAN_POINT('Origin',(-5.,17.,0.));
#43903=CARTESIAN_POINT('',(-4.,17.,0.));
#43904=CARTESIAN_POINT('Origin',(-5.,17.,0.));
#43905=CARTESIAN_POINT('',(-4.,17.,0.));
#43906=CARTESIAN_POINT('Origin',(-5.,19.,0.));
#43907=CARTESIAN_POINT('',(-4.,19.,0.));
#43908=CARTESIAN_POINT('',(-4.,19.,0.));
#43909=CARTESIAN_POINT('',(-5.,20.,0.));
#43910=CARTESIAN_POINT('Origin',(-5.,19.,0.));
#43911=CARTESIAN_POINT('',(-5.,20.,0.));
#43912=CARTESIAN_POINT('Origin',(-4.,20.,0.));
#43913=CARTESIAN_POINT('',(-19.,20.,0.));
#43914=CARTESIAN_POINT('',(-20.,20.,0.));
#43915=CARTESIAN_POINT('',(-19.,20.,0.));
#43916=CARTESIAN_POINT('Origin',(-19.,19.,0.));
#43917=CARTESIAN_POINT('',(-20.,19.,0.));
#43918=CARTESIAN_POINT('Origin',(-19.,19.,0.));
#43919=CARTESIAN_POINT('',(-20.,19.,0.));
#43920=CARTESIAN_POINT('Origin',(-19.,5.,0.));
#43921=CARTESIAN_POINT('',(-20.,5.,0.));
#43922=CARTESIAN_POINT('',(-20.,5.,0.));
#43923=CARTESIAN_POINT('Origin',(-19.,5.,0.));
#43924=CARTESIAN_POINT('Origin',(12.,-12.,0.));
#43925=CARTESIAN_POINT('',(9.,-12.,0.));
#43926=CARTESIAN_POINT('',(9.,-12.,0.));
#43927=CARTESIAN_POINT('Origin',(12.,-12.,0.));
#43928=CARTESIAN_POINT('Origin',(-12.,12.,0.));
#43929=CARTESIAN_POINT('',(-15.,12.,0.));
#43930=CARTESIAN_POINT('',(-15.,12.,0.));
#43931=CARTESIAN_POINT('Origin',(-12.,12.,0.));
#43932=CARTESIAN_POINT('Origin',(0.,0.,0.));
#43933=CARTESIAN_POINT('',(-4.,-4.89858719658941E-16,0.));
#43934=CARTESIAN_POINT('Origin',(12.,12.,0.));
#43935=CARTESIAN_POINT('',(9.,12.,0.));
#43936=CARTESIAN_POINT('',(9.,12.,0.));
#43937=CARTESIAN_POINT('Origin',(12.,12.,0.));
#43938=CARTESIAN_POINT('Origin',(-12.,-12.,0.));
#43939=CARTESIAN_POINT('',(-15.,-12.,0.));
#43940=CARTESIAN_POINT('',(-15.,-12.,0.));
#43941=CARTESIAN_POINT('Origin',(-12.,-12.,0.));
#43942=CARTESIAN_POINT('Origin',(-20.,20.,0.));
#43943=CARTESIAN_POINT('',(-20.,4.,0.));
#43944=CARTESIAN_POINT('Origin',(-4.,16.,0.));
#43945=CARTESIAN_POINT('',(-4.,20.,0.));
#43946=CARTESIAN_POINT('Origin',(4.,16.,0.));
#43947=CARTESIAN_POINT('',(7.,16.,0.));
#43948=CARTESIAN_POINT('Origin',(20.,20.,0.));
#43949=CARTESIAN_POINT('',(4.,20.,0.));
#43950=CARTESIAN_POINT('Origin',(16.,4.,0.));
#43951=CARTESIAN_POINT('',(20.,4.,0.));
#43952=CARTESIAN_POINT('Origin',(16.,-4.,0.));
#43953=CARTESIAN_POINT('',(16.,-7.,0.));
#43954=CARTESIAN_POINT('Origin',(20.,-20.,0.));
#43955=CARTESIAN_POINT('',(20.,-4.,0.));
#43956=CARTESIAN_POINT('Origin',(4.,-16.,0.));
#43957=CARTESIAN_POINT('',(4.,-20.,0.));
#43958=CARTESIAN_POINT('Origin',(-4.,-16.,0.));
#43959=CARTESIAN_POINT('',(-7.,-16.,0.));
#43960=CARTESIAN_POINT('Origin',(-20.,-20.,0.));
#43961=CARTESIAN_POINT('',(-4.,-20.,0.));
#43962=CARTESIAN_POINT('Origin',(-16.,-4.,0.));
#43963=CARTESIAN_POINT('',(-20.,-4.,0.));
#43964=CARTESIAN_POINT('Origin',(-16.,4.,0.));
#43965=CARTESIAN_POINT('',(-16.,7.,0.));
#43966=CARTESIAN_POINT('Origin',(0.,0.,0.));
#63724=UNCERTAINTY_MEASURE_WITH_UNIT(LENGTH_MEASURE(0.01),#63756,
'DISTANCE_ACCURACY_VALUE',
'Maximum model space distance between geometric entities at asserted c
onnectivities');
#63735=UNCERTAINTY_MEASURE_WITH_UNIT(LENGTH_MEASURE(0.01),#63756,
'DISTANCE_ACCURACY_VALUE',
'Maximum model space distance between geometric entities at asserted c
onnectivities');
#63744=(
GEOMETRIC_REPRESENTATION_CONTEXT(3)
GLOBAL_UNCERTAINTY_ASSIGNED_CONTEXT((#63724))
GLOBAL_UNIT_ASSIGNED_CONTEXT((#63756,#63758,#63759))
REPRESENTATION_CONTEXT('','3D')
);
#63755=(
GEOMETRIC_REPRESENTATION_CONTEXT(3)
GLOBAL_UNCERTAINTY_ASSIGNED_CONTEXT((#63735))
GLOBAL_UNIT_ASSIGNED_CONTEXT((#63756,#63758,#63759))
REPRESENTATION_CONTEXT('','3D')
);
#63756=(
LENGTH_UNIT()
NAMED_UNIT(*)
SI_UNIT(.MILLI.,.METRE.)
);
#63758=(
NAMED_UNIT(*)
PLANE_ANGLE_UNIT()
SI_UNIT($,.RADIAN.)
);
#63759=(
NAMED_UNIT(*)
SI_UNIT($,.STERADIAN.)
SOLID_ANGLE_UNIT()
);
#63768=SHAPE_DEFINITION_REPRESENTATION(#63827,#63866);
#63827=PRODUCT_DEFINITION_SHAPE('',$,#63886);
#63866=SHAPE_REPRESENTATION('',(#14741),#63744);
#63877=PRODUCT_DEFINITION_CONTEXT('part definition',#63936,'design');
#63886=PRODUCT_DEFINITION('Leg post','Leg post',#63905,#63877);
#63905=PRODUCT_DEFINITION_FORMATION('',$,#63946);
#63936=APPLICATION_CONTEXT(
'Core Data for Automotive Mechanical Design Process');
#63937=PRODUCT_CONTEXT('part definition',#63936,'mechanical');
#63946=PRODUCT('Leg post','Leg post',
'Independent aluminum extrusion section. Whole-mm nominal die dimensio
ns; parametric saw-cut length. Select structural loading, tolerances a
nd finish for the assembly application.',(#63937));
#63958=PRESENTATION_STYLE_ASSIGNMENT((#63965));
#63965=SURFACE_STYLE_USAGE(.BOTH.,#63972);
#63972=SURFACE_SIDE_STYLE('',(#63979));
#63979=SURFACE_STYLE_FILL_AREA(#63986);
#63986=FILL_AREA_STYLE('Dark blue',(#63993));
#63993=FILL_AREA_STYLE_COLOUR('Dark blue',#64000);
#64000=COLOUR_RGB('Dark blue',0.0901960784313725,0.270588235294118,0.513725490196078);
ENDSEC;
END-ISO-10303-21;
